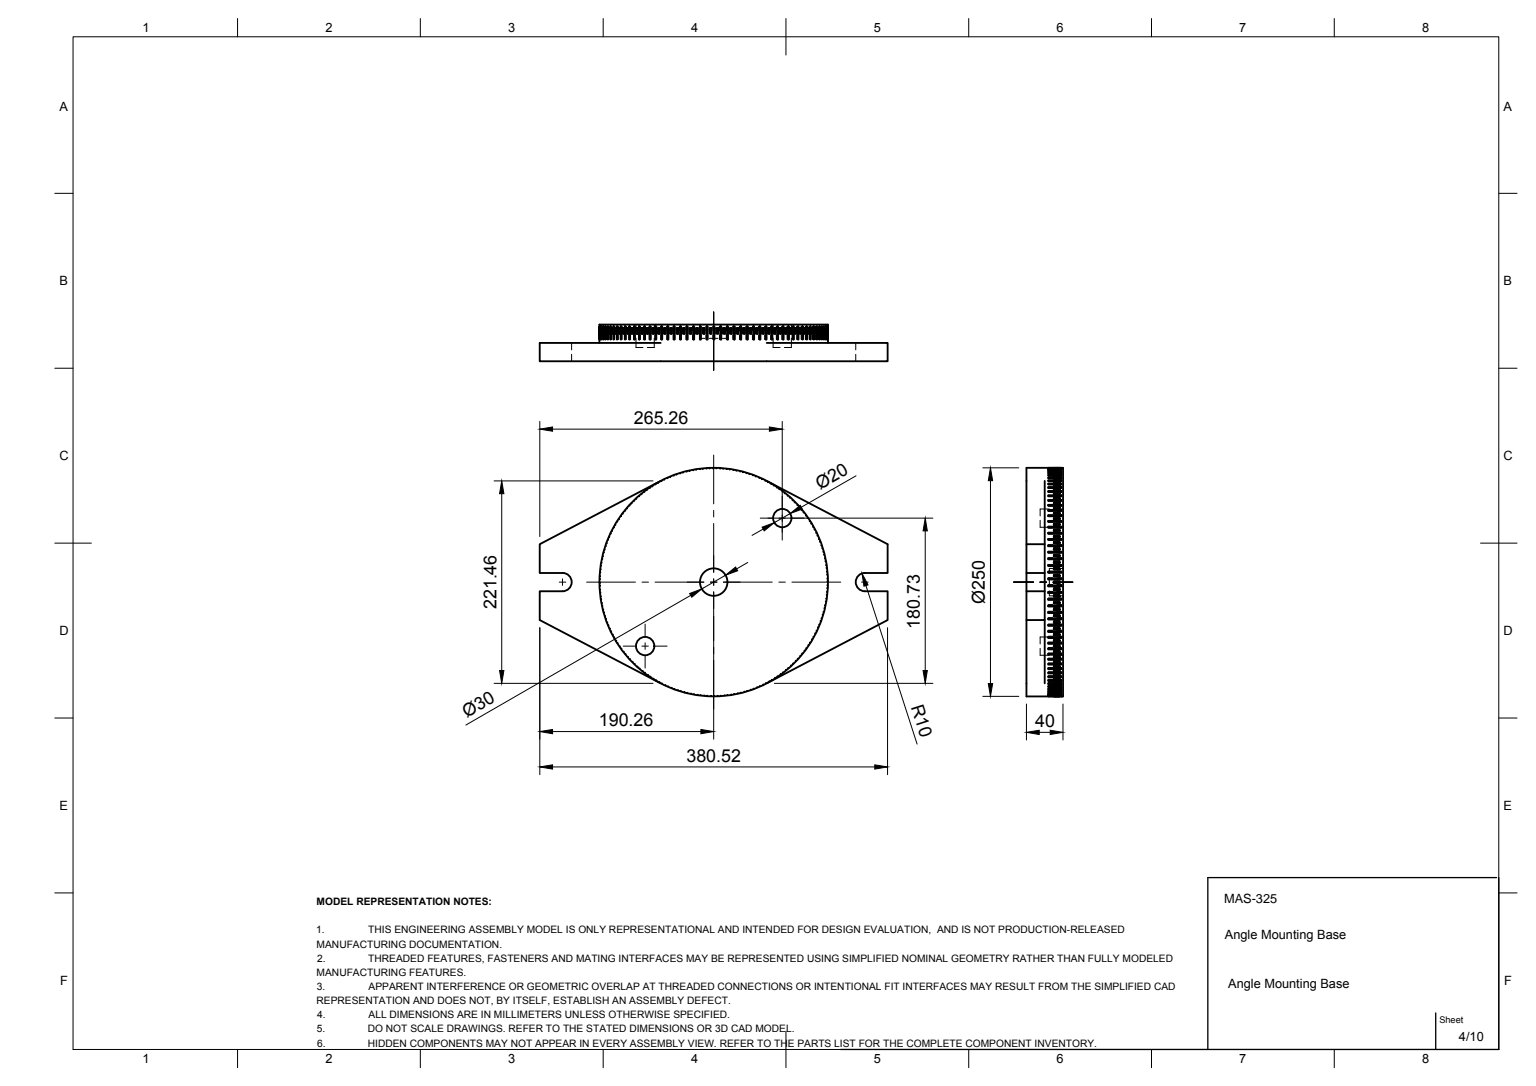
ISO-10303-21;
HEADER;
FILE_DESCRIPTION (('STEP AP214'),
    '1' );
FILE_NAME ('Angle Mounting Base.step',
    '2026-10-08T01:23:29',
    ( '' ),
    ( '' ),
    'SwSTEP 2.0',
    'SolidWorks 2025',
    '' );
FILE_SCHEMA (( 'AUTOMOTIVE_DESIGN' ));
ENDSEC;

DATA;
#2=FACE_OUTER_BOUND ( 'NONE', #26944, .T. ) ;
#3=VERTEX_POINT ( 'NONE', #17850 ) ;
#4=VERTEX_POINT ( 'NONE', #2063 ) ;
#5=EDGE_LOOP ( 'NONE', ( #45365, #39449, #49591, #6514 ) ) ;
#9=FACE_OUTER_BOUND ( 'NONE', #31225, .T. ) ;
#10=ORIENTED_EDGE ( 'NONE', *, *, #44040, .F. ) ;
#12=ORIENTED_EDGE ( 'NONE', *, *, #51700, .T. ) ;
#13=ORIENTED_EDGE ( 'NONE', *, *, #43268, .F. ) ;
#16=EDGE_CURVE ( 'NONE', #34125, #29247, #18107, .T. ) ;
#17=ADVANCED_FACE ( 'NONE', ( #34134 ), #14181, .T. ) ;
#18=ORIENTED_EDGE ( 'NONE', *, *, #15943, .T. ) ;
#19=AXIS2_PLACEMENT_3D ( 'NONE', #21420, #9597, #9087 ) ;
#21=EDGE_CURVE ( 'NONE', #1891, #35017, #9977, .T. ) ;
#22=CARTESIAN_POINT ( 'NONE',  ( -159.8192355313504720, -177.1207230881787780, -56.81883646197830018 ) ) ;
#24=CARTESIAN_POINT ( 'NONE',  ( -0.3054481938615447034, -177.1207230881787780, 115.3442529744090592 ) ) ;
#26=ORIENTED_EDGE ( 'NONE', *, *, #11216, .F. ) ;
#27=DIRECTION ( 'NONE',  ( -0.000000000000000000, 1.000000000000000000, -0.000000000000000000 ) ) ;
#28=EDGE_LOOP ( 'NONE', ( #8074, #9559, #4118, #19918 ) ) ;
#30=ORIENTED_EDGE ( 'NONE', *, *, #16889, .F. ) ;
#32=LINE ( 'NONE', #15292, #22958 ) ;
#33=CARTESIAN_POINT ( 'NONE',  ( -56.05401443572774411, -175.3837268820161057, 124.7702732086912931 ) ) ;
#34=CARTESIAN_POINT ( 'NONE',  ( 15.29189835570547551, -175.3837268820161057, 106.3450133598704213 ) ) ;
#35=VERTEX_POINT ( 'NONE', #9196 ) ;
#37=FACE_OUTER_BOUND ( 'NONE', #25266, .T. ) ;
#39=AXIS2_PLACEMENT_3D ( 'NONE', #35953, #36729, #8094 ) ;
#40=ORIENTED_EDGE ( 'NONE', *, *, #10845, .T. ) ;
#41=EDGE_CURVE ( 'NONE', #38866, #36143, #5787, .T. ) ;
#42=DIRECTION ( 'NONE',  ( -0.000000000000000000, 1.000000000000000000, -0.000000000000000000 ) ) ;
#44=DIRECTION ( 'NONE',  ( -0.8455960035018311727, 0.000000000000000000, 0.5338233779647826305 ) ) ;
#46=CARTESIAN_POINT ( 'NONE',  ( 63.31225588004632243, -183.6283474603465606, 55.92572546981597981 ) ) ;
#48=EDGE_CURVE ( 'NONE', #19235, #10210, #19545, .T. ) ;
#49=ORIENTED_EDGE ( 'NONE', *, *, #34843, .T. ) ;
#50=DIRECTION ( 'NONE',  ( -0.4031234292879665171, 0.000000000000000000, -0.9151456172430210145 ) ) ;
#51=ORIENTED_EDGE ( 'NONE', *, *, #6223, .F. ) ;
#53=CARTESIAN_POINT ( 'NONE',  ( -47.55243714407702527, -193.5000000000000000, 0.3758275821142491591 ) ) ;
#56=CARTESIAN_POINT ( 'NONE',  ( 74.95461934957533856, -175.3837268820161057, -11.83705339977243121 ) ) ;
#57=PLANE ( 'NONE',  #3915 ) ;
#58=CIRCLE ( 'NONE', #10119, 125.0000000000000000 ) ;
#61=LINE ( 'NONE', #8461, #49088 ) ;
#62=CARTESIAN_POINT ( 'NONE',  ( -135.4449840867448813, -193.5000000000000000, -88.39086586114740385 ) ) ;
#67=ORIENTED_EDGE ( 'NONE', *, *, #21766, .T. ) ;
#70=ORIENTED_EDGE ( 'NONE', *, *, #36153, .T. ) ;
#71=CARTESIAN_POINT ( 'NONE',  ( 74.13662511985246795, -189.7472609257535510, 18.47640724094593523 ) ) ;
#72=DIRECTION ( 'NONE',  ( 0.000000000000000000, 0.000000000000000000, 1.000000000000000000 ) ) ;
#73=EDGE_CURVE ( 'NONE', #1427, #18230, #29600, .T. ) ;
#74=CARTESIAN_POINT ( 'NONE',  ( -52.47502265695594303, -183.6283474603465606, -124.9361149384469627 ) ) ;
#75=DIRECTION ( 'NONE',  ( 0.000000000000000000, -0.000000000000000000, 1.000000000000000000 ) ) ;
#78=ORIENTED_EDGE ( 'NONE', *, *, #31301, .F. ) ;
#79=DIRECTION ( 'NONE',  ( -0.000000000000000000, 1.000000000000000000, -0.000000000000000000 ) ) ;
#80=DIRECTION ( 'NONE',  ( 0.6749830015182038956, 0.000000000000000000, 0.7378332790417333475 ) ) ;
#82=LINE ( 'NONE', #16386, #13659 ) ;
#83=FACE_OUTER_BOUND ( 'NONE', #49301, .T. ) ;
#85=DIRECTION ( 'NONE',  ( -0.000000000000000000, 1.000000000000000000, -0.000000000000000000 ) ) ;
#86=AXIS2_PLACEMENT_3D ( 'NONE', #8984, #303, #32633 ) ;
#88=CARTESIAN_POINT ( 'NONE',  ( -29.73468717939733708, -193.5000000000000000, 123.5865930638410930 ) ) ;
#89=DIRECTION ( 'NONE',  ( -0.2059786187411094538, 0.000000000000000000, 0.9785564922995017012 ) ) ;
#91=ORIENTED_EDGE ( 'NONE', *, *, #37914, .F. ) ;
#93=CARTESIAN_POINT ( 'NONE',  ( -171.9740864388383557, -189.7472609257535510, -11.18012358327903577 ) ) ;
#94=DIRECTION ( 'NONE',  ( -0.8757349421956412971, 0.000000000000000000, 0.4827922027307366970 ) ) ;
#97=LINE ( 'NONE', #16919, #528 ) ;
#98=DIRECTION ( 'NONE',  ( -0.9982437317643214625, 0.000000000000000000, -0.05924062789371441901 ) ) ;
#99=CARTESIAN_POINT ( 'NONE',  ( 141.7825277784304205, -193.5000000000000000, -9.999999999999987566 ) ) ;
#100=ORIENTED_EDGE ( 'NONE', *, *, #32040, .F. ) ;
#101=LINE ( 'NONE', #40291, #9133 ) ;
#102=ORIENTED_EDGE ( 'NONE', *, *, #46111, .F. ) ;
#105=LINE ( 'NONE', #39778, #22073 ) ;
#106=FACE_BOUND ( 'NONE', #42826, .T. ) ;
#108=DIRECTION ( 'NONE',  ( -0.1768902751225802927, 0.000000000000000000, 0.9842305779475953864 ) ) ;
#109=ORIENTED_EDGE ( 'NONE', *, *, #36766, .T. ) ;
#111=DIRECTION ( 'NONE',  ( 0.9785564922995032555, 0.000000000000000000, 0.2059786187411021818 ) ) ;
#112=DIRECTION ( 'NONE',  ( 0.000000000000000000, -1.000000000000000000, 0.000000000000000000 ) ) ;
#113=EDGE_CURVE ( 'NONE', #39629, #40896, #21795, .T. ) ;
#115=EDGE_LOOP ( 'NONE', ( #6615, #26573, #34341, #46200 ) ) ;
#116=CARTESIAN_POINT ( 'NONE',  ( -162.3451783319732726, -183.6283474603465606, 51.57055649762781968 ) ) ;
#117=VERTEX_POINT ( 'NONE', #22299 ) ;
#118=EDGE_LOOP ( 'NONE', ( #5505, #7567, #35660, #29019 ) ) ;
#119=CARTESIAN_POINT ( 'NONE',  ( -47.97059563285962724, -189.7472609257535510, -0.8610436117673480050 ) ) ;
#120=DIRECTION ( 'NONE',  ( 0.000000000000000000, 0.000000000000000000, -1.000000000000000000 ) ) ;
#121=VERTEX_POINT ( 'NONE', #29930 ) ;
#122=VECTOR ( 'NONE', #5953, 1000.000000000000000 ) ;
#123=ORIENTED_EDGE ( 'NONE', *, *, #8914, .F. ) ;
#124=CARTESIAN_POINT ( 'NONE',  ( 76.04209377433248562, -193.5000000000000000, -10.93003379476866677 ) ) ;
#125=CIRCLE ( 'NONE', #14436, 125.0000000000000000 ) ;
#126=AXIS2_PLACEMENT_3D ( 'NONE', #20035, #19509, #35530 ) ;
#127=EDGE_CURVE ( 'NONE', #48981, #10059, #6022, .T. ) ;
#128=CARTESIAN_POINT ( 'NONE',  ( 23.33927677392131628, -183.6283474603465606, -102.3089288139528747 ) ) ;
#130=FACE_OUTER_BOUND ( 'NONE', #50584, .T. ) ;
#131=FACE_OUTER_BOUND ( 'NONE', #2320, .T. ) ;
#134=DIRECTION ( 'NONE',  ( 0.000000000000000000, 0.000000000000000000, -1.000000000000000000 ) ) ;
#138=VERTEX_POINT ( 'NONE', #51213 ) ;
#140=EDGE_CURVE ( 'NONE', #35696, #40857, #2842, .T. ) ;
#142=FACE_OUTER_BOUND ( 'NONE', #28523, .T. ) ;
#143=FACE_OUTER_BOUND ( 'NONE', #34738, .T. ) ;
#145=AXIS2_PLACEMENT_3D ( 'NONE', #44882, #32531, #8363 ) ;
#148=CARTESIAN_POINT ( 'NONE',  ( -49.42645310536303782, -193.5000000000000000, -0.3202698538628417357 ) ) ;
#150=VERTEX_POINT ( 'NONE', #38840 ) ;
#151=DIRECTION ( 'NONE',  ( 0.000000000000000000, -0.000000000000000000, 1.000000000000000000 ) ) ;
#152=ORIENTED_EDGE ( 'NONE', *, *, #45435, .F. ) ;
#157=VECTOR ( 'NONE', #9488, 1000.000000000000000 ) ;
#159=CARTESIAN_POINT ( 'NONE',  ( -84.53143451966467126, -175.3837268820161057, -118.6432945265036807 ) ) ;
#162=AXIS2_PLACEMENT_3D ( 'NONE', #7997, #20089, #36113 ) ;
#163=ORIENTED_EDGE ( 'NONE', *, *, #20136, .T. ) ;
#165=ORIENTED_EDGE ( 'NONE', *, *, #4140, .T. ) ;
#166=DIRECTION ( 'NONE',  ( 0.000000000000000000, -0.000000000000000000, 1.000000000000000000 ) ) ;
#167=CARTESIAN_POINT ( 'NONE',  ( -139.0630283577175987, -193.5000000000000000, -86.13684908212448477 ) ) ;
#168=CARTESIAN_POINT ( 'NONE',  ( -15.24927435600541692, -177.1207230881787780, 120.5021863277719234 ) ) ;
#170=CARTESIAN_POINT ( 'NONE',  ( -144.0067397530739299, -183.6283474603465606, -80.61932246194588458 ) ) ;
#171=CARTESIAN_POINT ( 'NONE',  ( -41.24387117724851493, -189.7472609257535510, 124.7904286264581231 ) ) ;
#172=VERTEX_POINT ( 'NONE', #26760 ) ;
#173=DIRECTION ( 'NONE',  ( -0.8896570909947467687, 0.000000000000000000, -0.4566292373937140270 ) ) ;
#174=CARTESIAN_POINT ( 'NONE',  ( -134.9734323446613473, -175.3837268820161057, 88.85232316304892208 ) ) ;
#175=CIRCLE ( 'NONE', #31206, 125.0000000000000000 ) ;
#176=FACE_BOUND ( 'NONE', #45465, .T. ) ;
#177=VERTEX_POINT ( 'NONE', #42529 ) ;
#180=DIRECTION ( 'NONE',  ( -0.000000000000000000, 1.000000000000000000, -0.000000000000000000 ) ) ;
#183=ORIENTED_EDGE ( 'NONE', *, *, #47786, .F. ) ;
#185=DIRECTION ( 'NONE',  ( 0.4827922027307366970, 0.000000000000000000, 0.8757349421956412971 ) ) ;
#187=CARTESIAN_POINT ( 'NONE',  ( -148.0127667507368585, -183.6283474603465606, -75.61781872352626976 ) ) ;
#188=CARTESIAN_POINT ( 'NONE',  ( -48.47912675150885065, -193.5000000000000000, 6.938893903907228378E-15 ) ) ;
#189=DIRECTION ( 'NONE',  ( 0.000000000000000000, 0.000000000000000000, 1.000000000000000000 ) ) ;
#192=ADVANCED_FACE ( 'NONE', ( #46484 ), #50954, .F. ) ;
#193=FACE_OUTER_BOUND ( 'NONE', #27346, .T. ) ;
#194=VERTEX_POINT ( 'NONE', #14955 ) ;
#195=EDGE_CURVE ( 'NONE', #34486, #40282, #15361, .T. ) ;
#202=EDGE_CURVE ( 'NONE', #8838, #28521, #30963, .T. ) ;
#203=AXIS2_PLACEMENT_3D ( 'NONE', #1568, #37299, #37818 ) ;
#204=AXIS2_PLACEMENT_3D ( 'NONE', #4568, #29258, #44511 ) ;
#205=CARTESIAN_POINT ( 'NONE',  ( -157.8637630444124795, -175.3837268820161057, -60.49794494914009135 ) ) ;
#207=ORIENTED_EDGE ( 'NONE', *, *, #866, .T. ) ;
#209=DIRECTION ( 'NONE',  ( 0.000000000000000000, 0.000000000000000000, 1.000000000000000000 ) ) ;
#210=VERTEX_POINT ( 'NONE', #34890 ) ;
#211=AXIS2_PLACEMENT_3D ( 'NONE', #44344, #36428, #28543 ) ;
#212=AXIS2_PLACEMENT_3D ( 'NONE', #15523, #6858, #2909 ) ;
#213=EDGE_LOOP ( 'NONE', ( #16091, #33158, #8108, #2239 ) ) ;
#215=ORIENTED_EDGE ( 'NONE', *, *, #9578, .T. ) ;
#219=DIRECTION ( 'NONE',  ( 0.000000000000000000, 1.000000000000000000, 0.000000000000000000 ) ) ;
#220=ORIENTED_EDGE ( 'NONE', *, *, #16410, .F. ) ;
#223=ORIENTED_EDGE ( 'NONE', *, *, #649, .T. ) ;
#224=ORIENTED_EDGE ( 'NONE', *, *, #48940, .F. ) ;
#225=FACE_OUTER_BOUND ( 'NONE', #49522, .T. ) ;
#226=DIRECTION ( 'NONE',  ( -0.9890401873221633666, 0.000000000000000000, -0.1476465640024850756 ) ) ;
#227=FACE_OUTER_BOUND ( 'NONE', #2223, .T. ) ;
#229=FACE_OUTER_BOUND ( 'NONE', #4833, .T. ) ;
#230=CIRCLE ( 'NONE', #6149, 125.0000000000000000 ) ;
#234=CARTESIAN_POINT ( 'NONE',  ( -47.82630463331833681, -177.1207230881787780, 0.7575112421616305713 ) ) ;
#236=ADVANCED_FACE ( 'NONE', ( #38589 ), #47005, .T. ) ;
#238=ORIENTED_EDGE ( 'NONE', *, *, #26470, .F. ) ;
#239=CARTESIAN_POINT ( 'NONE',  ( 74.49773146996551532, -183.6283474603465606, -22.39848972532281834 ) ) ;
#241=FACE_OUTER_BOUND ( 'NONE', #10500, .T. ) ;
#243=EDGE_CURVE ( 'NONE', #48355, #27011, #50682, .T. ) ;
#244=ORIENTED_EDGE ( 'NONE', *, *, #45271, .T. ) ;
#245=EDGE_CURVE ( 'NONE', #35901, #35187, #7056, .T. ) ;
#246=VERTEX_POINT ( 'NONE', #50438 ) ;
#247=CIRCLE ( 'NONE', #6976, 125.0000000000000000 ) ;
#248=EDGE_LOOP ( 'NONE', ( #15059, #26707, #42311, #35212 ) ) ;
#249=CIRCLE ( 'NONE', #45592, 125.0000000000000000 ) ;
#251=LINE ( 'NONE', #40705, #46952 ) ;
#252=AXIS2_PLACEMENT_3D ( 'NONE', #33154, #25277, #24755 ) ;
#253=ADVANCED_FACE ( 'NONE', ( #3105 ), #7314, .F. ) ;
#255=CARTESIAN_POINT ( 'NONE',  ( -157.8637630444124795, -175.3837268820161057, -60.49794494914009846 ) ) ;
#257=EDGE_LOOP ( 'NONE', ( #21171, #20586, #46600, #11240 ) ) ;
#258=AXIS2_PLACEMENT_3D ( 'NONE', #32515, #48563, #24621 ) ;
#263=ORIENTED_EDGE ( 'NONE', *, *, #26885, .T. ) ;
#265=VERTEX_POINT ( 'NONE', #44078 ) ;
#266=CARTESIAN_POINT ( 'NONE',  ( -111.6834028793037987, -175.3837268820161057, 106.6827995071088253 ) ) ;
#267=VECTOR ( 'NONE', #9756, 1000.000000000000000 ) ;
#268=EDGE_CURVE ( 'NONE', #19322, #4539, #40375, .T. ) ;
#270=ADVANCED_FACE ( 'NONE', ( #39602 ), #440, .T. ) ;
#271=AXIS2_PLACEMENT_3D ( 'NONE', #37551, #38049, #18093 ) ;
#272=CARTESIAN_POINT ( 'NONE',  ( -102.9981419485577732, -193.5000000000000000, -111.3726929437936377 ) ) ;
#273=LINE ( 'NONE', #29176, #44951 ) ;
#274=DIRECTION ( 'NONE',  ( -0.6300878435817094392, 0.000000000000000000, -0.7765238627180437447 ) ) ;
#275=DIRECTION ( 'NONE',  ( 0.000000000000000000, 0.000000000000000000, -1.000000000000000000 ) ) ;
#278=ORIENTED_EDGE ( 'NONE', *, *, #14380, .F. ) ;
#280=ORIENTED_EDGE ( 'NONE', *, *, #40635, .T. ) ;
#281=DIRECTION ( 'NONE',  ( 0.000000000000000000, 0.000000000000000000, 1.000000000000000000 ) ) ;
#282=CARTESIAN_POINT ( 'NONE',  ( -117.6201219941651601, -193.5000000000000000, 104.1370384486469902 ) ) ;
#283=DIRECTION ( 'NONE',  ( 0.9785564922995060311, 0.000000000000000000, -0.2059786187410889424 ) ) ;
#285=VECTOR ( 'NONE', #4558, 999.9999999999998863 ) ;
#287=EDGE_LOOP ( 'NONE', ( #13570, #29381, #45686, #19106 ) ) ;
#291=( NAMED_UNIT ( * ) SI_UNIT ( $, .STERADIAN. ) SOLID_ANGLE_UNIT ( ) );
#292=ORIENTED_EDGE ( 'NONE', *, *, #4293, .T. ) ;
#293=DIRECTION ( 'NONE',  ( -0.7378332790417285736, 0.000000000000000000, 0.6749830015182091136 ) ) ;
#294=DIRECTION ( 'NONE',  ( 0.000000000000000000, 1.000000000000000000, 0.000000000000000000 ) ) ;
#297=PLANE ( 'NONE',  #12496 ) ;
#299=ORIENTED_EDGE ( 'NONE', *, *, #48513, .F. ) ;
#300=DIRECTION ( 'NONE',  ( -0.000000000000000000, 1.000000000000000000, -0.000000000000000000 ) ) ;
#302=LINE ( 'NONE', #51846, #44972 ) ;
#303=DIRECTION ( 'NONE',  ( 0.000000000000000000, -1.000000000000000000, -0.000000000000000000 ) ) ;
#307=DIRECTION ( 'NONE',  ( 0.000000000000000000, 1.000000000000000000, 0.000000000000000000 ) ) ;
#309=ADVANCED_FACE ( 'NONE', ( #15976 ), #8082, .T. ) ;
#310=AXIS2_PLACEMENT_3D ( 'NONE', #50252, #42607, #38132 ) ;
#311=EDGE_CURVE ( 'NONE', #37290, #775, #44603, .T. ) ;
#312=DIRECTION ( 'NONE',  ( -0.000000000000000000, 1.000000000000000000, -0.000000000000000000 ) ) ;
#313=EDGE_CURVE ( 'NONE', #8692, #47336, #37219, .T. ) ;
#317=EDGE_LOOP ( 'NONE', ( #32171, #36986, #20388, #10523 ) ) ;
#318=EDGE_LOOP ( 'NONE', ( #38235, #13867, #475, #2486 ) ) ;
#319=CARTESIAN_POINT ( 'NONE',  ( 52.36832552120769435, -189.7472609257535510, -72.15117186584490128 ) ) ;
#320=CARTESIAN_POINT ( 'NONE',  ( -41.24387117724851493, -189.7472609257535510, 124.7904286264581231 ) ) ;
#321=EDGE_LOOP ( 'NONE', ( #34166, #26853, #15993, #21976 ) ) ;
#322=EDGE_LOOP ( 'NONE', ( #10542, #48454, #37812, #15490 ) ) ;
#323=EDGE_CURVE ( 'NONE', #36975, #28008, #47779, .T. ) ;
#324=ORIENTED_EDGE ( 'NONE', *, *, #11588, .T. ) ;
#326=DIRECTION ( 'NONE',  ( 0.000000000000000000, 0.000000000000000000, 1.000000000000000000 ) ) ;
#327=CARTESIAN_POINT ( 'NONE',  ( -66.64622755927948106, -193.5000000000000000, 123.6727797384707515 ) ) ;
#328=ORIENTED_EDGE ( 'NONE', *, *, #49475, .F. ) ;
#330=EDGE_CURVE ( 'NONE', #27930, #47785, #15401, .T. ) ;
#331=ORIENTED_EDGE ( 'NONE', *, *, #18307, .T. ) ;
#332=DIRECTION ( 'NONE',  ( 0.000000000000000000, 0.000000000000000000, -1.000000000000000000 ) ) ;
#334=DIRECTION ( 'NONE',  ( 0.000000000000000000, -1.000000000000000000, 0.000000000000000000 ) ) ;
#335=EDGE_LOOP ( 'NONE', ( #354, #13466, #39178, #31091 ) ) ;
#337=CARTESIAN_POINT ( 'NONE',  ( -84.19171550243321178, -175.3837268820161057, 119.7898618611247485 ) ) ;
#341=VECTOR ( 'NONE', #5496, 1000.000000000000000 ) ;
#342=DIRECTION ( 'NONE',  ( 0.000000000000000000, 0.000000000000000000, -1.000000000000000000 ) ) ;
#345=VECTOR ( 'NONE', #6207, 1000.000000000000000 ) ;
#346=VERTEX_POINT ( 'NONE', #3887 ) ;
#347=ORIENTED_EDGE ( 'NONE', *, *, #7630, .T. ) ;
#348=EDGE_LOOP ( 'NONE', ( #40499, #34840, #43093, #48028 ) ) ;
#351=ORIENTED_EDGE ( 'NONE', *, *, #10876, .T. ) ;
#352=DIRECTION ( 'NONE',  ( 0.000000000000000000, 0.000000000000000000, 1.000000000000000000 ) ) ;
#354=ORIENTED_EDGE ( 'NONE', *, *, #40714, .F. ) ;
#355=CARTESIAN_POINT ( 'NONE',  ( -59.28786813212836648, -183.6283474603465606, 124.5318076226587465 ) ) ;
#357=CARTESIAN_POINT ( 'NONE',  ( 27.50603775690333563, -175.3837268820161057, -99.25348746834811209 ) ) ;
#360=ORIENTED_EDGE ( 'NONE', *, *, #30567, .T. ) ;
#361=FACE_BOUND ( 'NONE', #24793, .T. ) ;
#362=DIRECTION ( 'NONE',  ( 0.000000000000000000, -1.000000000000000000, 0.000000000000000000 ) ) ;
#363=ORIENTED_EDGE ( 'NONE', *, *, #47489, .F. ) ;
#370=ORIENTED_EDGE ( 'NONE', *, *, #34030, .F. ) ;
#375=DIRECTION ( 'NONE',  ( -0.000000000000000000, 1.000000000000000000, -0.000000000000000000 ) ) ;
#377=CIRCLE ( 'NONE', #16331, 125.0000000000000000 ) ;
#380=CARTESIAN_POINT ( 'NONE',  ( 67.66641500972446011, -193.5000000000000000, 46.20836643931067300 ) ) ;
#381=AXIS2_PLACEMENT_3D ( 'NONE', #38755, #31139, #39013 ) ;
#382=CARTESIAN_POINT ( 'NONE',  ( 67.29303306501927295, -175.3837268820161057, 47.13604789772129777 ) ) ;
#384=LINE ( 'NONE', #24315, #19709 ) ;
#385=EDGE_CURVE ( 'NONE', #3976, #38174, #2777, .T. ) ;
#388=PLANE ( 'NONE',  #37573 ) ;
#389=DIRECTION ( 'NONE',  ( -0.4566292373937018145, 0.000000000000000000, -0.8896570909947529859 ) ) ;
#390=AXIS2_PLACEMENT_3D ( 'NONE', #5869, #10563, #18713 ) ;
#391=LINE ( 'NONE', #24573, #45885 ) ;
#393=ORIENTED_EDGE ( 'NONE', *, *, #9573, .T. ) ;
#394=EDGE_CURVE ( 'NONE', #38668, #51204, #28813, .T. ) ;
#396=DIRECTION ( 'NONE',  ( -0.000000000000000000, 1.000000000000000000, -0.000000000000000000 ) ) ;
#397=CARTESIAN_POINT ( 'NONE',  ( -105.4063847101408840, -189.7472609257535510, -111.2847127925096657 ) ) ;
#404=DIRECTION ( 'NONE',  ( 0.000000000000000000, -0.000000000000000000, -1.000000000000000000 ) ) ;
#405=ORIENTED_EDGE ( 'NONE', *, *, #47135, .T. ) ;
#406=ORIENTED_EDGE ( 'NONE', *, *, #20390, .F. ) ;
#408=DIRECTION ( 'NONE',  ( 0.000000000000000000, 0.000000000000000000, -1.000000000000000000 ) ) ;
#409=DIRECTION ( 'NONE',  ( -0.000000000000000000, 1.000000000000000000, -0.000000000000000000 ) ) ;
#410=VECTOR ( 'NONE', #3277, 1000.000000000000000 ) ;
#411=VECTOR ( 'NONE', #28290, 1000.000000000000114 ) ;
#413=CARTESIAN_POINT ( 'NONE',  ( 61.38599058177058510, -189.7472609257535510, 59.62093586438192716 ) ) ;
#414=ORIENTED_EDGE ( 'NONE', *, *, #28899, .F. ) ;
#415=CARTESIAN_POINT ( 'NONE',  ( -161.6832731452239500, -175.3837268820161057, -53.00774697410101055 ) ) ;
#416=ORIENTED_EDGE ( 'NONE', *, *, #12405, .T. ) ;
#417=AXIS2_PLACEMENT_3D ( 'NONE', #40245, #307, #23211 ) ;
#418=ADVANCED_FACE ( 'NONE', ( #4154 ), #32244, .T. ) ;
#419=ORIENTED_EDGE ( 'NONE', *, *, #11216, .T. ) ;
#420=CARTESIAN_POINT ( 'NONE',  ( -58.17235712592530916, -183.6283474603465606, 123.6213615703899649 ) ) ;
#421=AXIS2_PLACEMENT_3D ( 'NONE', #37260, #26195, #17811 ) ;
#423=PLANE ( 'NONE',  #17324 ) ;
#424=VECTOR ( 'NONE', #5391, 999.9999999999998863 ) ;
#425=DIRECTION ( 'NONE',  ( 0.000000000000000000, -1.000000000000000000, 0.000000000000000000 ) ) ;
#426=DIRECTION ( 'NONE',  ( 0.000000000000000000, -1.000000000000000000, 0.000000000000000000 ) ) ;
#427=CARTESIAN_POINT ( 'NONE',  ( -172.9089226952081617, -175.3837268820161057, 11.92584929509620117 ) ) ;
#429=ORIENTED_EDGE ( 'NONE', *, *, #25783, .T. ) ;
#430=VECTOR ( 'NONE', #3916, 1000.000000000000227 ) ;
#432=DIRECTION ( 'NONE',  ( -0.6528221181905227155, 0.000000000000000000, 0.7575112421616191360 ) ) ;
#433=AXIS2_PLACEMENT_3D ( 'NONE', #44101, #16519, #40659 ) ;
#434=FACE_BOUND ( 'NONE', #5358, .T. ) ;
#435=ORIENTED_EDGE ( 'NONE', *, *, #51093, .T. ) ;
#436=EDGE_CURVE ( 'NONE', #23558, #41176, #21468, .T. ) ;
#437=DIRECTION ( 'NONE',  ( -0.000000000000000000, 1.000000000000000000, -0.000000000000000000 ) ) ;
#439=EDGE_LOOP ( 'NONE', ( #48444, #5234, #33273, #2136 ) ) ;
#440=PLANE ( 'NONE',  #29634 ) ;
#441=ORIENTED_EDGE ( 'NONE', *, *, #34593, .F. ) ;
#442=LINE ( 'NONE', #40137, #35182 ) ;
#444=FACE_BOUND ( 'NONE', #2815, .T. ) ;
#447=EDGE_CURVE ( 'NONE', #41848, #50197, #50115, .T. ) ;
#450=DIRECTION ( 'NONE',  ( -0.000000000000000000, 1.000000000000000000, -0.000000000000000000 ) ) ;
#451=ORIENTED_EDGE ( 'NONE', *, *, #12405, .F. ) ;
#452=ORIENTED_EDGE ( 'NONE', *, *, #45255, .T. ) ;
#454=ORIENTED_EDGE ( 'NONE', *, *, #27223, .T. ) ;
#455=CIRCLE ( 'NONE', #14742, 125.0000000000000000 ) ;
#457=VECTOR ( 'NONE', #6292, 1000.000000000000000 ) ;
#459=LINE ( 'NONE', #16516, #47341 ) ;
#460=CIRCLE ( 'NONE', #37427, 125.0000000000000000 ) ;
#461=VECTOR ( 'NONE', #50848, 1000.000000000000000 ) ;
#462=DIRECTION ( 'NONE',  ( -0.000000000000000000, 1.000000000000000000, -0.000000000000000000 ) ) ;
#463=ORIENTED_EDGE ( 'NONE', *, *, #19689, .T. ) ;
#464=LINE ( 'NONE', #17047, #51738 ) ;
#465=DIRECTION ( 'NONE',  ( -0.000000000000000000, 1.000000000000000000, -0.000000000000000000 ) ) ;
#466=ORIENTED_EDGE ( 'NONE', *, *, #5475, .F. ) ;
#467=VERTEX_POINT ( 'NONE', #40910 ) ;
#468=DIRECTION ( 'NONE',  ( 0.000000000000000000, 0.000000000000000000, 1.000000000000000000 ) ) ;
#470=LINE ( 'NONE', #12822, #33168 ) ;
#471=VERTEX_POINT ( 'NONE', #25411 ) ;
#472=EDGE_CURVE ( 'NONE', #25437, #18236, #29078, .T. ) ;
#474=DIRECTION ( 'NONE',  ( 0.000000000000000000, 1.000000000000000000, 0.000000000000000000 ) ) ;
#475=ORIENTED_EDGE ( 'NONE', *, *, #47971, .T. ) ;
#476=CARTESIAN_POINT ( 'NONE',  ( -111.3904503173946523, -193.5000000000000000, -106.8558168688113312 ) ) ;
#477=CARTESIAN_POINT ( 'NONE',  ( -171.2727421180348415, -193.5000000000000000, 23.38221600314377113 ) ) ;
#478=ORIENTED_EDGE ( 'NONE', *, *, #41754, .F. ) ;
#480=DIRECTION ( 'NONE',  ( -0.9982437317643222396, 0.000000000000000000, 0.05924062789370006937 ) ) ;
#481=PLANE ( 'NONE',  #41527 ) ;
#482=DIRECTION ( 'NONE',  ( 0.000000000000000000, 0.000000000000000000, 1.000000000000000000 ) ) ;
#484=DIRECTION ( 'NONE',  ( -0.000000000000000000, 1.000000000000000000, 0.000000000000000000 ) ) ;
#485=AXIS2_PLACEMENT_3D ( 'NONE', #11794, #47566, #31787 ) ;
#486=PLANE ( 'NONE',  #22221 ) ;
#487=VECTOR ( 'NONE', #43426, 1000.000000000000000 ) ;
#489=DIRECTION ( 'NONE',  ( 0.000000000000000000, 0.000000000000000000, -1.000000000000000000 ) ) ;
#490=EDGE_CURVE ( 'NONE', #1315, #121, #1960, .T. ) ;
#492=LINE ( 'NONE', #31262, #6402 ) ;
#493=EDGE_CURVE ( 'NONE', #46777, #16167, #41946, .T. ) ;
#494=DIRECTION ( 'NONE',  ( 0.7378332790417285736, 0.000000000000000000, -0.6749830015182091136 ) ) ;
#496=EDGE_LOOP ( 'NONE', ( #18205, #42343, #51625, #42919 ) ) ;
#498=DIRECTION ( 'NONE',  ( 0.7175072570443249420, 0.000000000000000000, 0.6965510290630033685 ) ) ;
#501=CARTESIAN_POINT ( 'NONE',  ( -47.51449116960048968, -175.3837268820161057, 0.2635871660690785045 ) ) ;
#502=CARTESIAN_POINT ( 'NONE',  ( 3.652658254809377336, -183.6283474603465606, -112.5098962032389522 ) ) ;
#503=VERTEX_POINT ( 'NONE', #45393 ) ;
#507=AXIS2_PLACEMENT_3D ( 'NONE', #38992, #47165, #35568 ) ;
#508=LINE ( 'NONE', #40199, #762 ) ;
#512=VERTEX_POINT ( 'NONE', #41693 ) ;
#514=DIRECTION ( 'NONE',  ( -0.000000000000000000, 1.000000000000000000, -0.000000000000000000 ) ) ;
#515=EDGE_LOOP ( 'NONE', ( #35303, #20587, #15349, #40172 ) ) ;
#516=DIRECTION ( 'NONE',  ( -0.000000000000000000, 1.000000000000000000, -0.000000000000000000 ) ) ;
#517=ORIENTED_EDGE ( 'NONE', *, *, #50630, .F. ) ;
#518=AXIS2_PLACEMENT_3D ( 'NONE', #30428, #18860, #10727 ) ;
#520=EDGE_LOOP ( 'NONE', ( #44694, #25345, #12703, #2844 ) ) ;
#523=CARTESIAN_POINT ( 'NONE',  ( -48.65601702663143868, -175.3837268820161057, 0.9842305779476024918 ) ) ;
#524=DIRECTION ( 'NONE',  ( 0.000000000000000000, 1.000000000000000000, 0.000000000000000000 ) ) ;
#525=DIRECTION ( 'NONE',  ( 0.9564009842765244240, 0.000000000000000000, -0.2920567706369695538 ) ) ;
#528=VECTOR ( 'NONE', #5098, 1000.000000000000000 ) ;
#530=VECTOR ( 'NONE', #17595, 1000.000000000000114 ) ;
#532=VECTOR ( 'NONE', #16412, 1000.000000000000000 ) ;
#533=ORIENTED_EDGE ( 'NONE', *, *, #2819, .F. ) ;
#535=CARTESIAN_POINT ( 'NONE',  ( -48.47912675150885065, -177.1207230881787780, 6.938893903907228378E-15 ) ) ;
#537=EDGE_CURVE ( 'NONE', #48832, #33712, #33804, .T. ) ;
#540=CYLINDRICAL_SURFACE ( 'NONE', #26625, 125.0000000000000000 ) ;
#541=CIRCLE ( 'NONE', #34986, 125.0000000000000000 ) ;
#542=PLANE ( 'NONE',  #18314 ) ;
#543=PLANE ( 'NONE',  #42489 ) ;
#545=ORIENTED_EDGE ( 'NONE', *, *, #18432, .T. ) ;
#546=ADVANCED_FACE ( 'NONE', ( #5447 ), #41169, .F. ) ;
#547=AXIS2_PLACEMENT_3D ( 'NONE', #8240, #28457, #27946 ) ;
#550=DIRECTION ( 'NONE',  ( -0.000000000000000000, -1.000000000000000000, 0.000000000000000000 ) ) ;
#551=ORIENTED_EDGE ( 'NONE', *, *, #41443, .F. ) ;
#553=CARTESIAN_POINT ( 'NONE',  ( -47.82630463331833681, -175.3837268820161057, 0.7575112421616305713 ) ) ;
#554=CARTESIAN_POINT ( 'NONE',  ( -59.86929868745811945, -183.6283474603465606, -124.4799742258549458 ) ) ;
#555=EDGE_CURVE ( 'NONE', #9556, #9203, #5961, .T. ) ;
#556=DIRECTION ( 'NONE',  ( 0.8455960035018234011, 0.000000000000000000, 0.5338233779647948429 ) ) ;
#558=CARTESIAN_POINT ( 'NONE',  ( -165.2002711502080672, -177.1207230881787780, 44.73448837594998651 ) ) ;
#560=DIRECTION ( 'NONE',  ( 0.000000000000000000, -1.000000000000000000, 0.000000000000000000 ) ) ;
#561=ADVANCED_FACE ( 'NONE', ( #17273 ), #45651, .T. ) ;
#562=ADVANCED_FACE ( 'NONE', ( #30126 ), #20957, .T. ) ;
#563=VERTEX_POINT ( 'NONE', #10148 ) ;
#564=DIRECTION ( 'NONE',  ( 0.000000000000000000, 0.000000000000000000, -1.000000000000000000 ) ) ;
#565=ORIENTED_EDGE ( 'NONE', *, *, #9989, .F. ) ;
#568=EDGE_CURVE ( 'NONE', #13340, #30763, #46948, .T. ) ;
#570=DIRECTION ( 'NONE',  ( -0.000000000000000000, 1.000000000000000000, -0.000000000000000000 ) ) ;
#571=AXIS2_PLACEMENT_3D ( 'NONE', #47908, #11884, #19515 ) ;
#572=EDGE_CURVE ( 'NONE', #18675, #17957, #26165, .T. ) ;
#573=DIRECTION ( 'NONE',  ( 0.4566292373937077542, 0.000000000000000000, 0.8896570909947499883 ) ) ;
#574=LINE ( 'NONE', #20541, #13865 ) ;
#576=DIRECTION ( 'NONE',  ( 0.000000000000000000, 0.000000000000000000, -1.000000000000000000 ) ) ;
#577=VECTOR ( 'NONE', #4041, 1000.000000000000000 ) ;
#581=ORIENTED_EDGE ( 'NONE', *, *, #32751, .F. ) ;
#583=AXIS2_PLACEMENT_3D ( 'NONE', #26617, #42121, #49770 ) ;
#585=CARTESIAN_POINT ( 'NONE',  ( -116.2964108826154330, -193.5000000000000000, -105.0038855142073260 ) ) ;
#586=AXIS2_PLACEMENT_3D ( 'NONE', #20301, #16649, #32387 ) ;
#588=AXIS2_PLACEMENT_3D ( 'NONE', #26268, #42293, #6829 ) ;
#589=LINE ( 'NONE', #24496, #50635 ) ;
#591=ORIENTED_EDGE ( 'NONE', *, *, #49335, .F. ) ;
#592=EDGE_LOOP ( 'NONE', ( #44540, #11697, #28068, #50995 ) ) ;
#593=DIRECTION ( 'NONE',  ( 0.9473263538541899509, 0.000000000000000000, 0.3202698538628415692 ) ) ;
#594=CARTESIAN_POINT ( 'NONE',  ( 76.28370911321322012, -177.1207230881787780, -7.696413904697510411 ) ) ;
#596=ORIENTED_EDGE ( 'NONE', *, *, #42681, .F. ) ;
#597=ADVANCED_FACE ( 'NONE', ( #6737 ), #50883, .T. ) ;
#598=DIRECTION ( 'NONE',  ( -0.000000000000000000, 1.000000000000000000, -0.000000000000000000 ) ) ;
#599=DIRECTION ( 'NONE',  ( -0.000000000000000000, 1.000000000000000000, -0.000000000000000000 ) ) ;
#600=VECTOR ( 'NONE', #9609, 1000.000000000000000 ) ;
#601=FACE_OUTER_BOUND ( 'NONE', #39994, .T. ) ;
#602=VERTEX_POINT ( 'NONE', #27200 ) ;
#603=CIRCLE ( 'NONE', #46761, 125.0000000000000000 ) ;
#604=DIRECTION ( 'NONE',  ( -0.9960498426152158968, 0.000000000000000000, -0.08879589532294571153 ) ) ;
#605=CARTESIAN_POINT ( 'NONE',  ( 67.29303306501925874, -175.3837268820161057, 47.13604789772129777 ) ) ;
#606=ORIENTED_EDGE ( 'NONE', *, *, #1748, .F. ) ;
#608=VECTOR ( 'NONE', #44679, 1000.000000000000114 ) ;
#609=EDGE_LOOP ( 'NONE', ( #43892, #41673, #35161, #47597 ) ) ;
#611=ADVANCED_FACE ( 'NONE', ( #22233 ), #22758, .F. ) ;
#613=ADVANCED_FACE ( 'NONE', ( #30368 ), #18310, .T. ) ;
#614=CARTESIAN_POINT ( 'NONE',  ( -102.0975050429523776, -183.6283474603465606, -111.8087531435654682 ) ) ;
#615=LINE ( 'NONE', #29498, #4504 ) ;
#616=DIRECTION ( 'NONE',  ( -0.7948544414133523750, 0.000000000000000000, -0.6068001458185945385 ) ) ;
#621=CARTESIAN_POINT ( 'NONE',  ( -47.55243714407701816, -189.7472609257535510, -0.3758275821142288420 ) ) ;
#622=DIRECTION ( 'NONE',  ( 0.000000000000000000, 0.000000000000000000, -1.000000000000000000 ) ) ;
#624=ORIENTED_EDGE ( 'NONE', *, *, #8566, .T. ) ;
#627=DIRECTION ( 'NONE',  ( 0.000000000000000000, -1.000000000000000000, -0.000000000000000000 ) ) ;
#628=AXIS2_PLACEMENT_3D ( 'NONE', #14923, #21763, #1775 ) ;
#633=EDGE_CURVE ( 'NONE', #35850, #14215, #51404, .T. ) ;
#635=EDGE_CURVE ( 'NONE', #30065, #6051, #38528, .T. ) ;
#637=ORIENTED_EDGE ( 'NONE', *, *, #43796, .F. ) ;
#638=CARTESIAN_POINT ( 'NONE',  ( -23.01747912075234836, -193.5000000000000000, -122.3793467049370634 ) ) ;
#641=EDGE_CURVE ( 'NONE', #20455, #18266, #17916, .T. ) ;
#642=FACE_OUTER_BOUND ( 'NONE', #50489, .T. ) ;
#644=EDGE_CURVE ( 'NONE', #25704, #37475, #2776, .T. ) ;
#645=DIRECTION ( 'NONE',  ( -0.8757349421956412971, 0.000000000000000000, 0.4827922027307366970 ) ) ;
#646=DIRECTION ( 'NONE',  ( 1.000000000000000000, -0.000000000000000000, 6.978251959525016136E-17 ) ) ;
#649=EDGE_CURVE ( 'NONE', #21906, #4350, #15399, .T. ) ;
#650=VERTEX_POINT ( 'NONE', #26700 ) ;
#651=CARTESIAN_POINT ( 'NONE',  ( -81.70897914701308196, -183.6283474603465606, -120.5021863277716534 ) ) ;
#652=ORIENTED_EDGE ( 'NONE', *, *, #33377, .T. ) ;
#653=VERTEX_POINT ( 'NONE', #42734 ) ;
#654=CIRCLE ( 'NONE', #29192, 125.0000000000000000 ) ;
#655=VECTOR ( 'NONE', #37602, 1000.000000000000114 ) ;
#656=CARTESIAN_POINT ( 'NONE',  ( -92.43312097795266880, -175.3837268820161057, -115.9484881370935483 ) ) ;
#657=DIRECTION ( 'NONE',  ( 0.000000000000000000, -1.000000000000000000, 0.000000000000000000 ) ) ;
#659=ORIENTED_EDGE ( 'NONE', *, *, #1459, .T. ) ;
#661=EDGE_CURVE ( 'NONE', #39966, #40406, #17095, .T. ) ;
#664=VERTEX_POINT ( 'NONE', #28494 ) ;
#665=CARTESIAN_POINT ( 'NONE',  ( 9.518239912201957864, -213.5000000000000000, 110.7307791902283043 ) ) ;
#666=ORIENTED_EDGE ( 'NONE', *, *, #48169, .F. ) ;
#668=CARTESIAN_POINT ( 'NONE',  ( -48.71401279728984690, -175.3837268820161057, 0.9720229140804159673 ) ) ;
#669=CARTESIAN_POINT ( 'NONE',  ( -9.671950287350391307, -177.1207230881787780, -118.8234112238815641 ) ) ;
#671=ORIENTED_EDGE ( 'NONE', *, *, #14170, .F. ) ;
#672=VERTEX_POINT ( 'NONE', #23531 ) ;
#675=CARTESIAN_POINT ( 'NONE',  ( 70.68712318874649725, -193.5000000000000000, -37.74128873232327663 ) ) ;
#676=CARTESIAN_POINT ( 'NONE',  ( -59.28786813212837359, -177.1207230881787780, 124.5318076226587323 ) ) ;
#677=DIRECTION ( 'NONE',  ( 0.000000000000000000, 0.000000000000000000, -1.000000000000000000 ) ) ;
#679=DIRECTION ( 'NONE',  ( 0.000000000000000000, -0.000000000000000000, -1.000000000000000000 ) ) ;
#682=ADVANCED_FACE ( 'NONE', ( #43509 ), #31674, .F. ) ;
#684=CARTESIAN_POINT ( 'NONE',  ( 2.266533711611407043, -189.7472609257535510, 113.1409892739925453 ) ) ;
#685=ORIENTED_EDGE ( 'NONE', *, *, #39363, .T. ) ;
#686=PLANE ( 'NONE',  #7824 ) ;
#688=ORIENTED_EDGE ( 'NONE', *, *, #14374, .T. ) ;
#691=CIRCLE ( 'NONE', #15817, 125.0000000000000000 ) ;
#694=CARTESIAN_POINT ( 'NONE',  ( -162.3451783319732442, -193.5000000000000000, 51.57055649762783389 ) ) ;
#697=FACE_OUTER_BOUND ( 'NONE', #41985, .T. ) ;
#698=ORIENTED_EDGE ( 'NONE', *, *, #20067, .T. ) ;
#702=ADVANCED_FACE ( 'NONE', ( #27983 ), #12209, .T. ) ;
#703=CARTESIAN_POINT ( 'NONE',  ( 75.02564229359539638, -175.3837268820161057, -19.27620354518634826 ) ) ;
#705=LINE ( 'NONE', #17971, #36499 ) ;
#707=FACE_OUTER_BOUND ( 'NONE', #11234, .T. ) ;
#708=DIRECTION ( 'NONE',  ( 0.6965510290629982615, 0.000000000000000000, -0.7175072570443298270 ) ) ;
#709=ORIENTED_EDGE ( 'NONE', *, *, #13446, .T. ) ;
#710=LINE ( 'NONE', #28803, #21329 ) ;
#712=ADVANCED_FACE ( 'NONE', ( #16169 ), #36129, .F. ) ;
#713=VECTOR ( 'NONE', #18142, 1000.000000000000000 ) ;
#714=LINE ( 'NONE', #49585, #32837 ) ;
#715=FACE_BOUND ( 'NONE', #39731, .T. ) ;
#716=VERTEX_POINT ( 'NONE', #8281 ) ;
#717=FACE_OUTER_BOUND ( 'NONE', #32723, .T. ) ;
#718=ORIENTED_EDGE ( 'NONE', *, *, #2218, .F. ) ;
#723=CARTESIAN_POINT ( 'NONE',  ( -106.2948367055610106, -189.7472609257535510, -110.8257356506552185 ) ) ;
#726=FACE_BOUND ( 'NONE', #3636, .T. ) ;
#728=VERTEX_POINT ( 'NONE', #39544 ) ;
#729=VECTOR ( 'NONE', #13592, 1000.000000000000114 ) ;
#731=EDGE_LOOP ( 'NONE', ( #11953, #13338, #18048, #14655 ) ) ;
#732=ORIENTED_EDGE ( 'NONE', *, *, #40407, .F. ) ;
#733=CARTESIAN_POINT ( 'NONE',  ( -49.45768324380835423, -183.6283474603465606, 0.2059786187410958813 ) ) ;
#735=CARTESIAN_POINT ( 'NONE',  ( -127.4665351220365892, -177.1207230881787780, -96.88131563365291754 ) ) ;
#736=ORIENTED_EDGE ( 'NONE', *, *, #2249, .F. ) ;
#741=VECTOR ( 'NONE', #42768, 1000.000000000000000 ) ;
#742=DIRECTION ( 'NONE',  ( 0.000000000000000000, -1.000000000000000000, 0.000000000000000000 ) ) ;
#743=LINE ( 'NONE', #44889, #7201 ) ;
#744=ORIENTED_EDGE ( 'NONE', *, *, #18260, .T. ) ;
#747=EDGE_LOOP ( 'NONE', ( #32037, #24725, #215, #545 ) ) ;
#749=PLANE ( 'NONE',  #44990 ) ;
#751=DIRECTION ( 'NONE',  ( -0.000000000000000000, -1.000000000000000000, 0.000000000000000000 ) ) ;
#752=ORIENTED_EDGE ( 'NONE', *, *, #16107, .F. ) ;
#754=LINE ( 'NONE', #16800, #2405 ) ;
#757=DIRECTION ( 'NONE',  ( -0.000000000000000000, 1.000000000000000000, -0.000000000000000000 ) ) ;
#758=ORIENTED_EDGE ( 'NONE', *, *, #47440, .F. ) ;
#760=CARTESIAN_POINT ( 'NONE',  ( -37.78865854180985195, -183.6283474603465606, -123.5388265266451242 ) ) ;
#762=VECTOR ( 'NONE', #33094, 1000.000000000000000 ) ;
#763=ADVANCED_FACE ( 'NONE', ( #11698 ), #48503, .F. ) ;
#765=CARTESIAN_POINT ( 'NONE',  ( 22.03849146056077757, -175.3837268820161057, 103.2098131075567267 ) ) ;
#767=AXIS2_PLACEMENT_3D ( 'NONE', #28514, #22135, #9088 ) ;
#768=CARTESIAN_POINT ( 'NONE',  ( -160.4991136281923332, -193.5000000000000000, 53.17445600718630061 ) ) ;
#770=CARTESIAN_POINT ( 'NONE',  ( -48.47912675150885065, -189.7472609257535510, 6.938893903907228378E-15 ) ) ;
#773=DIRECTION ( 'NONE',  ( 0.000000000000000000, -1.000000000000000000, 0.000000000000000000 ) ) ;
#774=EDGE_LOOP ( 'NONE', ( #44968, #19861, #24735, #2334 ) ) ;
#775=VERTEX_POINT ( 'NONE', #27723 ) ;
#776=DIRECTION ( 'NONE',  ( 0.000000000000000000, -0.000000000000000000, -1.000000000000000000 ) ) ;
#777=DIRECTION ( 'NONE',  ( 0.000000000000000000, 0.000000000000000000, -1.000000000000000000 ) ) ;
#779=VERTEX_POINT ( 'NONE', #32188 ) ;
#780=ORIENTED_EDGE ( 'NONE', *, *, #5158, .F. ) ;
#781=ORIENTED_EDGE ( 'NONE', *, *, #37550, .T. ) ;
#782=VECTOR ( 'NONE', #29574, 1000.000000000000000 ) ;
#783=DIRECTION ( 'NONE',  ( 0.000000000000000000, 0.000000000000000000, -1.000000000000000000 ) ) ;
#784=DIRECTION ( 'NONE',  ( 0.9720229140804089729, 0.000000000000000000, 0.2348860457809911206 ) ) ;
#787=VERTEX_POINT ( 'NONE', #11430 ) ;
#790=CARTESIAN_POINT ( 'NONE',  ( 23.33927677392130917, -183.6283474603465606, -102.3089288139528747 ) ) ;
#791=ORIENTED_EDGE ( 'NONE', *, *, #493, .T. ) ;
#792=CARTESIAN_POINT ( 'NONE',  ( -164.3791542526839180, -175.3837268820161057, 46.82076062204521349 ) ) ;
#794=VERTEX_POINT ( 'NONE', #32452 ) ;
#797=DIRECTION ( 'NONE',  ( -0.7765238627180393038, 0.000000000000000000, -0.6300878435817147682 ) ) ;
#799=EDGE_CURVE ( 'NONE', #11174, #43506, #40316, .T. ) ;
#800=EDGE_CURVE ( 'NONE', #35554, #10123, #31928, .T. ) ;
#801=LINE ( 'NONE', #5808, #45204 ) ;
#806=ORIENTED_EDGE ( 'NONE', *, *, #37358, .F. ) ;
#807=EDGE_CURVE ( 'NONE', #6494, #17445, #2198, .T. ) ;
#808=DIRECTION ( 'NONE',  ( -0.9027978299657416494, 0.000000000000000000, -0.4300652022765245608 ) ) ;
#810=LINE ( 'NONE', #33403, #44881 ) ;
#811=CARTESIAN_POINT ( 'NONE',  ( -124.9871112439422092, -175.3837268820161057, -98.85104101073275729 ) ) ;
#813=CARTESIAN_POINT ( 'NONE',  ( -140.5285791076019279, -189.7472609257535510, -83.08371579725672973 ) ) ;
#817=VECTOR ( 'NONE', #4352, 999.9999999999998863 ) ;
#823=DIRECTION ( 'NONE',  ( 0.05924062789371441901, 0.000000000000000000, -0.9982437317643214625 ) ) ;
#829=ORIENTED_EDGE ( 'NONE', *, *, #34198, .F. ) ;
#832=CARTESIAN_POINT ( 'NONE',  ( -171.7300019102062549, -193.5000000000000000, -20.83798868929510562 ) ) ;
#833=DIRECTION ( 'NONE',  ( 0.1768902751225666370, 0.000000000000000000, 0.9842305779475979399 ) ) ;
#834=DIRECTION ( 'NONE',  ( 0.000000000000000000, 0.000000000000000000, 1.000000000000000000 ) ) ;
#836=CARTESIAN_POINT ( 'NONE',  ( 63.10841233855954613, -193.5000000000000000, -54.07611884703302962 ) ) ;
#838=DIRECTION ( 'NONE',  ( -0.000000000000000000, 1.000000000000000000, -0.000000000000000000 ) ) ;
#839=DIRECTION ( 'NONE',  ( 0.000000000000000000, 1.000000000000000000, -0.000000000000000000 ) ) ;
#840=VERTEX_POINT ( 'NONE', #40068 ) ;
#842=EDGE_CURVE ( 'NONE', #32383, #1430, #31407, .T. ) ;
#845=CIRCLE ( 'NONE', #30231, 124.9999999999999858 ) ;
#846=AXIS2_PLACEMENT_3D ( 'NONE', #1945, #25341, #16944 ) ;
#849=ORIENTED_EDGE ( 'NONE', *, *, #7386, .T. ) ;
#850=ORIENTED_EDGE ( 'NONE', *, *, #23322, .T. ) ;
#851=DIRECTION ( 'NONE',  ( 0.000000000000000000, -1.000000000000000000, 0.000000000000000000 ) ) ;
#853=LINE ( 'NONE', #25048, #29478 ) ;
#854=CARTESIAN_POINT ( 'NONE',  ( -47.47956591500005885, -193.5000000000000000, -0.02963332782254939762 ) ) ;
#856=ORIENTED_EDGE ( 'NONE', *, *, #47489, .T. ) ;
#858=CARTESIAN_POINT ( 'NONE',  ( -5.113431607746556473, -193.5000000000000000, 117.2365833888819537 ) ) ;
#859=FACE_OUTER_BOUND ( 'NONE', #28097, .T. ) ;
#860=ORIENTED_EDGE ( 'NONE', *, *, #5508, .F. ) ;
#861=EDGE_CURVE ( 'NONE', #38326, #8427, #29287, .T. ) ;
#864=ORIENTED_EDGE ( 'NONE', *, *, #28901, .F. ) ;
#866=EDGE_CURVE ( 'NONE', #47840, #37031, #15636, .T. ) ;
#867=EDGE_LOOP ( 'NONE', ( #46785, #23788, #50525, #40212 ) ) ;
#869=LINE ( 'NONE', #16911, #34690 ) ;
#870=CARTESIAN_POINT ( 'NONE',  ( -153.7332855749581881, -193.5000000000000000, 67.42819922234390617 ) ) ;
#871=ORIENTED_EDGE ( 'NONE', *, *, #43423, .T. ) ;
#874=DIRECTION ( 'NONE',  ( -0.5586467658036415873, 0.000000000000000000, -0.8294056854502090959 ) ) ;
#875=VERTEX_POINT ( 'NONE', #37695 ) ;
#876=CARTESIAN_POINT ( 'NONE',  ( -37.08895481556041318, -183.6283474603465606, 124.4799742258550452 ) ) ;
#877=CARTESIAN_POINT ( 'NONE',  ( 75.43907105790114542, -193.5000000000000000, -4.503971736580765217 ) ) ;
#882=VECTOR ( 'NONE', #10796, 1000.000000000000000 ) ;
#883=ORIENTED_EDGE ( 'NONE', *, *, #5967, .F. ) ;
#885=VERTEX_POINT ( 'NONE', #20900 ) ;
#886=FACE_BOUND ( 'NONE', #8884, .T. ) ;
#887=PLANE ( 'NONE',  #37947 ) ;
#890=DIRECTION ( 'NONE',  ( 0.000000000000000000, 0.000000000000000000, -1.000000000000000000 ) ) ;
#894=CARTESIAN_POINT ( 'NONE',  ( 39.18328161278952138, -189.7472609257535510, 89.10837311819237527 ) ) ;
#895=VERTEX_POINT ( 'NONE', #24825 ) ;
#896=EDGE_CURVE ( 'NONE', #15597, #13271, #36917, .T. ) ;
#897=ORIENTED_EDGE ( 'NONE', *, *, #18009, .T. ) ;
#904=EDGE_CURVE ( 'NONE', #21757, #43156, #32958, .T. ) ;
#906=EDGE_CURVE ( 'NONE', #39920, #28294, #29044, .T. ) ;
#909=ORIENTED_EDGE ( 'NONE', *, *, #36556, .F. ) ;
#910=CARTESIAN_POINT ( 'NONE',  ( -48.47912675150885065, -177.1207230881787780, 6.938893903907228378E-15 ) ) ;
#911=EDGE_CURVE ( 'NONE', #19332, #33563, #21674, .T. ) ;
#912=ORIENTED_EDGE ( 'NONE', *, *, #15930, .T. ) ;
#913=DIRECTION ( 'NONE',  ( 0.8610436117673514467, 0.000000000000000000, 0.5085311186492273983 ) ) ;
#914=DIRECTION ( 'NONE',  ( 0.000000000000000000, 0.000000000000000000, -1.000000000000000000 ) ) ;
#923=EDGE_LOOP ( 'NONE', ( #21309, #38408, #51549, #25066 ) ) ;
#925=PLANE ( 'NONE',  #21797 ) ;
#926=EDGE_CURVE ( 'NONE', #40282, #34006, #49542, .T. ) ;
#929=DIRECTION ( 'NONE',  ( 0.2348860457809775482, 0.000000000000000000, 0.9720229140804121926 ) ) ;
#932=ADVANCED_FACE ( 'NONE', ( #28749 ), #41114, .T. ) ;
#933=EDGE_CURVE ( 'NONE', #20143, #3616, #35758, .T. ) ;
#934=ORIENTED_EDGE ( 'NONE', *, *, #18476, .T. ) ;
#935=DIRECTION ( 'NONE',  ( 0.000000000000000000, 0.000000000000000000, 1.000000000000000000 ) ) ;
#936=ORIENTED_EDGE ( 'NONE', *, *, #35799, .T. ) ;
#937=ORIENTED_EDGE ( 'NONE', *, *, #49984, .T. ) ;
#938=AXIS2_PLACEMENT_3D ( 'NONE', #18449, #43124, #7129 ) ;
#939=PLANE ( 'NONE',  #35045 ) ;
#940=PLANE ( 'NONE',  #18272 ) ;
#943=ORIENTED_EDGE ( 'NONE', *, *, #8920, .F. ) ;
#944=DIRECTION ( 'NONE',  ( 0.000000000000000000, -1.000000000000000000, 0.000000000000000000 ) ) ;
#946=EDGE_CURVE ( 'NONE', #41454, #49394, #18152, .T. ) ;
#947=ORIENTED_EDGE ( 'NONE', *, *, #41395, .F. ) ;
#948=CARTESIAN_POINT ( 'NONE',  ( -1.771278280434274155, -177.1207230881787780, -115.9455772817710084 ) ) ;
#949=DIRECTION ( 'NONE',  ( 0.000000000000000000, 0.000000000000000000, 1.000000000000000000 ) ) ;
#950=VECTOR ( 'NONE', #32180, 1000.000000000000000 ) ;
#951=DIRECTION ( 'NONE',  ( -0.8610436117673548884, 0.000000000000000000, -0.5085311186492216251 ) ) ;
#952=DIRECTION ( 'NONE',  ( -0.000000000000000000, 1.000000000000000000, -0.000000000000000000 ) ) ;
#953=DIRECTION ( 'NONE',  ( 0.000000000000000000, -0.000000000000000000, 1.000000000000000000 ) ) ;
#954=EDGE_LOOP ( 'NONE', ( #27376, #42178, #35892, #9109 ) ) ;
#955=FACE_OUTER_BOUND ( 'NONE', #46614, .T. ) ;
#958=DIRECTION ( 'NONE',  ( -0.000000000000000000, 1.000000000000000000, 0.000000000000000000 ) ) ;
#959=FACE_BOUND ( 'NONE', #7939, .T. ) ;
#961=CARTESIAN_POINT ( 'NONE',  ( 20.10322172534453244, -175.3837268820161057, -103.3076327631962954 ) ) ;
#962=EDGE_LOOP ( 'NONE', ( #46378, #36787, #38995, #31564 ) ) ;
#963=CARTESIAN_POINT ( 'NONE',  ( -48.47912675150885065, -177.1207230881787780, 6.938893903907228378E-15 ) ) ;
#964=EDGE_CURVE ( 'NONE', #13900, #12470, #48136, .T. ) ;
#967=CARTESIAN_POINT ( 'NONE',  ( 36.84288420123323249, -193.5000000000000000, 91.35181687837503262 ) ) ;
#968=ORIENTED_EDGE ( 'NONE', *, *, #13302, .F. ) ;
#970=EDGE_CURVE ( 'NONE', #42763, #14296, #20524, .T. ) ;
#971=EDGE_CURVE ( 'NONE', #12481, #41605, #26539, .T. ) ;
#973=AXIS2_PLACEMENT_3D ( 'NONE', #43646, #11589, #36993 ) ;
#974=CARTESIAN_POINT ( 'NONE',  ( -106.4764934152196645, -193.5000000000000000, -110.7307791902283043 ) ) ;
#975=VERTEX_POINT ( 'NONE', #15835 ) ;
#976=LINE ( 'NONE', #17029, #29407 ) ;
#979=ORIENTED_EDGE ( 'NONE', *, *, #41691, .T. ) ;
#980=DIRECTION ( 'NONE',  ( -0.000000000000000000, -1.000000000000000000, 0.000000000000000000 ) ) ;
#983=ORIENTED_EDGE ( 'NONE', *, *, #25650, .T. ) ;
#985=CARTESIAN_POINT ( 'NONE',  ( -49.47517659412406488, -175.3837268820161057, -0.08879589532293878651 ) ) ;
#986=CYLINDRICAL_SURFACE ( 'NONE', #16278, 125.0000000000000000 ) ;
#987=VECTOR ( 'NONE', #1151, 1000.000000000000000 ) ;
#989=EDGE_CURVE ( 'NONE', #1891, #26506, #4719, .T. ) ;
#990=VECTOR ( 'NONE', #16883, 1000.000000000000000 ) ;
#991=CARTESIAN_POINT ( 'NONE',  ( -48.24424070572786860, -193.5000000000000000, -0.9720229140804037549 ) ) ;
#992=CARTESIAN_POINT ( 'NONE',  ( -70.24606818074174441, -175.3837268820161057, -122.0745693923548885 ) ) ;
#993=VERTEX_POINT ( 'NONE', #554 ) ;
#994=CARTESIAN_POINT ( 'NONE',  ( -46.06708674231131084, -177.1207230881787780, -124.9767260852756863 ) ) ;
#996=ORIENTED_EDGE ( 'NONE', *, *, #9660, .T. ) ;
#997=EDGE_LOOP ( 'NONE', ( #1624, #5799, #27642, #44383 ) ) ;
#998=CARTESIAN_POINT ( 'NONE',  ( -48.47912675150885065, -175.3837268820161057, 6.938893903907228378E-15 ) ) ;
#999=EDGE_LOOP ( 'NONE', ( #14345, #29915, #10914, #12170 ) ) ;
#1002=CARTESIAN_POINT ( 'NONE',  ( -72.96029774493611342, -193.5000000000000000, 122.5792489240759409 ) ) ;
#1004=ORIENTED_EDGE ( 'NONE', *, *, #33599, .F. ) ;
#1005=CARTESIAN_POINT ( 'NONE',  ( -172.7479958471413966, -177.1207230881787780, -13.49993235881363418 ) ) ;
#1006=ORIENTED_EDGE ( 'NONE', *, *, #3159, .T. ) ;
#1007=AXIS2_PLACEMENT_3D ( 'NONE', #42136, #33499, #37944 ) ;
#1011=CARTESIAN_POINT ( 'NONE',  ( -1.578537454945990293, -183.6283474603465606, 114.7887733785766926 ) ) ;
#1012=AXIS2_PLACEMENT_3D ( 'NONE', #3323, #35369, #51682 ) ;
#1013=LINE ( 'NONE', #49120, #20489 ) ;
#1014=CARTESIAN_POINT ( 'NONE',  ( -154.2693405752510500, -189.7472609257535510, 66.58401203837827609 ) ) ;
#1015=ORIENTED_EDGE ( 'NONE', *, *, #49773, .T. ) ;
#1017=DIRECTION ( 'NONE',  ( 0.000000000000000000, 0.000000000000000000, -1.000000000000000000 ) ) ;
#1018=CARTESIAN_POINT ( 'NONE',  ( 21.49274850782854074, -193.5000000000000000, -103.5805805771126700 ) ) ;
#1019=DIRECTION ( 'NONE',  ( 0.000000000000000000, -1.000000000000000000, 0.000000000000000000 ) ) ;
#1020=DIRECTION ( 'NONE',  ( 0.000000000000000000, 0.000000000000000000, 1.000000000000000000 ) ) ;
#1024=DIRECTION ( 'NONE',  ( 0.000000000000000000, -1.000000000000000000, 0.000000000000000000 ) ) ;
#1028=ORIENTED_EDGE ( 'NONE', *, *, #30753, .T. ) ;
#1029=ORIENTED_EDGE ( 'NONE', *, *, #9171, .T. ) ;
#1031=PLANE ( 'NONE',  #16725 ) ;
#1032=LINE ( 'NONE', #44675, #32050 ) ;
#1034=DIRECTION ( 'NONE',  ( -0.000000000000000000, 1.000000000000000000, 0.000000000000000000 ) ) ;
#1035=VERTEX_POINT ( 'NONE', #35777 ) ;
#1038=VECTOR ( 'NONE', #4734, 1000.000000000000227 ) ;
#1040=AXIS2_PLACEMENT_3D ( 'NONE', #5163, #8318, #16466 ) ;
#1041=DIRECTION ( 'NONE',  ( 0.000000000000000000, 0.000000000000000000, 1.000000000000000000 ) ) ;
#1042=ORIENTED_EDGE ( 'NONE', *, *, #34030, .T. ) ;
#1044=DIRECTION ( 'NONE',  ( -0.9960498426152177842, 0.000000000000000000, 0.08879589532292482545 ) ) ;
#1045=VECTOR ( 'NONE', #12771, 1000.000000000000227 ) ;
#1047=ORIENTED_EDGE ( 'NONE', *, *, #10383, .F. ) ;
#1048=EDGE_CURVE ( 'NONE', #47759, #11883, #36044, .T. ) ;
#1052=CARTESIAN_POINT ( 'NONE',  ( 60.90550954139437323, -175.3837268820161057, 60.49794494914087295 ) ) ;
#1057=CARTESIAN_POINT ( 'NONE',  ( -155.9608607592037401, -183.6283474603465606, 63.81752780153057358 ) ) ;
#1059=DIRECTION ( 'NONE',  ( -0.000000000000000000, 1.000000000000000000, 0.000000000000000000 ) ) ;
#1060=ORIENTED_EDGE ( 'NONE', *, *, #36657, .T. ) ;
#1062=DIRECTION ( 'NONE',  ( 0.000000000000000000, -1.000000000000000000, 0.000000000000000000 ) ) ;
#1063=DIRECTION ( 'NONE',  ( 0.000000000000000000, 0.000000000000000000, 1.000000000000000000 ) ) ;
#1065=EDGE_LOOP ( 'NONE', ( #26857, #9484, #32742, #48666 ) ) ;
#1067=CARTESIAN_POINT ( 'NONE',  ( -168.9345475356665247, -193.5000000000000000, 29.43839964798726427 ) ) ;
#1069=DIRECTION ( 'NONE',  ( -0.000000000000000000, -1.000000000000000000, 0.000000000000000000 ) ) ;
#1070=ADVANCED_FACE ( 'NONE', ( #24224 ), #43672, .T. ) ;
#1072=LINE ( 'NONE', #4247, #48477 ) ;
#1074=CARTESIAN_POINT ( 'NONE',  ( -171.2399149993172500, -189.7472609257535510, -17.48697739784461547 ) ) ;
#1077=VECTOR ( 'NONE', #10028, 1000.000000000000114 ) ;
#1078=LINE ( 'NONE', #17655, #267 ) ;
#1082=FACE_OUTER_BOUND ( 'NONE', #774, .T. ) ;
#1083=EDGE_LOOP ( 'NONE', ( #33373, #19923, #40663, #49967 ) ) ;
#1084=AXIS2_PLACEMENT_3D ( 'NONE', #4869, #16702, #32704 ) ;
#1086=DIRECTION ( 'NONE',  ( -0.000000000000000000, 1.000000000000000000, -0.000000000000000000 ) ) ;
#1087=CARTESIAN_POINT ( 'NONE',  ( -172.6359455740846442, -177.1207230881787780, -14.49428645563791562 ) ) ;
#1088=CARTESIAN_POINT ( 'NONE',  ( -47.64924157374594671, -193.5000000000000000, 124.9972451320097377 ) ) ;
#1092=DIRECTION ( 'NONE',  ( -0.9929810960135169173, 0.000000000000000000, -0.1182731709213660498 ) ) ;
#1093=CARTESIAN_POINT ( 'NONE',  ( 36.10886851198522152, -177.1207230881787780, 92.03190238880812046 ) ) ;
#1095=VERTEX_POINT ( 'NONE', #48668 ) ;
#1098=DIRECTION ( 'NONE',  ( -0.1476465640024779702, 0.000000000000000000, -0.9890401873221644768 ) ) ;
#1099=CIRCLE ( 'NONE', #43897, 125.0000000000000000 ) ;
#1101=DIRECTION ( 'NONE',  ( 0.000000000000000000, -1.000000000000000000, 0.000000000000000000 ) ) ;
#1104=EDGE_LOOP ( 'NONE', ( #39856, #48441, #16840, #32095 ) ) ;
#1106=PLANE ( 'NONE',  #22538 ) ;
#1108=CARTESIAN_POINT ( 'NONE',  ( -48.47912675150885065, -183.6283474603465606, 1.000000000000006883 ) ) ;
#1109=ORIENTED_EDGE ( 'NONE', *, *, #6562, .F. ) ;
#1111=DIRECTION ( 'NONE',  ( -0.000000000000000000, 1.000000000000000000, 0.000000000000000000 ) ) ;
#1112=ORIENTED_EDGE ( 'NONE', *, *, #36486, .T. ) ;
#1115=EDGE_LOOP ( 'NONE', ( #13335, #18984, #15871, #12888 ) ) ;
#1116=DIRECTION ( 'NONE',  ( -0.000000000000000000, 1.000000000000000000, 0.000000000000000000 ) ) ;
#1117=ORIENTED_EDGE ( 'NONE', *, *, #17462, .T. ) ;
#1118=AXIS2_PLACEMENT_3D ( 'NONE', #44291, #51657, #20104 ) ;
#1119=DIRECTION ( 'NONE',  ( -0.5338233779647887367, 0.000000000000000000, -0.8455960035018273979 ) ) ;
#1121=DIRECTION ( 'NONE',  ( 0.6068001458185890984, 0.000000000000000000, 0.7948544414133565938 ) ) ;
#1122=EDGE_LOOP ( 'NONE', ( #3944, #25050, #48076, #48134 ) ) ;
#1123=ORIENTED_EDGE ( 'NONE', *, *, #4358, .F. ) ;
#1124=DIRECTION ( 'NONE',  ( -0.2920567706369628924, 0.000000000000000000, -0.9564009842765264224 ) ) ;
#1125=LINE ( 'NONE', #21898, #22530 ) ;
#1127=DIRECTION ( 'NONE',  ( 0.000000000000000000, 1.000000000000000000, 0.000000000000000000 ) ) ;
#1129=DIRECTION ( 'NONE',  ( 0.000000000000000000, 0.000000000000000000, 1.000000000000000000 ) ) ;
#1130=EDGE_CURVE ( 'NONE', #12681, #24651, #10601, .T. ) ;
#1131=ADVANCED_FACE ( 'NONE', ( #17398 ), #13432, .T. ) ;
#1132=ORIENTED_EDGE ( 'NONE', *, *, #23366, .T. ) ;
#1135=AXIS2_PLACEMENT_3D ( 'NONE', #38655, #26314, #14244 ) ;
#1136=ORIENTED_EDGE ( 'NONE', *, *, #6330, .F. ) ;
#1137=PLANE ( 'NONE',  #20696 ) ;
#1138=ORIENTED_EDGE ( 'NONE', *, *, #36258, .F. ) ;
#1139=CARTESIAN_POINT ( 'NONE',  ( -84.82349129030166068, -193.5000000000000000, -119.5996955107802222 ) ) ;
#1142=ORIENTED_EDGE ( 'NONE', *, *, #1857, .F. ) ;
#1144=DIRECTION ( 'NONE',  ( 0.000000000000000000, 0.000000000000000000, -1.000000000000000000 ) ) ;
#1146=ADVANCED_FACE ( 'NONE', ( #41812 ), #1852, .T. ) ;
#1147=AXIS2_PLACEMENT_3D ( 'NONE', #10818, #4415, #40654 ) ;
#1150=ORIENTED_EDGE ( 'NONE', *, *, #42462, .T. ) ;
#1151=DIRECTION ( 'NONE',  ( 0.4031234292879730674, 0.000000000000000000, -0.9151456172430181280 ) ) ;
#1156=DIRECTION ( 'NONE',  ( -0.000000000000000000, 1.000000000000000000, -0.000000000000000000 ) ) ;
#1159=VERTEX_POINT ( 'NONE', #10021 ) ;
#1160=DIRECTION ( 'NONE',  ( 0.000000000000000000, 0.000000000000000000, -1.000000000000000000 ) ) ;
#1162=LINE ( 'NONE', #12987, #20148 ) ;
#1164=DIRECTION ( 'NONE',  ( 0.000000000000000000, 0.000000000000000000, -1.000000000000000000 ) ) ;
#1166=CARTESIAN_POINT ( 'NONE',  ( -48.98765787015808115, -175.3837268820161057, 0.8610436117673582190 ) ) ;
#1169=CIRCLE ( 'NONE', #45683, 125.0000000000000000 ) ;
#1171=DIRECTION ( 'NONE',  ( 0.000000000000000000, -1.000000000000000000, 0.000000000000000000 ) ) ;
#1174=CIRCLE ( 'NONE', #7886, 125.0000000000000000 ) ;
#1175=ORIENTED_EDGE ( 'NONE', *, *, #16877, .T. ) ;
#1176=CARTESIAN_POINT ( 'NONE',  ( -15.81236726369127155, -183.6283474603465606, -120.6560517527615559 ) ) ;
#1177=DIRECTION ( 'NONE',  ( -0.8124868780056863082, 0.000000000000000000, 0.5829794791144649047 ) ) ;
#1178=CARTESIAN_POINT ( 'NONE',  ( -151.9915035862630646, -183.6283474603465606, 70.07273251429430161 ) ) ;
#1179=DIRECTION ( 'NONE',  ( 0.000000000000000000, 1.000000000000000000, 0.000000000000000000 ) ) ;
#1180=ORIENTED_EDGE ( 'NONE', *, *, #48158, .T. ) ;
#1181=AXIS2_PLACEMENT_3D ( 'NONE', #46702, #38019, #2299 ) ;
#1182=ORIENTED_EDGE ( 'NONE', *, *, #51706, .F. ) ;
#1186=CARTESIAN_POINT ( 'NONE',  ( 28.02885774092381865, -193.5000000000000000, 98.85104101073331151 ) ) ;
#1187=LINE ( 'NONE', #5418, #4841 ) ;
#1189=CARTESIAN_POINT ( 'NONE',  ( 18.00181100848372751, -183.6283474603465606, -105.8550183720733742 ) ) ;
#1190=EDGE_CURVE ( 'NONE', #42645, #40857, #17379, .T. ) ;
#1191=EDGE_CURVE ( 'NONE', #36985, #10779, #37494, .T. ) ;
#1192=DIRECTION ( 'NONE',  ( 0.7378332790417285736, 0.000000000000000000, -0.6749830015182091136 ) ) ;
#1194=DIRECTION ( 'NONE',  ( -0.000000000000000000, 1.000000000000000000, -0.000000000000000000 ) ) ;
#1195=EDGE_LOOP ( 'NONE', ( #16137, #29792, #13880, #18999 ) ) ;
#1196=ADVANCED_FACE ( 'NONE', ( #1614 ), #13179, .T. ) ;
#1198=PLANE ( 'NONE',  #3612 ) ;
#1200=FACE_OUTER_BOUND ( 'NONE', #51358, .T. ) ;
#1212=ADVANCED_FACE ( 'NONE', ( #27051 ), #30739, .T. ) ;
#1213=DIRECTION ( 'NONE',  ( -0.000000000000000000, 1.000000000000000000, -0.000000000000000000 ) ) ;
#1214=DIRECTION ( 'NONE',  ( 0.000000000000000000, 0.000000000000000000, 1.000000000000000000 ) ) ;
#1215=ORIENTED_EDGE ( 'NONE', *, *, #12852, .F. ) ;
#1216=EDGE_CURVE ( 'NONE', #37425, #42355, #6840, .T. ) ;
#1217=CARTESIAN_POINT ( 'NONE',  ( -106.2948367055610106, -193.5000000000000000, -110.8257356506552185 ) ) ;
#1218=ORIENTED_EDGE ( 'NONE', *, *, #43325, .F. ) ;
#1219=DIRECTION ( 'NONE',  ( 0.8610436117673585521, 0.000000000000000000, -0.5085311186492154079 ) ) ;
#1220=ADVANCED_FACE ( 'NONE', ( #2388 ), #51001, .T. ) ;
#1221=ORIENTED_EDGE ( 'NONE', *, *, #11832, .F. ) ;
#1223=VECTOR ( 'NONE', #24581, 1000.000000000000000 ) ;
#1225=DIRECTION ( 'NONE',  ( 0.000000000000000000, -0.000000000000000000, -1.000000000000000000 ) ) ;
#1228=VERTEX_POINT ( 'NONE', #26542 ) ;
#1230=EDGE_CURVE ( 'NONE', #41535, #24657, #42580, .T. ) ;
#1232=ORIENTED_EDGE ( 'NONE', *, *, #19726, .F. ) ;
#1233=ORIENTED_EDGE ( 'NONE', *, *, #37875, .T. ) ;
#1234=CARTESIAN_POINT ( 'NONE',  ( -88.78924379339714790, -193.5000000000000000, -118.3219948448692520 ) ) ;
#1236=VECTOR ( 'NONE', #14406, 1000.000000000000227 ) ;
#1239=PLANE ( 'NONE',  #145 ) ;
#1240=DIRECTION ( 'NONE',  ( 0.9785564922995060311, 0.000000000000000000, -0.2059786187410889424 ) ) ;
#1243=VECTOR ( 'NONE', #46234, 1000.000000000000000 ) ;
#1244=DIRECTION ( 'NONE',  ( 0.000000000000000000, 0.000000000000000000, 1.000000000000000000 ) ) ;
#1245=EDGE_CURVE ( 'NONE', #23736, #38723, #34435, .T. ) ;
#1246=CARTESIAN_POINT ( 'NONE',  ( 5.542374969221969039, -193.5000000000000000, 112.7238987608088365 ) ) ;
#1247=EDGE_LOOP ( 'NONE', ( #17224, #10364, #28770, #36287 ) ) ;
#1248=DIRECTION ( 'NONE',  ( 0.000000000000000000, -0.000000000000000000, 1.000000000000000000 ) ) ;
#1250=ORIENTED_EDGE ( 'NONE', *, *, #49274, .T. ) ;
#1254=CARTESIAN_POINT ( 'NONE',  ( 141.7825277784304205, -213.5000000000000000, 41.45482488023466772 ) ) ;
#1255=VECTOR ( 'NONE', #11183, 1000.000000000000000 ) ;
#1258=DIRECTION ( 'NONE',  ( 0.9785564922995032555, 0.000000000000000000, 0.2059786187411021818 ) ) ;
#1260=ADVANCED_FACE ( 'NONE', ( #11024 ), #43360, .T. ) ;
#1262=ORIENTED_EDGE ( 'NONE', *, *, #23043, .T. ) ;
#1263=DIRECTION ( 'NONE',  ( 0.000000000000000000, -1.000000000000000000, 0.000000000000000000 ) ) ;
#1264=AXIS2_PLACEMENT_3D ( 'NONE', #4825, #20847, #25057 ) ;
#1265=ORIENTED_EDGE ( 'NONE', *, *, #8650, .T. ) ;
#1267=CIRCLE ( 'NONE', #16395, 125.0000000000000000 ) ;
#1268=ORIENTED_EDGE ( 'NONE', *, *, #14115, .F. ) ;
#1269=LINE ( 'NONE', #1786, #32901 ) ;
#1272=CARTESIAN_POINT ( 'NONE',  ( -152.0588566364588132, -193.5000000000000000, -68.17212999877146729 ) ) ;
#1273=ORIENTED_EDGE ( 'NONE', *, *, #35449, .T. ) ;
#1277=CARTESIAN_POINT ( 'NONE',  ( -49.21696003055058810, -177.1207230881787780, 0.6749830015182108900 ) ) ;
#1280=CARTESIAN_POINT ( 'NONE',  ( -78.00521078983982193, -189.7472609257535510, 121.4627941443857111 ) ) ;
#1281=ORIENTED_EDGE ( 'NONE', *, *, #36487, .T. ) ;
#1282=AXIS2_PLACEMENT_3D ( 'NONE', #5837, #40755, #21323 ) ;
#1284=CIRCLE ( 'NONE', #23934, 125.0000000000000000 ) ;
#1286=CYLINDRICAL_SURFACE ( 'NONE', #37013, 125.0000000000000000 ) ;
#1287=ADVANCED_FACE ( 'NONE', ( #10509 ), #34685, .T. ) ;
#1288=DIRECTION ( 'NONE',  ( -0.000000000000000000, 1.000000000000000000, -0.000000000000000000 ) ) ;
#1290=DIRECTION ( 'NONE',  ( 0.9027978299657416494, 0.000000000000000000, 0.4300652022765245608 ) ) ;
#1291=EDGE_LOOP ( 'NONE', ( #28690, #31738, #8081, #30017 ) ) ;
#1292=AXIS2_PLACEMENT_3D ( 'NONE', #20681, #31736, #20159 ) ;
#1294=LINE ( 'NONE', #1811, #23423 ) ;
#1295=CARTESIAN_POINT ( 'NONE',  ( 41.41233698655025108, -183.6283474603465606, 86.85922373029362120 ) ) ;
#1296=VECTOR ( 'NONE', #32739, 1000.000000000000000 ) ;
#1298=DIRECTION ( 'NONE',  ( -0.000000000000000000, 1.000000000000000000, -0.000000000000000000 ) ) ;
#1300=ORIENTED_EDGE ( 'NONE', *, *, #51415, .F. ) ;
#1301=DIRECTION ( 'NONE',  ( 0.000000000000000000, 0.000000000000000000, 1.000000000000000000 ) ) ;
#1302=AXIS2_PLACEMENT_3D ( 'NONE', #21570, #13935, #41795 ) ;
#1303=CARTESIAN_POINT ( 'NONE',  ( -41.90263914168910730, -175.3837268820161057, -124.8268793598473536 ) ) ;
#1304=ORIENTED_EDGE ( 'NONE', *, *, #40768, .T. ) ;
#1305=DIRECTION ( 'NONE',  ( 0.000000000000000000, -1.000000000000000000, 0.000000000000000000 ) ) ;
#1306=ADVANCED_FACE ( 'NONE', ( #6325 ), #51257, .T. ) ;
#1307=VERTEX_POINT ( 'NONE', #39395 ) ;
#1309=DIRECTION ( 'NONE',  ( 0.000000000000000000, 0.000000000000000000, 1.000000000000000000 ) ) ;
#1311=DIRECTION ( 'NONE',  ( 0.000000000000000000, 0.000000000000000000, -1.000000000000000000 ) ) ;
#1315=VERTEX_POINT ( 'NONE', #31256 ) ;
#1317=CARTESIAN_POINT ( 'NONE',  ( -169.3144491972411458, -193.5000000000000000, -27.83926365844662243 ) ) ;
#1319=AXIS2_PLACEMENT_3D ( 'NONE', #32034, #7374, #44132 ) ;
#1320=CYLINDRICAL_SURFACE ( 'NONE', #34823, 125.0000000000000000 ) ;
#1321=AXIS2_PLACEMENT_3D ( 'NONE', #40544, #44773, #48975 ) ;
#1324=VERTEX_POINT ( 'NONE', #3403 ) ;
#1326=EDGE_CURVE ( 'NONE', #33159, #27840, #47310, .T. ) ;
#1328=CARTESIAN_POINT ( 'NONE',  ( -27.18512803868276251, -175.3837268820161057, -123.1729094355498404 ) ) ;
#1329=CARTESIAN_POINT ( 'NONE',  ( -49.03777351731249468, -183.6283474603465606, -0.8294056854502022125 ) ) ;
#1330=CYLINDRICAL_SURFACE ( 'NONE', #2156, 125.0000000000000000 ) ;
#1331=VERTEX_POINT ( 'NONE', #12050 ) ;
#1333=CARTESIAN_POINT ( 'NONE',  ( -28.74596282265200387, -183.6283474603465606, 123.4325817657431230 ) ) ;
#1336=ORIENTED_EDGE ( 'NONE', *, *, #2039, .T. ) ;
#1337=CIRCLE ( 'NONE', #12241, 125.0000000000000000 ) ;
#1339=CARTESIAN_POINT ( 'NONE',  ( -48.59739992243022755, -193.5000000000000000, 0.9929810960135230236 ) ) ;
#1340=FACE_OUTER_BOUND ( 'NONE', #45350, .T. ) ;
#1341=VECTOR ( 'NONE', #36641, 1000.000000000000114 ) ;
#1343=ORIENTED_EDGE ( 'NONE', *, *, #38802, .T. ) ;
#1347=VECTOR ( 'NONE', #15644, 1000.000000000000000 ) ;
#1350=LINE ( 'NONE', #33919, #27318 ) ;
#1352=EDGE_CURVE ( 'NONE', #50157, #51897, #16548, .T. ) ;
#1355=EDGE_CURVE ( 'NONE', #17812, #19399, #35716, .T. ) ;
#1356=DIRECTION ( 'NONE',  ( -0.000000000000000000, 1.000000000000000000, -0.000000000000000000 ) ) ;
#1357=CIRCLE ( 'NONE', #6443, 124.9999999999999858 ) ;
#1358=AXIS2_PLACEMENT_3D ( 'NONE', #26818, #2910, #38904 ) ;
#1362=ORIENTED_EDGE ( 'NONE', *, *, #1875, .F. ) ;
#1363=AXIS2_PLACEMENT_3D ( 'NONE', #49455, #13429, #21315 ) ;
#1364=AXIS2_PLACEMENT_3D ( 'NONE', #15252, #31267, #31014 ) ;
#1365=EDGE_LOOP ( 'NONE', ( #28857, #5254, #34237, #45166 ) ) ;
#1368=LINE ( 'NONE', #17925, #36265 ) ;
#1369=ORIENTED_EDGE ( 'NONE', *, *, #13916, .T. ) ;
#1370=AXIS2_PLACEMENT_3D ( 'NONE', #25566, #10325, #29765 ) ;
#1371=ORIENTED_EDGE ( 'NONE', *, *, #44149, .F. ) ;
#1374=CARTESIAN_POINT ( 'NONE',  ( -55.99477380783410041, -189.7472609257535510, 123.7720294769269742 ) ) ;
#1375=AXIS2_PLACEMENT_3D ( 'NONE', #1800, #6273, #26223 ) ;
#1377=DIRECTION ( 'NONE',  ( 0.000000000000000000, 1.000000000000000000, -0.000000000000000000 ) ) ;
#1378=AXIS2_PLACEMENT_3D ( 'NONE', #23024, #34580, #2290 ) ;
#1379=DIRECTION ( 'NONE',  ( -0.9842305779475967187, 0.000000000000000000, -0.1768902751225733538 ) ) ;
#1380=EDGE_LOOP ( 'NONE', ( #18598, #51441, #27941, #10825 ) ) ;
#1381=EDGE_CURVE ( 'NONE', #30637, #50432, #14027, .T. ) ;
#1382=CIRCLE ( 'NONE', #547, 125.0000000000000000 ) ;
#1385=ORIENTED_EDGE ( 'NONE', *, *, #18610, .T. ) ;
#1386=DIRECTION ( 'NONE',  ( 0.000000000000000000, -0.000000000000000000, -1.000000000000000000 ) ) ;
#1387=ORIENTED_EDGE ( 'NONE', *, *, #32294, .F. ) ;
#1388=CARTESIAN_POINT ( 'NONE',  ( -165.5546359831674295, -183.6283474603465606, 43.79868877201490562 ) ) ;
#1389=ORIENTED_EDGE ( 'NONE', *, *, #5272, .T. ) ;
#1390=ADVANCED_FACE ( 'NONE', ( #229 ), #43860, .T. ) ;
#1391=FACE_OUTER_BOUND ( 'NONE', #37604, .T. ) ;
#1392=CARTESIAN_POINT ( 'NONE',  ( 9.518239912201957864, -193.5000000000000000, 110.7307791902283043 ) ) ;
#1393=DIRECTION ( 'NONE',  ( -0.000000000000000000, 1.000000000000000000, -0.000000000000000000 ) ) ;
#1397=ORIENTED_EDGE ( 'NONE', *, *, #43576, .F. ) ;
#1398=CARTESIAN_POINT ( 'NONE',  ( 14.43219681437621205, -175.3837268820161057, 106.8558168688117860 ) ) ;
#1400=CARTESIAN_POINT ( 'NONE',  ( -48.47912675150885065, -175.3837268820161057, 6.938893903907228378E-15 ) ) ;
#1402=DIRECTION ( 'NONE',  ( -0.4566292373937018145, 0.000000000000000000, -0.8896570909947529859 ) ) ;
#1403=AXIS2_PLACEMENT_3D ( 'NONE', #46707, #26453, #42759 ) ;
#1404=VERTEX_POINT ( 'NONE', #4447 ) ;
#1407=VERTEX_POINT ( 'NONE', #31513 ) ;
#1409=EDGE_LOOP ( 'NONE', ( #45324, #25123, #5443, #33590 ) ) ;
#1410=VECTOR ( 'NONE', #21939, 1000.000000000000000 ) ;
#1411=FACE_OUTER_BOUND ( 'NONE', #11537, .T. ) ;
#1413=DIRECTION ( 'NONE',  ( -0.000000000000000000, 1.000000000000000000, -0.000000000000000000 ) ) ;
#1415=ORIENTED_EDGE ( 'NONE', *, *, #21138, .T. ) ;
#1416=VECTOR ( 'NONE', #47097, 1000.000000000000114 ) ;
#1417=CIRCLE ( 'NONE', #25764, 124.9999999999999858 ) ;
#1418=CARTESIAN_POINT ( 'NONE',  ( -166.6265240196292439, -193.5000000000000000, 40.81902153125349741 ) ) ;
#1419=CARTESIAN_POINT ( 'NONE',  ( 43.86477233319989466, -189.7472609257535510, -84.24728067915975771 ) ) ;
#1420=CARTESIAN_POINT ( 'NONE',  ( 72.12732647922463514, -193.5000000000000000, 28.81338593824055394 ) ) ;
#1421=AXIS2_PLACEMENT_3D ( 'NONE', #13531, #9336, #48766 ) ;
#1422=CARTESIAN_POINT ( 'NONE',  ( -171.9838957966129556, -189.7472609257535510, 19.27620354518722579 ) ) ;
#1423=ORIENTED_EDGE ( 'NONE', *, *, #37765, .F. ) ;
#1424=PLANE ( 'NONE',  #45461 ) ;
#1425=CIRCLE ( 'NONE', #36683, 124.9999999999999858 ) ;
#1426=EDGE_LOOP ( 'NONE', ( #34689, #15461, #25125, #12672 ) ) ;
#1427=VERTEX_POINT ( 'NONE', #27581 ) ;
#1428=DIRECTION ( 'NONE',  ( 0.000000000000000000, -0.000000000000000000, -1.000000000000000000 ) ) ;
#1430=VERTEX_POINT ( 'NONE', #8129 ) ;
#1431=ORIENTED_EDGE ( 'NONE', *, *, #38871, .T. ) ;
#1432=CARTESIAN_POINT ( 'NONE',  ( -48.47912675150885065, -188.5000000000000284, 15.00000000000000711 ) ) ;
#1433=LINE ( 'NONE', #13523, #32982 ) ;
#1434=AXIS2_PLACEMENT_3D ( 'NONE', #10702, #26728, #42764 ) ;
#1435=AXIS2_PLACEMENT_3D ( 'NONE', #12915, #12651, #28675 ) ;
#1437=DIRECTION ( 'NONE',  ( 0.9995608365087940150, 0.000000000000000000, 0.02963332782257007206 ) ) ;
#1438=ORIENTED_EDGE ( 'NONE', *, *, #13221, .T. ) ;
#1441=VECTOR ( 'NONE', #40097, 1000.000000000000000 ) ;
#1442=ADVANCED_FACE ( 'NONE', ( #43610 ), #32285, .T. ) ;
#1443=CARTESIAN_POINT ( 'NONE',  ( -49.29161362951453640, -177.1207230881787780, 0.5829794791144718991 ) ) ;
#1446=VERTEX_POINT ( 'NONE', #39904 ) ;
#1448=EDGE_CURVE ( 'NONE', #4651, #32642, #39181, .T. ) ;
#1452=VECTOR ( 'NONE', #32909, 1000.000000000000000 ) ;
#1454=CARTESIAN_POINT ( 'NONE',  ( 71.97629403264900816, -193.5000000000000000, -29.43839964798648268 ) ) ;
#1455=CARTESIAN_POINT ( 'NONE',  ( -22.62315034598912433, -183.6283474603465606, 121.2748789083720879 ) ) ;
#1456=ORIENTED_EDGE ( 'NONE', *, *, #49931, .F. ) ;
#1458=VECTOR ( 'NONE', #12419, 1000.000000000000000 ) ;
#1459=EDGE_CURVE ( 'NONE', #26931, #31330, #7607, .T. ) ;
#1460=EDGE_CURVE ( 'NONE', #6422, #44107, #5635, .T. ) ;
#1461=CIRCLE ( 'NONE', #44264, 125.0000000000000000 ) ;
#1464=ORIENTED_EDGE ( 'NONE', *, *, #42679, .F. ) ;
#1465=FACE_OUTER_BOUND ( 'NONE', #49649, .T. ) ;
#1466=VERTEX_POINT ( 'NONE', #15782 ) ;
#1469=DIRECTION ( 'NONE',  ( -0.000000000000000000, 1.000000000000000000, -0.000000000000000000 ) ) ;
#1472=VERTEX_POINT ( 'NONE', #28350 ) ;
#1473=CARTESIAN_POINT ( 'NONE',  ( 66.36634345758741915, -189.7472609257535510, 46.76022031560703596 ) ) ;
#1474=EDGE_LOOP ( 'NONE', ( #39536, #6604, #3195, #26345 ) ) ;
#1476=CYLINDRICAL_SURFACE ( 'NONE', #46396, 125.0000000000000000 ) ;
#1478=AXIS2_PLACEMENT_3D ( 'NONE', #9676, #2040, #17822 ) ;
#1480=ORIENTED_EDGE ( 'NONE', *, *, #21090, .F. ) ;
#1482=CARTESIAN_POINT ( 'NONE',  ( -121.1142239062970418, -193.5000000000000000, 101.7307360698549132 ) ) ;
#1484=DIRECTION ( 'NONE',  ( 0.000000000000000000, -0.000000000000000000, -1.000000000000000000 ) ) ;
#1485=LINE ( 'NONE', #44852, #45041 ) ;
#1486=CARTESIAN_POINT ( 'NONE',  ( -80.17897391495031911, -183.6283474603465606, 120.9136869416132498 ) ) ;
#1488=ORIENTED_EDGE ( 'NONE', *, *, #1518, .F. ) ;
#1490=CARTESIAN_POINT ( 'NONE',  ( -49.35486169370448550, -193.5000000000000000, -0.4827922027307481878 ) ) ;
#1491=ORIENTED_EDGE ( 'NONE', *, *, #11344, .F. ) ;
#1492=VERTEX_POINT ( 'NONE', #35991 ) ;
#1493=CARTESIAN_POINT ( 'NONE',  ( 57.12946453413545100, -193.5000000000000000, 66.87170886602000053 ) ) ;
#1496=FACE_OUTER_BOUND ( 'NONE', #51419, .T. ) ;
#1497=LINE ( 'NONE', #49596, #21745 ) ;
#1499=ORIENTED_EDGE ( 'NONE', *, *, #25402, .F. ) ;
#1500=EDGE_CURVE ( 'NONE', #31475, #26646, #15679, .T. ) ;
#1501=ADVANCED_FACE ( 'NONE', ( #31792 ), #47827, .F. ) ;
#1502=FACE_OUTER_BOUND ( 'NONE', #47137, .T. ) ;
#1503=VERTEX_POINT ( 'NONE', #31885 ) ;
#1504=ORIENTED_EDGE ( 'NONE', *, *, #23750, .F. ) ;
#1509=VECTOR ( 'NONE', #49312, 1000.000000000000000 ) ;
#1511=DIRECTION ( 'NONE',  ( -0.1768902751225592818, 0.000000000000000000, -0.9842305779475992722 ) ) ;
#1512=ADVANCED_FACE ( 'NONE', ( #47158 ), #35308, .T. ) ;
#1513=CARTESIAN_POINT ( 'NONE',  ( -46.12632737020501850, -177.1207230881787780, -123.9784823535113532 ) ) ;
#1517=EDGE_CURVE ( 'NONE', #37290, #42583, #47923, .T. ) ;
#1518=EDGE_CURVE ( 'NONE', #16167, #12446, #40015, .T. ) ;
#1523=ORIENTED_EDGE ( 'NONE', *, *, #45643, .F. ) ;
#1524=CIRCLE ( 'NONE', #51063, 125.0000000000000000 ) ;
#1526=ADVANCED_FACE ( 'NONE', ( #35827 ), #23242, .T. ) ;
#1529=DIRECTION ( 'NONE',  ( 0.000000000000000000, 0.000000000000000000, 1.000000000000000000 ) ) ;
#1530=ORIENTED_EDGE ( 'NONE', *, *, #4318, .T. ) ;
#1536=EDGE_LOOP ( 'NONE', ( #49246, #12763, #14368, #6720 ) ) ;
#1537=AXIS2_PLACEMENT_3D ( 'NONE', #40671, #219, #8630 ) ;
#1539=DIRECTION ( 'NONE',  ( -0.000000000000000000, 1.000000000000000000, 0.000000000000000000 ) ) ;
#1540=CARTESIAN_POINT ( 'NONE',  ( -31.47951320919342777, -177.1207230881787780, -122.8300162461135301 ) ) ;
#1543=ORIENTED_EDGE ( 'NONE', *, *, #21168, .F. ) ;
#1545=CARTESIAN_POINT ( 'NONE',  ( 76.09804998693969935, -189.7472609257535510, 10.27263529369908035 ) ) ;
#1547=CARTESIAN_POINT ( 'NONE',  ( -87.28630321566652128, -183.6283474603465606, 118.8234112238818483 ) ) ;
#1548=EDGE_LOOP ( 'NONE', ( #37061, #47666, #15788, #32243 ) ) ;
#1550=DIRECTION ( 'NONE',  ( 0.000000000000000000, 0.000000000000000000, 1.000000000000000000 ) ) ;
#1551=CARTESIAN_POINT ( 'NONE',  ( -157.5429198988176438, -175.3837268820161057, 61.07445476073480961 ) ) ;
#1554=EDGE_LOOP ( 'NONE', ( #48728, #48848, #29321, #42812 ) ) ;
#1555=AXIS2_PLACEMENT_3D ( 'NONE', #46658, #7224, #10650 ) ;
#1556=CIRCLE ( 'NONE', #18330, 125.0000000000000000 ) ;
#1557=VECTOR ( 'NONE', #5013, 1000.000000000000114 ) ;
#1558=FACE_OUTER_BOUND ( 'NONE', #34449, .T. ) ;
#1559=PLANE ( 'NONE',  #7687 ) ;
#1561=CARTESIAN_POINT ( 'NONE',  ( -48.47912675150885065, -177.1207230881787780, 6.938893903907228378E-15 ) ) ;
#1565=LINE ( 'NONE', #33617, #30129 ) ;
#1566=CARTESIAN_POINT ( 'NONE',  ( -19.28375372365792728, -189.7472609257535510, 121.5427093402341114 ) ) ;
#1567=DIRECTION ( 'NONE',  ( 0.000000000000000000, 0.000000000000000000, -1.000000000000000000 ) ) ;
#1568=CARTESIAN_POINT ( 'NONE',  ( -49.29161362951453640, -183.6283474603465606, 0.5829794791144718991 ) ) ;
#1569=EDGE_CURVE ( 'NONE', #44024, #49925, #28264, .T. ) ;
#1570=ADVANCED_FACE ( 'NONE', ( #27421 ), #7471, .F. ) ;
#1572=DIRECTION ( 'NONE',  ( 0.000000000000000000, 0.000000000000000000, -1.000000000000000000 ) ) ;
#1575=VERTEX_POINT ( 'NONE', #15106 ) ;
#1577=VECTOR ( 'NONE', #46399, 1000.000000000000114 ) ;
#1579=EDGE_LOOP ( 'NONE', ( #13682, #26359, #41007, #16265 ) ) ;
#1581=ORIENTED_EDGE ( 'NONE', *, *, #49509, .T. ) ;
#1583=FACE_OUTER_BOUND ( 'NONE', #3576, .T. ) ;
#1585=EDGE_CURVE ( 'NONE', #49925, #31203, #27158, .T. ) ;
#1587=DIRECTION ( 'NONE',  ( 0.000000000000000000, 0.000000000000000000, -1.000000000000000000 ) ) ;
#1589=ORIENTED_EDGE ( 'NONE', *, *, #20475, .T. ) ;
#1592=ORIENTED_EDGE ( 'NONE', *, *, #16049, .F. ) ;
#1594=EDGE_CURVE ( 'NONE', #38089, #37325, #46907, .T. ) ;
#1596=CARTESIAN_POINT ( 'NONE',  ( -32.87124591993210743, -193.5000000000000000, 124.0217483183788119 ) ) ;
#1599=VECTOR ( 'NONE', #1511, 1000.000000000000000 ) ;
#1600=ORIENTED_EDGE ( 'NONE', *, *, #14060, .T. ) ;
#1601=EDGE_CURVE ( 'NONE', #45652, #30169, #23292, .T. ) ;
#1602=CARTESIAN_POINT ( 'NONE',  ( 18.00181100848376303, -193.5000000000000000, -105.8550183720733742 ) ) ;
#1603=CARTESIAN_POINT ( 'NONE',  ( 55.91309001144630031, -183.6283474603465606, 68.75510947788670535 ) ) ;
#1605=VERTEX_POINT ( 'NONE', #9276 ) ;
#1608=AXIS2_PLACEMENT_3D ( 'NONE', #17791, #50624, #41950 ) ;
#1609=LINE ( 'NONE', #49691, #13125 ) ;
#1610=FACE_BOUND ( 'NONE', #35499, .T. ) ;
#1611=CARTESIAN_POINT ( 'NONE',  ( -159.8192355313504720, -177.1207230881787780, -56.81883646197830018 ) ) ;
#1613=CARTESIAN_POINT ( 'NONE',  ( -47.87232660569026166, -177.1207230881787780, 0.7948544414133635883 ) ) ;
#1614=FACE_OUTER_BOUND ( 'NONE', #12502, .T. ) ;
#1615=CARTESIAN_POINT ( 'NONE',  ( 38.71172987070728055, -175.3837268820161057, -89.56983042009262874 ) ) ;
#1616=CARTESIAN_POINT ( 'NONE',  ( 51.65665342072240662, -177.1207230881787780, 74.81861753132422166 ) ) ;
#1617=ORIENTED_EDGE ( 'NONE', *, *, #41907, .F. ) ;
#1618=CARTESIAN_POINT ( 'NONE',  ( -164.3791542526839180, -175.3837268820161057, 46.82076062204521349 ) ) ;
#1619=EDGE_CURVE ( 'NONE', #33402, #4, #12936, .T. ) ;
#1621=VECTOR ( 'NONE', #1192, 1000.000000000000000 ) ;
#1622=EDGE_CURVE ( 'NONE', #34403, #5990, #24777, .T. ) ;
#1624=ORIENTED_EDGE ( 'NONE', *, *, #28231, .F. ) ;
#1626=DIRECTION ( 'NONE',  ( 0.000000000000000000, 0.000000000000000000, 1.000000000000000000 ) ) ;
#1627=LINE ( 'NONE', #17664, #43724 ) ;
#1631=DIRECTION ( 'NONE',  ( 0.000000000000000000, 1.000000000000000000, 0.000000000000000000 ) ) ;
#1632=CARTESIAN_POINT ( 'NONE',  ( 54.54686566053560881, -177.1207230881787780, 69.00559874123592863 ) ) ;
#1638=ADVANCED_FACE ( 'NONE', ( #16383 ), #40795, .T. ) ;
#1639=PLANE ( 'NONE',  #41690 ) ;
#1640=ADVANCED_FACE ( 'NONE', ( #601 ), #44756, .F. ) ;
#1641=EDGE_CURVE ( 'NONE', #36857, #41966, #48448, .T. ) ;
#1643=DIRECTION ( 'NONE',  ( 0.000000000000000000, 0.000000000000000000, -1.000000000000000000 ) ) ;
#1644=ORIENTED_EDGE ( 'NONE', *, *, #44601, .F. ) ;
#1645=ORIENTED_EDGE ( 'NONE', *, *, #27554, .T. ) ;
#1647=CARTESIAN_POINT ( 'NONE',  ( 69.66827051661184100, -189.7472609257535510, -40.81902153125260213 ) ) ;
#1648=LINE ( 'NONE', #41309, #30310 ) ;
#1649=DIRECTION ( 'NONE',  ( 0.05924062789371441901, 0.000000000000000000, -0.9982437317643214625 ) ) ;
#1650=ORIENTED_EDGE ( 'NONE', *, *, #18108, .F. ) ;
#1651=AXIS2_PLACEMENT_3D ( 'NONE', #15372, #42953, #19316 ) ;
#1652=CARTESIAN_POINT ( 'NONE',  ( -58.29063029684667896, -183.6283474603465606, 124.6143426664034735 ) ) ;
#1654=ORIENTED_EDGE ( 'NONE', *, *, #39305, .F. ) ;
#1655=ADVANCED_FACE ( 'NONE', ( #16656 ), #8739, .F. ) ;
#1656=CARTESIAN_POINT ( 'NONE',  ( -48.47912675150885065, -183.6283474603465606, 6.938893903907228378E-15 ) ) ;
#1657=ORIENTED_EDGE ( 'NONE', *, *, #8173, .F. ) ;
#1658=CARTESIAN_POINT ( 'NONE',  ( -143.3583119192899744, -193.5000000000000000, -81.38144888055202841 ) ) ;
#1659=ORIENTED_EDGE ( 'NONE', *, *, #47832, .T. ) ;
#1660=DIRECTION ( 'NONE',  ( 0.000000000000000000, 0.000000000000000000, 1.000000000000000000 ) ) ;
#1661=LINE ( 'NONE', #1392, #15608 ) ;
#1664=ORIENTED_EDGE ( 'NONE', *, *, #10936, .T. ) ;
#1665=ORIENTED_EDGE ( 'NONE', *, *, #5139, .F. ) ;
#1666=CARTESIAN_POINT ( 'NONE',  ( -129.3001299485802633, -175.3837268820161057, -94.04236105995796891 ) ) ;
#1668=VECTOR ( 'NONE', #24624, 1000.000000000000000 ) ;
#1669=EDGE_LOOP ( 'NONE', ( #25620, #39974, #32774, #39054 ) ) ;
#1670=DIRECTION ( 'NONE',  ( -0.000000000000000000, -1.000000000000000000, 0.000000000000000000 ) ) ;
#1671=VERTEX_POINT ( 'NONE', #36084 ) ;
#1672=DIRECTION ( 'NONE',  ( -0.2920567706369764371, 0.000000000000000000, 0.9564009842765223146 ) ) ;
#1673=DIRECTION ( 'NONE',  ( 0.000000000000000000, 1.000000000000000000, 0.000000000000000000 ) ) ;
#1677=DIRECTION ( 'NONE',  ( -0.000000000000000000, 1.000000000000000000, -0.000000000000000000 ) ) ;
#1678=FACE_OUTER_BOUND ( 'NONE', #16337, .T. ) ;
#1680=ORIENTED_EDGE ( 'NONE', *, *, #6740, .T. ) ;
#1681=FACE_OUTER_BOUND ( 'NONE', #23617, .T. ) ;
#1682=DIRECTION ( 'NONE',  ( -0.000000000000000000, 1.000000000000000000, -0.000000000000000000 ) ) ;
#1683=PLANE ( 'NONE',  #41686 ) ;
#1684=CARTESIAN_POINT ( 'NONE',  ( -146.0653709326077490, -175.3837268820161057, -78.11481899503411341 ) ) ;
#1685=CIRCLE ( 'NONE', #22652, 125.0000000000000000 ) ;
#1688=DIRECTION ( 'NONE',  ( 0.000000000000000000, 1.000000000000000000, 0.000000000000000000 ) ) ;
#1691=DIRECTION ( 'NONE',  ( 0.000000000000000000, 0.000000000000000000, 1.000000000000000000 ) ) ;
#1692=ORIENTED_EDGE ( 'NONE', *, *, #36282, .T. ) ;
#1693=ORIENTED_EDGE ( 'NONE', *, *, #22106, .T. ) ;
#1694=DIRECTION ( 'NONE',  ( -0.000000000000000000, 1.000000000000000000, -0.000000000000000000 ) ) ;
#1697=ORIENTED_EDGE ( 'NONE', *, *, #26896, .T. ) ;
#1698=AXIS2_PLACEMENT_3D ( 'NONE', #42605, #6618, #30510 ) ;
#1700=ORIENTED_EDGE ( 'NONE', *, *, #15194, .T. ) ;
#1702=CARTESIAN_POINT ( 'NONE',  ( 64.01121016852529522, -189.7472609257535510, -54.50618404930953176 ) ) ;
#1703=PLANE ( 'NONE',  #31958 ) ;
#1705=ORIENTED_EDGE ( 'NONE', *, *, #22438, .T. ) ;
#1710=CARTESIAN_POINT ( 'NONE',  ( -171.5592422664403216, -193.5000000000000000, -21.82395850507255730 ) ) ;
#1711=CARTESIAN_POINT ( 'NONE',  ( 20.10322172534453244, -193.5000000000000000, -103.3076327631963096 ) ) ;
#1712=VERTEX_POINT ( 'NONE', #32663 ) ;
#1713=UNCERTAINTY_MEASURE_WITH_UNIT (LENGTH_MEASURE( 1.000000000000000082E-05 ), #20522, 'distance_accuracy_value', 'NONE');
#1715=VECTOR ( 'NONE', #14032, 1000.000000000000000 ) ;
#1716=ORIENTED_EDGE ( 'NONE', *, *, #3686, .F. ) ;
#1720=DIRECTION ( 'NONE',  ( -0.000000000000000000, 1.000000000000000000, -0.000000000000000000 ) ) ;
#1721=ADVANCED_FACE ( 'NONE', ( #20845 ), #48960, .T. ) ;
#1723=CARTESIAN_POINT ( 'NONE',  ( -77.77032474405883988, -189.7472609257535510, 120.4907712303052989 ) ) ;
#1724=CARTESIAN_POINT ( 'NONE',  ( -160.3527926973206661, -189.7472609257535510, -53.48161459190847467 ) ) ;
#1725=ORIENTED_EDGE ( 'NONE', *, *, #20475, .F. ) ;
#1726=CARTESIAN_POINT ( 'NONE',  ( -48.47912675150885065, -213.5000000000000000, 125.0000000000000568 ) ) ;
#1727=ADVANCED_FACE ( 'NONE', ( #859 ), #9020, .T. ) ;
#1728=ORIENTED_EDGE ( 'NONE', *, *, #38691, .F. ) ;
#1729=ORIENTED_EDGE ( 'NONE', *, *, #7976, .F. ) ;
#1730=CARTESIAN_POINT ( 'NONE',  ( 33.75048693540708911, -189.7472609257535510, 94.14505102712816154 ) ) ;
#1731=AXIS2_PLACEMENT_3D ( 'NONE', #9393, #41436, #5458 ) ;
#1732=EDGE_CURVE ( 'NONE', #23376, #3470, #13196, .T. ) ;
#1733=PLANE ( 'NONE',  #18597 ) ;
#1734=ORIENTED_EDGE ( 'NONE', *, *, #16599, .F. ) ;
#1735=CARTESIAN_POINT ( 'NONE',  ( -87.28630321566652128, -177.1207230881787780, 118.8234112238818483 ) ) ;
#1736=PLANE ( 'NONE',  #41465 ) ;
#1738=LINE ( 'NONE', #45901, #51749 ) ;
#1739=EDGE_CURVE ( 'NONE', #787, #51398, #33176, .T. ) ;
#1740=CARTESIAN_POINT ( 'NONE',  ( -160.3527926973206945, -193.5000000000000000, -53.48161459190837519 ) ) ;
#1742=ORIENTED_EDGE ( 'NONE', *, *, #10900, .F. ) ;
#1743=DIRECTION ( 'NONE',  ( 0.000000000000000000, -0.000000000000000000, -1.000000000000000000 ) ) ;
#1745=VECTOR ( 'NONE', #50030, 1000.000000000000000 ) ;
#1747=CARTESIAN_POINT ( 'NONE',  ( -168.4003408533108086, -183.6283474603465606, -35.26900067126609173 ) ) ;
#1748=EDGE_CURVE ( 'NONE', #24620, #11600, #35022, .T. ) ;
#1749=ORIENTED_EDGE ( 'NONE', *, *, #19202, .F. ) ;
#1751=AXIS2_PLACEMENT_3D ( 'NONE', #32827, #1024, #48879 ) ;
#1753=ADVANCED_FACE ( 'NONE', ( #14258 ), #37651, .T. ) ;
#1754=DIRECTION ( 'NONE',  ( -0.000000000000000000, 1.000000000000000000, -0.000000000000000000 ) ) ;
#1755=CARTESIAN_POINT ( 'NONE',  ( -48.47912675150885065, -175.3837268820161057, 6.938893903907228378E-15 ) ) ;
#1757=CARTESIAN_POINT ( 'NONE',  ( 76.51419089073348800, -183.6283474603465606, -1.292495564988658030 ) ) ;
#1758=VERTEX_POINT ( 'NONE', #22138 ) ;
#1761=PLANE ( 'NONE',  #9145 ) ;
#1762=LINE ( 'NONE', #12804, #36908 ) ;
#1763=CIRCLE ( 'NONE', #43702, 125.0000000000000000 ) ;
#1764=ADVANCED_FACE ( 'NONE', ( #25550 ), #13731, .F. ) ;
#1771=PLANE ( 'NONE',  #17215 ) ;
#1772=VERTEX_POINT ( 'NONE', #33947 ) ;
#1773=VERTEX_POINT ( 'NONE', #2430 ) ;
#1774=VERTEX_POINT ( 'NONE', #18201 ) ;
#1775=DIRECTION ( 'NONE',  ( 0.000000000000000000, 0.000000000000000000, 1.000000000000000000 ) ) ;
#1777=CIRCLE ( 'NONE', #28590, 125.0000000000000000 ) ;
#1778=EDGE_LOOP ( 'NONE', ( #14927, #1845, #30448, #207 ) ) ;
#1780=CARTESIAN_POINT ( 'NONE',  ( -137.9639882952644712, -183.6283474603465606, 87.27805883780237650 ) ) ;
#1781=VERTEX_POINT ( 'NONE', #5604 ) ;
#1782=CARTESIAN_POINT ( 'NONE',  ( -166.1003692892502102, -183.6283474603465606, -42.31126686685032467 ) ) ;
#1783=ORIENTED_EDGE ( 'NONE', *, *, #1517, .F. ) ;
#1785=ORIENTED_EDGE ( 'NONE', *, *, #48329, .T. ) ;
#1786=CARTESIAN_POINT ( 'NONE',  ( 141.7825277784304205, -193.5000000000000000, 41.45482488023466772 ) ) ;
#1787=DIRECTION ( 'NONE',  ( -0.000000000000000000, 1.000000000000000000, -0.000000000000000000 ) ) ;
#1790=ORIENTED_EDGE ( 'NONE', *, *, #41593, .T. ) ;
#1792=DIRECTION ( 'NONE',  ( -0.000000000000000000, 1.000000000000000000, -0.000000000000000000 ) ) ;
#1793=ADVANCED_FACE ( 'NONE', ( #42622 ), #49500, .T. ) ;
#1794=EDGE_CURVE ( 'NONE', #46340, #41311, #39223, .T. ) ;
#1795=PLANE ( 'NONE',  #271 ) ;
#1797=ORIENTED_EDGE ( 'NONE', *, *, #14382, .F. ) ;
#1798=CARTESIAN_POINT ( 'NONE',  ( -172.4465090799742484, -175.3837268820161057, -2.844930291600662908 ) ) ;
#1799=FACE_OUTER_BOUND ( 'NONE', #32616, .T. ) ;
#1800=CARTESIAN_POINT ( 'NONE',  ( -49.08592689732745384, -175.3837268820161057, 0.7948544414133550395 ) ) ;
#1803=DIRECTION ( 'NONE',  ( 0.000000000000000000, 1.000000000000000000, 0.000000000000000000 ) ) ;
#1804=DIRECTION ( 'NONE',  ( -0.000000000000000000, -1.000000000000000000, 0.000000000000000000 ) ) ;
#1805=CARTESIAN_POINT ( 'NONE',  ( -48.47912675150885065, -183.6283474603465606, 6.938893903907228378E-15 ) ) ;
#1806=VERTEX_POINT ( 'NONE', #34472 ) ;
#1808=ADVANCED_FACE ( 'NONE', ( #17692 ), #10307, .T. ) ;
#1811=CARTESIAN_POINT ( 'NONE',  ( 11.61413489515543418, -193.5000000000000000, -109.6074810615842381 ) ) ;
#1814=FACE_OUTER_BOUND ( 'NONE', #30369, .T. ) ;
#1818=CIRCLE ( 'NONE', #21103, 125.0000000000000000 ) ;
#1820=ORIENTED_EDGE ( 'NONE', *, *, #1619, .F. ) ;
#1821=AXIS2_PLACEMENT_3D ( 'NONE', #19278, #7447, #47383 ) ;
#1822=FACE_OUTER_BOUND ( 'NONE', #37747, .T. ) ;
#1823=ORIENTED_EDGE ( 'NONE', *, *, #22345, .F. ) ;
#1824=EDGE_CURVE ( 'NONE', #48760, #20039, #27474, .T. ) ;
#1825=CARTESIAN_POINT ( 'NONE',  ( -169.6719064342497916, -177.1207230881787780, 30.61552143554989414 ) ) ;
#1826=ORIENTED_EDGE ( 'NONE', *, *, #21827, .F. ) ;
#1827=DIRECTION ( 'NONE',  ( 0.000000000000000000, -1.000000000000000000, 0.000000000000000000 ) ) ;
#1828=VERTEX_POINT ( 'NONE', #49740 ) ;
#1829=VECTOR ( 'NONE', #24491, 1000.000000000000000 ) ;
#1830=FACE_OUTER_BOUND ( 'NONE', #26391, .T. ) ;
#1831=DIRECTION ( 'NONE',  ( -0.05924062789372142729, 0.000000000000000000, 0.9982437317643209074 ) ) ;
#1832=EDGE_LOOP ( 'NONE', ( #9607, #5027, #18686, #29002 ) ) ;
#1833=CARTESIAN_POINT ( 'NONE',  ( 62.13187335169531877, -183.6283474603465606, -58.22548115875871844 ) ) ;
#1838=ORIENTED_EDGE ( 'NONE', *, *, #18840, .T. ) ;
#1840=ORIENTED_EDGE ( 'NONE', *, *, #43935, .F. ) ;
#1843=CARTESIAN_POINT ( 'NONE',  ( -47.87232660569026166, -193.5000000000000000, 0.7948544414133635883 ) ) ;
#1844=ORIENTED_EDGE ( 'NONE', *, *, #39099, .T. ) ;
#1845=ORIENTED_EDGE ( 'NONE', *, *, #15707, .T. ) ;
#1847=ORIENTED_EDGE ( 'NONE', *, *, #37755, .T. ) ;
#1849=CARTESIAN_POINT ( 'NONE',  ( -170.9948556092908518, -175.3837268820161057, 19.12855698118476511 ) ) ;
#1850=ORIENTED_EDGE ( 'NONE', *, *, #38795, .F. ) ;
#1852=PLANE ( 'NONE',  #43357 ) ;
#1853=CARTESIAN_POINT ( 'NONE',  ( -126.8597349762179363, -183.6283474603465606, -96.08646119223961080 ) ) ;
#1854=VECTOR ( 'NONE', #46525, 999.9999999999998863 ) ;
#1857=EDGE_CURVE ( 'NONE', #27687, #15211, #7648, .T. ) ;
#1858=ORIENTED_EDGE ( 'NONE', *, *, #14910, .T. ) ;
#1860=AXIS2_PLACEMENT_3D ( 'NONE', #20882, #362, #28732 ) ;
#1862=CARTESIAN_POINT ( 'NONE',  ( 30.05499637021958392, -177.1207230881787780, -97.24912084693205827 ) ) ;
#1863=EDGE_CURVE ( 'NONE', #34248, #50432, #27093, .T. ) ;
#1866=VERTEX_POINT ( 'NONE', #2929 ) ;
#1869=DIRECTION ( 'NONE',  ( 0.000000000000000000, 0.000000000000000000, -1.000000000000000000 ) ) ;
#1872=EDGE_CURVE ( 'NONE', #18062, #31552, #18967, .T. ) ;
#1873=VECTOR ( 'NONE', #24437, 1000.000000000000000 ) ;
#1874=AXIS2_PLACEMENT_3D ( 'NONE', #3336, #35914, #19621 ) ;
#1875=EDGE_CURVE ( 'NONE', #31640, #9002, #31299, .T. ) ;
#1876=DIRECTION ( 'NONE',  ( 0.000000000000000000, 0.000000000000000000, 1.000000000000000000 ) ) ;
#1877=AXIS2_PLACEMENT_3D ( 'NONE', #1277, #24674, #489 ) ;
#1880=LINE ( 'NONE', #2407, #26158 ) ;
#1881=DIRECTION ( 'NONE',  ( -0.9646355819083614058, 0.000000000000000000, 0.2635871660690581320 ) ) ;
#1882=CARTESIAN_POINT ( 'NONE',  ( 71.44208735029287993, -193.5000000000000000, 35.26900067126700833 ) ) ;
#1884=EDGE_CURVE ( 'NONE', #29517, #13511, #23667, .T. ) ;
#1885=ORIENTED_EDGE ( 'NONE', *, *, #18794, .F. ) ;
#1887=DIRECTION ( 'NONE',  ( 0.000000000000000000, 1.000000000000000000, 0.000000000000000000 ) ) ;
#1888=DIRECTION ( 'NONE',  ( -0.1768902751225802927, 0.000000000000000000, 0.9842305779475953864 ) ) ;
#1889=ORIENTED_EDGE ( 'NONE', *, *, #2045, .T. ) ;
#1890=EDGE_LOOP ( 'NONE', ( #11084, #37044, #22681, #14693 ) ) ;
#1891=VERTEX_POINT ( 'NONE', #22657 ) ;
#1892=DIRECTION ( 'NONE',  ( 0.000000000000000000, -0.000000000000000000, -1.000000000000000000 ) ) ;
#1893=CIRCLE ( 'NONE', #11110, 125.0000000000000000 ) ;
#1894=FACE_OUTER_BOUND ( 'NONE', #25378, .T. ) ;
#1895=LINE ( 'NONE', #6114, #25506 ) ;
#1896=ORIENTED_EDGE ( 'NONE', *, *, #8682, .T. ) ;
#1897=EDGE_CURVE ( 'NONE', #31784, #30580, #42556, .T. ) ;
#1898=VECTOR ( 'NONE', #49414, 1000.000000000000000 ) ;
#1899=CARTESIAN_POINT ( 'NONE',  ( -166.9790462269952229, -183.6283474603465606, 36.52255268223130713 ) ) ;
#1901=ORIENTED_EDGE ( 'NONE', *, *, #33781, .F. ) ;
#1902=CARTESIAN_POINT ( 'NONE',  ( 43.57032560458359427, -175.3837268820161057, 83.08371579725745448 ) ) ;
#1903=ORIENTED_EDGE ( 'NONE', *, *, #6379, .T. ) ;
#1906=DIRECTION ( 'NONE',  ( 0.000000000000000000, -1.000000000000000000, 0.000000000000000000 ) ) ;
#1907=LINE ( 'NONE', #30284, #42263 ) ;
#1909=VECTOR ( 'NONE', #42535, 1000.000000000000000 ) ;
#1910=VECTOR ( 'NONE', #46145, 1000.000000000000000 ) ;
#1911=EDGE_LOOP ( 'NONE', ( #49021, #35930, #48876, #34096 ) ) ;
#1914=VERTEX_POINT ( 'NONE', #11065 ) ;
#1915=AXIS2_PLACEMENT_3D ( 'NONE', #1931, #29773, #33730 ) ;
#1917=CARTESIAN_POINT ( 'NONE',  ( 53.18081239921338721, -175.3837268820161057, -72.73415134495935774 ) ) ;
#1918=VERTEX_POINT ( 'NONE', #34725 ) ;
#1919=LINE ( 'NONE', #30290, #29956 ) ;
#1922=ORIENTED_EDGE ( 'NONE', *, *, #5475, .T. ) ;
#1924=VECTOR ( 'NONE', #39357, 1000.000000000000000 ) ;
#1926=EDGE_CURVE ( 'NONE', #44533, #27697, #19905, .T. ) ;
#1931=CARTESIAN_POINT ( 'NONE',  ( 19.33815737959698566, -193.5000000000000000, 105.0038855142078233 ) ) ;
#1932=CYLINDRICAL_SURFACE ( 'NONE', #30648, 124.9999999999999858 ) ;
#1933=DIRECTION ( 'NONE',  ( 0.000000000000000000, 1.000000000000000000, -0.000000000000000000 ) ) ;
#1934=VERTEX_POINT ( 'NONE', #43654 ) ;
#1935=AXIS2_PLACEMENT_3D ( 'NONE', #1986, #6721, #18026 ) ;
#1938=DIRECTION ( 'NONE',  ( -0.000000000000000000, 1.000000000000000000, -0.000000000000000000 ) ) ;
#1941=ORIENTED_EDGE ( 'NONE', *, *, #32061, .F. ) ;
#1942=LINE ( 'NONE', #42660, #19538 ) ;
#1943=EDGE_LOOP ( 'NONE', ( #11528, #24173, #21189, #38544 ) ) ;
#1944=ADVANCED_FACE ( 'NONE', ( #14779 ), #51815, .T. ) ;
#1945=CARTESIAN_POINT ( 'NONE',  ( -48.47912675150885065, -183.6283474603465606, 6.938893903907228378E-15 ) ) ;
#1946=CARTESIAN_POINT ( 'NONE',  ( 1.352451982137498288, -175.3837268820161057, 113.5465278748097120 ) ) ;
#1949=ORIENTED_EDGE ( 'NONE', *, *, #19178, .F. ) ;
#1952=ADVANCED_FACE ( 'NONE', ( #20507 ), #12362, .F. ) ;
#1955=ORIENTED_EDGE ( 'NONE', *, *, #25292, .T. ) ;
#1957=ORIENTED_EDGE ( 'NONE', *, *, #24495, .F. ) ;
#1958=CARTESIAN_POINT ( 'NONE',  ( 141.7825277784304205, -213.5000000000000000, -41.45482488023466061 ) ) ;
#1960=CIRCLE ( 'NONE', #9507, 125.0000000000000000 ) ;
#1963=ORIENTED_EDGE ( 'NONE', *, *, #18900, .T. ) ;
#1964=ORIENTED_EDGE ( 'NONE', *, *, #34614, .F. ) ;
#1966=CARTESIAN_POINT ( 'NONE',  ( 67.04262753014327814, -193.5000000000000000, -47.74645837849745078 ) ) ;
#1967=LINE ( 'NONE', #41909, #51215 ) ;
#1969=DIRECTION ( 'NONE',  ( 0.000000000000000000, 0.000000000000000000, -1.000000000000000000 ) ) ;
#1971=EDGE_LOOP ( 'NONE', ( #5226, #20764, #28467, #41892 ) ) ;
#1972=VECTOR ( 'NONE', #21782, 999.9999999999998863 ) ;
#1975=ORIENTED_EDGE ( 'NONE', *, *, #11541, .T. ) ;
#1978=CARTESIAN_POINT ( 'NONE',  ( 70.20858612167234014, -193.5000000000000000, 35.90758392117750475 ) ) ;
#1982=ORIENTED_EDGE ( 'NONE', *, *, #45039, .F. ) ;
#1984=ORIENTED_EDGE ( 'NONE', *, *, #32401, .F. ) ;
#1985=EDGE_LOOP ( 'NONE', ( #5666, #21081, #8976, #23007 ) ) ;
#1986=CARTESIAN_POINT ( 'NONE',  ( -48.47912675150885065, -177.1207230881787780, 6.938893903907228378E-15 ) ) ;
#1988=CARTESIAN_POINT ( 'NONE',  ( -37.67038537088846084, -193.5000000000000000, -124.5318076226586470 ) ) ;
#1989=ORIENTED_EDGE ( 'NONE', *, *, #51641, .F. ) ;
#1990=PLANE ( 'NONE',  #15601 ) ;
#1991=LINE ( 'NONE', #24874, #37273 ) ;
#1992=CARTESIAN_POINT ( 'NONE',  ( -77.03256798524175508, -193.5000000000000000, 121.6951149130964893 ) ) ;
#1994=FACE_OUTER_BOUND ( 'NONE', #3922, .T. ) ;
#1995=ORIENTED_EDGE ( 'NONE', *, *, #26288, .T. ) ;
#1997=DIRECTION ( 'NONE',  ( -0.000000000000000000, 1.000000000000000000, -0.000000000000000000 ) ) ;
#1998=EDGE_LOOP ( 'NONE', ( #183, #26411, #20566, #24622, #17383, #13588, #43539, #23784, #24926, #42730, #22517, #11040, #16486, #25501, #28493, #28545 ) ) ;
#2001=DIRECTION ( 'NONE',  ( 0.3482016354344059095, 0.000000000000000000, -0.9374196611341183427 ) ) ;
#2003=VECTOR ( 'NONE', #50671, 1000.000000000000000 ) ;
#2006=DIRECTION ( 'NONE',  ( -0.9027978299657387629, 0.000000000000000000, -0.4300652022765304450 ) ) ;
#2012=VECTOR ( 'NONE', #17562, 1000.000000000000114 ) ;
#2014=ORIENTED_EDGE ( 'NONE', *, *, #47509, .F. ) ;
#2015=ORIENTED_EDGE ( 'NONE', *, *, #42050, .T. ) ;
#2016=ORIENTED_EDGE ( 'NONE', *, *, #51904, .F. ) ;
#2017=DIRECTION ( 'NONE',  ( -0.000000000000000000, 1.000000000000000000, 0.000000000000000000 ) ) ;
#2018=DIRECTION ( 'NONE',  ( -0.9995608365087946812, 0.000000000000000000, 0.02963332782254913048 ) ) ;
#2019=PLANE ( 'NONE',  #17588 ) ;
#2020=CARTESIAN_POINT ( 'NONE',  ( -120.5074237604784315, -177.1207230881787780, 100.9358816284415781 ) ) ;
#2024=CARTESIAN_POINT ( 'NONE',  ( -141.2664123866436512, -189.7472609257535510, -83.75869879877495805 ) ) ;
#2025=ORIENTED_EDGE ( 'NONE', *, *, #35634, .T. ) ;
#2026=CARTESIAN_POINT ( 'NONE',  ( -48.47912675150885065, -189.7472609257535510, 6.938893903907228378E-15 ) ) ;
#2028=ORIENTED_EDGE ( 'NONE', *, *, #12541, .F. ) ;
#2030=EDGE_LOOP ( 'NONE', ( #1657, #44514, #47588, #33493 ) ) ;
#2031=DIRECTION ( 'NONE',  ( -0.000000000000000000, 1.000000000000000000, -0.000000000000000000 ) ) ;
#2032=VECTOR ( 'NONE', #85, 1000.000000000000000 ) ;
#2035=FACE_OUTER_BOUND ( 'NONE', #23237, .T. ) ;
#2036=EDGE_CURVE ( 'NONE', #28777, #33835, #10716, .T. ) ;
#2037=DIRECTION ( 'NONE',  ( -0.4031234292879792847, 0.000000000000000000, 0.9151456172430153524 ) ) ;
#2038=ORIENTED_EDGE ( 'NONE', *, *, #26229, .T. ) ;
#2039=EDGE_CURVE ( 'NONE', #24589, #21989, #4230, .T. ) ;
#2040=DIRECTION ( 'NONE',  ( 0.000000000000000000, -1.000000000000000000, 0.000000000000000000 ) ) ;
#2041=ORIENTED_EDGE ( 'NONE', *, *, #7479, .F. ) ;
#2042=CIRCLE ( 'NONE', #39797, 125.0000000000000000 ) ;
#2043=ORIENTED_EDGE ( 'NONE', *, *, #3488, .T. ) ;
#2044=CARTESIAN_POINT ( 'NONE',  ( -88.23625491228469286, -177.1207230881787780, 118.5089480183148254 ) ) ;
#2045=EDGE_CURVE ( 'NONE', #33001, #21060, #49330, .T. ) ;
#2046=DIRECTION ( 'NONE',  ( -0.000000000000000000, 1.000000000000000000, -0.000000000000000000 ) ) ;
#2049=DIRECTION ( 'NONE',  ( 0.000000000000000000, -1.000000000000000000, 0.000000000000000000 ) ) ;
#2051=CARTESIAN_POINT ( 'NONE',  ( -111.3295483157475445, -175.3837268820161057, 108.0501018472332504 ) ) ;
#2053=ORIENTED_EDGE ( 'NONE', *, *, #17300, .F. ) ;
#2054=AXIS2_PLACEMENT_3D ( 'NONE', #46645, #14851, #6948 ) ;
#2055=DIRECTION ( 'NONE',  ( 0.000000000000000000, -0.000000000000000000, -1.000000000000000000 ) ) ;
#2058=ORIENTED_EDGE ( 'NONE', *, *, #5070, .T. ) ;
#2061=DIRECTION ( 'NONE',  ( 0.000000000000000000, 0.000000000000000000, -1.000000000000000000 ) ) ;
#2062=EDGE_LOOP ( 'NONE', ( #4658, #12449, #38211, #24993 ) ) ;
#2063=CARTESIAN_POINT ( 'NONE',  ( -163.3245969606054473, -175.3837268820161057, -46.76022031560624015 ) ) ;
#2065=DIRECTION ( 'NONE',  ( 0.000000000000000000, 0.000000000000000000, 1.000000000000000000 ) ) ;
#2066=CARTESIAN_POINT ( 'NONE',  ( 70.98542830588607444, -177.1207230881787780, -36.78613984829961936 ) ) ;
#2067=DIRECTION ( 'NONE',  ( 0.000000000000000000, 1.000000000000000000, 0.000000000000000000 ) ) ;
#2068=CIRCLE ( 'NONE', #22220, 125.0000000000000000 ) ;
#2069=AXIS2_PLACEMENT_3D ( 'NONE', #33598, #33076, #49122 ) ;
#2070=CARTESIAN_POINT ( 'NONE',  ( -135.4449840867448813, -175.3837268820161057, -88.39086586114741806 ) ) ;
#2071=DIRECTION ( 'NONE',  ( 0.000000000000000000, 0.000000000000000000, 1.000000000000000000 ) ) ;
#2072=ORIENTED_EDGE ( 'NONE', *, *, #42858, .T. ) ;
#2073=AXIS2_PLACEMENT_3D ( 'NONE', #8206, #4261, #7684 ) ;
#2076=DIRECTION ( 'NONE',  ( -0.000000000000000000, 1.000000000000000000, -0.000000000000000000 ) ) ;
#2077=VERTEX_POINT ( 'NONE', #36808 ) ;
#2079=DIRECTION ( 'NONE',  ( 0.9929810960135178055, 0.000000000000000000, -0.1182731709213592358 ) ) ;
#2080=EDGE_CURVE ( 'NONE', #11778, #9277, #42598, .T. ) ;
#2081=CIRCLE ( 'NONE', #7973, 125.0000000000000000 ) ;
#2082=PLANE ( 'NONE',  #36811 ) ;
#2084=DIRECTION ( 'NONE',  ( 0.000000000000000000, 0.000000000000000000, -1.000000000000000000 ) ) ;
#2085=VERTEX_POINT ( 'NONE', #4491 ) ;
#2086=LINE ( 'NONE', #14200, #33435 ) ;
#2087=DIRECTION ( 'NONE',  ( 0.000000000000000000, 0.000000000000000000, -1.000000000000000000 ) ) ;
#2089=DIRECTION ( 'NONE',  ( 0.1182731709213523247, 0.000000000000000000, 0.9929810960135185827 ) ) ;
#2090=ORIENTED_EDGE ( 'NONE', *, *, #48491, .F. ) ;
#2091=DIRECTION ( 'NONE',  ( 0.000000000000000000, 0.000000000000000000, -1.000000000000000000 ) ) ;
#2094=CARTESIAN_POINT ( 'NONE',  ( 43.18784210722336780, -193.5000000000000000, -84.98333260264752198 ) ) ;
#2097=ORIENTED_EDGE ( 'NONE', *, *, #23885, .F. ) ;
#2099=EDGE_CURVE ( 'NONE', #40342, #34406, #37057, .T. ) ;
#2100=DIRECTION ( 'NONE',  ( 0.000000000000000000, 0.000000000000000000, -1.000000000000000000 ) ) ;
#2102=CARTESIAN_POINT ( 'NONE',  ( -45.12595152424214717, -177.1207230881787780, -123.9551692589637355 ) ) ;
#2103=EDGE_CURVE ( 'NONE', #5601, #15102, #31679, .T. ) ;
#2105=DIRECTION ( 'NONE',  ( -0.1768902751225802927, 0.000000000000000000, 0.9842305779475953864 ) ) ;
#2106=ORIENTED_EDGE ( 'NONE', *, *, #22584, .F. ) ;
#2107=CARTESIAN_POINT ( 'NONE',  ( 76.43863189440992301, -193.5000000000000000, -4.533605064403313456 ) ) ;
#2108=DIRECTION ( 'NONE',  ( 0.000000000000000000, 0.000000000000000000, 1.000000000000000000 ) ) ;
#2109=DIRECTION ( 'NONE',  ( 0.000000000000000000, -1.000000000000000000, -0.000000000000000000 ) ) ;
#2110=CARTESIAN_POINT ( 'NONE',  ( -162.7543581613524282, -177.1207230881787780, 50.65739320402010293 ) ) ;
#2112=LINE ( 'NONE', #34687, #2235 ) ;
#2114=ORIENTED_EDGE ( 'NONE', *, *, #17253, .F. ) ;
#2116=CARTESIAN_POINT ( 'NONE',  ( 71.44208735029287993, -193.5000000000000000, 35.26900067126700833 ) ) ;
#2117=VECTOR ( 'NONE', #32241, 1000.000000000000000 ) ;
#2118=DIRECTION ( 'NONE',  ( 0.000000000000000000, -0.000000000000000000, -1.000000000000000000 ) ) ;
#2122=AXIS2_PLACEMENT_3D ( 'NONE', #25183, #5984, #17568 ) ;
#2124=CARTESIAN_POINT ( 'NONE',  ( -76.79768193946081567, -189.7472609257535510, 120.7230919990160629 ) ) ;
#2125=DIRECTION ( 'NONE',  ( -0.8455960035018272869, 0.000000000000000000, 0.5338233779647886257 ) ) ;
#2126=CIRCLE ( 'NONE', #11346, 124.9999999999999858 ) ;
#2128=CIRCLE ( 'NONE', #24792, 125.0000000000000000 ) ;
#2129=CARTESIAN_POINT ( 'NONE',  ( -129.4514457347087273, -189.7472609257535510, 95.22858582633115532 ) ) ;
#2130=DIRECTION ( 'NONE',  ( 0.000000000000000000, -0.000000000000000000, 1.000000000000000000 ) ) ;
#2132=EDGE_LOOP ( 'NONE', ( #33701, #19771, #39541, #1015 ) ) ;
#2134=CARTESIAN_POINT ( 'NONE',  ( -48.47912675150885065, -177.1207230881787780, 6.938893903907228378E-15 ) ) ;
#2135=LINE ( 'NONE', #5331, #21984 ) ;
#2136=ORIENTED_EDGE ( 'NONE', *, *, #14737, .T. ) ;
#2137=EDGE_LOOP ( 'NONE', ( #2561, #78, #22612, #13279 ) ) ;
#2138=AXIS2_PLACEMENT_3D ( 'NONE', #39710, #3723, #28411 ) ;
#2139=ORIENTED_EDGE ( 'NONE', *, *, #42202, .F. ) ;
#2140=LINE ( 'NONE', #26062, #48572 ) ;
#2141=AXIS2_PLACEMENT_3D ( 'NONE', #4836, #36098, #32677 ) ;
#2142=VECTOR ( 'NONE', #41033, 1000.000000000000000 ) ;
#2144=ADVANCED_FACE ( 'NONE', ( #13154 ), #49936, .T. ) ;
#2146=DIRECTION ( 'NONE',  ( 0.000000000000000000, 0.000000000000000000, -1.000000000000000000 ) ) ;
#2147=CARTESIAN_POINT ( 'NONE',  ( -47.50057025920934706, -193.5000000000000000, 0.2059786187411091207 ) ) ;
#2148=ORIENTED_EDGE ( 'NONE', *, *, #17541, .T. ) ;
#2149=EDGE_CURVE ( 'NONE', #35111, #467, #45480, .T. ) ;
#2151=CARTESIAN_POINT ( 'NONE',  ( -18.54723674587610560, -175.3837268820161057, 120.3332351033025702 ) ) ;
#2152=DIRECTION ( 'NONE',  ( -0.000000000000000000, 1.000000000000000000, -0.000000000000000000 ) ) ;
#2153=DIRECTION ( 'NONE',  ( 0.000000000000000000, 0.000000000000000000, 1.000000000000000000 ) ) ;
#2156=AXIS2_PLACEMENT_3D ( 'NONE', #1843, #26531, #17388 ) ;
#2158=CIRCLE ( 'NONE', #26462, 125.0000000000000000 ) ;
#2166=DIRECTION ( 'NONE',  ( 0.000000000000000000, 0.000000000000000000, 1.000000000000000000 ) ) ;
#2169=AXIS2_PLACEMENT_3D ( 'NONE', #27163, #26913, #21756 ) ;
#2172=DIRECTION ( 'NONE',  ( 0.000000000000000000, -1.000000000000000000, 0.000000000000000000 ) ) ;
#2173=EDGE_CURVE ( 'NONE', #23894, #7466, #29954, .T. ) ;
#2174=LINE ( 'NONE', #6137, #44325 ) ;
#2175=VERTEX_POINT ( 'NONE', #14201 ) ;
#2176=LINE ( 'NONE', #34241, #43353 ) ;
#2177=ADVANCED_FACE ( 'NONE', ( #25759 ), #22068, .T. ) ;
#2178=ORIENTED_EDGE ( 'NONE', *, *, #4779, .F. ) ;
#2181=ORIENTED_EDGE ( 'NONE', *, *, #15241, .F. ) ;
#2182=DIRECTION ( 'NONE',  ( 0.000000000000000000, 1.000000000000000000, 0.000000000000000000 ) ) ;
#2183=ORIENTED_EDGE ( 'NONE', *, *, #5257, .T. ) ;
#2184=CIRCLE ( 'NONE', #42431, 125.0000000000000000 ) ;
#2186=DIRECTION ( 'NONE',  ( 0.05924062789372142729, 0.000000000000000000, -0.9982437317643209074 ) ) ;
#2189=AXIS2_PLACEMENT_3D ( 'NONE', #51766, #24168, #16022 ) ;
#2190=AXIS2_PLACEMENT_3D ( 'NONE', #2950, #14798, #2446 ) ;
#2193=DIRECTION ( 'NONE',  ( -0.000000000000000000, 1.000000000000000000, -0.000000000000000000 ) ) ;
#2194=ADVANCED_FACE ( 'NONE', ( #17875 ), #34415, .F. ) ;
#2195=EDGE_LOOP ( 'NONE', ( #8009, #47301, #15968, #2015 ) ) ;
#2197=ORIENTED_EDGE ( 'NONE', *, *, #48323, .T. ) ;
#2198=CIRCLE ( 'NONE', #4753, 125.0000000000000000 ) ;
#2204=CIRCLE ( 'NONE', #11538, 125.0000000000000000 ) ;
#2205=ORIENTED_EDGE ( 'NONE', *, *, #34534, .F. ) ;
#2206=DIRECTION ( 'NONE',  ( -0.9646355819083556327, 0.000000000000000000, -0.2635871660690782825 ) ) ;
#2207=AXIS2_PLACEMENT_3D ( 'NONE', #30730, #26794, #13685 ) ;
#2208=VECTOR ( 'NONE', #14856, 1000.000000000000000 ) ;
#2209=EDGE_CURVE ( 'NONE', #47040, #41966, #11300, .T. ) ;
#2213=ORIENTED_EDGE ( 'NONE', *, *, #24726, .T. ) ;
#2215=CARTESIAN_POINT ( 'NONE',  ( 72.89680503569744019, -189.7472609257535510, -25.37485791684303393 ) ) ;
#2217=EDGE_CURVE ( 'NONE', #46918, #35839, #50792, .T. ) ;
#2218=EDGE_CURVE ( 'NONE', #10123, #9353, #50208, .T. ) ;
#2219=EDGE_CURVE ( 'NONE', #24784, #51869, #10240, .T. ) ;
#2220=DIRECTION ( 'NONE',  ( 0.000000000000000000, 1.000000000000000000, -0.000000000000000000 ) ) ;
#2222=VERTEX_POINT ( 'NONE', #6304 ) ;
#2223=EDGE_LOOP ( 'NONE', ( #35752, #2510, #22672, #6847 ) ) ;
#2224=EDGE_CURVE ( 'NONE', #47240, #1828, #23907, .T. ) ;
#2227=LINE ( 'NONE', #14318, #31906 ) ;
#2230=EDGE_CURVE ( 'NONE', #41581, #27267, #31452, .T. ) ;
#2234=ORIENTED_EDGE ( 'NONE', *, *, #2553, .T. ) ;
#2235=VECTOR ( 'NONE', #22867, 999.9999999999998863 ) ;
#2236=EDGE_CURVE ( 'NONE', #20990, #18846, #14455, .T. ) ;
#2237=PLANE ( 'NONE',  #6429 ) ;
#2239=ORIENTED_EDGE ( 'NONE', *, *, #33660, .T. ) ;
#2242=AXIS2_PLACEMENT_3D ( 'NONE', #9038, #24282, #12444 ) ;
#2243=EDGE_CURVE ( 'NONE', #38668, #12031, #16385, .T. ) ;
#2244=DIRECTION ( 'NONE',  ( -0.05924062789372142729, 0.000000000000000000, 0.9982437317643209074 ) ) ;
#2246=DIRECTION ( 'NONE',  ( 0.000000000000000000, 1.000000000000000000, -0.000000000000000000 ) ) ;
#2247=AXIS2_PLACEMENT_3D ( 'NONE', #18861, #2837, #43043 ) ;
#2248=CIRCLE ( 'NONE', #8958, 125.0000000000000000 ) ;
#2249=EDGE_CURVE ( 'NONE', #15667, #19112, #3129, .T. ) ;
#2251=DIRECTION ( 'NONE',  ( 0.000000000000000000, 0.000000000000000000, 1.000000000000000000 ) ) ;
#2253=CARTESIAN_POINT ( 'NONE',  ( -163.4524646452521210, -189.7472609257535510, 46.44493303993096589 ) ) ;
#2254=AXIS2_PLACEMENT_3D ( 'NONE', #31687, #44306, #15153 ) ;
#2256=ADVANCED_FACE ( 'NONE', ( #39376 ), #26517, .T. ) ;
#2257=AXIS2_PLACEMENT_3D ( 'NONE', #20316, #616, #24522 ) ;
#2258=ORIENTED_EDGE ( 'NONE', *, *, #635, .T. ) ;
#2259=CARTESIAN_POINT ( 'NONE',  ( -48.71401279728984690, -193.5000000000000000, 0.9720229140804159673 ) ) ;
#2261=ORIENTED_EDGE ( 'NONE', *, *, #14771, .F. ) ;
#2262=CARTESIAN_POINT ( 'NONE',  ( 11.61413489515541997, -183.6283474603465606, -109.6074810615842381 ) ) ;
#2263=CARTESIAN_POINT ( 'NONE',  ( -47.63353074800702558, -193.5000000000000000, -0.5338233779647817423 ) ) ;
#2264=PLANE ( 'NONE',  #5271 ) ;
#2266=EDGE_CURVE ( 'NONE', #39640, #346, #7965, .T. ) ;
#2267=CARTESIAN_POINT ( 'NONE',  ( 38.01517884164422867, -189.7472609257535510, -88.85232316304832523 ) ) ;
#2268=ORIENTED_EDGE ( 'NONE', *, *, #32272, .F. ) ;
#2269=AXIS2_PLACEMENT_3D ( 'NONE', #44005, #40052, #10918 ) ;
#2272=ORIENTED_EDGE ( 'NONE', *, *, #7273, .F. ) ;
#2274=VERTEX_POINT ( 'NONE', #19166 ) ;
#2276=ORIENTED_EDGE ( 'NONE', *, *, #44355, .T. ) ;
#2277=CYLINDRICAL_SURFACE ( 'NONE', #18436, 125.0000000000000000 ) ;
#2279=FACE_OUTER_BOUND ( 'NONE', #45736, .T. ) ;
#2280=VECTOR ( 'NONE', #39192, 1000.000000000000227 ) ;
#2281=LINE ( 'NONE', #22767, #40526 ) ;
#2282=VERTEX_POINT ( 'NONE', #51234 ) ;
#2284=AXIS2_PLACEMENT_3D ( 'NONE', #9800, #38156, #25827 ) ;
#2285=CIRCLE ( 'NONE', #30784, 125.0000000000000000 ) ;
#2287=EDGE_CURVE ( 'NONE', #31475, #39687, #7343, .T. ) ;
#2288=AXIS2_PLACEMENT_3D ( 'NONE', #31879, #16117, #32132 ) ;
#2290=DIRECTION ( 'NONE',  ( 0.000000000000000000, 0.000000000000000000, 1.000000000000000000 ) ) ;
#2292=EDGE_LOOP ( 'NONE', ( #29245, #12023, #38810, #31381 ) ) ;
#2293=ORIENTED_EDGE ( 'NONE', *, *, #29216, .T. ) ;
#2295=DIRECTION ( 'NONE',  ( 0.000000000000000000, 1.000000000000000000, -0.000000000000000000 ) ) ;
#2296=DIRECTION ( 'NONE',  ( 0.000000000000000000, 0.000000000000000000, 1.000000000000000000 ) ) ;
#2298=LINE ( 'NONE', #18060, #28679 ) ;
#2299=DIRECTION ( 'NONE',  ( 0.000000000000000000, -0.000000000000000000, -1.000000000000000000 ) ) ;
#2303=CARTESIAN_POINT ( 'NONE',  ( -213.8817838414232426, -213.5000000000000000, 2.819679052520814125E-14 ) ) ;
#2306=ORIENTED_EDGE ( 'NONE', *, *, #30099, .F. ) ;
#2307=VECTOR ( 'NONE', #39160, 1000.000000000000000 ) ;
#2309=EDGE_CURVE ( 'NONE', #3221, #17784, #23371, .T. ) ;
#2310=VERTEX_POINT ( 'NONE', #38610 ) ;
#2311=PLANE ( 'NONE',  #21612 ) ;
#2312=VERTEX_POINT ( 'NONE', #11002 ) ;
#2314=FACE_OUTER_BOUND ( 'NONE', #26511, .T. ) ;
#2316=VERTEX_POINT ( 'NONE', #31235 ) ;
#2317=DIRECTION ( 'NONE',  ( -0.9473263538541899509, 0.000000000000000000, -0.3202698538628415692 ) ) ;
#2318=EDGE_LOOP ( 'NONE', ( #43891, #46362, #7589, #50847 ) ) ;
#2319=EDGE_CURVE ( 'NONE', #23283, #13008, #37350, .T. ) ;
#2320=EDGE_LOOP ( 'NONE', ( #363, #35446, #1659, #50731 ) ) ;
#2321=CARTESIAN_POINT ( 'NONE',  ( -159.0901268547125653, -177.1207230881787780, 58.22548115875957109 ) ) ;
#2322=VECTOR ( 'NONE', #598, 1000.000000000000000 ) ;
#2323=LINE ( 'NONE', #26474, #22249 ) ;
#2324=VECTOR ( 'NONE', #28642, 1000.000000000000000 ) ;
#2325=CARTESIAN_POINT ( 'NONE',  ( -55.05561436132770581, -193.5000000000000000, 124.8268793598474105 ) ) ;
#2327=EDGE_LOOP ( 'NONE', ( #48897, #47615, #28463, #49873 ) ) ;
#2328=VECTOR ( 'NONE', #22791, 1000.000000000000227 ) ;
#2334=ORIENTED_EDGE ( 'NONE', *, *, #40185, .T. ) ;
#2336=DIRECTION ( 'NONE',  ( -0.9027978299657446470, 0.000000000000000000, 0.4300652022765183435 ) ) ;
#2337=CIRCLE ( 'NONE', #31691, 125.0000000000000000 ) ;
#2338=CARTESIAN_POINT ( 'NONE',  ( -48.47912675150885065, -183.6283474603465606, 6.938893903907228378E-15 ) ) ;
#2340=DIRECTION ( 'NONE',  ( 0.000000000000000000, 0.000000000000000000, 1.000000000000000000 ) ) ;
#2341=CARTESIAN_POINT ( 'NONE',  ( -49.08592689732743963, -193.5000000000000000, -0.7948544414133539293 ) ) ;
#2342=VERTEX_POINT ( 'NONE', #11259 ) ;
#2343=DIRECTION ( 'NONE',  ( -0.000000000000000000, 1.000000000000000000, -0.000000000000000000 ) ) ;
#2344=VERTEX_POINT ( 'NONE', #27292 ) ;
#2345=VECTOR ( 'NONE', #42432, 1000.000000000000000 ) ;
#2348=DIRECTION ( 'NONE',  ( -0.9374196611341254481, 0.000000000000000000, 0.3482016354343867026 ) ) ;
#2350=AXIS2_PLACEMENT_3D ( 'NONE', #11123, #46898, #50569 ) ;
#2356=ORIENTED_EDGE ( 'NONE', *, *, #41519, .F. ) ;
#2358=VECTOR ( 'NONE', #40582, 1000.000000000000000 ) ;
#2359=ORIENTED_EDGE ( 'NONE', *, *, #51003, .T. ) ;
#2360=CARTESIAN_POINT ( 'NONE',  ( -117.6201219941651601, -189.7472609257535510, 104.1370384486469902 ) ) ;
#2363=DIRECTION ( 'NONE',  ( 0.000000000000000000, 0.000000000000000000, -1.000000000000000000 ) ) ;
#2366=DIRECTION ( 'NONE',  ( 0.000000000000000000, 0.000000000000000000, 1.000000000000000000 ) ) ;
#2367=ORIENTED_EDGE ( 'NONE', *, *, #31110, .T. ) ;
#2368=EDGE_CURVE ( 'NONE', #27409, #46293, #27248, .T. ) ;
#2370=DIRECTION ( 'NONE',  ( -0.000000000000000000, 1.000000000000000000, -0.000000000000000000 ) ) ;
#2371=ORIENTED_EDGE ( 'NONE', *, *, #35913, .T. ) ;
#2372=DIRECTION ( 'NONE',  ( 0.000000000000000000, -1.000000000000000000, 0.000000000000000000 ) ) ;
#2374=LINE ( 'NONE', #50719, #16669 ) ;
#2376=CARTESIAN_POINT ( 'NONE',  ( -47.74129347246712740, -193.5000000000000000, -0.6749830015182022303 ) ) ;
#2377=EDGE_LOOP ( 'NONE', ( #25299, #3325, #5231, #11655 ) ) ;
#2378=VERTEX_POINT ( 'NONE', #24649 ) ;
#2381=ORIENTED_EDGE ( 'NONE', *, *, #926, .F. ) ;
#2383=VECTOR ( 'NONE', #39835, 1000.000000000000114 ) ;
#2384=LINE ( 'NONE', #10505, #39086 ) ;
#2385=ORIENTED_EDGE ( 'NONE', *, *, #50042, .F. ) ;
#2388=FACE_OUTER_BOUND ( 'NONE', #37197, .T. ) ;
#2389=DIRECTION ( 'NONE',  ( 0.000000000000000000, 0.000000000000000000, 1.000000000000000000 ) ) ;
#2390=VECTOR ( 'NONE', #35749, 1000.000000000000114 ) ;
#2391=DIRECTION ( 'NONE',  ( 0.05924062789370006937, 0.000000000000000000, 0.9982437317643222396 ) ) ;
#2392=ORIENTED_EDGE ( 'NONE', *, *, #3355, .T. ) ;
#2393=CARTESIAN_POINT ( 'NONE',  ( -47.97059563285962724, -193.5000000000000000, -0.8610436117673480050 ) ) ;
#2394=FACE_OUTER_BOUND ( 'NONE', #9117, .T. ) ;
#2395=FACE_OUTER_BOUND ( 'NONE', #31810, .T. ) ;
#2396=ORIENTED_EDGE ( 'NONE', *, *, #26685, .F. ) ;
#2398=DIRECTION ( 'NONE',  ( 0.000000000000000000, -0.000000000000000000, -1.000000000000000000 ) ) ;
#2402=CARTESIAN_POINT ( 'NONE',  ( -48.07600332222087758, -193.5000000000000000, -0.9151456172430111335 ) ) ;
#2403=ORIENTED_EDGE ( 'NONE', *, *, #46389, .F. ) ;
#2404=DIRECTION ( 'NONE',  ( 0.000000000000000000, -1.000000000000000000, 0.000000000000000000 ) ) ;
#2405=VECTOR ( 'NONE', #32806, 1000.000000000000000 ) ;
#2407=CARTESIAN_POINT ( 'NONE',  ( 75.27070168362158142, -189.7472609257535510, 17.63462396184792524 ) ) ;
#2409=CARTESIAN_POINT ( 'NONE',  ( -164.0008810331606526, -175.3837268820161057, 47.74645837849825369 ) ) ;
#2410=EDGE_LOOP ( 'NONE', ( #3687, #37134, #46087, #48529 ) ) ;
#2414=DIRECTION ( 'NONE',  ( -0.000000000000000000, 1.000000000000000000, -0.000000000000000000 ) ) ;
#2418=EDGE_CURVE ( 'NONE', #24544, #32491, #3911, .T. ) ;
#2420=VERTEX_POINT ( 'NONE', #36213 ) ;
#2421=CARTESIAN_POINT ( 'NONE',  ( -158.0280232639029236, -193.5000000000000000, 60.19999396110247147 ) ) ;
#2422=VECTOR ( 'NONE', #45411, 1000.000000000000000 ) ;
#2424=PLANE ( 'NONE',  #5374 ) ;
#2428=VECTOR ( 'NONE', #37249, 1000.000000000000114 ) ;
#2429=CARTESIAN_POINT ( 'NONE',  ( -48.47912675150885065, -189.7472609257535510, 6.938893903907228378E-15 ) ) ;
#2430=CARTESIAN_POINT ( 'NONE',  ( -150.5215542367829755, -189.7472609257535510, -72.19655804061973470 ) ) ;
#2431=VERTEX_POINT ( 'NONE', #52017 ) ;
#2432=EDGE_CURVE ( 'NONE', #13215, #8540, #31769, .T. ) ;
#2433=DIRECTION ( 'NONE',  ( 0.9960498426152165630, 0.000000000000000000, 0.08879589532293852283 ) ) ;
#2436=ORIENTED_EDGE ( 'NONE', *, *, #40280, .T. ) ;
#2437=DIRECTION ( 'NONE',  ( 0.000000000000000000, -1.000000000000000000, -0.000000000000000000 ) ) ;
#2439=DIRECTION ( 'NONE',  ( 0.000000000000000000, -1.000000000000000000, -0.000000000000000000 ) ) ;
#2441=ORIENTED_EDGE ( 'NONE', *, *, #7273, .T. ) ;
#2442=CARTESIAN_POINT ( 'NONE',  ( -162.7543581613524282, -193.5000000000000000, 50.65739320402010293 ) ) ;
#2443=LINE ( 'NONE', #10574, #12410 ) ;
#2445=CARTESIAN_POINT ( 'NONE',  ( -112.1919339979530150, -189.7472609257535510, 107.5438431188761825 ) ) ;
#2446=DIRECTION ( 'NONE',  ( 0.3482016354344059095, 0.000000000000000000, -0.9374196611341183427 ) ) ;
#2449=CARTESIAN_POINT ( 'NONE',  ( 32.59960422616970988, -193.5000000000000000, -93.82025162277999186 ) ) ;
#2450=ORIENTED_EDGE ( 'NONE', *, *, #21802, .T. ) ;
#2451=DIRECTION ( 'NONE',  ( -0.000000000000000000, -1.000000000000000000, 0.000000000000000000 ) ) ;
#2454=CARTESIAN_POINT ( 'NONE',  ( -168.1141659785444915, -183.6283474603465606, -36.22785377503947046 ) ) ;
#2456=ORIENTED_EDGE ( 'NONE', *, *, #39642, .F. ) ;
#2459=ADVANCED_FACE ( 'NONE', ( #32011 ), #39883, .T. ) ;
#2460=CARTESIAN_POINT ( 'NONE',  ( -66.64622755927952369, -183.6283474603465606, 123.6727797384707372 ) ) ;
#2462=EDGE_CURVE ( 'NONE', #3624, #9307, #32539, .T. ) ;
#2463=ORIENTED_EDGE ( 'NONE', *, *, #47204, .F. ) ;
#2464=CARTESIAN_POINT ( 'NONE',  ( -124.9871112439422092, -189.7472609257535510, -98.85104101073275729 ) ) ;
#2465=ORIENTED_EDGE ( 'NONE', *, *, #39109, .F. ) ;
#2466=DIRECTION ( 'NONE',  ( 0.3482016354343995812, 0.000000000000000000, -0.9374196611341205632 ) ) ;
#2467=DIRECTION ( 'NONE',  ( -0.000000000000000000, 1.000000000000000000, -0.000000000000000000 ) ) ;
#2471=DIRECTION ( 'NONE',  ( -0.8757349421956310831, 0.000000000000000000, -0.4827922027307550712 ) ) ;
#2472=ADVANCED_FACE ( 'NONE', ( #44104 ), #40404, .T. ) ;
#2474=CIRCLE ( 'NONE', #15910, 125.0000000000000000 ) ;
#2476=ORIENTED_EDGE ( 'NONE', *, *, #18009, .F. ) ;
#2478=LINE ( 'NONE', #3492, #22267 ) ;
#2479=ORIENTED_EDGE ( 'NONE', *, *, #18877, .F. ) ;
#2480=CARTESIAN_POINT ( 'NONE',  ( -105.4063847101409692, -193.5000000000000000, -111.2847127925096231 ) ) ;
#2481=LINE ( 'NONE', #51111, #38427 ) ;
#2482=ADVANCED_FACE ( 'NONE', ( #12815 ), #27803, .T. ) ;
#2483=CARTESIAN_POINT ( 'NONE',  ( -48.47912675150885065, -175.3837268820161057, 6.938893903907228378E-15 ) ) ;
#2485=VERTEX_POINT ( 'NONE', #24920 ) ;
#2486=ORIENTED_EDGE ( 'NONE', *, *, #26176, .T. ) ;
#2487=ORIENTED_EDGE ( 'NONE', *, *, #30184, .F. ) ;
#2488=FACE_OUTER_BOUND ( 'NONE', #4253, .T. ) ;
#2489=CARTESIAN_POINT ( 'NONE',  ( -140.8230258362169707, -193.5000000000000000, 84.24728067916045404 ) ) ;
#2490=AXIS2_PLACEMENT_3D ( 'NONE', #7512, #26951, #23532 ) ;
#2492=CARTESIAN_POINT ( 'NONE',  ( -48.47912675150885065, -183.6283474603465606, 6.938893903907228378E-15 ) ) ;
#2493=ORIENTED_EDGE ( 'NONE', *, *, #18568, .T. ) ;
#2499=DIRECTION ( 'NONE',  ( 0.000000000000000000, 0.000000000000000000, 1.000000000000000000 ) ) ;
#2501=PLANE ( 'NONE',  #37696 ) ;
#2502=EDGE_LOOP ( 'NONE', ( #48239, #12553, #26115, #45439 ) ) ;
#2505=EDGE_CURVE ( 'NONE', #14785, #35111, #40937, .T. ) ;
#2506=APPLICATION_CONTEXT ( 'automotive_design' ) ;
#2508=LINE ( 'NONE', #42958, #48072 ) ;
#2509=CARTESIAN_POINT ( 'NONE',  ( 41.41233698655026529, -177.1207230881787780, 86.85922373029363541 ) ) ;
#2510=ORIENTED_EDGE ( 'NONE', *, *, #44355, .F. ) ;
#2511=EDGE_CURVE ( 'NONE', #29270, #18052, #20980, .T. ) ;
#2512=DIRECTION ( 'NONE',  ( -0.000000000000000000, 1.000000000000000000, -0.000000000000000000 ) ) ;
#2513=ADVANCED_FACE ( 'NONE', ( #22007 ), #1771, .T. ) ;
#2515=DIRECTION ( 'NONE',  ( 0.000000000000000000, -0.000000000000000000, -1.000000000000000000 ) ) ;
#2516=EDGE_CURVE ( 'NONE', #23682, #37758, #30616, .T. ) ;
#2520=EDGE_LOOP ( 'NONE', ( #49314, #26680, #12572, #49787 ) ) ;
#2521=AXIS2_PLACEMENT_3D ( 'NONE', #48638, #40455, #32587 ) ;
#2522=EDGE_CURVE ( 'NONE', #28521, #34600, #21239, .T. ) ;
#2523=CARTESIAN_POINT ( 'NONE',  ( 76.47090317495664635, -175.3837268820161057, -3.534122433557446374 ) ) ;
#2524=ORIENTED_EDGE ( 'NONE', *, *, #17558, .T. ) ;
#2526=DIRECTION ( 'NONE',  ( 0.000000000000000000, 1.000000000000000000, -0.000000000000000000 ) ) ;
#2528=ORIENTED_EDGE ( 'NONE', *, *, #33555, .F. ) ;
#2529=ADVANCED_FACE ( 'NONE', ( #45172 ), #5742, .F. ) ;
#2532=EDGE_CURVE ( 'NONE', #25859, #10098, #455, .T. ) ;
#2533=CARTESIAN_POINT ( 'NONE',  ( -49.38192458147459263, -193.5000000000000000, -0.4300652022765235616 ) ) ;
#2535=ORIENTED_EDGE ( 'NONE', *, *, #8208, .F. ) ;
#2536=DIRECTION ( 'NONE',  ( 0.000000000000000000, -1.000000000000000000, 0.000000000000000000 ) ) ;
#2538=LINE ( 'NONE', #43246, #5122 ) ;
#2540=ORIENTED_EDGE ( 'NONE', *, *, #21536, .F. ) ;
#2541=EDGE_LOOP ( 'NONE', ( #42345, #44908, #36123, #29624 ) ) ;
#2542=EDGE_CURVE ( 'NONE', #39427, #44067, #45945, .T. ) ;
#2544=AXIS2_PLACEMENT_3D ( 'NONE', #5844, #10530, #13704 ) ;
#2545=VERTEX_POINT ( 'NONE', #29107 ) ;
#2546=EDGE_CURVE ( 'NONE', #46197, #47219, #50829, .T. ) ;
#2547=DIRECTION ( 'NONE',  ( -0.000000000000000000, 1.000000000000000000, -0.000000000000000000 ) ) ;
#2548=DIRECTION ( 'NONE',  ( 0.8124868780056825335, 0.000000000000000000, -0.5829794791144703447 ) ) ;
#2550=DIRECTION ( 'NONE',  ( 0.000000000000000000, 0.000000000000000000, 1.000000000000000000 ) ) ;
#2551=CARTESIAN_POINT ( 'NONE',  ( -173.0003472773501301, -193.5000000000000000, 10.93003379476953363 ) ) ;
#2552=VERTEX_POINT ( 'NONE', #37773 ) ;
#2553=EDGE_CURVE ( 'NONE', #37393, #9572, #24779, .T. ) ;
#2554=DIRECTION ( 'NONE',  ( 0.000000000000000000, 0.000000000000000000, 1.000000000000000000 ) ) ;
#2555=ORIENTED_EDGE ( 'NONE', *, *, #23636, .T. ) ;
#2557=ORIENTED_EDGE ( 'NONE', *, *, #32057, .F. ) ;
#2558=ORIENTED_EDGE ( 'NONE', *, *, #42644, .F. ) ;
#2559=AXIS2_PLACEMENT_3D ( 'NONE', #25166, #40920, #28315 ) ;
#2560=DIRECTION ( 'NONE',  ( -0.000000000000000000, 1.000000000000000000, -0.000000000000000000 ) ) ;
#2561=ORIENTED_EDGE ( 'NONE', *, *, #40726, .F. ) ;
#2564=FACE_OUTER_BOUND ( 'NONE', #15807, .T. ) ;
#2565=ORIENTED_EDGE ( 'NONE', *, *, #37242, .T. ) ;
#2566=DIRECTION ( 'NONE',  ( 0.000000000000000000, -1.000000000000000000, -0.000000000000000000 ) ) ;
#2567=ORIENTED_EDGE ( 'NONE', *, *, #23366, .F. ) ;
#2568=ORIENTED_EDGE ( 'NONE', *, *, #36896, .T. ) ;
#2569=CARTESIAN_POINT ( 'NONE',  ( 45.24245851652180761, -177.1207230881787780, -81.19354792697733103 ) ) ;
#2570=CARTESIAN_POINT ( 'NONE',  ( -173.3968853974275817, -189.7472609257535510, 4.533605064404172325 ) ) ;
#2571=FACE_OUTER_BOUND ( 'NONE', #38785, .T. ) ;
#2572=ORIENTED_EDGE ( 'NONE', *, *, #5502, .T. ) ;
#2575=EDGE_CURVE ( 'NONE', #11294, #18907, #49367, .T. ) ;
#2580=LINE ( 'NONE', #26748, #34707 ) ;
#2581=FACE_OUTER_BOUND ( 'NONE', #41266, .T. ) ;
#2583=EDGE_CURVE ( 'NONE', #35261, #563, #6240, .T. ) ;
#2584=AXIS2_PLACEMENT_3D ( 'NONE', #9700, #14426, #14179 ) ;
#2587=ORIENTED_EDGE ( 'NONE', *, *, #23706, .F. ) ;
#2590=ORIENTED_EDGE ( 'NONE', *, *, #36258, .T. ) ;
#2591=DIRECTION ( 'NONE',  ( 0.7378332790417189146, 0.000000000000000000, 0.6749830015182196608 ) ) ;
#2592=VERTEX_POINT ( 'NONE', #46198 ) ;
#2593=DIRECTION ( 'NONE',  ( -0.000000000000000000, 1.000000000000000000, -0.000000000000000000 ) ) ;
#2595=EDGE_CURVE ( 'NONE', #32858, #10769, #10175, .T. ) ;
#2596=CARTESIAN_POINT ( 'NONE',  ( -48.98765787015808115, -177.1207230881787780, 0.8610436117673582190 ) ) ;
#2598=CARTESIAN_POINT ( 'NONE',  ( 76.52053249983504202, -177.1207230881787780, -0.2918682030015415929 ) ) ;
#2600=EDGE_LOOP ( 'NONE', ( #29938, #35646, #9190, #20573 ) ) ;
#2605=ORIENTED_EDGE ( 'NONE', *, *, #15077, .T. ) ;
#2606=LINE ( 'NONE', #2360, #6627 ) ;
#2607=CIRCLE ( 'NONE', #31972, 125.0000000000000000 ) ;
#2608=VECTOR ( 'NONE', #8345, 1000.000000000000000 ) ;
#2609=LINE ( 'NONE', #18393, #50257 ) ;
#2610=LINE ( 'NONE', #46507, #25614 ) ;
#2611=ORIENTED_EDGE ( 'NONE', *, *, #31301, .T. ) ;
#2612=CARTESIAN_POINT ( 'NONE',  ( -1.230335819511603423, -177.1207230881787780, 115.7261930397108216 ) ) ;
#2613=DIRECTION ( 'NONE',  ( 0.000000000000000000, -1.000000000000000000, 0.000000000000000000 ) ) ;
#2616=ORIENTED_EDGE ( 'NONE', *, *, #33444, .F. ) ;
#2617=DIRECTION ( 'NONE',  ( 0.000000000000000000, 0.000000000000000000, 1.000000000000000000 ) ) ;
#2618=ORIENTED_EDGE ( 'NONE', *, *, #38250, .F. ) ;
#2619=CYLINDRICAL_SURFACE ( 'NONE', #46048, 125.0000000000000000 ) ;
#2620=DIRECTION ( 'NONE',  ( 0.000000000000000000, 1.000000000000000000, 0.000000000000000000 ) ) ;
#2621=DIRECTION ( 'NONE',  ( -0.000000000000000000, 1.000000000000000000, -0.000000000000000000 ) ) ;
#2623=ORIENTED_EDGE ( 'NONE', *, *, #43907, .T. ) ;
#2624=CARTESIAN_POINT ( 'NONE',  ( -165.7578939544008847, -177.1207230881787780, -43.25148278810627289 ) ) ;
#2625=ORIENTED_EDGE ( 'NONE', *, *, #34946, .T. ) ;
#2626=CYLINDRICAL_SURFACE ( 'NONE', #30391, 125.0000000000000000 ) ;
#2627=CARTESIAN_POINT ( 'NONE',  ( -48.47912675150885065, -183.6283474603465606, 6.938893903907228378E-15 ) ) ;
#2628=CIRCLE ( 'NONE', #24452, 125.0000000000000000 ) ;
#2630=CARTESIAN_POINT ( 'NONE',  ( -48.82732838694323618, -193.5000000000000000, -0.9374196611341184537 ) ) ;
#2631=CARTESIAN_POINT ( 'NONE',  ( -48.47912675150885065, -175.3837268820161057, 6.938893903907228378E-15 ) ) ;
#2632=CARTESIAN_POINT ( 'NONE',  ( -173.2765435274470178, -177.1207230881787780, -7.113702696401505321 ) ) ;
#2634=DIRECTION ( 'NONE',  ( 0.9995608365087940150, 0.000000000000000000, 0.02963332782257007206 ) ) ;
#2636=ADVANCED_FACE ( 'NONE', ( #42492 ), #26724, .T. ) ;
#2637=FACE_OUTER_BOUND ( 'NONE', #47312, .T. ) ;
#2638=DIRECTION ( 'NONE',  ( 0.000000000000000000, 1.000000000000000000, -0.000000000000000000 ) ) ;
#2640=EDGE_LOOP ( 'NONE', ( #1975, #28396, #14696, #2611 ) ) ;
#2641=FACE_OUTER_BOUND ( 'NONE', #17449, .T. ) ;
#2642=CARTESIAN_POINT ( 'NONE',  ( -142.6204786402482512, -193.5000000000000000, -80.70646587903381430 ) ) ;
#2643=AXIS2_PLACEMENT_3D ( 'NONE', #9378, #17008, #13042 ) ;
#2644=FACE_OUTER_BOUND ( 'NONE', #5378, .T. ) ;
#2645=DIRECTION ( 'NONE',  ( -0.000000000000000000, 1.000000000000000000, -0.000000000000000000 ) ) ;
#2646=VERTEX_POINT ( 'NONE', #50648 ) ;
#2647=AXIS2_PLACEMENT_3D ( 'NONE', #50867, #22499, #38513 ) ;
#2649=DIRECTION ( 'NONE',  ( 0.000000000000000000, 0.000000000000000000, 1.000000000000000000 ) ) ;
#2650=EDGE_CURVE ( 'NONE', #23558, #3648, #13912, .T. ) ;
#2651=DIRECTION ( 'NONE',  ( 0.000000000000000000, -0.000000000000000000, -1.000000000000000000 ) ) ;
#2652=PLANE ( 'NONE',  #17006 ) ;
#2653=VERTEX_POINT ( 'NONE', #50394 ) ;
#2654=DIRECTION ( 'NONE',  ( -0.9473263538541946138, 0.000000000000000000, 0.3202698538628279690 ) ) ;
#2655=VECTOR ( 'NONE', #16564, 1000.000000000000000 ) ;
#2656=EDGE_CURVE ( 'NONE', #14204, #8140, #22541, .T. ) ;
#2658=ORIENTED_EDGE ( 'NONE', *, *, #8920, .T. ) ;
#2659=VERTEX_POINT ( 'NONE', #47233 ) ;
#2660=AXIS2_PLACEMENT_3D ( 'NONE', #15162, #50910, #22781 ) ;
#2661=EDGE_LOOP ( 'NONE', ( #31636, #28193, #50067, #25252 ) ) ;
#2663=EDGE_CURVE ( 'NONE', #45569, #15488, #18072, .T. ) ;
#2664=PLANE ( 'NONE',  #31209 ) ;
#2665=DIRECTION ( 'NONE',  ( -0.7948544414133523750, 0.000000000000000000, -0.6068001458185945385 ) ) ;
#2666=ORIENTED_EDGE ( 'NONE', *, *, #21957, .F. ) ;
#2667=CARTESIAN_POINT ( 'NONE',  ( -48.47912675150885065, -177.1207230881787780, 6.938893903907228378E-15 ) ) ;
#2668=DIRECTION ( 'NONE',  ( 0.000000000000000000, 0.000000000000000000, 1.000000000000000000 ) ) ;
#2669=CARTESIAN_POINT ( 'NONE',  ( -109.9568094315246327, -193.5000000000000000, -108.8370090194290611 ) ) ;
#2671=ORIENTED_EDGE ( 'NONE', *, *, #13934, .T. ) ;
#2673=ORIENTED_EDGE ( 'NONE', *, *, #29493, .F. ) ;
#2674=DIRECTION ( 'NONE',  ( 0.9995608365087944591, 0.000000000000000000, -0.02963332782255633305 ) ) ;
#2677=CARTESIAN_POINT ( 'NONE',  ( -48.47912675150885065, -177.1207230881787780, 6.938893903907228378E-15 ) ) ;
#2679=CIRCLE ( 'NONE', #162, 125.0000000000000000 ) ;
#2680=FACE_OUTER_BOUND ( 'NONE', #16960, .T. ) ;
#2681=ORIENTED_EDGE ( 'NONE', *, *, #31985, .T. ) ;
#2683=EDGE_CURVE ( 'NONE', #25185, #3968, #40708, .T. ) ;
#2684=ORIENTED_EDGE ( 'NONE', *, *, #21170, .F. ) ;
#2686=DIRECTION ( 'NONE',  ( 0.1768902751225733261, 0.000000000000000000, -0.9842305779475966077 ) ) ;
#2687=ORIENTED_EDGE ( 'NONE', *, *, #25384, .F. ) ;
#2691=ADVANCED_FACE ( 'NONE', ( #46448 ), #14644, .F. ) ;
#2694=CARTESIAN_POINT ( 'NONE',  ( 56.46549106873199975, -193.5000000000000000, -66.05018866041275771 ) ) ;
#2695=ORIENTED_EDGE ( 'NONE', *, *, #19894, .T. ) ;
#2696=DIRECTION ( 'NONE',  ( -0.7765238627180482966, 0.000000000000000000, 0.6300878435817038881 ) ) ;
#2697=ORIENTED_EDGE ( 'NONE', *, *, #48030, .T. ) ;
#2698=VECTOR ( 'NONE', #20468, 1000.000000000000227 ) ;
#2700=VECTOR ( 'NONE', #15612, 999.9999999999998863 ) ;
#2701=FACE_OUTER_BOUND ( 'NONE', #12692, .T. ) ;
#2704=CARTESIAN_POINT ( 'NONE',  ( 72.31641062551800303, -175.3837268820161057, 32.14713283941990341 ) ) ;
#2705=EDGE_CURVE ( 'NONE', #38799, #6533, #30656, .T. ) ;
#2707=FACE_OUTER_BOUND ( 'NONE', #37893, .T. ) ;
#2708=VERTEX_POINT ( 'NONE', #11205 ) ;
#2709=DIRECTION ( 'NONE',  ( 0.000000000000000000, 0.000000000000000000, 1.000000000000000000 ) ) ;
#2710=DIRECTION ( 'NONE',  ( -0.000000000000000000, 1.000000000000000000, -0.000000000000000000 ) ) ;
#2711=ADVANCED_FACE ( 'NONE', ( #6766 ), #50917, .F. ) ;
#2712=DIRECTION ( 'NONE',  ( -0.000000000000000000, -1.000000000000000000, 0.000000000000000000 ) ) ;
#2713=CARTESIAN_POINT ( 'NONE',  ( -47.51449116960048968, -175.3837268820161057, -0.2635871660690578544 ) ) ;
#2716=ORIENTED_EDGE ( 'NONE', *, *, #33376, .T. ) ;
#2718=VECTOR ( 'NONE', #45275, 1000.000000000000114 ) ;
#2720=ORIENTED_EDGE ( 'NONE', *, *, #17747, .T. ) ;
#2721=DIRECTION ( 'NONE',  ( -0.000000000000000000, 1.000000000000000000, -0.000000000000000000 ) ) ;
#2723=DIRECTION ( 'NONE',  ( 0.000000000000000000, 0.000000000000000000, -1.000000000000000000 ) ) ;
#2724=DIRECTION ( 'NONE',  ( -0.000000000000000000, 1.000000000000000000, -0.000000000000000000 ) ) ;
#2725=CARTESIAN_POINT ( 'NONE',  ( -12.42681898335384894, -175.3837268820161057, 118.6432945265039365 ) ) ;
#2729=ORIENTED_EDGE ( 'NONE', *, *, #49819, .F. ) ;
#2731=EDGE_LOOP ( 'NONE', ( #36758, #38492, #14858, #19836 ) ) ;
#2732=PLANE ( 'NONE',  #45962 ) ;
#2733=DIRECTION ( 'NONE',  ( 0.5586467658036476935, 0.000000000000000000, 0.8294056854502049880 ) ) ;
#2734=VECTOR ( 'NONE', #46732, 999.9999999999998863 ) ;
#2736=LINE ( 'NONE', #3508, #15313 ) ;
#2738=ORIENTED_EDGE ( 'NONE', *, *, #39768, .T. ) ;
#2739=EDGE_CURVE ( 'NONE', #38573, #25631, #20615, .T. ) ;
#2741=EDGE_CURVE ( 'NONE', #44939, #32649, #46975, .T. ) ;
#2742=DIRECTION ( 'NONE',  ( -0.000000000000000000, 1.000000000000000000, -0.000000000000000000 ) ) ;
#2744=ORIENTED_EDGE ( 'NONE', *, *, #51706, .T. ) ;
#2745=ORIENTED_EDGE ( 'NONE', *, *, #39538, .T. ) ;
#2748=PLANE ( 'NONE',  #38418 ) ;
#2750=AXIS2_PLACEMENT_3D ( 'NONE', #2259, #50351, #46404 ) ;
#2751=CARTESIAN_POINT ( 'NONE',  ( -149.9407190013152160, -175.3837268820161057, -73.01058346660458653 ) ) ;
#2752=CARTESIAN_POINT ( 'NONE',  ( -72.96029774493612763, -183.6283474603465606, 122.5792489240759551 ) ) ;
#2753=ORIENTED_EDGE ( 'NONE', *, *, #51082, .T. ) ;
#2754=EDGE_CURVE ( 'NONE', #11828, #31627, #7016, .T. ) ;
#2755=DIRECTION ( 'NONE',  ( 0.1476465640024851034, 0.000000000000000000, -0.9890401873221634776 ) ) ;
#2756=EDGE_CURVE ( 'NONE', #23765, #23329, #39055, .T. ) ;
#2758=VERTEX_POINT ( 'NONE', #39328 ) ;
#2759=DIRECTION ( 'NONE',  ( -0.000000000000000000, 1.000000000000000000, -0.000000000000000000 ) ) ;
#2762=EDGE_LOOP ( 'NONE', ( #32489, #11370, #14078, #37120 ) ) ;
#2763=FACE_OUTER_BOUND ( 'NONE', #10866, .T. ) ;
#2764=FACE_OUTER_BOUND ( 'NONE', #6925, .T. ) ;
#2765=DIRECTION ( 'NONE',  ( 0.000000000000000000, 0.000000000000000000, 1.000000000000000000 ) ) ;
#2766=VECTOR ( 'NONE', #31801, 1000.000000000000000 ) ;
#2768=AXIS2_PLACEMENT_3D ( 'NONE', #11508, #44083, #43820 ) ;
#2769=DIRECTION ( 'NONE',  ( 0.000000000000000000, 0.000000000000000000, 1.000000000000000000 ) ) ;
#2772=CARTESIAN_POINT ( 'NONE',  ( -48.30223647638628393, -177.1207230881787780, 0.9842305779476049343 ) ) ;
#2773=LINE ( 'NONE', #19839, #47981 ) ;
#2775=ORIENTED_EDGE ( 'NONE', *, *, #16233, .F. ) ;
#2776=LINE ( 'NONE', #39301, #47285 ) ;
#2777=CIRCLE ( 'NONE', #49803, 125.0000000000000000 ) ;
#2778=ORIENTED_EDGE ( 'NONE', *, *, #22631, .F. ) ;
#2780=EDGE_LOOP ( 'NONE', ( #20754, #6754, #3639, #10849 ) ) ;
#2783=ORIENTED_EDGE ( 'NONE', *, *, #39292, .F. ) ;
#2789=ORIENTED_EDGE ( 'NONE', *, *, #28552, .T. ) ;
#2790=CIRCLE ( 'NONE', #9518, 125.0000000000000000 ) ;
#2794=CARTESIAN_POINT ( 'NONE',  ( -30.31202594373736403, -183.6283474603465606, -123.6727797384705951 ) ) ;
#2795=DIRECTION ( 'NONE',  ( 0.000000000000000000, -0.000000000000000000, 1.000000000000000000 ) ) ;
#2796=CARTESIAN_POINT ( 'NONE',  ( -53.47502265695599277, -183.6283474603465606, -123.9001241957025883 ) ) ;
#2797=ORIENTED_EDGE ( 'NONE', *, *, #15728, .F. ) ;
#2798=EDGE_CURVE ( 'NONE', #22576, #12684, #35686, .T. ) ;
#2800=EDGE_CURVE ( 'NONE', #875, #23517, #12747, .T. ) ;
#2802=EDGE_CURVE ( 'NONE', #50437, #895, #27749, .T. ) ;
#2803=CARTESIAN_POINT ( 'NONE',  ( 36.19006208304271155, -183.6283474603465606, 90.59430563621340582 ) ) ;
#2804=VERTEX_POINT ( 'NONE', #31955 ) ;
#2805=DIRECTION ( 'NONE',  ( 0.9564009842765244240, 0.000000000000000000, -0.2920567706369695538 ) ) ;
#2808=ORIENTED_EDGE ( 'NONE', *, *, #15183, .F. ) ;
#2809=ADVANCED_FACE ( 'NONE', ( #23556 ), #12237, .T. ) ;
#2810=CARTESIAN_POINT ( 'NONE',  ( -48.82732838694325750, -175.3837268820161057, 0.9374196611341252261 ) ) ;
#2812=DIRECTION ( 'NONE',  ( -0.000000000000000000, 1.000000000000000000, 0.000000000000000000 ) ) ;
#2814=DIRECTION ( 'NONE',  ( 0.000000000000000000, -0.000000000000000000, 1.000000000000000000 ) ) ;
#2815=EDGE_LOOP ( 'NONE', ( #38971, #23611, #27214, #47047 ) ) ;
#2816=EDGE_CURVE ( 'NONE', #20677, #44868, #51959, .T. ) ;
#2818=ORIENTED_EDGE ( 'NONE', *, *, #42612, .T. ) ;
#2819=EDGE_CURVE ( 'NONE', #31354, #6533, #39569, .T. ) ;
#2821=CARTESIAN_POINT ( 'NONE',  ( 69.66827051661184100, -189.7472609257535510, -40.81902153125259503 ) ) ;
#2822=CARTESIAN_POINT ( 'NONE',  ( -118.4510020108455137, -193.5000000000000000, 103.5805805771131674 ) ) ;
#2824=CARTESIAN_POINT ( 'NONE',  ( -49.47868758801764955, -183.6283474603465606, -0.02963332782256313663 ) ) ;
#2825=DIRECTION ( 'NONE',  ( 0.000000000000000000, 1.000000000000000000, 0.000000000000000000 ) ) ;
#2826=ORIENTED_EDGE ( 'NONE', *, *, #19915, .F. ) ;
#2827=DIRECTION ( 'NONE',  ( -0.05924062789370006937, 0.000000000000000000, -0.9982437317643222396 ) ) ;
#2828=VECTOR ( 'NONE', #40963, 1000.000000000000114 ) ;
#2829=DIRECTION ( 'NONE',  ( -0.000000000000000000, 1.000000000000000000, 0.000000000000000000 ) ) ;
#2830=ADVANCED_FACE ( 'NONE', ( #19614 ), #28007, .F. ) ;
#2833=VERTEX_POINT ( 'NONE', #8047 ) ;
#2834=DIRECTION ( 'NONE',  ( -0.000000000000000000, 1.000000000000000000, -0.000000000000000000 ) ) ;
#2835=DIRECTION ( 'NONE',  ( 0.000000000000000000, 0.000000000000000000, 1.000000000000000000 ) ) ;
#2837=DIRECTION ( 'NONE',  ( -0.9564009842765264224, 0.000000000000000000, 0.2920567706369628924 ) ) ;
#2838=EDGE_LOOP ( 'NONE', ( #36866, #51259, #46977, #20278 ) ) ;
#2839=DIRECTION ( 'NONE',  ( 0.000000000000000000, 0.000000000000000000, 1.000000000000000000 ) ) ;
#2840=LINE ( 'NONE', #50952, #5182 ) ;
#2842=LINE ( 'NONE', #43569, #1924 ) ;
#2843=VECTOR ( 'NONE', #42616, 1000.000000000000000 ) ;
#2844=ORIENTED_EDGE ( 'NONE', *, *, #27890, .T. ) ;
#2845=ADVANCED_FACE ( 'NONE', ( #24588 ), #51689, .T. ) ;
#2846=DIRECTION ( 'NONE',  ( 0.9374196611341183427, 0.000000000000000000, 0.3482016354344059095 ) ) ;
#2847=FACE_BOUND ( 'NONE', #3385, .T. ) ;
#2850=VERTEX_POINT ( 'NONE', #35905 ) ;
#2851=ORIENTED_EDGE ( 'NONE', *, *, #33148, .F. ) ;
#2852=ADVANCED_FACE ( 'NONE', ( #15948 ), #36157, .T. ) ;
#2854=ORIENTED_EDGE ( 'NONE', *, *, #33907, .F. ) ;
#2855=CARTESIAN_POINT ( 'NONE',  ( -47.53180039765465636, -193.5000000000000000, -0.3202698538628280800 ) ) ;
#2857=CIRCLE ( 'NONE', #35600, 125.0000000000000000 ) ;
#2861=AXIS2_PLACEMENT_3D ( 'NONE', #30360, #6475, #34315 ) ;
#2862=ADVANCED_FACE ( 'NONE', ( #48779 ), #8312, .T. ) ;
#2864=CARTESIAN_POINT ( 'NONE',  ( 62.59443091842027940, -183.6283474603465606, -57.33816169485142211 ) ) ;
#2865=ORIENTED_EDGE ( 'NONE', *, *, #40463, .T. ) ;
#2866=CARTESIAN_POINT ( 'NONE',  ( -47.97059563285963435, -183.6283474603465606, 0.8610436117673654355 ) ) ;
#2868=VERTEX_POINT ( 'NONE', #684 ) ;
#2869=CARTESIAN_POINT ( 'NONE',  ( 9.518239912201957864, -213.5000000000000000, -110.7307791902283043 ) ) ;
#2870=VERTEX_POINT ( 'NONE', #12507 ) ;
#2871=DIRECTION ( 'NONE',  ( -0.4566292373937018145, 0.000000000000000000, -0.8896570909947529859 ) ) ;
#2872=ORIENTED_EDGE ( 'NONE', *, *, #6919, .F. ) ;
#2873=DIRECTION ( 'NONE',  ( 0.000000000000000000, 0.000000000000000000, 1.000000000000000000 ) ) ;
#2874=ORIENTED_EDGE ( 'NONE', *, *, #6026, .T. ) ;
#2875=EDGE_CURVE ( 'NONE', #25045, #32314, #22264, .T. ) ;
#2878=ORIENTED_EDGE ( 'NONE', *, *, #23932, .T. ) ;
#2882=EDGE_LOOP ( 'NONE', ( #45557, #45621, #1268, #44318 ) ) ;
#2883=CARTESIAN_POINT ( 'NONE',  ( -47.78257572244585560, -193.5000000000000000, -0.7175072570443230546 ) ) ;
#2886=EDGE_LOOP ( 'NONE', ( #13, #47836, #40281, #29504 ) ) ;
#2887=CYLINDRICAL_SURFACE ( 'NONE', #23860, 125.0000000000000000 ) ;
#2889=CARTESIAN_POINT ( 'NONE',  ( -165.6791976657750354, -193.5000000000000000, 40.49875167739066484 ) ) ;
#2890=SHAPE_REPRESENTATION ( 'Angle Mounting Base', ( #31742 ), #46023 ) ;
#2892=EDGE_CURVE ( 'NONE', #30709, #13937, #25888, .T. ) ;
#2893=EDGE_LOOP ( 'NONE', ( #13406, #34994, #35244, #25037 ) ) ;
#2894=LINE ( 'NONE', #10269, #38868 ) ;
#2895=DIRECTION ( 'NONE',  ( -0.000000000000000000, 1.000000000000000000, -0.000000000000000000 ) ) ;
#2896=EDGE_CURVE ( 'NONE', #39380, #11174, #39873, .T. ) ;
#2897=CARTESIAN_POINT ( 'NONE',  ( 71.44208735029287993, -183.6283474603465606, 35.26900067126700833 ) ) ;
#2898=VERTEX_POINT ( 'NONE', #21425 ) ;
#2901=AXIS2_PLACEMENT_3D ( 'NONE', #3705, #31833, #19474 ) ;
#2903=AXIS2_PLACEMENT_3D ( 'NONE', #29131, #37549, #37280 ) ;
#2904=PLANE ( 'NONE',  #6793 ) ;
#2905=FACE_OUTER_BOUND ( 'NONE', #6954, .T. ) ;
#2908=ADVANCED_FACE ( 'NONE', ( #9350 ), #25376, .T. ) ;
#2909=DIRECTION ( 'NONE',  ( 0.1182731709213523247, 0.000000000000000000, 0.9929810960135185827 ) ) ;
#2910=DIRECTION ( 'NONE',  ( -0.000000000000000000, -1.000000000000000000, 0.000000000000000000 ) ) ;
#2912=CARTESIAN_POINT ( 'NONE',  ( -164.2512865680372727, -193.5000000000000000, -47.13604789772046644 ) ) ;
#2913=CARTESIAN_POINT ( 'NONE',  ( -170.9669310976187830, -193.5000000000000000, -24.93467037017130394 ) ) ;
#2914=ORIENTED_EDGE ( 'NONE', *, *, #26626, .F. ) ;
#2915=AXIS2_PLACEMENT_3D ( 'NONE', #4289, #20311, #40535 ) ;
#2917=CYLINDRICAL_SURFACE ( 'NONE', #1135, 125.0000000000000000 ) ;
#2919=ORIENTED_EDGE ( 'NONE', *, *, #23417, .F. ) ;
#2923=EDGE_CURVE ( 'NONE', #25127, #43983, #33772, .T. ) ;
#2924=DIRECTION ( 'NONE',  ( 0.05924062789370748011, 0.000000000000000000, 0.9982437317643217956 ) ) ;
#2926=DIRECTION ( 'NONE',  ( -0.000000000000000000, 1.000000000000000000, -0.000000000000000000 ) ) ;
#2928=LINE ( 'NONE', #18966, #28309 ) ;
#2929=CARTESIAN_POINT ( 'NONE',  ( -164.6073096293132494, -177.1207230881787780, 43.47841891815208726 ) ) ;
#2931=LINE ( 'NONE', #23933, #8839 ) ;
#2934=LINE ( 'NONE', #6376, #35599 ) ;
#2935=VERTEX_POINT ( 'NONE', #50080 ) ;
#2936=VECTOR ( 'NONE', #7553, 1000.000000000000000 ) ;
#2937=CARTESIAN_POINT ( 'NONE',  ( -37.67038537088847505, -183.6283474603465606, -124.5318076226586470 ) ) ;
#2938=FACE_OUTER_BOUND ( 'NONE', #31043, .T. ) ;
#2939=DIRECTION ( 'NONE',  ( 0.000000000000000000, -1.000000000000000000, -0.000000000000000000 ) ) ;
#2940=VECTOR ( 'NONE', #26490, 999.9999999999998863 ) ;
#2941=EDGE_LOOP ( 'NONE', ( #10313, #30842, #37717, #37536 ) ) ;
#2943=DIRECTION ( 'NONE',  ( -0.000000000000000000, 1.000000000000000000, -0.000000000000000000 ) ) ;
#2944=DIRECTION ( 'NONE',  ( 0.000000000000000000, 0.000000000000000000, 1.000000000000000000 ) ) ;
#2947=EDGE_CURVE ( 'NONE', #48835, #49515, #19779, .T. ) ;
#2948=CARTESIAN_POINT ( 'NONE',  ( -29.85296035031868911, -177.1207230881787780, 122.5936119678275844 ) ) ;
#2950=CARTESIAN_POINT ( 'NONE',  ( -4.794493649713349015, -193.5000000000000000, -117.1181148702518726 ) ) ;
#2954=LINE ( 'NONE', #18734, #18101 ) ;
#2955=EDGE_CURVE ( 'NONE', #44801, #16051, #10562, .T. ) ;
#2956=VECTOR ( 'NONE', #9154, 1000.000000000000000 ) ;
#2957=ORIENTED_EDGE ( 'NONE', *, *, #8334, .F. ) ;
#2961=CARTESIAN_POINT ( 'NONE',  ( -170.6250538923603131, -189.7472609257535510, 26.55884942729649723 ) ) ;
#2963=CARTESIAN_POINT ( 'NONE',  ( -49.47868758801764955, -177.1207230881787780, -0.02963332782256313663 ) ) ;
#2965=CARTESIAN_POINT ( 'NONE',  ( -103.4012653778457462, -183.6283474603465606, -112.2878385610366649 ) ) ;
#2966=ORIENTED_EDGE ( 'NONE', *, *, #30159, .T. ) ;
#2967=CARTESIAN_POINT ( 'NONE',  ( -109.5001801941309196, -183.6283474603465606, -107.9473519284343297 ) ) ;
#2969=DIRECTION ( 'NONE',  ( 0.000000000000000000, -1.000000000000000000, 0.000000000000000000 ) ) ;
#2970=CARTESIAN_POINT ( 'NONE',  ( 43.57032560458359427, -193.5000000000000000, 83.08371579725746869 ) ) ;
#2973=VECTOR ( 'NONE', #14794, 1000.000000000000000 ) ;
#2974=AXIS2_PLACEMENT_3D ( 'NONE', #47893, #24748, #16346 ) ;
#2975=ORIENTED_EDGE ( 'NONE', *, *, #31753, .F. ) ;
#2976=DIRECTION ( 'NONE',  ( 0.000000000000000000, 0.000000000000000000, 1.000000000000000000 ) ) ;
#2977=PLANE ( 'NONE',  #48113 ) ;
#2979=ORIENTED_EDGE ( 'NONE', *, *, #51076, .F. ) ;
#2980=DIRECTION ( 'NONE',  ( -0.9374196611341206742, 0.000000000000000000, -0.3482016354343996367 ) ) ;
#2984=DIRECTION ( 'NONE',  ( 0.000000000000000000, 0.000000000000000000, -1.000000000000000000 ) ) ;
#2985=VECTOR ( 'NONE', #49150, 1000.000000000000000 ) ;
#2986=EDGE_CURVE ( 'NONE', #10698, #24816, #16980, .T. ) ;
#2987=DIRECTION ( 'NONE',  ( -0.4566292373937200777, 0.000000000000000000, 0.8896570909947436601 ) ) ;
#2991=ORIENTED_EDGE ( 'NONE', *, *, #23932, .F. ) ;
#2993=CIRCLE ( 'NONE', #32357, 125.0000000000000000 ) ;
#2994=CARTESIAN_POINT ( 'NONE',  ( 15.23368049493604381, -175.3837268820161057, -107.5438431188757420 ) ) ;
#2996=DIRECTION ( 'NONE',  ( -0.9151456172430181280, 0.000000000000000000, -0.4031234292879730674 ) ) ;
#2998=CARTESIAN_POINT ( 'NONE',  ( -96.65280530915691770, -177.1207230881787780, -115.3442529744087324 ) ) ;
#2999=ORIENTED_EDGE ( 'NONE', *, *, #10007, .F. ) ;
#3002=ORIENTED_EDGE ( 'NONE', *, *, #25192, .T. ) ;
#3003=ORIENTED_EDGE ( 'NONE', *, *, #37644, .F. ) ;
#3005=CARTESIAN_POINT ( 'NONE',  ( 66.42899531795131907, -177.1207230881787780, 49.20491319441622124 ) ) ;
#3006=DIRECTION ( 'NONE',  ( -0.1182731709213523247, 0.000000000000000000, -0.9929810960135185827 ) ) ;
#3009=VECTOR ( 'NONE', #26277, 1000.000000000000114 ) ;
#3012=CARTESIAN_POINT ( 'NONE',  ( -70.75782287548091176, -193.5000000000000000, 122.9986166548864901 ) ) ;
#3013=CARTESIAN_POINT ( 'NONE',  ( -139.4082623311987277, -175.3837268820161057, 84.30834960113001841 ) ) ;
#3014=ORIENTED_EDGE ( 'NONE', *, *, #49400, .T. ) ;
#3016=VERTEX_POINT ( 'NONE', #5934 ) ;
#3017=FACE_OUTER_BOUND ( 'NONE', #25613, .T. ) ;
#3018=VECTOR ( 'NONE', #35769, 1000.000000000000000 ) ;
#3019=PLANE ( 'NONE',  #44621 ) ;
#3021=AXIS2_PLACEMENT_3D ( 'NONE', #42183, #18796, #50100 ) ;
#3022=CYLINDRICAL_SURFACE ( 'NONE', #14781, 125.0000000000000000 ) ;
#3023=DIRECTION ( 'NONE',  ( 0.6965510290629882695, 0.000000000000000000, 0.7175072570443395970 ) ) ;
#3024=DIRECTION ( 'NONE',  ( -0.5829794791144820021, 0.000000000000000000, 0.8124868780056742068 ) ) ;
#3025=AXIS2_PLACEMENT_3D ( 'NONE', #14367, #25930, #18321 ) ;
#3026=CARTESIAN_POINT ( 'NONE',  ( -118.1688136093591908, -193.5000000000000000, -103.7706487676296661 ) ) ;
#3028=VECTOR ( 'NONE', #25182, 1000.000000000000227 ) ;
#3029=VERTEX_POINT ( 'NONE', #34032 ) ;
#3030=DIRECTION ( 'NONE',  ( 0.000000000000000000, 1.000000000000000000, 0.000000000000000000 ) ) ;
#3031=CARTESIAN_POINT ( 'NONE',  ( -48.07600332222088468, -183.6283474603465606, 0.9151456172430280089 ) ) ;
#3032=EDGE_LOOP ( 'NONE', ( #2625, #17208, #41097, #37453 ) ) ;
#3034=VERTEX_POINT ( 'NONE', #8812 ) ;
#3035=DIRECTION ( 'NONE',  ( 0.000000000000000000, 0.000000000000000000, 1.000000000000000000 ) ) ;
#3036=EDGE_LOOP ( 'NONE', ( #29313, #32102, #4306, #26916 ) ) ;
#3038=PLANE ( 'NONE',  #41079 ) ;
#3039=AXIS2_PLACEMENT_3D ( 'NONE', #40366, #33015, #32504 ) ;
#3044=VERTEX_POINT ( 'NONE', #3983 ) ;
#3050=ORIENTED_EDGE ( 'NONE', *, *, #20215, .F. ) ;
#3051=ORIENTED_EDGE ( 'NONE', *, *, #800, .T. ) ;
#3052=EDGE_CURVE ( 'NONE', #24818, #177, #30697, .T. ) ;
#3053=ORIENTED_EDGE ( 'NONE', *, *, #4211, .F. ) ;
#3054=PLANE ( 'NONE',  #30107 ) ;
#3055=CARTESIAN_POINT ( 'NONE',  ( -23.01747912075234836, -177.1207230881787780, -122.3793467049370776 ) ) ;
#3057=EDGE_CURVE ( 'NONE', #5120, #41700, #23681, .T. ) ;
#3058=CARTESIAN_POINT ( 'NONE',  ( -156.7610986364826999, -183.6283474603465606, -62.45009659481509345 ) ) ;
#3060=DIRECTION ( 'NONE',  ( 0.000000000000000000, -1.000000000000000000, 0.000000000000000000 ) ) ;
#3061=AXIS2_PLACEMENT_3D ( 'NONE', #18088, #17832, #5240 ) ;
#3062=CYLINDRICAL_SURFACE ( 'NONE', #20469, 125.0000000000000000 ) ;
#3063=ORIENTED_EDGE ( 'NONE', *, *, #46846, .F. ) ;
#3064=CIRCLE ( 'NONE', #49224, 125.0000000000000000 ) ;
#3065=PLANE ( 'NONE',  #19855 ) ;
#3067=DIRECTION ( 'NONE',  ( 0.000000000000000000, 0.000000000000000000, 1.000000000000000000 ) ) ;
#3068=VERTEX_POINT ( 'NONE', #7423 ) ;
#3069=VERTEX_POINT ( 'NONE', #47100 ) ;
#3070=DIRECTION ( 'NONE',  ( 0.000000000000000000, -1.000000000000000000, 0.000000000000000000 ) ) ;
#3072=ADVANCED_FACE ( 'NONE', ( #23444 ), #18980, .T. ) ;
#3073=DIRECTION ( 'NONE',  ( 0.000000000000000000, -0.000000000000000000, -1.000000000000000000 ) ) ;
#3074=DIRECTION ( 'NONE',  ( -0.1768902751225666370, 0.000000000000000000, -0.9842305779475979399 ) ) ;
#3075=DIRECTION ( 'NONE',  ( 0.6300878435817148793, 0.000000000000000000, -0.7765238627180394149 ) ) ;
#3076=ORIENTED_EDGE ( 'NONE', *, *, #47711, .T. ) ;
#3077=FACE_OUTER_BOUND ( 'NONE', #12073, .T. ) ;
#3078=VERTEX_POINT ( 'NONE', #34 ) ;
#3079=ORIENTED_EDGE ( 'NONE', *, *, #4152, .T. ) ;
#3080=CARTESIAN_POINT ( 'NONE',  ( 11.10560377650620012, -177.1207230881787780, -108.7464374498168951 ) ) ;
#3081=AXIS2_PLACEMENT_3D ( 'NONE', #13770, #38898, #15013 ) ;
#3082=CARTESIAN_POINT ( 'NONE',  ( 46.01898237923986557, -193.5000000000000000, -81.82363577055902226 ) ) ;
#3083=VECTOR ( 'NONE', #40563, 1000.000000000000000 ) ;
#3087=CARTESIAN_POINT ( 'NONE',  ( -129.9529520667707914, -175.3837268820161057, -94.79987230211959570 ) ) ;
#3088=VECTOR ( 'NONE', #45524, 1000.000000000000000 ) ;
#3090=CARTESIAN_POINT ( 'NONE',  ( -49.47517659412406488, -177.1207230881787780, -0.08879589532293878651 ) ) ;
#3092=CARTESIAN_POINT ( 'NONE',  ( -99.22478721462988460, -193.5000000000000000, -113.1409892739921901 ) ) ;
#3093=PLANE ( 'NONE',  #8942 ) ;
#3097=AXIS2_PLACEMENT_3D ( 'NONE', #45252, #17896, #49183 ) ;
#3098=PLANE ( 'NONE',  #40657 ) ;
#3100=VECTOR ( 'NONE', #26864, 1000.000000000000000 ) ;
#3101=CARTESIAN_POINT ( 'NONE',  ( 31.28129687248616619, -183.6283474603465606, 96.24590808611479531 ) ) ;
#3103=ORIENTED_EDGE ( 'NONE', *, *, #44152, .F. ) ;
#3104=EDGE_CURVE ( 'NONE', #47705, #1934, #47877, .T. ) ;
#3105=FACE_OUTER_BOUND ( 'NONE', #21896, .T. ) ;
#3109=FACE_BOUND ( 'NONE', #5872, .T. ) ;
#3110=DIRECTION ( 'NONE',  ( 0.000000000000000000, 1.000000000000000000, 0.000000000000000000 ) ) ;
#3111=ADVANCED_FACE ( 'NONE', ( #35001 ), #35505, .T. ) ;
#3112=EDGE_CURVE ( 'NONE', #41165, #35901, #7227, .T. ) ;
#3113=PLANE ( 'NONE',  #19333 ) ;
#3114=ORIENTED_EDGE ( 'NONE', *, *, #18878, .F. ) ;
#3116=ORIENTED_EDGE ( 'NONE', *, *, #22392, .F. ) ;
#3117=DIRECTION ( 'NONE',  ( 0.000000000000000000, 1.000000000000000000, 0.000000000000000000 ) ) ;
#3119=VECTOR ( 'NONE', #28363, 1000.000000000000000 ) ;
#3121=EDGE_LOOP ( 'NONE', ( #15323, #40152, #28164, #32190 ) ) ;
#3122=DIRECTION ( 'NONE',  ( -0.000000000000000000, -1.000000000000000000, 0.000000000000000000 ) ) ;
#3123=AXIS2_PLACEMENT_3D ( 'NONE', #668, #4342, #27991 ) ;
#3124=ADVANCED_FACE ( 'NONE', ( #11077 ), #43139, .T. ) ;
#3129=LINE ( 'NONE', #30715, #7153 ) ;
#3130=ORIENTED_EDGE ( 'NONE', *, *, #18472, .F. ) ;
#3132=AXIS2_PLACEMENT_3D ( 'NONE', #26330, #21355, #13998 ) ;
#3134=CARTESIAN_POINT ( 'NONE',  ( -167.9436818089035626, -183.6283474603465606, 36.78613984830037253 ) ) ;
#3135=ORIENTED_EDGE ( 'NONE', *, *, #15115, .F. ) ;
#3136=CARTESIAN_POINT ( 'NONE',  ( 72.14504940832446778, -175.3837268820161057, -32.78426643622660208 ) ) ;
#3137=ORIENTED_EDGE ( 'NONE', *, *, #21168, .T. ) ;
#3138=AXIS2_PLACEMENT_3D ( 'NONE', #20212, #28603, #28349 ) ;
#3139=LINE ( 'NONE', #11784, #27555 ) ;
#3142=DIRECTION ( 'NONE',  ( 0.000000000000000000, 0.000000000000000000, 1.000000000000000000 ) ) ;
#3144=CIRCLE ( 'NONE', #32518, 125.0000000000000000 ) ;
#3145=LINE ( 'NONE', #43604, #15646 ) ;
#3146=EDGE_CURVE ( 'NONE', #16791, #46777, #7146, .T. ) ;
#3147=VERTEX_POINT ( 'NONE', #23186 ) ;
#3151=DIRECTION ( 'NONE',  ( -0.9842305779475992722, 0.000000000000000000, 0.1768902751225592818 ) ) ;
#3152=CARTESIAN_POINT ( 'NONE',  ( 17.15229921100054611, -193.5000000000000000, -106.3838142112212921 ) ) ;
#3157=CARTESIAN_POINT ( 'NONE',  ( 72.89680503569744019, -175.3837268820161057, -25.37485791684304104 ) ) ;
#3158=DIRECTION ( 'NONE',  ( 0.000000000000000000, -0.000000000000000000, -1.000000000000000000 ) ) ;
#3159=EDGE_CURVE ( 'NONE', #47840, #4101, #20007, .T. ) ;
#3160=DIRECTION ( 'NONE',  ( 0.000000000000000000, 0.000000000000000000, -1.000000000000000000 ) ) ;
#3162=CIRCLE ( 'NONE', #36734, 125.0000000000000000 ) ;
#3163=VECTOR ( 'NONE', #33338, 1000.000000000000114 ) ;
#3164=CARTESIAN_POINT ( 'NONE',  ( -157.5429198988176438, -175.3837268820161057, 61.07445476073478829 ) ) ;
#3166=DIRECTION ( 'NONE',  ( 0.7765238627180393038, 0.000000000000000000, 0.6300878435817147682 ) ) ;
#3167=CIRCLE ( 'NONE', #16614, 125.0000000000000000 ) ;
#3168=ADVANCED_FACE ( 'NONE', ( #51824 ), #15827, .F. ) ;
#3169=CARTESIAN_POINT ( 'NONE',  ( -9.070200226166578616, -183.6283474603465606, -117.5715283571803980 ) ) ;
#3170=EDGE_CURVE ( 'NONE', #41712, #41605, #3212, .T. ) ;
#3172=EDGE_LOOP ( 'NONE', ( #6180, #10770, #244, #46153 ) ) ;
#3174=EDGE_CURVE ( 'NONE', #172, #14931, #16075, .T. ) ;
#3178=EDGE_CURVE ( 'NONE', #45491, #50412, #37419, .T. ) ;
#3179=PLANE ( 'NONE',  #51395 ) ;
#3187=AXIS2_PLACEMENT_3D ( 'NONE', #17874, #21564, #37593 ) ;
#3188=EDGE_LOOP ( 'NONE', ( #1250, #23013, #46451, #42945 ) ) ;
#3191=ORIENTED_EDGE ( 'NONE', *, *, #24243, .F. ) ;
#3193=ADVANCED_FACE ( 'NONE', ( #4503 ), #28915, .T. ) ;
#3194=CARTESIAN_POINT ( 'NONE',  ( -71.22983192549011733, -193.5000000000000000, -121.8950816227732759 ) ) ;
#3195=ORIENTED_EDGE ( 'NONE', *, *, #34838, .T. ) ;
#3196=EDGE_CURVE ( 'NONE', #2898, #19322, #17290, .T. ) ;
#3202=VERTEX_POINT ( 'NONE', #44706 ) ;
#3203=VECTOR ( 'NONE', #38566, 1000.000000000000000 ) ;
#3204=DIRECTION ( 'NONE',  ( -0.000000000000000000, 1.000000000000000000, -0.000000000000000000 ) ) ;
#3205=ORIENTED_EDGE ( 'NONE', *, *, #15658, .F. ) ;
#3206=DIRECTION ( 'NONE',  ( -0.000000000000000000, 1.000000000000000000, -0.000000000000000000 ) ) ;
#3208=EDGE_LOOP ( 'NONE', ( #33028, #12217, #24797, #7841 ) ) ;
#3210=LINE ( 'NONE', #36284, #21274 ) ;
#3212=LINE ( 'NONE', #43913, #15596 ) ;
#3213=EDGE_CURVE ( 'NONE', #15652, #2485, #44976, .T. ) ;
#3214=ORIENTED_EDGE ( 'NONE', *, *, #14447, .F. ) ;
#3215=ADVANCED_FACE ( 'NONE', ( #16322 ), #44183, .T. ) ;
#3216=CIRCLE ( 'NONE', #39296, 10.00000000000000000 ) ;
#3217=DIRECTION ( 'NONE',  ( -0.8896570909947530970, 0.000000000000000000, 0.4566292373937018700 ) ) ;
#3218=EDGE_LOOP ( 'NONE', ( #25213, #23302, #5416, #36452 ) ) ;
#3220=FACE_OUTER_BOUND ( 'NONE', #22079, .T. ) ;
#3221=VERTEX_POINT ( 'NONE', #37067 ) ;
#3222=CARTESIAN_POINT ( 'NONE',  ( -44.48323084606168720, -183.6283474603465606, 124.9361149384469769 ) ) ;
#3223=CARTESIAN_POINT ( 'NONE',  ( -160.0666658415768211, -189.7472609257535510, 54.07611884703388228 ) ) ;
#3224=ORIENTED_EDGE ( 'NONE', *, *, #49030, .F. ) ;
#3227=VECTOR ( 'NONE', #30725, 1000.000000000000114 ) ;
#3228=VERTEX_POINT ( 'NONE', #40481 ) ;
#3229=DIRECTION ( 'NONE',  ( -0.9995608365087946812, 0.000000000000000000, 0.02963332782254913048 ) ) ;
#3230=VERTEX_POINT ( 'NONE', #5292 ) ;
#3231=CARTESIAN_POINT ( 'NONE',  ( -32.87124591993210743, -189.7472609257535510, 124.0217483183788119 ) ) ;
#3233=ORIENTED_EDGE ( 'NONE', *, *, #42858, .F. ) ;
#3234=EDGE_CURVE ( 'NONE', #31475, #44335, #32337, .T. ) ;
#3235=DIRECTION ( 'NONE',  ( 0.000000000000000000, -1.000000000000000000, 0.000000000000000000 ) ) ;
#3236=FACE_OUTER_BOUND ( 'NONE', #16434, .T. ) ;
#3237=LINE ( 'NONE', #11103, #27422 ) ;
#3238=ADVANCED_FACE ( 'NONE', ( #21308 ), #28653, .T. ) ;
#3239=EDGE_CURVE ( 'NONE', #42978, #2870, #16859, .T. ) ;
#3240=DIRECTION ( 'NONE',  ( 0.000000000000000000, -1.000000000000000000, 0.000000000000000000 ) ) ;
#3241=EDGE_CURVE ( 'NONE', #33090, #39789, #12099, .T. ) ;
#3243=CIRCLE ( 'NONE', #27576, 125.0000000000000000 ) ;
#3244=CIRCLE ( 'NONE', #11634, 125.0000000000000000 ) ;
#3245=FACE_OUTER_BOUND ( 'NONE', #3352, .T. ) ;
#3246=LINE ( 'NONE', #2970, #39435 ) ;
#3247=DIRECTION ( 'NONE',  ( 0.000000000000000000, 0.000000000000000000, -1.000000000000000000 ) ) ;
#3248=EDGE_LOOP ( 'NONE', ( #17782, #36932, #27312, #37146 ) ) ;
#3250=ORIENTED_EDGE ( 'NONE', *, *, #19208, .F. ) ;
#3251=FACE_OUTER_BOUND ( 'NONE', #51139, .T. ) ;
#3253=ORIENTED_EDGE ( 'NONE', *, *, #9309, .F. ) ;
#3255=EDGE_LOOP ( 'NONE', ( #32611, #29820, #3806, #22783 ) ) ;
#3256=LINE ( 'NONE', #31353, #44938 ) ;
#3258=CARTESIAN_POINT ( 'NONE',  ( -47.48307690889363641, -193.5000000000000000, 0.08879589532294547560 ) ) ;
#3259=DIRECTION ( 'NONE',  ( 0.000000000000000000, -1.000000000000000000, -0.000000000000000000 ) ) ;
#3261=FACE_OUTER_BOUND ( 'NONE', #23587, .T. ) ;
#3262=ORIENTED_EDGE ( 'NONE', *, *, #33020, .T. ) ;
#3263=ORIENTED_EDGE ( 'NONE', *, *, #21170, .T. ) ;
#3269=DIRECTION ( 'NONE',  ( -0.000000000000000000, 1.000000000000000000, 0.000000000000000000 ) ) ;
#3271=PLANE ( 'NONE',  #34788 ) ;
#3272=ORIENTED_EDGE ( 'NONE', *, *, #34338, .F. ) ;
#3273=DIRECTION ( 'NONE',  ( 0.000000000000000000, -1.000000000000000000, -0.000000000000000000 ) ) ;
#3274=LINE ( 'NONE', #50849, #15651 ) ;
#3277=DIRECTION ( 'NONE',  ( -0.9785564922995060311, 0.000000000000000000, 0.2059786187410889424 ) ) ;
#3278=DIRECTION ( 'NONE',  ( -0.5586467658036535777, 0.000000000000000000, 0.8294056854502011022 ) ) ;
#3280=ORIENTED_EDGE ( 'NONE', *, *, #2319, .T. ) ;
#3281=DIRECTION ( 'NONE',  ( 0.000000000000000000, 0.000000000000000000, -1.000000000000000000 ) ) ;
#3282=VECTOR ( 'NONE', #26512, 1000.000000000000227 ) ;
#3287=ORIENTED_EDGE ( 'NONE', *, *, #19178, .T. ) ;
#3290=DIRECTION ( 'NONE',  ( -0.000000000000000000, 1.000000000000000000, 0.000000000000000000 ) ) ;
#3295=EDGE_CURVE ( 'NONE', #39399, #14153, #9229, .T. ) ;
#3296=LINE ( 'NONE', #4077, #47590 ) ;
#3297=AXIS2_PLACEMENT_3D ( 'NONE', #30598, #51624, #11677 ) ;
#3298=LINE ( 'NONE', #24302, #51346 ) ;
#3300=VERTEX_POINT ( 'NONE', #46271 ) ;
#3301=CARTESIAN_POINT ( 'NONE',  ( -126.3604277550460750, -193.5000000000000000, 96.49160960477099991 ) ) ;
#3305=DIRECTION ( 'NONE',  ( 0.6528221181905227155, 0.000000000000000000, -0.7575112421616191360 ) ) ;
#3309=CARTESIAN_POINT ( 'NONE',  ( -63.96873441216510514, -193.5000000000000000, -123.0287672223651612 ) ) ;
#3312=ORIENTED_EDGE ( 'NONE', *, *, #3999, .F. ) ;
#3313=DIRECTION ( 'NONE',  ( -0.000000000000000000, 1.000000000000000000, -0.000000000000000000 ) ) ;
#3314=AXIS2_PLACEMENT_3D ( 'NONE', #24386, #13346, #48581 ) ;
#3317=ORIENTED_EDGE ( 'NONE', *, *, #1641, .F. ) ;
#3318=VERTEX_POINT ( 'NONE', #30475 ) ;
#3321=DIRECTION ( 'NONE',  ( 0.000000000000000000, -1.000000000000000000, 0.000000000000000000 ) ) ;
#3322=DIRECTION ( 'NONE',  ( 0.000000000000000000, -0.000000000000000000, 1.000000000000000000 ) ) ;
#3323=CARTESIAN_POINT ( 'NONE',  ( -154.0877180371535928, -193.5000000000000000, -66.87170886601927577 ) ) ;
#3325=ORIENTED_EDGE ( 'NONE', *, *, #32706, .F. ) ;
#3326=EDGE_CURVE ( 'NONE', #33929, #15769, #22077, .T. ) ;
#3327=VECTOR ( 'NONE', #33820, 1000.000000000000000 ) ;
#3329=ORIENTED_EDGE ( 'NONE', *, *, #5103, .T. ) ;
#3331=EDGE_LOOP ( 'NONE', ( #41235, #21299, #11048, #39196 ) ) ;
#3332=ORIENTED_EDGE ( 'NONE', *, *, #37399, .F. ) ;
#3333=ADVANCED_FACE ( 'NONE', ( #10252 ), #1330, .T. ) ;
#3334=CARTESIAN_POINT ( 'NONE',  ( -48.30901192927175458, -189.7472609257535510, -123.9998842437354227 ) ) ;
#3335=DIRECTION ( 'NONE',  ( -0.8124868780056863082, 0.000000000000000000, 0.5829794791144649047 ) ) ;
#3336=CARTESIAN_POINT ( 'NONE',  ( 74.60098876342242136, -177.1207230881787780, 21.82395850507348811 ) ) ;
#3337=CARTESIAN_POINT ( 'NONE',  ( -118.4510020108455137, -175.3837268820161057, 103.5805805771131674 ) ) ;
#3338=EDGE_LOOP ( 'NONE', ( #51, #12060, #16979, #19414 ) ) ;
#3339=DIRECTION ( 'NONE',  ( -0.1768902751225802927, 0.000000000000000000, 0.9842305779475953864 ) ) ;
#3340=ORIENTED_EDGE ( 'NONE', *, *, #50117, .F. ) ;
#3342=VERTEX_POINT ( 'NONE', #33408 ) ;
#3343=CARTESIAN_POINT ( 'NONE',  ( -48.47912675150885065, -183.6283474603465606, 6.938893903907228378E-15 ) ) ;
#3344=CARTESIAN_POINT ( 'NONE',  ( 8.750818922897904528, -175.3837268820161057, -111.1293539894138434 ) ) ;
#3346=DIRECTION ( 'NONE',  ( 0.7175072570443348230, 0.000000000000000000, -0.6965510290629933765 ) ) ;
#3347=LINE ( 'NONE', #15447, #49201 ) ;
#3348=PLANE ( 'NONE',  #34808 ) ;
#3349=LINE ( 'NONE', #22285, #2003 ) ;
#3351=ADVANCED_FACE ( 'NONE', ( #6583 ), #14210, .T. ) ;
#3352=EDGE_LOOP ( 'NONE', ( #51491, #5309, #27605, #29110 ) ) ;
#3353=DIRECTION ( 'NONE',  ( 0.000000000000000000, 0.000000000000000000, 1.000000000000000000 ) ) ;
#3354=DIRECTION ( 'NONE',  ( 0.8455960035018234011, 0.000000000000000000, 0.5338233779647948429 ) ) ;
#3355=EDGE_CURVE ( 'NONE', #43312, #40054, #1337, .T. ) ;
#3356=FACE_OUTER_BOUND ( 'NONE', #1998, .T. ) ;
#3358=ADVANCED_FACE ( 'NONE', ( #21580 ), #9740, .F. ) ;
#3359=CARTESIAN_POINT ( 'NONE',  ( -146.2338470511239166, -193.5000000000000000, 76.29032973288703090 ) ) ;
#3360=CYLINDRICAL_SURFACE ( 'NONE', #33676, 125.0000000000000000 ) ;
#3361=ORIENTED_EDGE ( 'NONE', *, *, #2511, .F. ) ;
#3363=VERTEX_POINT ( 'NONE', #46518 ) ;
#3364=AXIS2_PLACEMENT_3D ( 'NONE', #22470, #50329, #22198 ) ;
#3365=AXIS2_PLACEMENT_3D ( 'NONE', #10603, #26108, #30063 ) ;
#3367=FACE_BOUND ( 'NONE', #35965, .T. ) ;
#3368=CARTESIAN_POINT ( 'NONE',  ( -48.47912675150885065, -189.7472609257535510, -0.9999999999999931166 ) ) ;
#3369=EDGE_CURVE ( 'NONE', #38792, #48181, #51830, .T. ) ;
#3370=CARTESIAN_POINT ( 'NONE',  ( -40.24578378811990831, -189.7472609257535510, 124.7285535218268251 ) ) ;
#3372=VERTEX_POINT ( 'NONE', #13680 ) ;
#3374=AXIS2_PLACEMENT_3D ( 'NONE', #51221, #7823, #27544 ) ;
#3376=DIRECTION ( 'NONE',  ( -0.000000000000000000, 1.000000000000000000, -0.000000000000000000 ) ) ;
#3377=EDGE_CURVE ( 'NONE', #48181, #6100, #25504, .T. ) ;
#3378=DIRECTION ( 'NONE',  ( -0.7378332790417333475, 0.000000000000000000, 0.6749830015182038956 ) ) ;
#3382=DIRECTION ( 'NONE',  ( 0.000000000000000000, 0.000000000000000000, -1.000000000000000000 ) ) ;
#3384=LINE ( 'NONE', #7842, #26468 ) ;
#3385=EDGE_LOOP ( 'NONE', ( #29736, #48906, #996, #36839 ) ) ;
#3386=CARTESIAN_POINT ( 'NONE',  ( 28.02885774092381865, -193.5000000000000000, 98.85104101073331151 ) ) ;
#3389=ADVANCED_FACE ( 'NONE', ( #50470 ), #5822, .T. ) ;
#3391=ORIENTED_EDGE ( 'NONE', *, *, #16645, .T. ) ;
#3392=DIRECTION ( 'NONE',  ( 0.000000000000000000, 0.000000000000000000, 1.000000000000000000 ) ) ;
#3394=ORIENTED_EDGE ( 'NONE', *, *, #20125, .F. ) ;
#3398=ORIENTED_EDGE ( 'NONE', *, *, #3355, .F. ) ;
#3400=DIRECTION ( 'NONE',  ( 0.000000000000000000, -0.000000000000000000, -1.000000000000000000 ) ) ;
#3402=DIRECTION ( 'NONE',  ( 0.1768902751225802927, 0.000000000000000000, -0.9842305779475953864 ) ) ;
#3403=CARTESIAN_POINT ( 'NONE',  ( -155.9608607592036833, -177.1207230881787780, 63.81752780153064464 ) ) ;
#3405=ORIENTED_EDGE ( 'NONE', *, *, #13325, .F. ) ;
#3407=LINE ( 'NONE', #6844, #23762 ) ;
#3410=PLANE ( 'NONE',  #39661 ) ;
#3412=ADVANCED_FACE ( 'NONE', ( #38365 ), #42294, .T. ) ;
#3413=AXIS2_PLACEMENT_3D ( 'NONE', #41633, #49804, #37435 ) ;
#3414=CARTESIAN_POINT ( 'NONE',  ( -33.86391487983341619, -193.5000000000000000, 124.1426420773540542 ) ) ;
#3415=DIRECTION ( 'NONE',  ( 0.000000000000000000, 1.000000000000000000, 0.000000000000000000 ) ) ;
#3417=CARTESIAN_POINT ( 'NONE',  ( 75.17589904515341459, -189.7472609257535510, -18.28755301364250840 ) ) ;
#3418=FACE_OUTER_BOUND ( 'NONE', #12100, .T. ) ;
#3419=VERTEX_POINT ( 'NONE', #50721 ) ;
#3420=ORIENTED_EDGE ( 'NONE', *, *, #51153, .F. ) ;
#3424=CARTESIAN_POINT ( 'NONE',  ( 75.48400724637754422, -177.1207230881787780, -16.06677968424457248 ) ) ;
#3425=LINE ( 'NONE', #10802, #22018 ) ;
#3429=AXIS2_PLACEMENT_3D ( 'NONE', #42594, #6608, #22630 ) ;
#3430=ORIENTED_EDGE ( 'NONE', *, *, #28488, .F. ) ;
#3432=VERTEX_POINT ( 'NONE', #35443 ) ;
#3433=CARTESIAN_POINT ( 'NONE',  ( -238.7407812814481076, -213.5000000000000000, 41.45482488023466772 ) ) ;
#3434=CARTESIAN_POINT ( 'NONE',  ( -137.9639882952644143, -177.1207230881787780, 87.27805883780240492 ) ) ;
#3435=VERTEX_POINT ( 'NONE', #22856 ) ;
#3438=DIRECTION ( 'NONE',  ( -0.7765238627180437447, 0.000000000000000000, 0.6300878435817094392 ) ) ;
#3440=ORIENTED_EDGE ( 'NONE', *, *, #33669, .F. ) ;
#3441=EDGE_CURVE ( 'NONE', #6834, #16650, #6830, .T. ) ;
#3442=DIRECTION ( 'NONE',  ( 0.000000000000000000, 0.000000000000000000, 1.000000000000000000 ) ) ;
#3443=ORIENTED_EDGE ( 'NONE', *, *, #29152, .T. ) ;
#3444=FACE_OUTER_BOUND ( 'NONE', #21415, .T. ) ;
#3445=EDGE_LOOP ( 'NONE', ( #14608, #14809, #20458, #12759 ) ) ;
#3446=EDGE_CURVE ( 'NONE', #47743, #3034, #15233, .T. ) ;
#3448=EDGE_CURVE ( 'NONE', #716, #19679, #26645, .T. ) ;
#3449=PLANE ( 'NONE',  #28266 ) ;
#3450=CARTESIAN_POINT ( 'NONE',  ( -48.13092511607445090, -189.7472609257535510, -0.9374196611341135688 ) ) ;
#3453=ORIENTED_EDGE ( 'NONE', *, *, #34271, .F. ) ;
#3454=ADVANCED_FACE ( 'NONE', ( #11013 ), #42821, .T. ) ;
#3455=DIRECTION ( 'NONE',  ( -0.000000000000000000, -1.000000000000000000, 0.000000000000000000 ) ) ;
#3456=CARTESIAN_POINT ( 'NONE',  ( 5.139251539934009294, -193.5000000000000000, 111.8087531435658093 ) ) ;
#3457=SHAPE_REPRESENTATION_RELATIONSHIP ( 'NONE' , 'NONE' ,  #2890, #36813 ) ;
#3458=ORIENTED_EDGE ( 'NONE', *, *, #48473, .F. ) ;
#3460=LINE ( 'NONE', #15560, #14024 ) ;
#3462=LINE ( 'NONE', #18471, #31550 ) ;
#3466=CARTESIAN_POINT ( 'NONE',  ( 70.19984492582109681, -189.7472609257535510, 39.24667733211968823 ) ) ;
#3467=EDGE_CURVE ( 'NONE', #50634, #25658, #43347, .T. ) ;
#3469=DIRECTION ( 'NONE',  ( 0.000000000000000000, 0.000000000000000000, 1.000000000000000000 ) ) ;
#3470=VERTEX_POINT ( 'NONE', #51495 ) ;
#3471=EDGE_CURVE ( 'NONE', #194, #34268, #35193, .T. ) ;
#3473=FACE_OUTER_BOUND ( 'NONE', #49138, .T. ) ;
#3475=DIRECTION ( 'NONE',  ( 0.000000000000000000, 1.000000000000000000, -0.000000000000000000 ) ) ;
#3476=CARTESIAN_POINT ( 'NONE',  ( 57.66105628977221897, -189.7472609257535510, 66.02470404298190942 ) ) ;
#3478=AXIS2_PLACEMENT_3D ( 'NONE', #45075, #48227, #120 ) ;
#3482=CARTESIAN_POINT ( 'NONE',  ( 74.77174840718836890, -177.1207230881787780, 20.83798868929603643 ) ) ;
#3484=CARTESIAN_POINT ( 'NONE',  ( -131.8938452225253855, -193.5000000000000000, 93.09664195018558530 ) ) ;
#3485=ORIENTED_EDGE ( 'NONE', *, *, #45972, .F. ) ;
#3486=ORIENTED_EDGE ( 'NONE', *, *, #22210, .T. ) ;
#3488=EDGE_CURVE ( 'NONE', #16247, #46453, #38618, .T. ) ;
#3492=CARTESIAN_POINT ( 'NONE',  ( -10.02015192278479816, -193.5000000000000000, -117.8859915627474351 ) ) ;
#3493=ORIENTED_EDGE ( 'NONE', *, *, #21501, .F. ) ;
#3495=DIRECTION ( 'NONE',  ( 0.000000000000000000, 0.000000000000000000, -1.000000000000000000 ) ) ;
#3497=CARTESIAN_POINT ( 'NONE',  ( -96.65280530915693191, -183.6283474603465606, -115.3442529744087466 ) ) ;
#3498=CARTESIAN_POINT ( 'NONE',  ( -5.732832253866456007, -193.5000000000000000, -117.4638425504666657 ) ) ;
#3499=CIRCLE ( 'NONE', #26911, 125.0000000000000000 ) ;
#3501=ORIENTED_EDGE ( 'NONE', *, *, #7872, .F. ) ;
#3503=ORIENTED_EDGE ( 'NONE', *, *, #40056, .F. ) ;
#3505=CARTESIAN_POINT ( 'NONE',  ( -167.1668396246903114, -183.6283474603465606, -35.90758392117663078 ) ) ;
#3506=CARTESIAN_POINT ( 'NONE',  ( 72.95485052494851175, -177.1207230881787780, -29.64437826672757481 ) ) ;
#3507=DIRECTION ( 'NONE',  ( 1.000000000000000000, 0.000000000000000000, -6.978251959525016136E-17 ) ) ;
#3508=CARTESIAN_POINT ( 'NONE',  ( 62.86098202833237281, -177.1207230881787780, 56.81883646197908178 ) ) ;
#3509=DIRECTION ( 'NONE',  ( 0.8858462335218260097, 0.000000000000000000, 0.4639789333096864810 ) ) ;
#3510=ORIENTED_EDGE ( 'NONE', *, *, #20220, .T. ) ;
#3511=PLANE ( 'NONE',  #37265 ) ;
#3512=EDGE_CURVE ( 'NONE', #32383, #25127, #28319, .T. ) ;
#3514=EDGE_CURVE ( 'NONE', #27512, #39811, #15771, .T. ) ;
#3515=DIRECTION ( 'NONE',  ( 0.9646355819083594074, 0.000000000000000000, -0.2635871660690647933 ) ) ;
#3517=AXIS2_PLACEMENT_3D ( 'NONE', #39236, #31600, #7449 ) ;
#3518=EDGE_CURVE ( 'NONE', #32642, #26711, #11787, .T. ) ;
#3519=ORIENTED_EDGE ( 'NONE', *, *, #6256, .T. ) ;
#3520=ORIENTED_EDGE ( 'NONE', *, *, #42548, .T. ) ;
#3521=CIRCLE ( 'NONE', #24526, 125.0000000000000000 ) ;
#3522=EDGE_LOOP ( 'NONE', ( #20710, #17163, #20618, #27399 ) ) ;
#3523=CIRCLE ( 'NONE', #29518, 124.9999999999999858 ) ;
#3525=CARTESIAN_POINT ( 'NONE',  ( 51.65665342072240662, -193.5000000000000000, 74.81861753132422166 ) ) ;
#3528=CARTESIAN_POINT ( 'NONE',  ( 16.59365244519689497, -177.1207230881787780, -105.5544085257710805 ) ) ;
#3535=CARTESIAN_POINT ( 'NONE',  ( -140.5933766095837427, -193.5000000000000000, -84.49831343337065448 ) ) ;
#3536=VERTEX_POINT ( 'NONE', #40674 ) ;
#3537=AXIS2_PLACEMENT_3D ( 'NONE', #27575, #39391, #28346 ) ;
#3542=CARTESIAN_POINT ( 'NONE',  ( -59.86929868745821182, -177.1207230881787780, -124.4799742258549600 ) ) ;
#3543=EDGE_CURVE ( 'NONE', #2646, #9485, #17440, .T. ) ;
#3544=AXIS2_PLACEMENT_3D ( 'NONE', #17089, #5521, #33095 ) ;
#3546=ORIENTED_EDGE ( 'NONE', *, *, #5199, .T. ) ;
#3549=LINE ( 'NONE', #8013, #32962 ) ;
#3555=DIRECTION ( 'NONE',  ( -0.000000000000000000, 1.000000000000000000, -0.000000000000000000 ) ) ;
#3556=VECTOR ( 'NONE', #19381, 1000.000000000000000 ) ;
#3557=AXIS2_PLACEMENT_3D ( 'NONE', #42425, #30334, #46386 ) ;
#3560=CARTESIAN_POINT ( 'NONE',  ( -166.6265240196292439, -189.7472609257535510, 40.81902153125349031 ) ) ;
#3561=ORIENTED_EDGE ( 'NONE', *, *, #20174, .T. ) ;
#3564=PLANE ( 'NONE',  #16864 ) ;
#3565=DIRECTION ( 'NONE',  ( 0.000000000000000000, 0.000000000000000000, 1.000000000000000000 ) ) ;
#3569=LINE ( 'NONE', #31946, #6456 ) ;
#3570=DIRECTION ( 'NONE',  ( -0.000000000000000000, 1.000000000000000000, -0.000000000000000000 ) ) ;
#3571=DIRECTION ( 'NONE',  ( -0.9960498426152177842, 0.000000000000000000, 0.08879589532292482545 ) ) ;
#3573=FACE_OUTER_BOUND ( 'NONE', #49897, .T. ) ;
#3574=FACE_OUTER_BOUND ( 'NONE', #7080, .T. ) ;
#3576=EDGE_LOOP ( 'NONE', ( #33450, #11548, #45678, #21384 ) ) ;
#3577=EDGE_CURVE ( 'NONE', #21083, #43984, #39245, .T. ) ;
#3579=AXIS2_PLACEMENT_3D ( 'NONE', #33927, #46051, #2651 ) ;
#3580=DIRECTION ( 'NONE',  ( 0.000000000000000000, 1.000000000000000000, 0.000000000000000000 ) ) ;
#3583=EDGE_LOOP ( 'NONE', ( #15764, #3824, #5741, #16773 ) ) ;
#3584=VERTEX_POINT ( 'NONE', #8634 ) ;
#3585=CARTESIAN_POINT ( 'NONE',  ( 60.02977459919873837, -189.7472609257535510, 60.01515274641012354 ) ) ;
#3587=DIRECTION ( 'NONE',  ( -0.000000000000000000, -1.000000000000000000, 0.000000000000000000 ) ) ;
#3588=CARTESIAN_POINT ( 'NONE',  ( -81.14588623932559130, -193.5000000000000000, 120.6560517527618117 ) ) ;
#3589=VERTEX_POINT ( 'NONE', #36476 ) ;
#3590=PLANE ( 'NONE',  #36779 ) ;
#3591=EDGE_LOOP ( 'NONE', ( #33582, #4812, #21268, #17034 ) ) ;
#3592=AXIS2_PLACEMENT_3D ( 'NONE', #10470, #34643, #23354 ) ;
#3593=ORIENTED_EDGE ( 'NONE', *, *, #34601, .F. ) ;
#3594=CARTESIAN_POINT ( 'NONE',  ( -140.5285791076019279, -193.5000000000000000, -83.08371579725672973 ) ) ;
#3595=VECTOR ( 'NONE', #37562, 1000.000000000000114 ) ;
#3597=AXIS2_PLACEMENT_3D ( 'NONE', #2464, #26367, #6670 ) ;
#3598=EDGE_CURVE ( 'NONE', #20728, #14521, #45183, .T. ) ;
#3599=LINE ( 'NONE', #35393, #38722 ) ;
#3600=DIRECTION ( 'NONE',  ( -0.000000000000000000, -1.000000000000000000, 0.000000000000000000 ) ) ;
#3601=CARTESIAN_POINT ( 'NONE',  ( -62.43888699632653783, -189.7472609257535510, 124.2180546213279371 ) ) ;
#3602=DIRECTION ( 'NONE',  ( 0.000000000000000000, 1.000000000000000000, 0.000000000000000000 ) ) ;
#3604=AXIS2_PLACEMENT_3D ( 'NONE', #8347, #20686, #44356 ) ;
#3609=DIRECTION ( 'NONE',  ( 0.000000000000000000, 0.000000000000000000, -1.000000000000000000 ) ) ;
#3610=ORIENTED_EDGE ( 'NONE', *, *, #799, .T. ) ;
#3611=CARTESIAN_POINT ( 'NONE',  ( -47.60339180931321579, -175.3837268820161057, -0.4827922027307358088 ) ) ;
#3612=AXIS2_PLACEMENT_3D ( 'NONE', #17524, #28534, #24602 ) ;
#3615=DIRECTION ( 'NONE',  ( -0.5085311186492216251, 0.000000000000000000, 0.8610436117673548884 ) ) ;
#3616=VERTEX_POINT ( 'NONE', #20202 ) ;
#3617=VECTOR ( 'NONE', #19775, 1000.000000000000000 ) ;
#3618=DIRECTION ( 'NONE',  ( -0.8896570909947530970, 0.000000000000000000, 0.4566292373937018700 ) ) ;
#3619=FACE_BOUND ( 'NONE', #26900, .T. ) ;
#3621=EDGE_LOOP ( 'NONE', ( #35276, #11424, #48111, #42430 ) ) ;
#3622=LINE ( 'NONE', #39366, #20176 ) ;
#3623=CIRCLE ( 'NONE', #45591, 125.0000000000000000 ) ;
#3624=VERTEX_POINT ( 'NONE', #1005 ) ;
#3625=EDGE_CURVE ( 'NONE', #20913, #8106, #40417, .T. ) ;
#3627=DIRECTION ( 'NONE',  ( -0.000000000000000000, 1.000000000000000000, -0.000000000000000000 ) ) ;
#3631=DIRECTION ( 'NONE',  ( 0.000000000000000000, 0.000000000000000000, -1.000000000000000000 ) ) ;
#3632=EDGE_CURVE ( 'NONE', #21416, #51078, #4440, .T. ) ;
#3635=CARTESIAN_POINT ( 'NONE',  ( 64.46023522152407281, -177.1207230881787780, -51.19472891551279758 ) ) ;
#3636=EDGE_LOOP ( 'NONE', ( #41958, #31796, #11032, #22327 ) ) ;
#3639=ORIENTED_EDGE ( 'NONE', *, *, #16504, .T. ) ;
#3642=DIRECTION ( 'NONE',  ( -0.000000000000000000, 1.000000000000000000, -0.000000000000000000 ) ) ;
#3643=ORIENTED_EDGE ( 'NONE', *, *, #33662, .T. ) ;
#3644=DIRECTION ( 'NONE',  ( -0.000000000000000000, 1.000000000000000000, -0.000000000000000000 ) ) ;
#3645=CIRCLE ( 'NONE', #41390, 125.0000000000000000 ) ;
#3647=CARTESIAN_POINT ( 'NONE',  ( -48.47912675150885065, -189.7472609257535510, 6.938893903907228378E-15 ) ) ;
#3648=VERTEX_POINT ( 'NONE', #12577 ) ;
#3651=EDGE_LOOP ( 'NONE', ( #3780, #414, #50924, #21620 ) ) ;
#3652=AXIS2_PLACEMENT_3D ( 'NONE', #13894, #21001, #1017 ) ;
#3654=ORIENTED_EDGE ( 'NONE', *, *, #25015, .T. ) ;
#3656=DIRECTION ( 'NONE',  ( 0.000000000000000000, 0.000000000000000000, 1.000000000000000000 ) ) ;
#3658=LINE ( 'NONE', #52037, #37267 ) ;
#3659=PLANE ( 'NONE',  #19945 ) ;
#3660=DIRECTION ( 'NONE',  ( -0.000000000000000000, 1.000000000000000000, -0.000000000000000000 ) ) ;
#3661=FACE_OUTER_BOUND ( 'NONE', #318, .T. ) ;
#3663=ORIENTED_EDGE ( 'NONE', *, *, #17023, .F. ) ;
#3666=LINE ( 'NONE', #19963, #26308 ) ;
#3667=CARTESIAN_POINT ( 'NONE',  ( -48.47912675150885065, -189.7472609257535510, 6.938893903907228378E-15 ) ) ;
#3668=CARTESIAN_POINT ( 'NONE',  ( 62.86098202833237281, -193.5000000000000000, 56.81883646197908178 ) ) ;
#3671=DIRECTION ( 'NONE',  ( 0.000000000000000000, -1.000000000000000000, 0.000000000000000000 ) ) ;
#3674=ORIENTED_EDGE ( 'NONE', *, *, #11614, .T. ) ;
#3675=ORIENTED_EDGE ( 'NONE', *, *, #4659, .F. ) ;
#3678=DIRECTION ( 'NONE',  ( 0.000000000000000000, 1.000000000000000000, -0.000000000000000000 ) ) ;
#3681=ORIENTED_EDGE ( 'NONE', *, *, #33800, .F. ) ;
#3682=VECTOR ( 'NONE', #30122, 1000.000000000000000 ) ;
#3685=AXIS2_PLACEMENT_3D ( 'NONE', #39846, #426, #43801 ) ;
#3686=EDGE_CURVE ( 'NONE', #1781, #2708, #38422, .T. ) ;
#3687=ORIENTED_EDGE ( 'NONE', *, *, #7290, .F. ) ;
#3688=VERTEX_POINT ( 'NONE', #16803 ) ;
#3689=VERTEX_POINT ( 'NONE', #32809 ) ;
#3690=LINE ( 'NONE', #19718, #7417 ) ;
#3691=ADVANCED_FACE ( 'NONE', ( #13097 ), #33066, .T. ) ;
#3692=VECTOR ( 'NONE', #36741, 999.9999999999998863 ) ;
#3694=EDGE_CURVE ( 'NONE', #44232, #19435, #24140, .T. ) ;
#3695=EDGE_CURVE ( 'NONE', #34352, #1095, #14921, .T. ) ;
#3696=DIRECTION ( 'NONE',  ( 0.000000000000000000, 0.000000000000000000, 1.000000000000000000 ) ) ;
#3697=DIRECTION ( 'NONE',  ( 0.000000000000000000, 0.000000000000000000, -1.000000000000000000 ) ) ;
#3698=FACE_OUTER_BOUND ( 'NONE', #20305, .T. ) ;
#3700=ORIENTED_EDGE ( 'NONE', *, *, #38529, .T. ) ;
#3701=ADVANCED_FACE ( 'NONE', ( #29637 ), #6253, .T. ) ;
#3704=VERTEX_POINT ( 'NONE', #33845 ) ;
#3705=CARTESIAN_POINT ( 'NONE',  ( -48.98765787015808115, -193.5000000000000000, 0.8610436117673582190 ) ) ;
#3706=VERTEX_POINT ( 'NONE', #38038 ) ;
#3708=DIRECTION ( 'NONE',  ( 0.5338233779647826305, 0.000000000000000000, 0.8455960035018311727 ) ) ;
#3710=DIRECTION ( 'NONE',  ( 0.000000000000000000, 0.000000000000000000, 1.000000000000000000 ) ) ;
#3713=CARTESIAN_POINT ( 'NONE',  ( -12.13476221271688615, -175.3837268820161057, 119.5996955107804638 ) ) ;
#3714=CARTESIAN_POINT ( 'NONE',  ( 0.000000000000000000, 0.000000000000000000, 0.000000000000000000 ) ) ;
#3715=ORIENTED_EDGE ( 'NONE', *, *, #33903, .F. ) ;
#3719=CARTESIAN_POINT ( 'NONE',  ( -41.90263914168912152, -189.7472609257535510, -124.8268793598473536 ) ) ;
#3721=ORIENTED_EDGE ( 'NONE', *, *, #970, .T. ) ;
#3722=LINE ( 'NONE', #47634, #21732 ) ;
#3723=DIRECTION ( 'NONE',  ( -0.08879589532293158394, 0.000000000000000000, -0.9960498426152172291 ) ) ;
#3724=AXIS2_PLACEMENT_3D ( 'NONE', #33735, #41100, #24813 ) ;
#3725=ORIENTED_EDGE ( 'NONE', *, *, #47380, .F. ) ;
#3726=PLANE ( 'NONE',  #21571 ) ;
#3730=DIRECTION ( 'NONE',  ( 0.000000000000000000, -0.000000000000000000, -1.000000000000000000 ) ) ;
#3731=DIRECTION ( 'NONE',  ( -0.000000000000000000, 1.000000000000000000, -0.000000000000000000 ) ) ;
#3732=CARTESIAN_POINT ( 'NONE',  ( -168.8371699641976420, -193.5000000000000000, 33.74820638215509661 ) ) ;
#3733=CIRCLE ( 'NONE', #51577, 125.0000000000000000 ) ;
#3734=DIRECTION ( 'NONE',  ( 0.000000000000000000, 1.000000000000000000, 0.000000000000000000 ) ) ;
#3736=CARTESIAN_POINT ( 'NONE',  ( -128.7986236165182561, -189.7472609257535510, 94.47107458416955694 ) ) ;
#3737=DIRECTION ( 'NONE',  ( 0.000000000000000000, -1.000000000000000000, 0.000000000000000000 ) ) ;
#3742=EDGE_CURVE ( 'NONE', #45844, #6703, #45430, .T. ) ;
#3749=ORIENTED_EDGE ( 'NONE', *, *, #43872, .T. ) ;
#3751=PLANE ( 'NONE',  #37614 ) ;
#3752=ADVANCED_FACE ( 'NONE', ( #13364 ), #21251, .T. ) ;
#3753=VECTOR ( 'NONE', #41517, 999.9999999999998863 ) ;
#3754=AXIS2_PLACEMENT_3D ( 'NONE', #27662, #51580, #11636 ) ;
#3755=ADVANCED_FACE ( 'NONE', ( #38297 ), #41984, .T. ) ;
#3756=LINE ( 'NONE', #19785, #16895 ) ;
#3758=ORIENTED_EDGE ( 'NONE', *, *, #11765, .T. ) ;
#3759=VERTEX_POINT ( 'NONE', #45958 ) ;
#3760=CIRCLE ( 'NONE', #417, 125.0000000000000000 ) ;
#3761=ADVANCED_FACE ( 'NONE', ( #37535 ), #5490, .F. ) ;
#3762=ORIENTED_EDGE ( 'NONE', *, *, #47933, .F. ) ;
#3767=AXIS2_PLACEMENT_3D ( 'NONE', #11777, #44892, #8883 ) ;
#3768=CARTESIAN_POINT ( 'NONE',  ( -80.85382946868867293, -183.6283474603465606, 119.6996507684852702 ) ) ;
#3769=CIRCLE ( 'NONE', #24782, 125.0000000000000000 ) ;
#3770=DIRECTION ( 'NONE',  ( -0.000000000000000000, 0.000000000000000000, 1.000000000000000000 ) ) ;
#3771=ORIENTED_EDGE ( 'NONE', *, *, #29189, .F. ) ;
#3772=FACE_OUTER_BOUND ( 'NONE', #41187, .T. ) ;
#3775=AXIS2_PLACEMENT_3D ( 'NONE', #37382, #48963, #33462 ) ;
#3779=EDGE_LOOP ( 'NONE', ( #28599, #10335, #2234, #9123 ) ) ;
#3780=ORIENTED_EDGE ( 'NONE', *, *, #51858, .F. ) ;
#3781=DIRECTION ( 'NONE',  ( 0.000000000000000000, 0.000000000000000000, -1.000000000000000000 ) ) ;
#3783=ORIENTED_EDGE ( 'NONE', *, *, #24230, .F. ) ;
#3789=ADVANCED_FACE ( 'NONE', ( #9945 ), #14152, .T. ) ;
#3791=CARTESIAN_POINT ( 'NONE',  ( 41.00573479224733120, -193.5000000000000000, -87.27805883780175122 ) ) ;
#3792=LINE ( 'NONE', #27450, #43895 ) ;
#3793=FACE_BOUND ( 'NONE', #51894, .T. ) ;
#3796=EDGE_LOOP ( 'NONE', ( #30914, #37786, #31611, #20331 ) ) ;
#3797=VECTOR ( 'NONE', #47550, 1000.000000000000000 ) ;
#3798=AXIS2_PLACEMENT_3D ( 'NONE', #34752, #15073, #47642 ) ;
#3799=CARTESIAN_POINT ( 'NONE',  ( -104.9497554727471851, -189.7472609257535510, -110.3950557015149059 ) ) ;
#3800=DIRECTION ( 'NONE',  ( 0.000000000000000000, 1.000000000000000000, 0.000000000000000000 ) ) ;
#3801=CARTESIAN_POINT ( 'NONE',  ( -48.47912675150885065, -188.5000000000000284, 6.938893903907228378E-15 ) ) ;
#3803=CIRCLE ( 'NONE', #1292, 125.0000000000000000 ) ;
#3805=DIRECTION ( 'NONE',  ( 0.9785564922995046988, 0.000000000000000000, -0.2059786187410953262 ) ) ;
#3806=ORIENTED_EDGE ( 'NONE', *, *, #6979, .T. ) ;
#3807=EDGE_CURVE ( 'NONE', #40896, #36109, #23352, .T. ) ;
#3808=EDGE_LOOP ( 'NONE', ( #16865, #1142, #41787, #25674 ) ) ;
#3809=AXIS2_PLACEMENT_3D ( 'NONE', #15432, #47479, #11463 ) ;
#3810=LINE ( 'NONE', #31669, #46183 ) ;
#3811=LINE ( 'NONE', #11172, #19423 ) ;
#3815=EDGE_CURVE ( 'NONE', #30848, #16149, #10739, .T. ) ;
#3817=EDGE_CURVE ( 'NONE', #38590, #27501, #47241, .T. ) ;
#3819=ADVANCED_FACE ( 'NONE', ( #3077 ), #11214, .T. ) ;
#3820=VECTOR ( 'NONE', #31240, 1000.000000000000000 ) ;
#3822=VECTOR ( 'NONE', #15616, 1000.000000000000000 ) ;
#3823=CARTESIAN_POINT ( 'NONE',  ( 56.77503207194100554, -189.7472609257535510, -67.42819922234311036 ) ) ;
#3824=ORIENTED_EDGE ( 'NONE', *, *, #29102, .T. ) ;
#3825=CARTESIAN_POINT ( 'NONE',  ( -34.51936650669028239, -193.5000000000000000, -124.2180546213278092 ) ) ;
#3829=DIRECTION ( 'NONE',  ( 0.000000000000000000, 1.000000000000000000, 0.000000000000000000 ) ) ;
#3830=DIRECTION ( 'NONE',  ( -0.8896570909947467687, 0.000000000000000000, -0.4566292373937140270 ) ) ;
#3831=EDGE_CURVE ( 'NONE', #30477, #33788, #6524, .T. ) ;
#3833=CYLINDRICAL_SURFACE ( 'NONE', #50092, 125.0000000000000000 ) ;
#3835=EDGE_LOOP ( 'NONE', ( #49525, #43121, #26532, #32502 ) ) ;
#3836=EDGE_CURVE ( 'NONE', #40857, #26725, #46717, .T. ) ;
#3837=VERTEX_POINT ( 'NONE', #19120 ) ;
#3838=DIRECTION ( 'NONE',  ( 0.000000000000000000, 1.000000000000000000, 0.000000000000000000 ) ) ;
#3840=AXIS2_PLACEMENT_3D ( 'NONE', #16280, #31799, #36491 ) ;
#3841=ADVANCED_FACE ( 'NONE', ( #6775 ), #3590, .T. ) ;
#3842=CARTESIAN_POINT ( 'NONE',  ( 75.95066919219054569, -175.3837268820161057, -11.92584929509534852 ) ) ;
#3845=DIRECTION ( 'NONE',  ( 0.000000000000000000, 1.000000000000000000, 0.000000000000000000 ) ) ;
#3846=ORIENTED_EDGE ( 'NONE', *, *, #19059, .T. ) ;
#3848=EDGE_CURVE ( 'NONE', #794, #14931, #34610, .T. ) ;
#3849=EDGE_CURVE ( 'NONE', #49882, #20620, #50223, .T. ) ;
#3851=ORIENTED_EDGE ( 'NONE', *, *, #8610, .F. ) ;
#3852=CARTESIAN_POINT ( 'NONE',  ( -152.3176060415594861, -193.5000000000000000, -69.58857822034967455 ) ) ;
#3853=ORIENTED_EDGE ( 'NONE', *, *, #33442, .T. ) ;
#3854=VERTEX_POINT ( 'NONE', #46983 ) ;
#3856=AXIS2_PLACEMENT_3D ( 'NONE', #21699, #49302, #935 ) ;
#3858=AXIS2_PLACEMENT_3D ( 'NONE', #27969, #15906, #43496 ) ;
#3859=DIRECTION ( 'NONE',  ( 0.000000000000000000, 0.000000000000000000, 1.000000000000000000 ) ) ;
#3860=CARTESIAN_POINT ( 'NONE',  ( -108.5723883981724640, -183.6283474603465606, 109.6074810615846076 ) ) ;
#3863=VECTOR ( 'NONE', #4430, 1000.000000000000000 ) ;
#3864=ORIENTED_EDGE ( 'NONE', *, *, #31105, .F. ) ;
#3866=AXIS2_PLACEMENT_3D ( 'NONE', #18798, #28583, #26398 ) ;
#3867=ORIENTED_EDGE ( 'NONE', *, *, #25349, .T. ) ;
#3868=LINE ( 'NONE', #31968, #7780 ) ;
#3869=LINE ( 'NONE', #36422, #39936 ) ;
#3870=CARTESIAN_POINT ( 'NONE',  ( -92.78132261338707565, -189.7472609257535510, -116.8859077982276773 ) ) ;
#3871=CARTESIAN_POINT ( 'NONE',  ( 74.03660210627325000, -175.3837268820161057, -19.12855698118388048 ) ) ;
#3872=CARTESIAN_POINT ( 'NONE',  ( 70.91428087927182844, -175.3837268820161057, -33.48461921608517855 ) ) ;
#3873=ORIENTED_EDGE ( 'NONE', *, *, #38240, .T. ) ;
#3876=FACE_BOUND ( 'NONE', #49373, .T. ) ;
#3878=CIRCLE ( 'NONE', #18212, 125.0000000000000000 ) ;
#3881=AXIS2_PLACEMENT_3D ( 'NONE', #35987, #23884, #31252 ) ;
#3886=ADVANCED_FACE ( 'NONE', ( #15441 ), #31445, .T. ) ;
#3887=CARTESIAN_POINT ( 'NONE',  ( -136.1415351158078408, -189.7472609257535510, -89.10837311819175000 ) ) ;
#3888=VERTEX_POINT ( 'NONE', #46460 ) ;
#3890=FACE_BOUND ( 'NONE', #1247, .T. ) ;
#3892=DIRECTION ( 'NONE',  ( 0.000000000000000000, -0.000000000000000000, 1.000000000000000000 ) ) ;
#3893=EDGE_LOOP ( 'NONE', ( #21888, #46622, #33513, #1785 ) ) ;
#3896=AXIS2_PLACEMENT_3D ( 'NONE', #6064, #22081, #46022 ) ;
#3898=ORIENTED_EDGE ( 'NONE', *, *, #36868, .T. ) ;
#3900=CIRCLE ( 'NONE', #17352, 125.0000000000000000 ) ;
#3901=DIRECTION ( 'NONE',  ( -0.000000000000000000, 1.000000000000000000, -0.000000000000000000 ) ) ;
#3905=DIRECTION ( 'NONE',  ( -0.9842305779475967187, 0.000000000000000000, -0.1768902751225733538 ) ) ;
#3906=EDGE_CURVE ( 'NONE', #9933, #12964, #35083, .T. ) ;
#3908=DIRECTION ( 'NONE',  ( 0.9890401873221623674, 0.000000000000000000, 0.1476465640024917925 ) ) ;
#3909=ORIENTED_EDGE ( 'NONE', *, *, #33659, .T. ) ;
#3910=LINE ( 'NONE', #35966, #19985 ) ;
#3911=LINE ( 'NONE', #8370, #28936 ) ;
#3914=EDGE_LOOP ( 'NONE', ( #31853, #31954, #5133, #18373 ) ) ;
#3915=AXIS2_PLACEMENT_3D ( 'NONE', #3732, #45000, #16098 ) ;
#3916=DIRECTION ( 'NONE',  ( 0.9960498426152171181, 0.000000000000000000, -0.08879589532293157006 ) ) ;
#3920=CIRCLE ( 'NONE', #1403, 125.0000000000000000 ) ;
#3921=DIRECTION ( 'NONE',  ( 0.000000000000000000, -1.000000000000000000, 0.000000000000000000 ) ) ;
#3922=EDGE_LOOP ( 'NONE', ( #22340, #34109, #41447, #45541 ) ) ;
#3926=ORIENTED_EDGE ( 'NONE', *, *, #2947, .F. ) ;
#3928=VECTOR ( 'NONE', #36672, 1000.000000000000000 ) ;
#3930=AXIS2_PLACEMENT_3D ( 'NONE', #20465, #23629, #12584 ) ;
#3931=CARTESIAN_POINT ( 'NONE',  ( 48.06131630543706734, -189.7472609257535510, -79.40367028273054473 ) ) ;
#3934=VECTOR ( 'NONE', #20581, 1000.000000000000000 ) ;
#3935=VECTOR ( 'NONE', #12702, 1000.000000000000114 ) ;
#3937=VERTEX_POINT ( 'NONE', #31965 ) ;
#3940=CARTESIAN_POINT ( 'NONE',  ( 75.17589904515342880, -193.5000000000000000, -18.28755301364250130 ) ) ;
#3943=DIRECTION ( 'NONE',  ( 0.000000000000000000, 0.000000000000000000, -1.000000000000000000 ) ) ;
#3944=ORIENTED_EDGE ( 'NONE', *, *, #46560, .F. ) ;
#3945=PLANE ( 'NONE',  #30724 ) ;
#3946=CARTESIAN_POINT ( 'NONE',  ( -117.8923552450418697, -193.5000000000000000, 102.7511748916629699 ) ) ;
#3948=ORIENTED_EDGE ( 'NONE', *, *, #47365, .T. ) ;
#3950=ORIENTED_EDGE ( 'NONE', *, *, #13011, .T. ) ;
#3953=CARTESIAN_POINT ( 'NONE',  ( 14.37129481273059106, -193.5000000000000000, -108.0501018472328241 ) ) ;
#3956=DIRECTION ( 'NONE',  ( 0.000000000000000000, -0.000000000000000000, -1.000000000000000000 ) ) ;
#3957=AXIS2_PLACEMENT_3D ( 'NONE', #27496, #39326, #47231 ) ;
#3961=ORIENTED_EDGE ( 'NONE', *, *, #21032, .F. ) ;
#3963=ORIENTED_EDGE ( 'NONE', *, *, #44529, .F. ) ;
#3965=DIRECTION ( 'NONE',  ( -0.000000000000000000, 1.000000000000000000, -0.000000000000000000 ) ) ;
#3966=VECTOR ( 'NONE', #42362, 1000.000000000000227 ) ;
#3968=VERTEX_POINT ( 'NONE', #48543 ) ;
#3970=FACE_OUTER_BOUND ( 'NONE', #28921, .T. ) ;
#3971=CARTESIAN_POINT ( 'NONE',  ( -47.49008656418669005, -193.5000000000000000, -0.1476465640024710591 ) ) ;
#3972=CARTESIAN_POINT ( 'NONE',  ( 61.38599058177057799, -193.5000000000000000, 59.62093586438192006 ) ) ;
#3975=DIRECTION ( 'NONE',  ( -0.000000000000000000, 1.000000000000000000, -0.000000000000000000 ) ) ;
#3976=VERTEX_POINT ( 'NONE', #36167 ) ;
#3977=CARTESIAN_POINT ( 'NONE',  ( -15.81236726369125023, -177.1207230881787780, -120.6560517527615417 ) ) ;
#3978=ORIENTED_EDGE ( 'NONE', *, *, #20019, .T. ) ;
#3980=EDGE_CURVE ( 'NONE', #26956, #24349, #40970, .T. ) ;
#3983=CARTESIAN_POINT ( 'NONE',  ( 72.82672500347334221, -189.7472609257535510, 25.70779184431859221 ) ) ;
#3984=ORIENTED_EDGE ( 'NONE', *, *, #46384, .F. ) ;
#3988=AXIS2_PLACEMENT_3D ( 'NONE', #46783, #19421, #3142 ) ;
#3989=CARTESIAN_POINT ( 'NONE',  ( -48.47912675150885065, -177.1207230881787780, 6.938893903907228378E-15 ) ) ;
#3990=EDGE_LOOP ( 'NONE', ( #1850, #328, #47951, #29352 ) ) ;
#3991=LINE ( 'NONE', #8190, #4806 ) ;
#3992=DIRECTION ( 'NONE',  ( 0.000000000000000000, 1.000000000000000000, -0.000000000000000000 ) ) ;
#3994=DIRECTION ( 'NONE',  ( 0.000000000000000000, -0.000000000000000000, 1.000000000000000000 ) ) ;
#3995=EDGE_CURVE ( 'NONE', #3221, #47296, #9097, .T. ) ;
#3996=VERTEX_POINT ( 'NONE', #48788 ) ;
#3997=DIRECTION ( 'NONE',  ( 0.000000000000000000, 1.000000000000000000, -0.000000000000000000 ) ) ;
#3999=EDGE_CURVE ( 'NONE', #2485, #25619, #44327, .T. ) ;
#4000=ORIENTED_EDGE ( 'NONE', *, *, #8294, .T. ) ;
#4006=CARTESIAN_POINT ( 'NONE',  ( 7.991501969728815880, -189.7472609257535510, 110.3950557015152611 ) ) ;
#4008=DIRECTION ( 'NONE',  ( 0.000000000000000000, 0.000000000000000000, -1.000000000000000000 ) ) ;
#4011=EDGE_CURVE ( 'NONE', #19237, #2758, #11984, .T. ) ;
#4012=AXIS2_PLACEMENT_3D ( 'NONE', #15781, #27822, #32560 ) ;
#4014=DIRECTION ( 'NONE',  ( 0.000000000000000000, 0.000000000000000000, -1.000000000000000000 ) ) ;
#4016=EDGE_CURVE ( 'NONE', #41557, #3584, #8058, .T. ) ;
#4017=CYLINDRICAL_SURFACE ( 'NONE', #126, 125.0000000000000000 ) ;
#4018=CARTESIAN_POINT ( 'NONE',  ( -124.1938582159088327, -193.5000000000000000, -99.45993886622791536 ) ) ;
#4020=EDGE_LOOP ( 'NONE', ( #24596, #9949, #28125, #19542 ) ) ;
#4021=ORIENTED_EDGE ( 'NONE', *, *, #2650, .F. ) ;
#4022=CARTESIAN_POINT ( 'NONE',  ( -49.42645310536304493, -177.1207230881787780, 0.3202698538628349079 ) ) ;
#4023=DIRECTION ( 'NONE',  ( -0.000000000000000000, 1.000000000000000000, -0.000000000000000000 ) ) ;
#4025=VECTOR ( 'NONE', #38998, 1000.000000000000227 ) ;
#4026=VECTOR ( 'NONE', #33269, 1000.000000000000000 ) ;
#4030=DIRECTION ( 'NONE',  ( 0.000000000000000000, -1.000000000000000000, 0.000000000000000000 ) ) ;
#4031=LINE ( 'NONE', #23985, #10742 ) ;
#4032=AXIS2_PLACEMENT_3D ( 'NONE', #15098, #35052, #26894 ) ;
#4033=FACE_OUTER_BOUND ( 'NONE', #29892, .T. ) ;
#4035=EDGE_LOOP ( 'NONE', ( #36750, #17969, #34335, #27032 ) ) ;
#4037=ORIENTED_EDGE ( 'NONE', *, *, #40112, .F. ) ;
#4039=DIRECTION ( 'NONE',  ( -0.08879589532294572540, 0.000000000000000000, 0.9960498426152160079 ) ) ;
#4041=DIRECTION ( 'NONE',  ( 0.000000000000000000, 0.000000000000000000, 1.000000000000000000 ) ) ;
#4045=DIRECTION ( 'NONE',  ( -0.5586467658036535777, 0.000000000000000000, 0.8294056854502011022 ) ) ;
#4048=LINE ( 'NONE', #35835, #19019 ) ;
#4050=ORIENTED_EDGE ( 'NONE', *, *, #33519, .F. ) ;
#4051=VERTEX_POINT ( 'NONE', #44838 ) ;
#4052=ORIENTED_EDGE ( 'NONE', *, *, #3467, .T. ) ;
#4054=LINE ( 'NONE', #23505, #4865 ) ;
#4055=VERTEX_POINT ( 'NONE', #32222 ) ;
#4059=EDGE_CURVE ( 'NONE', #39414, #30881, #24346, .T. ) ;
#4060=FACE_OUTER_BOUND ( 'NONE', #45746, .T. ) ;
#4061=EDGE_LOOP ( 'NONE', ( #35971, #44863, #7815, #34052 ) ) ;
#4062=DIRECTION ( 'NONE',  ( -0.000000000000000000, -1.000000000000000000, 0.000000000000000000 ) ) ;
#4063=ORIENTED_EDGE ( 'NONE', *, *, #51076, .T. ) ;
#4065=ORIENTED_EDGE ( 'NONE', *, *, #30121, .T. ) ;
#4066=DIRECTION ( 'NONE',  ( -0.000000000000000000, 1.000000000000000000, -0.000000000000000000 ) ) ;
#4067=FACE_BOUND ( 'NONE', #49442, .T. ) ;
#4068=VECTOR ( 'NONE', #47425, 1000.000000000000000 ) ;
#4069=AXIS2_PLACEMENT_3D ( 'NONE', #17936, #13996, #48249 ) ;
#4070=DIRECTION ( 'NONE',  ( -0.6528221181905174975, 0.000000000000000000, -0.7575112421616236880 ) ) ;
#4071=ORIENTED_EDGE ( 'NONE', *, *, #40206, .F. ) ;
#4074=DIRECTION ( 'NONE',  ( 0.000000000000000000, 1.000000000000000000, 0.000000000000000000 ) ) ;
#4075=CARTESIAN_POINT ( 'NONE',  ( 46.31065297101394407, -183.6283474603465606, 79.94433946042836681 ) ) ;
#4076=EDGE_CURVE ( 'NONE', #503, #28684, #12760, .T. ) ;
#4077=CARTESIAN_POINT ( 'NONE',  ( -158.6498865914718124, -193.5000000000000000, 56.90809649257574421 ) ) ;
#4082=VERTEX_POINT ( 'NONE', #415 ) ;
#4083=VECTOR ( 'NONE', #35684, 1000.000000000000000 ) ;
#4084=ADVANCED_FACE ( 'NONE', ( #697 ), #40882, .T. ) ;
#4086=LINE ( 'NONE', #40573, #5192 ) ;
#4087=ORIENTED_EDGE ( 'NONE', *, *, #5082, .F. ) ;
#4088=ADVANCED_FACE ( 'NONE', ( #32997 ), #37466, .T. ) ;
#4089=VERTEX_POINT ( 'NONE', #1473 ) ;
#4090=DIRECTION ( 'NONE',  ( 0.000000000000000000, 0.000000000000000000, -1.000000000000000000 ) ) ;
#4091=CIRCLE ( 'NONE', #1537, 125.0000000000000000 ) ;
#4095=CARTESIAN_POINT ( 'NONE',  ( 52.98246549829695340, -175.3837268820161057, 73.01058346660533971 ) ) ;
#4096=ORIENTED_EDGE ( 'NONE', *, *, #2705, .T. ) ;
#4097=DIRECTION ( 'NONE',  ( -0.000000000000000000, 1.000000000000000000, -0.000000000000000000 ) ) ;
#4098=CARTESIAN_POINT ( 'NONE',  ( 25.43954814678888710, -193.5000000000000000, 100.8019320314832754 ) ) ;
#4101=VERTEX_POINT ( 'NONE', #29576 ) ;
#4102=EDGE_LOOP ( 'NONE', ( #26664, #13919, #30502, #51583 ) ) ;
#4103=VERTEX_POINT ( 'NONE', #9106 ) ;
#4104=DIRECTION ( 'NONE',  ( 0.000000000000000000, -0.000000000000000000, -1.000000000000000000 ) ) ;
#4106=DIRECTION ( 'NONE',  ( 0.7175072570443348230, 0.000000000000000000, -0.6965510290629933765 ) ) ;
#4107=VECTOR ( 'NONE', #16339, 1000.000000000000000 ) ;
#4109=DIRECTION ( 'NONE',  ( -0.000000000000000000, 1.000000000000000000, -0.000000000000000000 ) ) ;
#4112=ORIENTED_EDGE ( 'NONE', *, *, #31050, .T. ) ;
#4113=CIRCLE ( 'NONE', #39325, 125.0000000000000000 ) ;
#4114=CARTESIAN_POINT ( 'NONE',  ( -48.47912675150885065, -189.7472609257535510, 6.938893903907228378E-15 ) ) ;
#4116=VERTEX_POINT ( 'NONE', #13027 ) ;
#4118=ORIENTED_EDGE ( 'NONE', *, *, #6032, .F. ) ;
#4120=ORIENTED_EDGE ( 'NONE', *, *, #16380, .T. ) ;
#4121=DIRECTION ( 'NONE',  ( 0.8757349421956412971, 0.000000000000000000, -0.4827922027307366970 ) ) ;
#4122=PLANE ( 'NONE',  #9860 ) ;
#4123=EDGE_CURVE ( 'NONE', #46209, #20432, #41149, .T. ) ;
#4125=EDGE_CURVE ( 'NONE', #25351, #1446, #51867, .T. ) ;
#4127=CARTESIAN_POINT ( 'NONE',  ( -48.47912675150885065, -189.7472609257535510, 6.938893903907228378E-15 ) ) ;
#4128=EDGE_LOOP ( 'NONE', ( #13411, #34901, #51105, #15440 ) ) ;
#4130=VERTEX_POINT ( 'NONE', #1726 ) ;
#4131=EDGE_CURVE ( 'NONE', #40700, #7086, #13554, .T. ) ;
#4134=CARTESIAN_POINT ( 'NONE',  ( -168.8371699641976420, -189.7472609257535510, 33.74820638215509661 ) ) ;
#4135=EDGE_CURVE ( 'NONE', #9572, #12713, #45116, .T. ) ;
#4137=CARTESIAN_POINT ( 'NONE',  ( -164.3791542526839180, -175.3837268820161057, 46.82076062204521349 ) ) ;
#4138=CARTESIAN_POINT ( 'NONE',  ( 53.56330073376472001, -175.3837268820161057, 72.19655804062048787 ) ) ;
#4139=DIRECTION ( 'NONE',  ( -0.000000000000000000, 1.000000000000000000, -0.000000000000000000 ) ) ;
#4140=EDGE_CURVE ( 'NONE', #44024, #33166, #5422, .T. ) ;
#4144=EDGE_CURVE ( 'NONE', #47580, #36397, #25388, .T. ) ;
#4145=FACE_BOUND ( 'NONE', #15335, .T. ) ;
#4149=LINE ( 'NONE', #16226, #2117 ) ;
#4152=EDGE_CURVE ( 'NONE', #35261, #2420, #17522, .T. ) ;
#4153=VERTEX_POINT ( 'NONE', #33783 ) ;
#4154=FACE_OUTER_BOUND ( 'NONE', #11429, .T. ) ;
#4155=VERTEX_POINT ( 'NONE', #29835 ) ;
#4156=EDGE_CURVE ( 'NONE', #20290, #11975, #8220, .T. ) ;
#4157=PLANE ( 'NONE',  #7515 ) ;
#4158=FACE_BOUND ( 'NONE', #36801, .T. ) ;
#4160=ORIENTED_EDGE ( 'NONE', *, *, #25675, .F. ) ;
#4162=EDGE_CURVE ( 'NONE', #35348, #16442, #29266, .T. ) ;
#4164=AXIS2_PLACEMENT_3D ( 'NONE', #28924, #33420, #27957 ) ;
#4165=ORIENTED_EDGE ( 'NONE', *, *, #25943, .T. ) ;
#4166=CARTESIAN_POINT ( 'NONE',  ( -121.5885020763900997, -177.1207230881787780, -101.3904297239420913 ) ) ;
#4171=CARTESIAN_POINT ( 'NONE',  ( 64.72501964220592185, -189.7472609257535510, 53.00774697410174952 ) ) ;
#4172=EDGE_LOOP ( 'NONE', ( #8707, #13728, #4050, #28756 ) ) ;
#4174=VERTEX_POINT ( 'NONE', #42174 ) ;
#4176=VECTOR ( 'NONE', #28040, 1000.000000000000114 ) ;
#4177=FACE_OUTER_BOUND ( 'NONE', #20003, .T. ) ;
#4178=ORIENTED_EDGE ( 'NONE', *, *, #8611, .F. ) ;
#4179=DIRECTION ( 'NONE',  ( 0.000000000000000000, -1.000000000000000000, -0.000000000000000000 ) ) ;
#4180=VERTEX_POINT ( 'NONE', #37979 ) ;
#4182=EDGE_CURVE ( 'NONE', #7899, #43082, #30102, .T. ) ;
#4183=CARTESIAN_POINT ( 'NONE',  ( 56.77503207194101265, -193.5000000000000000, -67.42819922234311036 ) ) ;
#4184=ORIENTED_EDGE ( 'NONE', *, *, #7927, .T. ) ;
#4185=DIRECTION ( 'NONE',  ( 0.000000000000000000, 0.000000000000000000, -1.000000000000000000 ) ) ;
#4187=ADVANCED_FACE ( 'NONE', ( #10131 ), #26146, .F. ) ;
#4189=ORIENTED_EDGE ( 'NONE', *, *, #3471, .T. ) ;
#4190=FACE_OUTER_BOUND ( 'NONE', #38485, .T. ) ;
#4191=DIRECTION ( 'NONE',  ( -0.000000000000000000, 1.000000000000000000, -0.000000000000000000 ) ) ;
#4196=ORIENTED_EDGE ( 'NONE', *, *, #1190, .T. ) ;
#4200=CIRCLE ( 'NONE', #24331, 125.0000000000000000 ) ;
#4201=AXIS2_PLACEMENT_3D ( 'NONE', #9570, #24820, #33994 ) ;
#4202=CARTESIAN_POINT ( 'NONE',  ( 55.35935253854128746, -177.1207230881787780, 69.58857822035042773 ) ) ;
#4203=VERTEX_POINT ( 'NONE', #2253 ) ;
#4204=FACE_OUTER_BOUND ( 'NONE', #35289, .T. ) ;
#4206=DIRECTION ( 'NONE',  ( -0.5085311186492094127, 0.000000000000000000, -0.8610436117673619938 ) ) ;
#4207=LINE ( 'NONE', #32300, #3119 ) ;
#4209=VERTEX_POINT ( 'NONE', #18790 ) ;
#4210=ORIENTED_EDGE ( 'NONE', *, *, #18447, .T. ) ;
#4211=EDGE_CURVE ( 'NONE', #17485, #20084, #3243, .T. ) ;
#4214=CARTESIAN_POINT ( 'NONE',  ( -45.06671089634842531, -183.6283474603465606, -124.9534129907280686 ) ) ;
#4215=DIRECTION ( 'NONE',  ( -0.000000000000000000, 1.000000000000000000, -0.000000000000000000 ) ) ;
#4217=ORIENTED_EDGE ( 'NONE', *, *, #38282, .T. ) ;
#4218=CARTESIAN_POINT ( 'NONE',  ( 43.18784210722336780, -189.7472609257535510, -84.98333260264752198 ) ) ;
#4219=VERTEX_POINT ( 'NONE', #14870 ) ;
#4220=ORIENTED_EDGE ( 'NONE', *, *, #48097, .F. ) ;
#4222=PLANE ( 'NONE',  #8261 ) ;
#4223=ADVANCED_FACE ( 'NONE', ( #30882 ), #6466, .T. ) ;
#4225=VECTOR ( 'NONE', #49225, 1000.000000000000114 ) ;
#4226=CIRCLE ( 'NONE', #19352, 125.0000000000000000 ) ;
#4229=CARTESIAN_POINT ( 'NONE',  ( 68.59638248015004081, -183.6283474603465606, -43.79868877201407429 ) ) ;
#4230=LINE ( 'NONE', #44437, #26660 ) ;
#4231=ORIENTED_EDGE ( 'NONE', *, *, #42962, .F. ) ;
#4232=DIRECTION ( 'NONE',  ( -0.1768902751225592818, 0.000000000000000000, -0.9842305779475992722 ) ) ;
#4233=VERTEX_POINT ( 'NONE', #34548 ) ;
#4234=DIRECTION ( 'NONE',  ( 0.5586467658036535777, 0.000000000000000000, -0.8294056854502011022 ) ) ;
#4235=ORIENTED_EDGE ( 'NONE', *, *, #15568, .T. ) ;
#4238=ADVANCED_FACE ( 'NONE', ( #23265 ), #50600, .T. ) ;
#4239=CARTESIAN_POINT ( 'NONE',  ( 22.03849146056077757, -175.3837268820161057, 103.2098131075567409 ) ) ;
#4241=DIRECTION ( 'NONE',  ( 0.000000000000000000, 0.000000000000000000, 1.000000000000000000 ) ) ;
#4243=CARTESIAN_POINT ( 'NONE',  ( -170.2790847791494855, -177.1207230881787780, -28.10285082451570915 ) ) ;
#4246=VERTEX_POINT ( 'NONE', #10907 ) ;
#4247=CARTESIAN_POINT ( 'NONE',  ( -160.2705093830644216, -183.6283474603465606, -55.92572546981520532 ) ) ;
#4249=CARTESIAN_POINT ( 'NONE',  ( 60.19403481868999961, -189.7472609257535510, -59.71720175837096178 ) ) ;
#4250=ORIENTED_EDGE ( 'NONE', *, *, #5910, .T. ) ;
#4251=DIRECTION ( 'NONE',  ( -0.000000000000000000, 0.000000000000000000, 1.000000000000000000 ) ) ;
#4253=EDGE_LOOP ( 'NONE', ( #2783, #29583, #4518, #10762 ) ) ;
#4254=LINE ( 'NONE', #24477, #11163 ) ;
#4256=DIRECTION ( 'NONE',  ( -0.000000000000000000, 1.000000000000000000, -0.000000000000000000 ) ) ;
#4257=CYLINDRICAL_SURFACE ( 'NONE', #15215, 124.9999999999999858 ) ;
#4258=EDGE_CURVE ( 'NONE', #993, #30377, #22493, .T. ) ;
#4259=AXIS2_PLACEMENT_3D ( 'NONE', #33486, #1933, #41604 ) ;
#4260=CARTESIAN_POINT ( 'NONE',  ( -169.0136227435421006, -189.7472609257535510, -33.11246405730813080 ) ) ;
#4261=DIRECTION ( 'NONE',  ( -0.000000000000000000, 1.000000000000000000, -0.000000000000000000 ) ) ;
#4264=CIRCLE ( 'NONE', #16881, 125.0000000000000000 ) ;
#4265=CARTESIAN_POINT ( 'NONE',  ( -49.44376233341720450, -183.6283474603465606, -0.2635871660690713436 ) ) ;
#4266=LINE ( 'NONE', #51579, #29502 ) ;
#4268=DIRECTION ( 'NONE',  ( 0.000000000000000000, -0.000000000000000000, -1.000000000000000000 ) ) ;
#4270=DIRECTION ( 'NONE',  ( 0.000000000000000000, 1.000000000000000000, 0.000000000000000000 ) ) ;
#4271=EDGE_CURVE ( 'NONE', #1934, #26319, #31786, .T. ) ;
#4272=CARTESIAN_POINT ( 'NONE',  ( -157.1522883217072604, -193.5000000000000000, 59.71720175837172206 ) ) ;
#4274=ORIENTED_EDGE ( 'NONE', *, *, #29167, .T. ) ;
#4275=VECTOR ( 'NONE', #14574, 1000.000000000000000 ) ;
#4276=EDGE_LOOP ( 'NONE', ( #30527, #32688, #9706, #20593 ) ) ;
#4277=DIRECTION ( 'NONE',  ( -0.7378332790417239107, 0.000000000000000000, -0.6749830015182142207 ) ) ;
#4279=CARTESIAN_POINT ( 'NONE',  ( -121.0298553105864556, -193.5000000000000000, -100.5610240384918939 ) ) ;
#4280=ORIENTED_EDGE ( 'NONE', *, *, #32049, .F. ) ;
#4282=ORIENTED_EDGE ( 'NONE', *, *, #3518, .F. ) ;
#4283=EDGE_CURVE ( 'NONE', #49807, #47473, #42662, .T. ) ;
#4284=CARTESIAN_POINT ( 'NONE',  ( -40.96347969518279086, -189.7472609257535510, -123.7720294769269174 ) ) ;
#4285=DIRECTION ( 'NONE',  ( 0.000000000000000000, -0.000000000000000000, -1.000000000000000000 ) ) ;
#4288=DIRECTION ( 'NONE',  ( -0.05924062789370748011, 0.000000000000000000, -0.9982437317643217956 ) ) ;
#4289=CARTESIAN_POINT ( 'NONE',  ( -48.47912675150885065, -175.3837268820161057, 6.938893903907228378E-15 ) ) ;
#4290=ORIENTED_EDGE ( 'NONE', *, *, #38831, .T. ) ;
#4291=CARTESIAN_POINT ( 'NONE',  ( 67.66641500972446011, -189.7472609257535510, 46.20836643931067300 ) ) ;
#4292=AXIS2_PLACEMENT_3D ( 'NONE', #5312, #21599, #1626 ) ;
#4293=EDGE_CURVE ( 'NONE', #16129, #47736, #15852, .T. ) ;
#4294=DIRECTION ( 'NONE',  ( -0.000000000000000000, 1.000000000000000000, -0.000000000000000000 ) ) ;
#4296=DIRECTION ( 'NONE',  ( 0.000000000000000000, 0.000000000000000000, -1.000000000000000000 ) ) ;
#4297=LINE ( 'NONE', #16133, #40837 ) ;
#4298=AXIS2_PLACEMENT_3D ( 'NONE', #43565, #51211, #27263 ) ;
#4299=ORIENTED_EDGE ( 'NONE', *, *, #11765, .F. ) ;
#4301=ADVANCED_FACE ( 'NONE', ( #39279 ), #39003, .F. ) ;
#4302=VERTEX_POINT ( 'NONE', #30351 ) ;
#4304=CARTESIAN_POINT ( 'NONE',  ( -49.46816693883101124, -177.1207230881787780, -0.1476465640024848536 ) ) ;
#4306=ORIENTED_EDGE ( 'NONE', *, *, #48812, .F. ) ;
#4307=FACE_OUTER_BOUND ( 'NONE', #5428, .T. ) ;
#4308=DIRECTION ( 'NONE',  ( 0.000000000000000000, 1.000000000000000000, 0.000000000000000000 ) ) ;
#4309=ORIENTED_EDGE ( 'NONE', *, *, #11179, .T. ) ;
#4310=CARTESIAN_POINT ( 'NONE',  ( -135.6699833737243353, -193.5000000000000000, 89.56983042009326823 ) ) ;
#4311=ORIENTED_EDGE ( 'NONE', *, *, #15775, .T. ) ;
#4312=LINE ( 'NONE', #29263, #26578 ) ;
#4313=VERTEX_POINT ( 'NONE', #51383 ) ;
#4314=CARTESIAN_POINT ( 'NONE',  ( -33.52607327456453845, -175.3837268820161057, -124.1024020384603261 ) ) ;
#4315=FACE_BOUND ( 'NONE', #34583, .T. ) ;
#4316=VECTOR ( 'NONE', #40787, 1000.000000000000114 ) ;
#4317=CARTESIAN_POINT ( 'NONE',  ( -238.7407812814481076, -193.5000000000000000, -41.45482488023466061 ) ) ;
#4318=EDGE_CURVE ( 'NONE', #44107, #25533, #15374, .T. ) ;
#4322=DIRECTION ( 'NONE',  ( 0.000000000000000000, 0.000000000000000000, 1.000000000000000000 ) ) ;
#4323=CARTESIAN_POINT ( 'NONE',  ( -48.47912675150885065, -175.3837268820161057, 6.938893903907228378E-15 ) ) ;
#4324=VERTEX_POINT ( 'NONE', #27446 ) ;
#4325=DIRECTION ( 'NONE',  ( -0.1182731709213730997, 0.000000000000000000, 0.9929810960135161402 ) ) ;
#4326=EDGE_LOOP ( 'NONE', ( #15229, #15017, #23343, #38726 ) ) ;
#4327=ORIENTED_EDGE ( 'NONE', *, *, #7454, .F. ) ;
#4330=ORIENTED_EDGE ( 'NONE', *, *, #22980, .T. ) ;
#4332=EDGE_LOOP ( 'NONE', ( #33824, #856, #51355, #20098 ) ) ;
#4333=CARTESIAN_POINT ( 'NONE',  ( -95.18697522258266019, -193.5000000000000000, 115.9455772817713353 ) ) ;
#4334=VECTOR ( 'NONE', #36421, 1000.000000000000114 ) ;
#4335=AXIS2_PLACEMENT_3D ( 'NONE', #28942, #8996, #25032 ) ;
#4337=VERTEX_POINT ( 'NONE', #7492 ) ;
#4342=DIRECTION ( 'NONE',  ( 0.000000000000000000, -1.000000000000000000, -0.000000000000000000 ) ) ;
#4343=EDGE_CURVE ( 'NONE', #23051, #42721, #23511, .T. ) ;
#4346=CARTESIAN_POINT ( 'NONE',  ( -22.44626007086657182, -193.5000000000000000, 122.2591094863196730 ) ) ;
#4348=CIRCLE ( 'NONE', #33722, 125.0000000000000000 ) ;
#4350=VERTEX_POINT ( 'NONE', #28725 ) ;
#4351=LINE ( 'NONE', #47737, #18226 ) ;
#4352=DIRECTION ( 'NONE',  ( -0.8124868780056742068, 0.000000000000000000, -0.5829794791144820021 ) ) ;
#4356=DIRECTION ( 'NONE',  ( -0.000000000000000000, 1.000000000000000000, -0.000000000000000000 ) ) ;
#4357=ORIENTED_EDGE ( 'NONE', *, *, #26907, .T. ) ;
#4358=EDGE_CURVE ( 'NONE', #15950, #4441, #47698, .T. ) ;
#4359=EDGE_CURVE ( 'NONE', #46675, #35017, #19181, .T. ) ;
#4360=VERTEX_POINT ( 'NONE', #44780 ) ;
#4361=CARTESIAN_POINT ( 'NONE',  ( 61.38599058177057799, -189.7472609257535510, 59.62093586438192006 ) ) ;
#4363=ORIENTED_EDGE ( 'NONE', *, *, #23692, .T. ) ;
#4364=EDGE_CURVE ( 'NONE', #28891, #6751, #28388, .T. ) ;
#4365=PLANE ( 'NONE',  #34189 ) ;
#4367=AXIS2_PLACEMENT_3D ( 'NONE', #35197, #34430, #11018 ) ;
#4374=AXIS2_PLACEMENT_3D ( 'NONE', #5002, #41231, #12340 ) ;
#4375=ORIENTED_EDGE ( 'NONE', *, *, #28128, .T. ) ;
#4376=CARTESIAN_POINT ( 'NONE',  ( -62.32061382540517513, -193.5000000000000000, 123.2250735253144285 ) ) ;
#4378=DIRECTION ( 'NONE',  ( 0.000000000000000000, -1.000000000000000000, -0.000000000000000000 ) ) ;
#4380=DIRECTION ( 'NONE',  ( -0.000000000000000000, 1.000000000000000000, -0.000000000000000000 ) ) ;
#4383=CARTESIAN_POINT ( 'NONE',  ( -83.89965873179625078, -175.3837268820161057, 118.8334608768482354 ) ) ;
#4384=LINE ( 'NONE', #41161, #21512 ) ;
#4388=FACE_BOUND ( 'NONE', #15368, .T. ) ;
#4391=VECTOR ( 'NONE', #43968, 1000.000000000000000 ) ;
#4395=CARTESIAN_POINT ( 'NONE',  ( -150.1390659022305840, -175.3837268820161057, 72.73415134496005408 ) ) ;
#4396=VERTEX_POINT ( 'NONE', #355 ) ;
#4398=FACE_BOUND ( 'NONE', #31223, .T. ) ;
#4399=PLANE ( 'NONE',  #39663 ) ;
#4400=ORIENTED_EDGE ( 'NONE', *, *, #49706, .T. ) ;
#4406=ORIENTED_EDGE ( 'NONE', *, *, #43041, .T. ) ;
#4410=CARTESIAN_POINT ( 'NONE',  ( -126.8597349762179931, -177.1207230881787780, -96.08646119223956816 ) ) ;
#4411=ORIENTED_EDGE ( 'NONE', *, *, #1619, .T. ) ;
#4412=EDGE_CURVE ( 'NONE', #15918, #28294, #35851, .T. ) ;
#4413=DIRECTION ( 'NONE',  ( -0.000000000000000000, 1.000000000000000000, -0.000000000000000000 ) ) ;
#4415=DIRECTION ( 'NONE',  ( 0.000000000000000000, -1.000000000000000000, 0.000000000000000000 ) ) ;
#4417=VECTOR ( 'NONE', #13847, 1000.000000000000000 ) ;
#4421=EDGE_CURVE ( 'NONE', #26319, #38573, #101, .T. ) ;
#4425=ORIENTED_EDGE ( 'NONE', *, *, #50692, .T. ) ;
#4426=VECTOR ( 'NONE', #13631, 1000.000000000000227 ) ;
#4427=VECTOR ( 'NONE', #10079, 1000.000000000000000 ) ;
#4430=DIRECTION ( 'NONE',  ( -0.000000000000000000, 1.000000000000000000, -0.000000000000000000 ) ) ;
#4432=CARTESIAN_POINT ( 'NONE',  ( 74.49773146996551532, -177.1207230881787780, -22.39848972532283256 ) ) ;
#4434=ADVANCED_FACE ( 'NONE', ( #36106 ), #16148, .F. ) ;
#4437=DIRECTION ( 'NONE',  ( -0.000000000000000000, 1.000000000000000000, -0.000000000000000000 ) ) ;
#4438=VERTEX_POINT ( 'NONE', #24537 ) ;
#4440=LINE ( 'NONE', #20457, #25005 ) ;
#4441=VERTEX_POINT ( 'NONE', #5626 ) ;
#4442=ORIENTED_EDGE ( 'NONE', *, *, #20036, .F. ) ;
#4444=CARTESIAN_POINT ( 'NONE',  ( -49.17567778057185990, -189.7472609257535510, 0.7175072570443320474 ) ) ;
#4445=DIRECTION ( 'NONE',  ( 0.000000000000000000, 0.000000000000000000, 1.000000000000000000 ) ) ;
#4447=CARTESIAN_POINT ( 'NONE',  ( -153.7332855749581881, -189.7472609257535510, 67.42819922234392038 ) ) ;
#4448=AXIS2_PLACEMENT_3D ( 'NONE', #41669, #2759, #13822 ) ;
#4451=LINE ( 'NONE', #11623, #39596 ) ;
#4453=EDGE_CURVE ( 'NONE', #30289, #36857, #49765, .T. ) ;
#4455=AXIS2_PLACEMENT_3D ( 'NONE', #23479, #35292, #34515 ) ;
#4458=PLANE ( 'NONE',  #25670 ) ;
#4459=CARTESIAN_POINT ( 'NONE',  ( -48.47912675150885065, -177.1207230881787780, 6.938893903907228378E-15 ) ) ;
#4460=CARTESIAN_POINT ( 'NONE',  ( -49.40581635894069024, -193.5000000000000000, 0.3758275821142362250 ) ) ;
#4461=ORIENTED_EDGE ( 'NONE', *, *, #32429, .T. ) ;
#4462=ORIENTED_EDGE ( 'NONE', *, *, #40585, .F. ) ;
#4463=AXIS2_PLACEMENT_3D ( 'NONE', #8652, #40436, #4989 ) ;
#4466=ADVANCED_FACE ( 'NONE', ( #40816 ), #37400, .T. ) ;
#4467=CARTESIAN_POINT ( 'NONE',  ( -14.28570516517293676, -193.5000000000000000, 120.2323164553486663 ) ) ;
#4469=CARTESIAN_POINT ( 'NONE',  ( -134.9506378406916554, -189.7472609257535510, 90.26448786734091811 ) ) ;
#4470=DIRECTION ( 'NONE',  ( 0.8455960035018272869, 0.000000000000000000, -0.5338233779647886257 ) ) ;
#4471=FACE_OUTER_BOUND ( 'NONE', #42996, .T. ) ;
#4473=EDGE_CURVE ( 'NONE', #14259, #19641, #9042, .T. ) ;
#4474=EDGE_CURVE ( 'NONE', #26506, #46675, #25841, .T. ) ;
#4478=CARTESIAN_POINT ( 'NONE',  ( 68.79964045138288498, -183.6283474603465606, 43.25148278810711844 ) ) ;
#4479=ADVANCED_FACE ( 'NONE', ( #5885 ), #4846, .F. ) ;
#4480=DIRECTION ( 'NONE',  ( -0.4566292373937018145, 0.000000000000000000, -0.8896570909947529859 ) ) ;
#4481=ORIENTED_EDGE ( 'NONE', *, *, #2986, .F. ) ;
#4484=CYLINDRICAL_SURFACE ( 'NONE', #20837, 124.9999999999999858 ) ;
#4485=VECTOR ( 'NONE', #13696, 1000.000000000000000 ) ;
#4487=CIRCLE ( 'NONE', #3652, 125.0000000000000000 ) ;
#4489=CARTESIAN_POINT ( 'NONE',  ( -47.74129347246713451, -189.7472609257535510, 0.6749830015182212151 ) ) ;
#4490=FACE_OUTER_BOUND ( 'NONE', #25109, .T. ) ;
#4491=CARTESIAN_POINT ( 'NONE',  ( -102.5006284722404502, -177.1207230881787780, -112.7238987608084386 ) ) ;
#4492=EDGE_LOOP ( 'NONE', ( #22196, #39135, #9926, #37270 ) ) ;
#4493=EDGE_CURVE ( 'NONE', #18044, #33603, #41596, .T. ) ;
#4494=CARTESIAN_POINT ( 'NONE',  ( 74.00867759460086859, -175.3837268820161057, 24.93467037017222410 ) ) ;
#4497=CARTESIAN_POINT ( 'NONE',  ( 49.88781503343062695, -193.5000000000000000, -75.49882471933871386 ) ) ;
#4500=FACE_OUTER_BOUND ( 'NONE', #42787, .T. ) ;
#4501=FACE_OUTER_BOUND ( 'NONE', #20780, .T. ) ;
#4502=DIRECTION ( 'NONE',  ( -0.3482016354343866471, 0.000000000000000000, -0.9374196611341253371 ) ) ;
#4503=FACE_OUTER_BOUND ( 'NONE', #39069, .T. ) ;
#4504=VECTOR ( 'NONE', #9541, 1000.000000000000000 ) ;
#4507=CARTESIAN_POINT ( 'NONE',  ( -8.721998590732194856, -177.1207230881787780, -118.5089480183145270 ) ) ;
#4508=AXIS2_PLACEMENT_3D ( 'NONE', #50657, #14651, #34861 ) ;
#4509=CARTESIAN_POINT ( 'NONE',  ( 45.36094686508022988, -183.6283474603465606, -82.57748230379237953 ) ) ;
#4511=EDGE_LOOP ( 'NONE', ( #44369, #16068, #13485, #31467 ) ) ;
#4512=DIRECTION ( 'NONE',  ( 0.000000000000000000, -0.000000000000000000, 1.000000000000000000 ) ) ;
#4513=CARTESIAN_POINT ( 'NONE',  ( 59.80284513346456521, -183.6283474603465606, 62.45009659481583952 ) ) ;
#4515=LINE ( 'NONE', #558, #44397 ) ;
#4516=CARTESIAN_POINT ( 'NONE',  ( -47.74129347246712740, -175.3837268820161057, -0.6749830015182022303 ) ) ;
#4517=ADVANCED_FACE ( 'NONE', ( #33721 ), #13756, .T. ) ;
#4518=ORIENTED_EDGE ( 'NONE', *, *, #28497, .T. ) ;
#4519=CARTESIAN_POINT ( 'NONE',  ( -168.6933499419502880, -183.6283474603465606, 30.40954281680879845 ) ) ;
#4520=ORIENTED_EDGE ( 'NONE', *, *, #26121, .T. ) ;
#4522=CARTESIAN_POINT ( 'NONE',  ( 67.66641500972444589, -175.3837268820161057, 46.20836643931066590 ) ) ;
#4524=DIRECTION ( 'NONE',  ( 0.000000000000000000, -0.000000000000000000, 1.000000000000000000 ) ) ;
#4525=DIRECTION ( 'NONE',  ( -0.000000000000000000, 1.000000000000000000, -0.000000000000000000 ) ) ;
#4527=AXIS2_PLACEMENT_3D ( 'NONE', #31728, #48012, #32231 ) ;
#4532=ORIENTED_EDGE ( 'NONE', *, *, #7051, .T. ) ;
#4534=EDGE_CURVE ( 'NONE', #45319, #37719, #41870, .T. ) ;
#4536=DIRECTION ( 'NONE',  ( 0.000000000000000000, -1.000000000000000000, -0.000000000000000000 ) ) ;
#4537=DIRECTION ( 'NONE',  ( 0.000000000000000000, 0.000000000000000000, 1.000000000000000000 ) ) ;
#4538=ORIENTED_EDGE ( 'NONE', *, *, #15846, .F. ) ;
#4539=VERTEX_POINT ( 'NONE', #10074 ) ;
#4540=ORIENTED_EDGE ( 'NONE', *, *, #27541, .F. ) ;
#4541=CARTESIAN_POINT ( 'NONE',  ( 70.49476099643867144, -177.1207230881787780, 34.94873081740416865 ) ) ;
#4542=PLANE ( 'NONE',  #35367 ) ;
#4544=ORIENTED_EDGE ( 'NONE', *, *, #47788, .T. ) ;
#4546=DIRECTION ( 'NONE',  ( 0.6965510290629982615, 0.000000000000000000, -0.7175072570443298270 ) ) ;
#4549=ORIENTED_EDGE ( 'NONE', *, *, #4125, .F. ) ;
#4550=EDGE_CURVE ( 'NONE', #51567, #49394, #18474, .T. ) ;
#4551=DIRECTION ( 'NONE',  ( 0.9890401873221644768, 0.000000000000000000, -0.1476465640024779702 ) ) ;
#4552=CARTESIAN_POINT ( 'NONE',  ( -95.18697522258271704, -183.6283474603465606, 115.9455772817713211 ) ) ;
#4553=AXIS2_PLACEMENT_3D ( 'NONE', #4827, #25304, #37906 ) ;
#4554=ORIENTED_EDGE ( 'NONE', *, *, #36426, .F. ) ;
#4555=DIRECTION ( 'NONE',  ( -0.6528221181905280446, 0.000000000000000000, 0.7575112421616145841 ) ) ;
#4556=AXIS2_PLACEMENT_3D ( 'NONE', #49890, #38819, #46725 ) ;
#4557=CARTESIAN_POINT ( 'NONE',  ( -173.1763543514842070, -183.6283474603465606, 8.694908215728892387 ) ) ;
#4558=DIRECTION ( 'NONE',  ( 0.9027978299657446470, 0.000000000000000000, -0.4300652022765183435 ) ) ;
#4561=EDGE_CURVE ( 'NONE', #9866, #10499, #44362, .T. ) ;
#4562=VERTEX_POINT ( 'NONE', #51074 ) ;
#4563=ORIENTED_EDGE ( 'NONE', *, *, #33251, .T. ) ;
#4564=DIRECTION ( 'NONE',  ( 0.000000000000000000, -1.000000000000000000, 0.000000000000000000 ) ) ;
#4567=DIRECTION ( 'NONE',  ( 0.000000000000000000, 0.000000000000000000, -1.000000000000000000 ) ) ;
#4568=CARTESIAN_POINT ( 'NONE',  ( 2.066935079424583765, -175.3837268820161057, -114.3245189510257802 ) ) ;
#4569=ORIENTED_EDGE ( 'NONE', *, *, #31332, .F. ) ;
#4571=VECTOR ( 'NONE', #929, 1000.000000000000114 ) ;
#4575=ORIENTED_EDGE ( 'NONE', *, *, #1732, .F. ) ;
#4576=CARTESIAN_POINT ( 'NONE',  ( -172.4422607493951318, -193.5000000000000000, 16.06677968424543579 ) ) ;
#4577=EDGE_LOOP ( 'NONE', ( #13481, #12977, #4037, #45093 ) ) ;
#4579=CYLINDRICAL_SURFACE ( 'NONE', #29880, 125.0000000000000000 ) ;
#4580=DIRECTION ( 'NONE',  ( -0.9027978299657416494, 0.000000000000000000, -0.4300652022765245608 ) ) ;
#4581=LINE ( 'NONE', #24548, #3083 ) ;
#4583=ORIENTED_EDGE ( 'NONE', *, *, #2249, .T. ) ;
#4584=DIRECTION ( 'NONE',  ( -0.000000000000000000, -1.000000000000000000, 0.000000000000000000 ) ) ;
#4585=ORIENTED_EDGE ( 'NONE', *, *, #5919, .T. ) ;
#4586=ORIENTED_EDGE ( 'NONE', *, *, #26085, .F. ) ;
#4587=CARTESIAN_POINT ( 'NONE',  ( -56.05401443572781517, -189.7472609257535510, 124.7702732086913073 ) ) ;
#4590=CIRCLE ( 'NONE', #33952, 125.0000000000000000 ) ;
#4592=ORIENTED_EDGE ( 'NONE', *, *, #10571, .T. ) ;
#4593=DIRECTION ( 'NONE',  ( -0.000000000000000000, -1.000000000000000000, 0.000000000000000000 ) ) ;
#4598=ORIENTED_EDGE ( 'NONE', *, *, #2892, .F. ) ;
#4599=DIRECTION ( 'NONE',  ( -0.8858462335218260097, 0.000000000000000000, 0.4639789333096864810 ) ) ;
#4600=VECTOR ( 'NONE', #34095, 1000.000000000000114 ) ;
#4603=CARTESIAN_POINT ( 'NONE',  ( 8.879953965148887463, -193.5000000000000000, 109.9360785596608849 ) ) ;
#4606=DIRECTION ( 'NONE',  ( 0.000000000000000000, 0.000000000000000000, -1.000000000000000000 ) ) ;
#4608=ORIENTED_EDGE ( 'NONE', *, *, #18532, .F. ) ;
#4609=ORIENTED_EDGE ( 'NONE', *, *, #926, .T. ) ;
#4611=CARTESIAN_POINT ( 'NONE',  ( -164.0008810331606810, -175.3837268820161057, 47.74645837849822527 ) ) ;
#4612=EDGE_CURVE ( 'NONE', #1159, #16305, #30546, .T. ) ;
#4615=CARTESIAN_POINT ( 'NONE',  ( -44.48323084606168720, -177.1207230881787780, 124.9361149384469769 ) ) ;
#4616=EDGE_LOOP ( 'NONE', ( #6012, #2106, #35546, #45814 ) ) ;
#4617=EDGE_LOOP ( 'NONE', ( #13248, #5203, #688, #36367 ) ) ;
#4620=FACE_OUTER_BOUND ( 'NONE', #7190, .T. ) ;
#4621=ORIENTED_EDGE ( 'NONE', *, *, #23988, .T. ) ;
#4622=AXIS2_PLACEMENT_3D ( 'NONE', #51448, #24802, #28469 ) ;
#4625=AXIS2_PLACEMENT_3D ( 'NONE', #12304, #39889, #27808 ) ;
#4626=AXIS2_PLACEMENT_3D ( 'NONE', #22164, #46350, #2186 ) ;
#4628=DIRECTION ( 'NONE',  ( -0.000000000000000000, 1.000000000000000000, -0.000000000000000000 ) ) ;
#4629=ORIENTED_EDGE ( 'NONE', *, *, #30401, .T. ) ;
#4630=CARTESIAN_POINT ( 'NONE',  ( 59.00260725618640123, -193.5000000000000000, -63.81752780152988436 ) ) ;
#4631=VERTEX_POINT ( 'NONE', #15064 ) ;
#4635=VECTOR ( 'NONE', #23816, 1000.000000000000000 ) ;
#4637=CARTESIAN_POINT ( 'NONE',  ( 66.03142248012325410, -193.5000000000000000, 50.12318939044039467 ) ) ;
#4640=EDGE_CURVE ( 'NONE', #2552, #31987, #31067, .T. ) ;
#4641=CARTESIAN_POINT ( 'NONE',  ( -123.6678354051270361, -189.7472609257535510, 99.85818990449065780 ) ) ;
#4647=ADVANCED_FACE ( 'NONE', ( #10847 ), #51563, .T. ) ;
#4648=LINE ( 'NONE', #32764, #33705 ) ;
#4650=FACE_BOUND ( 'NONE', #14053, .T. ) ;
#4651=VERTEX_POINT ( 'NONE', #32352 ) ;
#4652=DIRECTION ( 'NONE',  ( 0.1182731709213592358, 0.000000000000000000, 0.9929810960135178055 ) ) ;
#4653=ORIENTED_EDGE ( 'NONE', *, *, #18778, .T. ) ;
#4654=CARTESIAN_POINT ( 'NONE',  ( -12.13476221271687194, -175.3837268820161057, 119.5996955107804780 ) ) ;
#4656=CARTESIAN_POINT ( 'NONE',  ( 26.52087324849106054, -173.5000000000000284, -70.00000000000002842 ) ) ;
#4658=ORIENTED_EDGE ( 'NONE', *, *, #24720, .T. ) ;
#4659=EDGE_CURVE ( 'NONE', #36146, #24293, #3722, .T. ) ;
#4660=DIRECTION ( 'NONE',  ( 0.000000000000000000, 1.000000000000000000, -0.000000000000000000 ) ) ;
#4661=ADVANCED_FACE ( 'NONE', ( #39463 ), #27647, .F. ) ;
#4664=LINE ( 'NONE', #20692, #16209 ) ;
#4667=VECTOR ( 'NONE', #41285, 1000.000000000000000 ) ;
#4668=CARTESIAN_POINT ( 'NONE',  ( 37.29583330861160562, -193.5000000000000000, -89.54698061029594669 ) ) ;
#4670=ORIENTED_EDGE ( 'NONE', *, *, #10541, .F. ) ;
#4671=LINE ( 'NONE', #20702, #43538 ) ;
#4672=DIRECTION ( 'NONE',  ( 0.6068001458185890984, 0.000000000000000000, 0.7948544414133565938 ) ) ;
#4673=ORIENTED_EDGE ( 'NONE', *, *, #48285, .T. ) ;
#4674=AXIS2_PLACEMENT_3D ( 'NONE', #28400, #49174, #8434 ) ;
#4675=ADVANCED_FACE ( 'NONE', ( #47888 ), #23954, .T. ) ;
#4676=LINE ( 'NONE', #20437, #51135 ) ;
#4677=AXIS2_PLACEMENT_3D ( 'NONE', #5702, #16753, #40892 ) ;
#4679=CARTESIAN_POINT ( 'NONE',  ( -48.47912675150885065, -177.1207230881787780, 6.938893903907228378E-15 ) ) ;
#4680=AXIS2_PLACEMENT_3D ( 'NONE', #998, #48056, #8886 ) ;
#4681=VECTOR ( 'NONE', #33708, 1000.000000000000114 ) ;
#4683=CARTESIAN_POINT ( 'NONE',  ( -67.22356632362119910, -183.6283474603465606, -123.5865930638409793 ) ) ;
#4685=DIRECTION ( 'NONE',  ( -0.6749830015182091136, 0.000000000000000000, -0.7378332790417285736 ) ) ;
#4687=ORIENTED_EDGE ( 'NONE', *, *, #30225, .T. ) ;
#4688=ORIENTED_EDGE ( 'NONE', *, *, #24709, .T. ) ;
#4690=VERTEX_POINT ( 'NONE', #7673 ) ;
#4694=CARTESIAN_POINT ( 'NONE',  ( -47.87232660569026166, -189.7472609257535510, 0.7948544414133635883 ) ) ;
#4695=VERTEX_POINT ( 'NONE', #46 ) ;
#4698=ORIENTED_EDGE ( 'NONE', *, *, #33940, .T. ) ;
#4701=AXIS2_PLACEMENT_3D ( 'NONE', #33605, #29137, #45199 ) ;
#4702=LINE ( 'NONE', #24414, #23895 ) ;
#4704=DIRECTION ( 'NONE',  ( 0.000000000000000000, -1.000000000000000000, 0.000000000000000000 ) ) ;
#4706=AXIS2_PLACEMENT_3D ( 'NONE', #39392, #48334, #3400 ) ;
#4708=VECTOR ( 'NONE', #28360, 1000.000000000000227 ) ;
#4710=EDGE_CURVE ( 'NONE', #8813, #19788, #42704, .T. ) ;
#4712=PLANE ( 'NONE',  #25368 ) ;
#4713=DIRECTION ( 'NONE',  ( 0.000000000000000000, 1.000000000000000000, -0.000000000000000000 ) ) ;
#4714=CARTESIAN_POINT ( 'NONE',  ( -60.86541030502398542, -183.6283474603465606, -124.3848060646151623 ) ) ;
#4715=FACE_OUTER_BOUND ( 'NONE', #30165, .T. ) ;
#4716=ORIENTED_EDGE ( 'NONE', *, *, #47844, .F. ) ;
#4718=DIRECTION ( 'NONE',  ( 0.000000000000000000, 0.000000000000000000, -1.000000000000000000 ) ) ;
#4719=CIRCLE ( 'NONE', #34085, 125.0000000000000000 ) ;
#4722=PLANE ( 'NONE',  #25324 ) ;
#4723=ORIENTED_EDGE ( 'NONE', *, *, #47073, .T. ) ;
#4725=EDGE_CURVE ( 'NONE', #32204, #25437, #15027, .T. ) ;
#4726=CIRCLE ( 'NONE', #46705, 125.0000000000000000 ) ;
#4727=ORIENTED_EDGE ( 'NONE', *, *, #49335, .T. ) ;
#4728=ADVANCED_FACE ( 'NONE', ( #19749 ), #297, .T. ) ;
#4731=EDGE_CURVE ( 'NONE', #3968, #48534, #35781, .T. ) ;
#4734=DIRECTION ( 'NONE',  ( 0.3482016354343995812, 0.000000000000000000, -0.9374196611341205632 ) ) ;
#4735=EDGE_CURVE ( 'NONE', #12446, #23845, #31850, .T. ) ;
#4737=CARTESIAN_POINT ( 'NONE',  ( -172.4422607493951318, -183.6283474603465606, 16.06677968424543579 ) ) ;
#4738=CARTESIAN_POINT ( 'NONE',  ( 64.29733702426837283, -193.5000000000000000, 53.91167979418564471 ) ) ;
#4741=VERTEX_POINT ( 'NONE', #27891 ) ;
#4744=ORIENTED_EDGE ( 'NONE', *, *, #24342, .T. ) ;
#4745=PLANE ( 'NONE',  #40182 ) ;
#4750=DIRECTION ( 'NONE',  ( -0.8858462335218260097, 0.000000000000000000, -0.4639789333096864810 ) ) ;
#4751=ORIENTED_EDGE ( 'NONE', *, *, #50761, .F. ) ;
#4753=AXIS2_PLACEMENT_3D ( 'NONE', #40576, #4593, #4090 ) ;
#4754=AXIS2_PLACEMENT_3D ( 'NONE', #12685, #41071, #342 ) ;
#4755=CARTESIAN_POINT ( 'NONE',  ( -115.4536696835168641, -193.5000000000000000, -105.5434062319793185 ) ) ;
#4756=VECTOR ( 'NONE', #16926, 1000.000000000000000 ) ;
#4758=DIRECTION ( 'NONE',  ( 0.000000000000000000, -1.000000000000000000, 0.000000000000000000 ) ) ;
#4761=AXIS2_PLACEMENT_3D ( 'NONE', #17497, #1171, #20632 ) ;
#4762=DIRECTION ( 'NONE',  ( 0.9785564922995032555, 0.000000000000000000, 0.2059786187411021818 ) ) ;
#4765=CIRCLE ( 'NONE', #21543, 125.0000000000000000 ) ;
#4766=EDGE_CURVE ( 'NONE', #19096, #21817, #46921, .T. ) ;
#4767=LINE ( 'NONE', #1333, #33226 ) ;
#4768=DIRECTION ( 'NONE',  ( -0.000000000000000000, 1.000000000000000000, -0.000000000000000000 ) ) ;
#4773=LINE ( 'NONE', #24471, #15670 ) ;
#4775=ADVANCED_FACE ( 'NONE', ( #32096 ), #12113, .T. ) ;
#4776=ORIENTED_EDGE ( 'NONE', *, *, #15874, .T. ) ;
#4777=EDGE_CURVE ( 'NONE', #20693, #27989, #4515, .T. ) ;
#4778=LINE ( 'NONE', #13184, #38228 ) ;
#4779=EDGE_CURVE ( 'NONE', #26640, #6875, #11345, .T. ) ;
#4780=DIRECTION ( 'NONE',  ( 0.9151456172430210145, 0.000000000000000000, -0.4031234292879665171 ) ) ;
#4781=ORIENTED_EDGE ( 'NONE', *, *, #34306, .F. ) ;
#4783=CIRCLE ( 'NONE', #8943, 125.0000000000000000 ) ;
#4786=DIRECTION ( 'NONE',  ( -0.5829794791144703447, 0.000000000000000000, -0.8124868780056825335 ) ) ;
#4788=FACE_OUTER_BOUND ( 'NONE', #5093, .T. ) ;
#4789=PLANE ( 'NONE',  #23904 ) ;
#4790=CARTESIAN_POINT ( 'NONE',  ( -36.09284319799462537, -183.6283474603465606, 124.3848060646152618 ) ) ;
#4792=ADVANCED_FACE ( 'NONE', ( #50169 ), #22561, .T. ) ;
#4794=CIRCLE ( 'NONE', #38320, 124.9999999999999858 ) ;
#4795=ADVANCED_FACE ( 'NONE', ( #34376 ), #18090, .T. ) ;
#4798=FACE_OUTER_BOUND ( 'NONE', #44198, .T. ) ;
#4799=CARTESIAN_POINT ( 'NONE',  ( 73.09196206113300320, -193.5000000000000000, 29.07697310430963356 ) ) ;
#4800=ORIENTED_EDGE ( 'NONE', *, *, #490, .F. ) ;
#4801=AXIS2_PLACEMENT_3D ( 'NONE', #41455, #40478, #32083 ) ;
#4802=AXIS2_PLACEMENT_3D ( 'NONE', #39219, #17132, #28669 ) ;
#4806=VECTOR ( 'NONE', #42, 1000.000000000000000 ) ;
#4810=ORIENTED_EDGE ( 'NONE', *, *, #45737, .T. ) ;
#4812=ORIENTED_EDGE ( 'NONE', *, *, #34491, .F. ) ;
#4813=DIRECTION ( 'NONE',  ( 0.2348860457809842095, 0.000000000000000000, -0.9720229140804107493 ) ) ;
#4814=CARTESIAN_POINT ( 'NONE',  ( -64.08700758308646073, -189.7472609257535510, -124.0217483183786982 ) ) ;
#4820=PLANE ( 'NONE',  #15978 ) ;
#4821=VECTOR ( 'NONE', #6518, 1000.000000000000000 ) ;
#4823=VERTEX_POINT ( 'NONE', #46221 ) ;
#4824=AXIS2_PLACEMENT_3D ( 'NONE', #45269, #34196, #17413 ) ;
#4825=CARTESIAN_POINT ( 'NONE',  ( -48.47912675150885065, -183.6283474603465606, 6.938893903907228378E-15 ) ) ;
#4826=ORIENTED_EDGE ( 'NONE', *, *, #50049, .T. ) ;
#4827=CARTESIAN_POINT ( 'NONE',  ( -49.29161362951452929, -189.7472609257535510, -0.5829794791144748967 ) ) ;
#4831=DIRECTION ( 'NONE',  ( -0.8858462335218260097, -0.000000000000000000, 0.4639789333096864810 ) ) ;
#4832=CARTESIAN_POINT ( 'NONE',  ( -49.40581635894068313, -193.5000000000000000, -0.3758275821142418316 ) ) ;
#4833=EDGE_LOOP ( 'NONE', ( #26547, #7152, #9128, #12730 ) ) ;
#4834=VECTOR ( 'NONE', #8231, 1000.000000000000000 ) ;
#4836=CARTESIAN_POINT ( 'NONE',  ( -48.47912675150885065, -183.6283474603465606, 6.938893903907228378E-15 ) ) ;
#4837=CARTESIAN_POINT ( 'NONE',  ( -55.71438232577009586, -175.3837268820161057, -124.7904286264580662 ) ) ;
#4838=AXIS2_PLACEMENT_3D ( 'NONE', #45796, #33459, #13475 ) ;
#4839=VERTEX_POINT ( 'NONE', #38574 ) ;
#4840=CARTESIAN_POINT ( 'NONE',  ( -2.700932609314997457, -193.5000000000000000, -116.3157639405751809 ) ) ;
#4841=VECTOR ( 'NONE', #1469, 1000.000000000000000 ) ;
#4842=LINE ( 'NONE', #24534, #43832 ) ;
#4844=EDGE_CURVE ( 'NONE', #47870, #32445, #46467, .T. ) ;
#4845=ORIENTED_EDGE ( 'NONE', *, *, #38552, .T. ) ;
#4846=PLANE ( 'NONE',  #51947 ) ;
#4849=EDGE_CURVE ( 'NONE', #36987, #11325, #45697, .T. ) ;
#4851=ADVANCED_FACE ( 'NONE', ( #42244 ), #45440, .F. ) ;
#4852=ORIENTED_EDGE ( 'NONE', *, *, #48458, .T. ) ;
#4854=VERTEX_POINT ( 'NONE', #25712 ) ;
#4857=PLANE ( 'NONE',  #23177 ) ;
#4858=CARTESIAN_POINT ( 'NONE',  ( -95.18697522258271704, -183.6283474603465606, 115.9455772817713211 ) ) ;
#4861=VERTEX_POINT ( 'NONE', #18358 ) ;
#4862=DIRECTION ( 'NONE',  ( 0.7378332790417239107, 0.000000000000000000, 0.6749830015182142207 ) ) ;
#4864=ORIENTED_EDGE ( 'NONE', *, *, #31099, .T. ) ;
#4865=VECTOR ( 'NONE', #20072, 1000.000000000000114 ) ;
#4866=VECTOR ( 'NONE', #2621, 1000.000000000000000 ) ;
#4867=EDGE_CURVE ( 'NONE', #39129, #23608, #33853, .T. ) ;
#4868=CARTESIAN_POINT ( 'NONE',  ( -238.7407812814481076, -213.5000000000000000, -41.45482488023466061 ) ) ;
#4869=CARTESIAN_POINT ( 'NONE',  ( -49.25565061422690150, -175.3837268820161057, 0.6300878435817109935 ) ) ;
#4870=EDGE_LOOP ( 'NONE', ( #49194, #278, #42297, #16027 ) ) ;
#4871=AXIS2_PLACEMENT_3D ( 'NONE', #6688, #14838, #14311 ) ;
#4872=ORIENTED_EDGE ( 'NONE', *, *, #30380, .T. ) ;
#4874=ADVANCED_FACE ( 'NONE', ( #29909 ), #9956, .F. ) ;
#4875=CARTESIAN_POINT ( 'NONE',  ( -135.6699833737243637, -189.7472609257535510, 89.56983042009322560 ) ) ;
#4877=EDGE_LOOP ( 'NONE', ( #5711, #24882, #28345, #18724 ) ) ;
#4880=DIRECTION ( 'NONE',  ( -0.6068001458185834363, 0.000000000000000000, -0.7948544414133608127 ) ) ;
#4881=DIRECTION ( 'NONE',  ( -0.9995608365087940150, 0.000000000000000000, -0.02963332782257007206 ) ) ;
#4885=ORIENTED_EDGE ( 'NONE', *, *, #26417, .T. ) ;
#4887=AXIS2_PLACEMENT_3D ( 'NONE', #49172, #36541, #24461 ) ;
#4888=DIRECTION ( 'NONE',  ( 0.000000000000000000, -0.000000000000000000, -1.000000000000000000 ) ) ;
#4889=LINE ( 'NONE', #25367, #27703 ) ;
#4890=DIRECTION ( 'NONE',  ( 0.000000000000000000, -0.000000000000000000, -1.000000000000000000 ) ) ;
#4891=CARTESIAN_POINT ( 'NONE',  ( -38.66762320617019100, -183.6283474603465606, -124.6143426664033882 ) ) ;
#4893=ORIENTED_EDGE ( 'NONE', *, *, #34825, .T. ) ;
#4894=ORIENTED_EDGE ( 'NONE', *, *, #50777, .F. ) ;
#4896=ORIENTED_EDGE ( 'NONE', *, *, #42575, .T. ) ;
#4898=ORIENTED_EDGE ( 'NONE', *, *, #19246, .T. ) ;
#4899=AXIS2_PLACEMENT_3D ( 'NONE', #44054, #48266, #20658 ) ;
#4900=DIRECTION ( 'NONE',  ( 0.000000000000000000, -1.000000000000000000, 0.000000000000000000 ) ) ;
#4901=AXIS2_PLACEMENT_3D ( 'NONE', #31826, #20248, #35491 ) ;
#4902=FACE_OUTER_BOUND ( 'NONE', #17787, .T. ) ;
#4903=VECTOR ( 'NONE', #37370, 1000.000000000000000 ) ;
#4904=DIRECTION ( 'NONE',  ( 0.000000000000000000, 0.000000000000000000, -1.000000000000000000 ) ) ;
#4905=FACE_OUTER_BOUND ( 'NONE', #322, .T. ) ;
#4906=EDGE_CURVE ( 'NONE', #32338, #38633, #38047, .T. ) ;
#4907=LINE ( 'NONE', #9104, #34320 ) ;
#4911=ORIENTED_EDGE ( 'NONE', *, *, #15194, .F. ) ;
#4912=CARTESIAN_POINT ( 'NONE',  ( 1.755575411425465360, -193.5000000000000000, 114.4616734920527392 ) ) ;
#4913=CIRCLE ( 'NONE', #34273, 124.9999999999999858 ) ;
#4915=CARTESIAN_POINT ( 'NONE',  ( -34.63763967761164508, -175.3837268820161057, -123.2250735253142864 ) ) ;
#4916=DIRECTION ( 'NONE',  ( -1.000000000000000000, -0.000000000000000000, 4.884776371667511665E-16 ) ) ;
#4917=LINE ( 'NONE', #41415, #16303 ) ;
#4918=CARTESIAN_POINT ( 'NONE',  ( 25.43954814678887644, -183.6283474603465606, 100.8019320314832754 ) ) ;
#4925=FACE_BOUND ( 'NONE', #25137, .T. ) ;
#4927=EDGE_CURVE ( 'NONE', #29810, #35254, #10720, .T. ) ;
#4928=LINE ( 'NONE', #20952, #28960 ) ;
#4930=DIRECTION ( 'NONE',  ( -0.000000000000000000, 1.000000000000000000, -0.000000000000000000 ) ) ;
#4932=DIRECTION ( 'NONE',  ( 0.9929810960135161402, 0.000000000000000000, 0.1182731709213730997 ) ) ;
#4933=ORIENTED_EDGE ( 'NONE', *, *, #7554, .F. ) ;
#4936=AXIS2_PLACEMENT_3D ( 'NONE', #22735, #14597, #30600 ) ;
#4940=ORIENTED_EDGE ( 'NONE', *, *, #48536, .T. ) ;
#4941=AXIS2_PLACEMENT_3D ( 'NONE', #49927, #22062, #22592 ) ;
#4943=CARTESIAN_POINT ( 'NONE',  ( -47.97059563285963435, -189.7472609257535510, 0.8610436117673654355 ) ) ;
#4945=EDGE_LOOP ( 'NONE', ( #14046, #15469, #22508, #16520 ) ) ;
#4949=CARTESIAN_POINT ( 'NONE',  ( -111.3295483157475729, -175.3837268820161057, 108.0501018472332362 ) ) ;
#4951=ORIENTED_EDGE ( 'NONE', *, *, #20866, .F. ) ;
#4953=CARTESIAN_POINT ( 'NONE',  ( -62.97606545226379637, -175.3837268820161057, -123.1496609813404177 ) ) ;
#4954=CARTESIAN_POINT ( 'NONE',  ( -164.3791542526839464, -189.7472609257535510, 46.82076062204520639 ) ) ;
#4955=AXIS2_PLACEMENT_3D ( 'NONE', #38295, #21768, #14396 ) ;
#4959=ORIENTED_EDGE ( 'NONE', *, *, #30356, .F. ) ;
#4960=CARTESIAN_POINT ( 'NONE',  ( -49.35486169370448550, -177.1207230881787780, -0.4827922027307481878 ) ) ;
#4963=ORIENTED_EDGE ( 'NONE', *, *, #9017, .F. ) ;
#4964=CARTESIAN_POINT ( 'NONE',  ( -99.02518858244150124, -175.3837268820161057, 114.3245189510261497 ) ) ;
#4965=ORIENTED_EDGE ( 'NONE', *, *, #23692, .F. ) ;
#4966=FACE_OUTER_BOUND ( 'NONE', #39955, .T. ) ;
#4969=EDGE_CURVE ( 'NONE', #34216, #27501, #3347, .T. ) ;
#4970=CARTESIAN_POINT ( 'NONE',  ( -48.47912675150885065, -183.6283474603465606, 6.938893903907228378E-15 ) ) ;
#4971=EDGE_LOOP ( 'NONE', ( #23890, #46570, #15532, #46947 ) ) ;
#4972=DIRECTION ( 'NONE',  ( 0.000000000000000000, 0.000000000000000000, 1.000000000000000000 ) ) ;
#4973=ORIENTED_EDGE ( 'NONE', *, *, #41733, .T. ) ;
#4974=ORIENTED_EDGE ( 'NONE', *, *, #43975, .T. ) ;
#4975=FACE_OUTER_BOUND ( 'NONE', #29299, .T. ) ;
#4976=ADVANCED_FACE ( 'NONE', ( #38822 ), #19128, .T. ) ;
#4981=ORIENTED_EDGE ( 'NONE', *, *, #51911, .T. ) ;
#4983=DIRECTION ( 'NONE',  ( 0.000000000000000000, -0.000000000000000000, -1.000000000000000000 ) ) ;
#4985=CARTESIAN_POINT ( 'NONE',  ( -48.64924157374594671, -175.3837268820161057, 124.9998842437354227 ) ) ;
#4986=LINE ( 'NONE', #49390, #2698 ) ;
#4987=LINE ( 'NONE', #17336, #2828 ) ;
#4989=DIRECTION ( 'NONE',  ( 0.000000000000000000, 0.000000000000000000, 1.000000000000000000 ) ) ;
#4991=ORIENTED_EDGE ( 'NONE', *, *, #4182, .T. ) ;
#4992=DIRECTION ( 'NONE',  ( 0.000000000000000000, 0.000000000000000000, -1.000000000000000000 ) ) ;
#4994=CARTESIAN_POINT ( 'NONE',  ( 75.21854001195777073, -177.1207230881787780, -8.665274887905439982 ) ) ;
#4995=PLANE ( 'NONE',  #14420 ) ;
#4996=AXIS2_PLACEMENT_3D ( 'NONE', #29745, #9792, #2668 ) ;
#4997=EDGE_LOOP ( 'NONE', ( #1117, #27493, #34912, #45983 ) ) ;
#4998=ORIENTED_EDGE ( 'NONE', *, *, #20880, .T. ) ;
#5001=DIRECTION ( 'NONE',  ( 0.2348860457809707758, 0.000000000000000000, 0.9720229140804138579 ) ) ;
#5002=CARTESIAN_POINT ( 'NONE',  ( -48.47912675150885065, -177.1207230881787780, 6.938893903907228378E-15 ) ) ;
#5003=FACE_OUTER_BOUND ( 'NONE', #257, .T. ) ;
#5008=CARTESIAN_POINT ( 'NONE',  ( -47.70260288879080690, -183.6283474603465606, -0.6300878435817026668 ) ) ;
#5010=DIRECTION ( 'NONE',  ( -0.000000000000000000, -1.000000000000000000, 0.000000000000000000 ) ) ;
#5011=AXIS2_PLACEMENT_3D ( 'NONE', #24563, #40578, #12727 ) ;
#5012=ORIENTED_EDGE ( 'NONE', *, *, #33400, .F. ) ;
#5013=DIRECTION ( 'NONE',  ( -0.4566292373937018145, 0.000000000000000000, -0.8896570909947529859 ) ) ;
#5014=VECTOR ( 'NONE', #10304, 1000.000000000000227 ) ;
#5015=EDGE_CURVE ( 'NONE', #38434, #8106, #15623, .T. ) ;
#5019=CARTESIAN_POINT ( 'NONE',  ( -12.13476221271688615, -175.3837268820161057, 119.5996955107804638 ) ) ;
#5021=DIRECTION ( 'NONE',  ( 0.000000000000000000, 0.000000000000000000, 1.000000000000000000 ) ) ;
#5023=DIRECTION ( 'NONE',  ( -0.9785564922995017012, 0.000000000000000000, -0.2059786187411094538 ) ) ;
#5024=ORIENTED_EDGE ( 'NONE', *, *, #40626, .F. ) ;
#5025=CARTESIAN_POINT ( 'NONE',  ( -146.0653709326077490, -189.7472609257535510, -78.11481899503411341 ) ) ;
#5026=DIRECTION ( 'NONE',  ( -0.000000000000000000, 1.000000000000000000, -0.000000000000000000 ) ) ;
#5027=ORIENTED_EDGE ( 'NONE', *, *, #17642, .F. ) ;
#5029=CARTESIAN_POINT ( 'NONE',  ( 67.66641500972444589, -189.7472609257535510, 46.20836643931066590 ) ) ;
#5030=DIRECTION ( 'NONE',  ( -0.4031234292879600778, 0.000000000000000000, -0.9151456172430237901 ) ) ;
#5031=DIRECTION ( 'NONE',  ( 0.9473263538541899509, 0.000000000000000000, 0.3202698538628415692 ) ) ;
#5037=EDGE_CURVE ( 'NONE', #51798, #2804, #27249, .T. ) ;
#5038=DIRECTION ( 'NONE',  ( 0.000000000000000000, 1.000000000000000000, -0.000000000000000000 ) ) ;
#5039=ORIENTED_EDGE ( 'NONE', *, *, #14585, .T. ) ;
#5040=CARTESIAN_POINT ( 'NONE',  ( -171.4559849729830603, -183.6283474603465606, 22.39848972532371718 ) ) ;
#5042=CARTESIAN_POINT ( 'NONE',  ( -38.66762320617019100, -177.1207230881787780, -124.6143426664033882 ) ) ;
#5043=CARTESIAN_POINT ( 'NONE',  ( -166.8403286750647680, -189.7472609257535510, -40.19484891389974734 ) ) ;
#5044=ADVANCED_FACE ( 'NONE', ( #47501 ), #7802, .F. ) ;
#5046=CARTESIAN_POINT ( 'NONE',  ( -141.5426765053792906, -183.6283474603465606, 81.94739446021134199 ) ) ;
#5047=DIRECTION ( 'NONE',  ( -0.000000000000000000, 1.000000000000000000, -0.000000000000000000 ) ) ;
#5048=ORIENTED_EDGE ( 'NONE', *, *, #36756, .F. ) ;
#5049=VECTOR ( 'NONE', #16956, 1000.000000000000000 ) ;
#5050=CARTESIAN_POINT ( 'NONE',  ( 76.04209377433249983, -189.7472609257535510, -10.93003379476865611 ) ) ;
#5052=DIRECTION ( 'NONE',  ( -0.1768902751225666370, 0.000000000000000000, -0.9842305779475979399 ) ) ;
#5053=DIRECTION ( 'NONE',  ( -0.000000000000000000, 1.000000000000000000, -0.000000000000000000 ) ) ;
#5055=CARTESIAN_POINT ( 'NONE',  ( -143.2689064740322067, -183.6283474603465606, -79.94433946042767047 ) ) ;
#5057=DIRECTION ( 'NONE',  ( -0.000000000000000000, 1.000000000000000000, -0.000000000000000000 ) ) ;
#5058=ORIENTED_EDGE ( 'NONE', *, *, #13061, .T. ) ;
#5062=VECTOR ( 'NONE', #26047, 1000.000000000000000 ) ;
#5064=ORIENTED_EDGE ( 'NONE', *, *, #34902, .F. ) ;
#5066=ORIENTED_EDGE ( 'NONE', *, *, #27417, .T. ) ;
#5067=EDGE_CURVE ( 'NONE', #21790, #47759, #31199, .T. ) ;
#5068=CARTESIAN_POINT ( 'NONE',  ( -48.47912675150885065, -177.1207230881787780, 6.938893903907228378E-15 ) ) ;
#5069=EDGE_CURVE ( 'NONE', #48404, #40700, #47252, .T. ) ;
#5070=EDGE_CURVE ( 'NONE', #25951, #26701, #11220, .T. ) ;
#5072=FACE_OUTER_BOUND ( 'NONE', #25891, .T. ) ;
#5073=CARTESIAN_POINT ( 'NONE',  ( -49.47868758801764955, -193.5000000000000000, -0.02963332782256313663 ) ) ;
#5074=ORIENTED_EDGE ( 'NONE', *, *, #34657, .F. ) ;
#5075=ORIENTED_EDGE ( 'NONE', *, *, #13394, .T. ) ;
#5078=DIRECTION ( 'NONE',  ( 0.8455960035018199594, 0.000000000000000000, 0.5338233779648003940 ) ) ;
#5079=VERTEX_POINT ( 'NONE', #44341 ) ;
#5080=CIRCLE ( 'NONE', #34444, 125.0000000000000000 ) ;
#5082=EDGE_CURVE ( 'NONE', #471, #24853, #29032, .T. ) ;
#5083=CARTESIAN_POINT ( 'NONE',  ( 76.01188277843577623, -189.7472609257535510, 11.26891947860283061 ) ) ;
#5084=VERTEX_POINT ( 'NONE', #28021 ) ;
#5087=PLANE ( 'NONE',  #38323 ) ;
#5090=CARTESIAN_POINT ( 'NONE',  ( -40.24578378811990831, -193.5000000000000000, 124.7285535218268251 ) ) ;
#5091=EDGE_CURVE ( 'NONE', #36064, #46209, #37443, .T. ) ;
#5093=EDGE_LOOP ( 'NONE', ( #12922, #7712, #8845, #13939 ) ) ;
#5094=CARTESIAN_POINT ( 'NONE',  ( 70.98542830588607444, -193.5000000000000000, -36.78613984829961936 ) ) ;
#5095=EDGE_CURVE ( 'NONE', #17485, #23694, #24870, .T. ) ;
#5096=CARTESIAN_POINT ( 'NONE',  ( -167.1668396246903114, -177.1207230881787780, -35.90758392117661657 ) ) ;
#5097=ORIENTED_EDGE ( 'NONE', *, *, #46111, .T. ) ;
#5098=DIRECTION ( 'NONE',  ( -0.000000000000000000, 1.000000000000000000, -0.000000000000000000 ) ) ;
#5099=ADVANCED_FACE ( 'NONE', ( #16751 ), #44062, .T. ) ;
#5100=CARTESIAN_POINT ( 'NONE',  ( -48.41988612361514299, -193.5000000000000000, -0.9982437317643144681 ) ) ;
#5101=VERTEX_POINT ( 'NONE', #40358 ) ;
#5103=EDGE_CURVE ( 'NONE', #38078, #5877, #10589, .T. ) ;
#5104=CARTESIAN_POINT ( 'NONE',  ( 63.82222181224018698, -175.3837268820161057, 52.57768177182521896 ) ) ;
#5105=VECTOR ( 'NONE', #33395, 1000.000000000000000 ) ;
#5106=AXIS2_PLACEMENT_3D ( 'NONE', #48415, #36310, #5052 ) ;
#5107=ORIENTED_EDGE ( 'NONE', *, *, #22979, .T. ) ;
#5108=LINE ( 'NONE', #638, #4756 ) ;
#5109=ORIENTED_EDGE ( 'NONE', *, *, #9017, .T. ) ;
#5111=LINE ( 'NONE', #13249, #29420 ) ;
#5112=VERTEX_POINT ( 'NONE', #4915 ) ;
#5113=PLANE ( 'NONE',  #22351 ) ;
#5114=CARTESIAN_POINT ( 'NONE',  ( -49.32472275501068282, -175.3837268820161057, 0.5338233779647895139 ) ) ;
#5115=CYLINDRICAL_SURFACE ( 'NONE', #12301, 125.0000000000000000 ) ;
#5116=DIRECTION ( 'NONE',  ( 0.9646355819083594074, 0.000000000000000000, -0.2635871660690647933 ) ) ;
#5117=EDGE_CURVE ( 'NONE', #12735, #1095, #3869, .T. ) ;
#5119=DIRECTION ( 'NONE',  ( -0.000000000000000000, 1.000000000000000000, -0.000000000000000000 ) ) ;
#5120=VERTEX_POINT ( 'NONE', #32756 ) ;
#5122=VECTOR ( 'NONE', #7259, 1000.000000000000000 ) ;
#5125=EDGE_LOOP ( 'NONE', ( #45449, #7926, #8710, #24424 ) ) ;
#5126=EDGE_LOOP ( 'NONE', ( #38864, #2851, #48361, #29230 ) ) ;
#5127=CARTESIAN_POINT ( 'NONE',  ( 75.47134233844786877, -193.5000000000000000, -3.504489105734896803 ) ) ;
#5128=ADVANCED_FACE ( 'NONE', ( #40616 ), #19890, .F. ) ;
#5130=CARTESIAN_POINT ( 'NONE',  ( -127.4665351220365608, -183.6283474603465606, -96.88131563365296017 ) ) ;
#5131=ORIENTED_EDGE ( 'NONE', *, *, #3446, .F. ) ;
#5132=DIRECTION ( 'NONE',  ( 0.000000000000000000, 1.000000000000000000, 0.000000000000000000 ) ) ;
#5133=ORIENTED_EDGE ( 'NONE', *, *, #47370, .T. ) ;
#5134=DIRECTION ( 'NONE',  ( -0.000000000000000000, 1.000000000000000000, -0.000000000000000000 ) ) ;
#5136=VECTOR ( 'NONE', #32364, 1000.000000000000000 ) ;
#5137=ADVANCED_FACE ( 'NONE', ( #48273 ), #423, .T. ) ;
#5138=EDGE_CURVE ( 'NONE', #4337, #30281, #32413, .T. ) ;
#5139=EDGE_CURVE ( 'NONE', #48181, #3854, #31970, .T. ) ;
#5140=DIRECTION ( 'NONE',  ( -0.000000000000000000, 1.000000000000000000, -0.000000000000000000 ) ) ;
#5143=ORIENTED_EDGE ( 'NONE', *, *, #51972, .T. ) ;
#5148=CARTESIAN_POINT ( 'NONE',  ( 76.43863189440992301, -189.7472609257535510, -4.533605064403313456 ) ) ;
#5151=PLANE ( 'NONE',  #40637 ) ;
#5152=ORIENTED_EDGE ( 'NONE', *, *, #16410, .T. ) ;
#5158=EDGE_CURVE ( 'NONE', #13423, #4690, #7250, .T. ) ;
#5159=FACE_OUTER_BOUND ( 'NONE', #50140, .T. ) ;
#5160=CARTESIAN_POINT ( 'NONE',  ( -164.8312043469690593, -193.5000000000000000, -42.87565520599202529 ) ) ;
#5161=CARTESIAN_POINT ( 'NONE',  ( -47.78257572244586271, -175.3837268820161057, 0.7175072570443418174 ) ) ;
#5162=EDGE_CURVE ( 'NONE', #13423, #2282, #11044, .T. ) ;
#5163=CARTESIAN_POINT ( 'NONE',  ( -48.47912675150885065, -177.1207230881787780, 6.938893903907228378E-15 ) ) ;
#5165=EDGE_LOOP ( 'NONE', ( #21508, #34881, #44394, #32658 ) ) ;
#5166=CARTESIAN_POINT ( 'NONE',  ( 74.77174840718836890, -193.5000000000000000, 20.83798868929603643 ) ) ;
#5168=EDGE_CURVE ( 'NONE', #15221, #12949, #31021, .T. ) ;
#5169=EDGE_LOOP ( 'NONE', ( #28365, #758, #11382, #15914 ) ) ;
#5173=ORIENTED_EDGE ( 'NONE', *, *, #14048, .T. ) ;
#5176=DIRECTION ( 'NONE',  ( -0.9374196611341254481, 0.000000000000000000, 0.3482016354343867026 ) ) ;
#5177=LINE ( 'NONE', #44849, #32921 ) ;
#5181=FACE_OUTER_BOUND ( 'NONE', #49947, .T. ) ;
#5182=VECTOR ( 'NONE', #23344, 1000.000000000000000 ) ;
#5183=CARTESIAN_POINT ( 'NONE',  ( 61.98524708613674505, -193.5000000000000000, 56.33604425924832526 ) ) ;
#5184=FACE_BOUND ( 'NONE', #9444, .T. ) ;
#5185=ORIENTED_EDGE ( 'NONE', *, *, #7290, .T. ) ;
#5186=CARTESIAN_POINT ( 'NONE',  ( 76.01188277843579044, -175.3837268820161057, 11.26891947860284482 ) ) ;
#5187=ORIENTED_EDGE ( 'NONE', *, *, #8035, .F. ) ;
#5188=CARTESIAN_POINT ( 'NONE',  ( 28.02885774092381865, -175.3837268820161057, 98.85104101073331151 ) ) ;
#5192=VECTOR ( 'NONE', #375, 1000.000000000000000 ) ;
#5193=DIRECTION ( 'NONE',  ( -0.8757349421956412971, 0.000000000000000000, 0.4827922027307366970 ) ) ;
#5196=DIRECTION ( 'NONE',  ( 0.000000000000000000, 1.000000000000000000, 0.000000000000000000 ) ) ;
#5197=ORIENTED_EDGE ( 'NONE', *, *, #34887, .T. ) ;
#5198=ADVANCED_FACE ( 'NONE', ( #47067 ), #27073, .T. ) ;
#5199=EDGE_CURVE ( 'NONE', #4116, #16039, #30718, .T. ) ;
#5201=VERTEX_POINT ( 'NONE', #15262 ) ;
#5202=VERTEX_POINT ( 'NONE', #47327 ) ;
#5203=ORIENTED_EDGE ( 'NONE', *, *, #22179, .F. ) ;
#5206=LINE ( 'NONE', #735, #33567 ) ;
#5207=EDGE_LOOP ( 'NONE', ( #18500, #49859, #9155, #27760 ) ) ;
#5208=FACE_OUTER_BOUND ( 'NONE', #6742, .T. ) ;
#5209=LINE ( 'NONE', #19465, #21120 ) ;
#5210=LINE ( 'NONE', #33574, #49032 ) ;
#5211=CIRCLE ( 'NONE', #51389, 125.0000000000000000 ) ;
#5212=ORIENTED_EDGE ( 'NONE', *, *, #7324, .F. ) ;
#5214=VECTOR ( 'NONE', #33926, 1000.000000000000114 ) ;
#5223=DIRECTION ( 'NONE',  ( 0.000000000000000000, 0.000000000000000000, -1.000000000000000000 ) ) ;
#5226=ORIENTED_EDGE ( 'NONE', *, *, #9874, .F. ) ;
#5227=DIRECTION ( 'NONE',  ( -0.000000000000000000, 1.000000000000000000, -0.000000000000000000 ) ) ;
#5228=FACE_OUTER_BOUND ( 'NONE', #31964, .T. ) ;
#5229=ORIENTED_EDGE ( 'NONE', *, *, #31741, .F. ) ;
#5231=ORIENTED_EDGE ( 'NONE', *, *, #33191, .T. ) ;
#5232=AXIS2_PLACEMENT_3D ( 'NONE', #20289, #839, #28944 ) ;
#5234=ORIENTED_EDGE ( 'NONE', *, *, #20200, .F. ) ;
#5235=DIRECTION ( 'NONE',  ( 0.000000000000000000, 0.000000000000000000, 1.000000000000000000 ) ) ;
#5236=VECTOR ( 'NONE', #17591, 1000.000000000000114 ) ;
#5237=CARTESIAN_POINT ( 'NONE',  ( -8.721998590732173540, -183.6283474603465606, -118.5089480183145128 ) ) ;
#5238=CIRCLE ( 'NONE', #36266, 125.0000000000000000 ) ;
#5239=CARTESIAN_POINT ( 'NONE',  ( 30.05499637021958392, -177.1207230881787780, -97.24912084693205827 ) ) ;
#5240=DIRECTION ( 'NONE',  ( 0.000000000000000000, 0.000000000000000000, 1.000000000000000000 ) ) ;
#5241=ORIENTED_EDGE ( 'NONE', *, *, #50570, .F. ) ;
#5242=DIRECTION ( 'NONE',  ( 0.000000000000000000, -1.000000000000000000, -0.000000000000000000 ) ) ;
#5245=DIRECTION ( 'NONE',  ( 0.000000000000000000, 0.000000000000000000, 1.000000000000000000 ) ) ;
#5248=LINE ( 'NONE', #1280, #11450 ) ;
#5249=VERTEX_POINT ( 'NONE', #32438 ) ;
#5250=EDGE_LOOP ( 'NONE', ( #33276, #26247, #50368, #36390 ) ) ;
#5252=CARTESIAN_POINT ( 'NONE',  ( -213.8817838414232426, -193.5000000000000000, 10.00000000000002842 ) ) ;
#5253=ORIENTED_EDGE ( 'NONE', *, *, #37515, .T. ) ;
#5254=ORIENTED_EDGE ( 'NONE', *, *, #20417, .F. ) ;
#5257=EDGE_CURVE ( 'NONE', #21902, #30065, #47547, .T. ) ;
#5262=ORIENTED_EDGE ( 'NONE', *, *, #51590, .F. ) ;
#5263=PLANE ( 'NONE',  #49320 ) ;
#5264=EDGE_CURVE ( 'NONE', #48345, #10459, #24037, .T. ) ;
#5267=CIRCLE ( 'NONE', #34613, 125.0000000000000000 ) ;
#5268=DIRECTION ( 'NONE',  ( -0.6068001458185945385, 0.000000000000000000, 0.7948544414133523750 ) ) ;
#5269=VERTEX_POINT ( 'NONE', #48219 ) ;
#5270=FACE_OUTER_BOUND ( 'NONE', #4332, .T. ) ;
#5271=AXIS2_PLACEMENT_3D ( 'NONE', #30114, #21720, #42185 ) ;
#5272=EDGE_CURVE ( 'NONE', #49114, #27618, #4783, .T. ) ;
#5273=CIRCLE ( 'NONE', #34619, 125.0000000000000000 ) ;
#5275=CARTESIAN_POINT ( 'NONE',  ( -145.4373324222574126, -193.5000000000000000, -78.89300572996837957 ) ) ;
#5276=ORIENTED_EDGE ( 'NONE', *, *, #36574, .T. ) ;
#5279=ORIENTED_EDGE ( 'NONE', *, *, #28788, .T. ) ;
#5281=DIRECTION ( 'NONE',  ( 0.000000000000000000, 0.000000000000000000, -1.000000000000000000 ) ) ;
#5283=ADVANCED_FACE ( 'NONE', ( #8266 ), #5115, .T. ) ;
#5285=VERTEX_POINT ( 'NONE', #4075 ) ;
#5286=CARTESIAN_POINT ( 'NONE',  ( -152.8876895714563773, -189.7472609257535510, 66.89437584437912676 ) ) ;
#5288=CARTESIAN_POINT ( 'NONE',  ( -149.3265790242249125, -193.5000000000000000, 72.15117186584558340 ) ) ;
#5289=ORIENTED_EDGE ( 'NONE', *, *, #47163, .T. ) ;
#5291=LINE ( 'NONE', #49173, #50959 ) ;
#5292=CARTESIAN_POINT ( 'NONE',  ( -129.3001299485802633, -189.7472609257535510, -94.04236105995799733 ) ) ;
#5293=ORIENTED_EDGE ( 'NONE', *, *, #31357, .T. ) ;
#5294=ORIENTED_EDGE ( 'NONE', *, *, #4156, .T. ) ;
#5295=AXIS2_PLACEMENT_3D ( 'NONE', #32308, #3678, #47329 ) ;
#5296=CARTESIAN_POINT ( 'NONE',  ( 27.50603775690334274, -189.7472609257535510, -99.25348746834811209 ) ) ;
#5297=DIRECTION ( 'NONE',  ( 0.000000000000000000, 0.000000000000000000, 1.000000000000000000 ) ) ;
#5298=DIRECTION ( 'NONE',  ( -0.000000000000000000, -1.000000000000000000, 0.000000000000000000 ) ) ;
#5299=EDGE_LOOP ( 'NONE', ( #8382, #39030, #44092, #3263 ) ) ;
#5300=DIRECTION ( 'NONE',  ( -0.9960498426152171181, 0.000000000000000000, 0.08879589532293157006 ) ) ;
#5301=CARTESIAN_POINT ( 'NONE',  ( -94.25732089370191602, -183.6283474603465606, 116.3157639405754935 ) ) ;
#5303=EDGE_LOOP ( 'NONE', ( #23409, #19625, #6002, #41668 ) ) ;
#5304=AXIS2_PLACEMENT_3D ( 'NONE', #26809, #27589, #15007 ) ;
#5305=CARTESIAN_POINT ( 'NONE',  ( -149.9407190013152160, -175.3837268820161057, -73.01058346660458653 ) ) ;
#5306=VECTOR ( 'NONE', #45460, 999.9999999999998863 ) ;
#5307=DIRECTION ( 'NONE',  ( -0.000000000000000000, 1.000000000000000000, -0.000000000000000000 ) ) ;
#5309=ORIENTED_EDGE ( 'NONE', *, *, #48392, .F. ) ;
#5312=CARTESIAN_POINT ( 'NONE',  ( -47.55243714407701816, -193.5000000000000000, -0.3758275821142288420 ) ) ;
#5317=DIRECTION ( 'NONE',  ( 0.000000000000000000, -1.000000000000000000, -0.000000000000000000 ) ) ;
#5321=PLANE ( 'NONE',  #31229 ) ;
#5324=EDGE_LOOP ( 'NONE', ( #6168, #51958, #1138, #12611 ) ) ;
#5325=LINE ( 'NONE', #9775, #25753 ) ;
#5326=ADVANCED_FACE ( 'NONE', ( #24814 ), #40830, .T. ) ;
#5327=EDGE_CURVE ( 'NONE', #41796, #265, #4581, .T. ) ;
#5330=PLANE ( 'NONE',  #36364 ) ;
#5331=CARTESIAN_POINT ( 'NONE',  ( -30.31202594373736403, -183.6283474603465606, -123.6727797384705951 ) ) ;
#5332=ORIENTED_EDGE ( 'NONE', *, *, #2505, .T. ) ;
#5333=VERTEX_POINT ( 'NONE', #24296 ) ;
#5335=EDGE_LOOP ( 'NONE', ( #36991, #42920, #19832, #29285 ) ) ;
#5336=CARTESIAN_POINT ( 'NONE',  ( -47.48307690889363641, -175.3837268820161057, 0.08879589532294547560 ) ) ;
#5338=DIRECTION ( 'NONE',  ( 0.000000000000000000, 1.000000000000000000, 0.000000000000000000 ) ) ;
#5339=ORIENTED_EDGE ( 'NONE', *, *, #20842, .F. ) ;
#5343=AXIS2_PLACEMENT_3D ( 'NONE', #35132, #51439, #3074 ) ;
#5345=ORIENTED_EDGE ( 'NONE', *, *, #24348, .F. ) ;
#5346=CARTESIAN_POINT ( 'NONE',  ( -48.47912675150885065, -183.6283474603465606, 6.938893903907228378E-15 ) ) ;
#5349=DIRECTION ( 'NONE',  ( 0.000000000000000000, 0.000000000000000000, 1.000000000000000000 ) ) ;
#5351=ORIENTED_EDGE ( 'NONE', *, *, #43170, .F. ) ;
#5353=DIRECTION ( 'NONE',  ( 0.000000000000000000, -1.000000000000000000, 0.000000000000000000 ) ) ;
#5354=CARTESIAN_POINT ( 'NONE',  ( 43.18784210722336780, -175.3837268820161057, -84.98333260264752198 ) ) ;
#5358=EDGE_LOOP ( 'NONE', ( #20860, #24051, #4052, #2729 ) ) ;
#5361=VECTOR ( 'NONE', #10453, 1000.000000000000000 ) ;
#5362=EDGE_LOOP ( 'NONE', ( #20699, #6750, #37266, #13609 ) ) ;
#5365=LINE ( 'NONE', #21382, #11134 ) ;
#5366=PLANE ( 'NONE',  #20302 ) ;
#5367=ORIENTED_EDGE ( 'NONE', *, *, #45780, .F. ) ;
#5368=ADVANCED_FACE ( 'NONE', ( #16936 ), #32695, .T. ) ;
#5371=CARTESIAN_POINT ( 'NONE',  ( -121.1142239062970418, -177.1207230881787780, 101.7307360698549132 ) ) ;
#5372=DIRECTION ( 'NONE',  ( 0.000000000000000000, 0.000000000000000000, -1.000000000000000000 ) ) ;
#5374=AXIS2_PLACEMENT_3D ( 'NONE', #13726, #45793, #9789 ) ;
#5375=PLANE ( 'NONE',  #42542 ) ;
#5377=FACE_OUTER_BOUND ( 'NONE', #10324, .T. ) ;
#5378=EDGE_LOOP ( 'NONE', ( #34765, #47494, #37205, #48118 ) ) ;
#5380=CARTESIAN_POINT ( 'NONE',  ( 67.04262753014327814, -175.3837268820161057, -47.74645837849745078 ) ) ;
#5381=LINE ( 'NONE', #50311, #38771 ) ;
#5382=ORIENTED_EDGE ( 'NONE', *, *, #23427, .F. ) ;
#5385=DIRECTION ( 'NONE',  ( 0.000000000000000000, 1.000000000000000000, 0.000000000000000000 ) ) ;
#5386=ADVANCED_FACE ( 'NONE', ( #15908 ), #1683, .T. ) ;
#5387=ADVANCED_FACE ( 'NONE', ( #26101 ), #33213, .T. ) ;
#5388=DIRECTION ( 'NONE',  ( -1.000000000000000000, 0.000000000000000000, 0.000000000000000000 ) ) ;
#5391=DIRECTION ( 'NONE',  ( 0.9473263538541923934, 0.000000000000000000, -0.3202698538628350744 ) ) ;
#5393=LINE ( 'NONE', #16961, #2358 ) ;
#5394=LINE ( 'NONE', #45600, #34231 ) ;
#5396=EDGE_CURVE ( 'NONE', #35024, #19199, #37937, .T. ) ;
#5397=CIRCLE ( 'NONE', #31405, 125.0000000000000000 ) ;
#5400=ORIENTED_EDGE ( 'NONE', *, *, #11730, .T. ) ;
#5402=VECTOR ( 'NONE', #24607, 1000.000000000000000 ) ;
#5405=FACE_OUTER_BOUND ( 'NONE', #51753, .T. ) ;
#5406=DIRECTION ( 'NONE',  ( 0.000000000000000000, -1.000000000000000000, 0.000000000000000000 ) ) ;
#5407=DIRECTION ( 'NONE',  ( 0.000000000000000000, 0.000000000000000000, 1.000000000000000000 ) ) ;
#5408=EDGE_LOOP ( 'NONE', ( #22235, #33553, #31997, #33040 ) ) ;
#5409=UNCERTAINTY_MEASURE_WITH_UNIT (LENGTH_MEASURE( 1.000000000000000082E-05 ), #30388, 'distance_accuracy_value', 'NONE');
#5410=AXIS2_PLACEMENT_3D ( 'NONE', #45356, #45104, #17229 ) ;
#5411=EDGE_CURVE ( 'NONE', #43356, #50666, #49781, .T. ) ;
#5412=VERTEX_POINT ( 'NONE', #18235 ) ;
#5414=ORIENTED_EDGE ( 'NONE', *, *, #50955, .F. ) ;
#5415=DIRECTION ( 'NONE',  ( 0.000000000000000000, 0.000000000000000000, 1.000000000000000000 ) ) ;
#5416=ORIENTED_EDGE ( 'NONE', *, *, #49738, .T. ) ;
#5417=LINE ( 'NONE', #37457, #600 ) ;
#5418=CARTESIAN_POINT ( 'NONE',  ( -114.9600645115007040, -193.5000000000000000, 105.8550183720738573 ) ) ;
#5420=FACE_OUTER_BOUND ( 'NONE', #30721, .T. ) ;
#5421=ORIENTED_EDGE ( 'NONE', *, *, #12784, .F. ) ;
#5422=LINE ( 'NONE', #5690, #1509 ) ;
#5423=ORIENTED_EDGE ( 'NONE', *, *, #8027, .F. ) ;
#5424=EDGE_CURVE ( 'NONE', #23290, #43364, #45832, .T. ) ;
#5425=ORIENTED_EDGE ( 'NONE', *, *, #41298, .T. ) ;
#5426=CYLINDRICAL_SURFACE ( 'NONE', #4448, 124.9999999999999858 ) ;
#5428=EDGE_LOOP ( 'NONE', ( #8463, #44744, #29369, #10462 ) ) ;
#5429=AXIS2_PLACEMENT_3D ( 'NONE', #37844, #48655, #17384 ) ;
#5430=AXIS2_PLACEMENT_3D ( 'NONE', #16273, #44126, #12051 ) ;
#5432=EDGE_CURVE ( 'NONE', #13401, #43754, #25580, .T. ) ;
#5433=DIRECTION ( 'NONE',  ( -0.000000000000000000, 1.000000000000000000, -0.000000000000000000 ) ) ;
#5434=EDGE_CURVE ( 'NONE', #43746, #8800, #49261, .T. ) ;
#5436=FACE_OUTER_BOUND ( 'NONE', #36883, .T. ) ;
#5437=EDGE_CURVE ( 'NONE', #32747, #5648, #13253, .T. ) ;
#5439=CIRCLE ( 'NONE', #12116, 125.0000000000000000 ) ;
#5440=EDGE_CURVE ( 'NONE', #10662, #41535, #38304, .T. ) ;
#5443=ORIENTED_EDGE ( 'NONE', *, *, #28532, .T. ) ;
#5444=EDGE_CURVE ( 'NONE', #8565, #25286, #13509, .T. ) ;
#5445=FACE_OUTER_BOUND ( 'NONE', #43971, .T. ) ;
#5447=FACE_OUTER_BOUND ( 'NONE', #9918, .T. ) ;
#5448=EDGE_CURVE ( 'NONE', #44462, #31730, #18215, .T. ) ;
#5451=EDGE_CURVE ( 'NONE', #11371, #27267, #50300, .T. ) ;
#5453=ADVANCED_FACE ( 'NONE', ( #14291 ), #21915, .F. ) ;
#5454=CARTESIAN_POINT ( 'NONE',  ( -29.73468717939733352, -183.6283474603465606, 123.5865930638411214 ) ) ;
#5455=CARTESIAN_POINT ( 'NONE',  ( -49.40581635894068313, -175.3837268820161057, -0.3758275821142418316 ) ) ;
#5456=ORIENTED_EDGE ( 'NONE', *, *, #9300, .F. ) ;
#5458=DIRECTION ( 'NONE',  ( 0.000000000000000000, 0.000000000000000000, 1.000000000000000000 ) ) ;
#5459=EDGE_LOOP ( 'NONE', ( #5048, #9096, #35272, #33423 ) ) ;
#5460=EDGE_LOOP ( 'NONE', ( #39614, #21710, #49628, #19288 ) ) ;
#5462=VERTEX_POINT ( 'NONE', #5898 ) ;
#5463=DIRECTION ( 'NONE',  ( 0.000000000000000000, 0.000000000000000000, 1.000000000000000000 ) ) ;
#5464=DIRECTION ( 'NONE',  ( -0.000000000000000000, 1.000000000000000000, -0.000000000000000000 ) ) ;
#5466=ORIENTED_EDGE ( 'NONE', *, *, #14048, .F. ) ;
#5468=AXIS2_PLACEMENT_3D ( 'NONE', #47416, #41727, #46923 ) ;
#5469=CARTESIAN_POINT ( 'NONE',  ( -5.732832253866456007, -189.7472609257535510, -117.4638425504666657 ) ) ;
#5470=DIRECTION ( 'NONE',  ( 0.000000000000000000, -1.000000000000000000, 0.000000000000000000 ) ) ;
#5471=ORIENTED_EDGE ( 'NONE', *, *, #18589, .F. ) ;
#5472=VECTOR ( 'NONE', #45970, 1000.000000000000000 ) ;
#5473=EDGE_CURVE ( 'NONE', #15110, #25409, #11631, .T. ) ;
#5474=VECTOR ( 'NONE', #23585, 1000.000000000000000 ) ;
#5475=EDGE_CURVE ( 'NONE', #12908, #49029, #23467, .T. ) ;
#5476=LINE ( 'NONE', #49364, #25652 ) ;
#5477=ORIENTED_EDGE ( 'NONE', *, *, #14101, .T. ) ;
#5481=VECTOR ( 'NONE', #50711, 1000.000000000000000 ) ;
#5482=EDGE_LOOP ( 'NONE', ( #32676, #1742, #46403, #31873 ) ) ;
#5483=CARTESIAN_POINT ( 'NONE',  ( 52.98246549829696050, -189.7472609257535510, 73.01058346660535392 ) ) ;
#5488=DIRECTION ( 'NONE',  ( 0.000000000000000000, -1.000000000000000000, 0.000000000000000000 ) ) ;
#5489=ORIENTED_EDGE ( 'NONE', *, *, #8679, .T. ) ;
#5490=PLANE ( 'NONE',  #32571 ) ;
#5491=AXIS2_PLACEMENT_3D ( 'NONE', #40733, #37060, #40218 ) ;
#5493=ORIENTED_EDGE ( 'NONE', *, *, #26912, .F. ) ;
#5494=CARTESIAN_POINT ( 'NONE',  ( 71.15591247552653442, -193.5000000000000000, 36.22785377504035154 ) ) ;
#5495=DIRECTION ( 'NONE',  ( 0.000000000000000000, 0.000000000000000000, 1.000000000000000000 ) ) ;
#5496=DIRECTION ( 'NONE',  ( -0.000000000000000000, 1.000000000000000000, -0.000000000000000000 ) ) ;
#5497=DIRECTION ( 'NONE',  ( 0.000000000000000000, 0.000000000000000000, -1.000000000000000000 ) ) ;
#5500=DIRECTION ( 'NONE',  ( -0.000000000000000000, 1.000000000000000000, -0.000000000000000000 ) ) ;
#5501=ADVANCED_FACE ( 'NONE', ( #10859 ), #23212, .T. ) ;
#5502=EDGE_CURVE ( 'NONE', #45026, #10698, #39229, .T. ) ;
#5504=DIRECTION ( 'NONE',  ( -0.5338233779648003940, 0.000000000000000000, 0.8455960035018199594 ) ) ;
#5505=ORIENTED_EDGE ( 'NONE', *, *, #16880, .T. ) ;
#5508=EDGE_CURVE ( 'NONE', #5830, #32508, #3237, .T. ) ;
#5509=DIRECTION ( 'NONE',  ( 0.000000000000000000, 0.000000000000000000, 1.000000000000000000 ) ) ;
#5510=ORIENTED_EDGE ( 'NONE', *, *, #9989, .T. ) ;
#5511=CIRCLE ( 'NONE', #1282, 125.0000000000000000 ) ;
#5512=VECTOR ( 'NONE', #2943, 1000.000000000000000 ) ;
#5514=CARTESIAN_POINT ( 'NONE',  ( -48.47912675150885065, -175.3837268820161057, 6.938893903907228378E-15 ) ) ;
#5515=DIRECTION ( 'NONE',  ( -0.9027978299657387629, 0.000000000000000000, -0.4300652022765304450 ) ) ;
#5517=ORIENTED_EDGE ( 'NONE', *, *, #14542, .T. ) ;
#5518=ORIENTED_EDGE ( 'NONE', *, *, #1824, .F. ) ;
#5519=VECTOR ( 'NONE', #35938, 1000.000000000000000 ) ;
#5521=DIRECTION ( 'NONE',  ( 0.5829794791144762289, 0.000000000000000000, -0.8124868780056783146 ) ) ;
#5522=VECTOR ( 'NONE', #15169, 1000.000000000000114 ) ;
#5524=FACE_OUTER_BOUND ( 'NONE', #36809, .T. ) ;
#5526=VECTOR ( 'NONE', #51236, 1000.000000000000227 ) ;
#5527=PLANE ( 'NONE',  #44497 ) ;
#5528=ORIENTED_EDGE ( 'NONE', *, *, #33302, .T. ) ;
#5529=EDGE_CURVE ( 'NONE', #47477, #47750, #46877, .T. ) ;
#5530=CARTESIAN_POINT ( 'NONE',  ( 74.60098876342242136, -177.1207230881787780, 21.82395850507348811 ) ) ;
#5532=CIRCLE ( 'NONE', #13043, 125.0000000000000000 ) ;
#5533=PLANE ( 'NONE',  #29241 ) ;
#5535=DIRECTION ( 'NONE',  ( 0.000000000000000000, -1.000000000000000000, 0.000000000000000000 ) ) ;
#5536=ORIENTED_EDGE ( 'NONE', *, *, #41761, .F. ) ;
#5537=CARTESIAN_POINT ( 'NONE',  ( -48.30223647638627682, -183.6283474603465606, -0.9842305779475897243 ) ) ;
#5541=ORIENTED_EDGE ( 'NONE', *, *, #2287, .T. ) ;
#5542=VECTOR ( 'NONE', #10519, 1000.000000000000000 ) ;
#5545=ORIENTED_EDGE ( 'NONE', *, *, #21761, .T. ) ;
#5549=CARTESIAN_POINT ( 'NONE',  ( -47.51449116960048968, -183.6283474603465606, 0.2635871660690785045 ) ) ;
#5551=CARTESIAN_POINT ( 'NONE',  ( -48.47912675150885065, -189.7472609257535510, 6.938893903907228378E-15 ) ) ;
#5553=ORIENTED_EDGE ( 'NONE', *, *, #49819, .T. ) ;
#5554=LINE ( 'NONE', #1067, #26549 ) ;
#5555=LINE ( 'NONE', #41269, #10217 ) ;
#5557=EDGE_LOOP ( 'NONE', ( #36293, #25069, #33914, #15885 ) ) ;
#5558=VECTOR ( 'NONE', #9093, 1000.000000000000000 ) ;
#5559=FACE_OUTER_BOUND ( 'NONE', #34033, .T. ) ;
#5561=DIRECTION ( 'NONE',  ( 0.000000000000000000, -1.000000000000000000, 0.000000000000000000 ) ) ;
#5562=VECTOR ( 'NONE', #22502, 1000.000000000000000 ) ;
#5563=LINE ( 'NONE', #33658, #14853 ) ;
#5564=ORIENTED_EDGE ( 'NONE', *, *, #8610, .T. ) ;
#5566=VECTOR ( 'NONE', #14978, 1000.000000000000000 ) ;
#5568=LINE ( 'NONE', #9245, #46615 ) ;
#5569=AXIS2_PLACEMENT_3D ( 'NONE', #4960, #48845, #20979 ) ;
#5572=CARTESIAN_POINT ( 'NONE',  ( 70.68712318874649725, -177.1207230881787780, -37.74128873232327663 ) ) ;
#5573=CYLINDRICAL_SURFACE ( 'NONE', #4292, 125.0000000000000000 ) ;
#5575=CARTESIAN_POINT ( 'NONE',  ( -48.47912675150885065, -175.3837268820161057, 6.938893903907228378E-15 ) ) ;
#5577=VECTOR ( 'NONE', #46162, 1000.000000000000000 ) ;
#5578=VECTOR ( 'NONE', #12460, 1000.000000000000000 ) ;
#5579=DIRECTION ( 'NONE',  ( 0.000000000000000000, 1.000000000000000000, -0.000000000000000000 ) ) ;
#5583=ORIENTED_EDGE ( 'NONE', *, *, #7892, .T. ) ;
#5584=CIRCLE ( 'NONE', #34919, 125.0000000000000000 ) ;
#5585=AXIS2_PLACEMENT_3D ( 'NONE', #22620, #38632, #47052 ) ;
#5586=VERTEX_POINT ( 'NONE', #43165 ) ;
#5587=CARTESIAN_POINT ( 'NONE',  ( -172.4422607493951318, -183.6283474603465606, 16.06677968424543579 ) ) ;
#5588=CARTESIAN_POINT ( 'NONE',  ( -47.60339180931321579, -175.3837268820161057, 0.4827922027307559594 ) ) ;
#5589=ORIENTED_EDGE ( 'NONE', *, *, #2595, .T. ) ;
#5590=AXIS2_PLACEMENT_3D ( 'NONE', #45310, #25070, #32681 ) ;
#5591=EDGE_LOOP ( 'NONE', ( #43211, #45296, #40113, #2197 ) ) ;
#5594=ADVANCED_FACE ( 'NONE', ( #2707 ), #7443, .T. ) ;
#5595=DIRECTION ( 'NONE',  ( -0.9960498426152165630, 0.000000000000000000, -0.08879589532293852283 ) ) ;
#5598=EDGE_CURVE ( 'NONE', #12133, #37972, #51327, .T. ) ;
#5599=DIRECTION ( 'NONE',  ( -0.000000000000000000, -0.000000000000000000, -1.000000000000000000 ) ) ;
#5600=CARTESIAN_POINT ( 'NONE',  ( -120.2975302769383177, -193.5000000000000000, 102.3089288139533863 ) ) ;
#5601=VERTEX_POINT ( 'NONE', #18745 ) ;
#5603=LINE ( 'NONE', #50772, #13497 ) ;
#5604=CARTESIAN_POINT ( 'NONE',  ( -0.6536498292959314060, -177.1207230881787780, 114.4068333132749160 ) ) ;
#5605=ORIENTED_EDGE ( 'NONE', *, *, #2319, .F. ) ;
#5606=CIRCLE ( 'NONE', #30625, 125.0000000000000000 ) ;
#5607=DIRECTION ( 'NONE',  ( 0.8124868780056783146, 0.000000000000000000, 0.5829794791144762289 ) ) ;
#5608=VERTEX_POINT ( 'NONE', #6914 ) ;
#5609=DIRECTION ( 'NONE',  ( 0.000000000000000000, -0.000000000000000000, 1.000000000000000000 ) ) ;
#5610=ORIENTED_EDGE ( 'NONE', *, *, #32127, .T. ) ;
#5611=CARTESIAN_POINT ( 'NONE',  ( -115.4536696835168641, -177.1207230881787780, -105.5434062319793185 ) ) ;
#5612=CARTESIAN_POINT ( 'NONE',  ( -47.82630463331833681, -193.5000000000000000, 0.7575112421616305713 ) ) ;
#5614=ADVANCED_FACE ( 'NONE', ( #47377 ), #18486, .T. ) ;
#5616=CIRCLE ( 'NONE', #34961, 125.0000000000000000 ) ;
#5617=ORIENTED_EDGE ( 'NONE', *, *, #17319, .F. ) ;
#5620=DIRECTION ( 'NONE',  ( 0.8757349421956345248, 0.000000000000000000, 0.4827922027307490205 ) ) ;
#5621=ORIENTED_EDGE ( 'NONE', *, *, #13741, .T. ) ;
#5622=CARTESIAN_POINT ( 'NONE',  ( 75.32224018181403835, -183.6283474603465606, 7.024906801079482399 ) ) ;
#5623=VECTOR ( 'NONE', #6841, 1000.000000000000000 ) ;
#5624=ORIENTED_EDGE ( 'NONE', *, *, #2149, .F. ) ;
#5625=EDGE_CURVE ( 'NONE', #14548, #37490, #43383, .T. ) ;
#5626=CARTESIAN_POINT ( 'NONE',  ( -96.30460367372252506, -177.1207230881787780, -114.4068333132746176 ) ) ;
#5629=EDGE_LOOP ( 'NONE', ( #22899, #38030, #37962, #5923, #47415, #25959, #8043, #1488 ) ) ;
#5630=LINE ( 'NONE', #14022, #24944 ) ;
#5632=AXIS2_PLACEMENT_3D ( 'NONE', #44312, #11716, #20637 ) ;
#5633=EDGE_CURVE ( 'NONE', #25704, #15236, #35029, .T. ) ;
#5634=CARTESIAN_POINT ( 'NONE',  ( -159.3947744408687868, -177.1207230881787780, -55.44293326708444880 ) ) ;
#5635=CIRCLE ( 'NONE', #3930, 125.0000000000000000 ) ;
#5637=EDGE_LOOP ( 'NONE', ( #37783, #3398, #18844, #15034 ) ) ;
#5641=FACE_OUTER_BOUND ( 'NONE', #4326, .T. ) ;
#5642=DIRECTION ( 'NONE',  ( 0.000000000000000000, 0.000000000000000000, 1.000000000000000000 ) ) ;
#5644=FACE_OUTER_BOUND ( 'NONE', #37064, .T. ) ;
#5645=ORIENTED_EDGE ( 'NONE', *, *, #19703, .T. ) ;
#5646=CARTESIAN_POINT ( 'NONE',  ( 10.73478887071927623, -193.5000000000000000, -110.0850225811106924 ) ) ;
#5648=VERTEX_POINT ( 'NONE', #10597 ) ;
#5649=EDGE_CURVE ( 'NONE', #27687, #38097, #26629, .T. ) ;
#5651=CARTESIAN_POINT ( 'NONE',  ( -148.6149069237406195, -177.1207230881787780, -74.81861753132355375 ) ) ;
#5652=VERTEX_POINT ( 'NONE', #15578 ) ;
#5654=CARTESIAN_POINT ( 'NONE',  ( -173.0003472773501301, -175.3837268820161057, 10.93003379476953363 ) ) ;
#5655=LINE ( 'NONE', #49010, #22906 ) ;
#5656=AXIS2_PLACEMENT_3D ( 'NONE', #2810, #50920, #14922 ) ;
#5657=VECTOR ( 'NONE', #42595, 1000.000000000000114 ) ;
#5658=ORIENTED_EDGE ( 'NONE', *, *, #8929, .F. ) ;
#5660=ORIENTED_EDGE ( 'NONE', *, *, #44539, .F. ) ;
#5661=DIRECTION ( 'NONE',  ( 0.000000000000000000, 0.000000000000000000, -1.000000000000000000 ) ) ;
#5662=LINE ( 'NONE', #30075, #45994 ) ;
#5663=AXIS2_PLACEMENT_3D ( 'NONE', #33160, #36853, #21078 ) ;
#5664=LINE ( 'NONE', #37706, #28615 ) ;
#5665=DIRECTION ( 'NONE',  ( 0.05924062789372142729, 0.000000000000000000, -0.9982437317643209074 ) ) ;
#5666=ORIENTED_EDGE ( 'NONE', *, *, #26885, .F. ) ;
#5670=DIRECTION ( 'NONE',  ( -0.08879589532294572540, 0.000000000000000000, 0.9960498426152160079 ) ) ;
#5672=VECTOR ( 'NONE', #3335, 1000.000000000000114 ) ;
#5673=CARTESIAN_POINT ( 'NONE',  ( -150.1390659022305840, -193.5000000000000000, 72.73415134496005408 ) ) ;
#5674=CARTESIAN_POINT ( 'NONE',  ( -173.4460699164830260, -189.7472609257535510, -2.874563619423225802 ) ) ;
#5676=EDGE_CURVE ( 'NONE', #22186, #47386, #40246, .T. ) ;
#5677=ADVANCED_FACE ( 'NONE', ( #15849 ), #57, .T. ) ;
#5680=VERTEX_POINT ( 'NONE', #23712 ) ;
#5681=CARTESIAN_POINT ( 'NONE',  ( 75.95066919219054569, -189.7472609257535510, -11.92584929509534852 ) ) ;
#5684=FACE_OUTER_BOUND ( 'NONE', #24849, .T. ) ;
#5686=LINE ( 'NONE', #50088, #17861 ) ;
#5687=DIRECTION ( 'NONE',  ( 0.000000000000000000, 1.000000000000000000, 0.000000000000000000 ) ) ;
#5688=EDGE_LOOP ( 'NONE', ( #17704, #42800, #33501, #1995 ) ) ;
#5690=CARTESIAN_POINT ( 'NONE',  ( 36.10886851198520731, -183.6283474603465606, 92.03190238880812046 ) ) ;
#5692=EDGE_CURVE ( 'NONE', #28453, #40339, #14849, .T. ) ;
#5699=EDGE_LOOP ( 'NONE', ( #23017, #27167, #41644, #2043 ) ) ;
#5700=AXIS2_PLACEMENT_3D ( 'NONE', #48762, #7769, #23797 ) ;
#5702=CARTESIAN_POINT ( 'NONE',  ( -48.47912675150885065, -189.7472609257535510, 6.938893903907228378E-15 ) ) ;
#5707=FACE_BOUND ( 'NONE', #317, .T. ) ;
#5708=EDGE_LOOP ( 'NONE', ( #4940, #41134, #29638, #12674 ) ) ;
#5711=ORIENTED_EDGE ( 'NONE', *, *, #27958, .F. ) ;
#5713=ORIENTED_EDGE ( 'NONE', *, *, #23669, .T. ) ;
#5714=CARTESIAN_POINT ( 'NONE',  ( -5.732832253866456007, -193.5000000000000000, -117.4638425504666657 ) ) ;
#5718=CARTESIAN_POINT ( 'NONE',  ( -49.25565061422690150, -193.5000000000000000, 0.6300878435817109935 ) ) ;
#5719=CARTESIAN_POINT ( 'NONE',  ( -139.0630283577175987, -177.1207230881787780, -86.13684908212448477 ) ) ;
#5720=ORIENTED_EDGE ( 'NONE', *, *, #6762, .T. ) ;
#5721=FACE_OUTER_BOUND ( 'NONE', #49848, .T. ) ;
#5722=ORIENTED_EDGE ( 'NONE', *, *, #45979, .F. ) ;
#5725=EDGE_CURVE ( 'NONE', #50565, #16442, #32367, .T. ) ;
#5726=CARTESIAN_POINT ( 'NONE',  ( -166.0019676197264005, -175.3837268820161057, 39.55227055146321646 ) ) ;
#5727=VECTOR ( 'NONE', #51066, 1000.000000000000000 ) ;
#5729=VECTOR ( 'NONE', #40351, 1000.000000000000000 ) ;
#5730=( NAMED_UNIT ( * ) SI_UNIT ( $, .STERADIAN. ) SOLID_ANGLE_UNIT ( ) );
#5731=CARTESIAN_POINT ( 'NONE',  ( -173.4190745413846457, -175.3837268820161057, -3.874202661594927211 ) ) ;
#5732=DIRECTION ( 'NONE',  ( 0.000000000000000000, 1.000000000000000000, -0.000000000000000000 ) ) ;
#5737=EDGE_CURVE ( 'NONE', #41712, #26081, #603, .T. ) ;
#5739=DIRECTION ( 'NONE',  ( 0.000000000000000000, 0.000000000000000000, -1.000000000000000000 ) ) ;
#5741=ORIENTED_EDGE ( 'NONE', *, *, #911, .F. ) ;
#5742=PLANE ( 'NONE',  #12203 ) ;
#5744=CIRCLE ( 'NONE', #44340, 125.0000000000000000 ) ;
#5745=ORIENTED_EDGE ( 'NONE', *, *, #39261, .F. ) ;
#5746=EDGE_CURVE ( 'NONE', #36146, #21174, #28421, .T. ) ;
#5747=VERTEX_POINT ( 'NONE', #48155 ) ;
#5748=DIRECTION ( 'NONE',  ( 0.000000000000000000, 0.000000000000000000, 1.000000000000000000 ) ) ;
#5751=DIRECTION ( 'NONE',  ( 0.000000000000000000, 0.000000000000000000, -1.000000000000000000 ) ) ;
#5752=CARTESIAN_POINT ( 'NONE',  ( 2.066935079424583765, -175.3837268820161057, -114.3245189510257802 ) ) ;
#5756=ORIENTED_EDGE ( 'NONE', *, *, #14737, .F. ) ;
#5760=CARTESIAN_POINT ( 'NONE',  ( -48.13092511607445800, -193.5000000000000000, 0.9374196611341301111 ) ) ;
#5763=LINE ( 'NONE', #28861, #36425 ) ;
#5768=ADVANCED_FACE ( 'NONE', ( #8207 ), #32636, .F. ) ;
#5771=DIRECTION ( 'NONE',  ( -0.000000000000000000, 1.000000000000000000, -0.000000000000000000 ) ) ;
#5772=ORIENTED_EDGE ( 'NONE', *, *, #19487, .F. ) ;
#5773=CARTESIAN_POINT ( 'NONE',  ( -48.88225018079680950, -189.7472609257535510, -0.9151456172430169067 ) ) ;
#5776=CARTESIAN_POINT ( 'NONE',  ( -169.9131040279660567, -183.6283474603465606, 29.64437826672833864 ) ) ;
#5779=ORIENTED_EDGE ( 'NONE', *, *, #27503, .F. ) ;
#5780=VECTOR ( 'NONE', #50346, 1000.000000000000000 ) ;
#5782=DIRECTION ( 'NONE',  ( 0.9473263538541923934, 0.000000000000000000, -0.3202698538628350744 ) ) ;
#5783=CIRCLE ( 'NONE', #14136, 125.0000000000000000 ) ;
#5785=DIRECTION ( 'NONE',  ( 0.000000000000000000, 0.000000000000000000, 1.000000000000000000 ) ) ;
#5787=LINE ( 'NONE', #46237, #8629 ) ;
#5788=ORIENTED_EDGE ( 'NONE', *, *, #37813, .T. ) ;
#5791=DIRECTION ( 'NONE',  ( 0.000000000000000000, -1.000000000000000000, 0.000000000000000000 ) ) ;
#5796=EDGE_LOOP ( 'NONE', ( #23948, #26673, #21207, #21353 ) ) ;
#5799=ORIENTED_EDGE ( 'NONE', *, *, #10845, .F. ) ;
#5800=DIRECTION ( 'NONE',  ( 0.000000000000000000, 1.000000000000000000, -0.000000000000000000 ) ) ;
#5802=LINE ( 'NONE', #21816, #49444 ) ;
#5804=VERTEX_POINT ( 'NONE', #18170 ) ;
#5805=EDGE_CURVE ( 'NONE', #12980, #23327, #50242, .T. ) ;
#5808=CARTESIAN_POINT ( 'NONE',  ( 46.40005841627164074, -177.1207230881787780, 81.38144888055276738 ) ) ;
#5810=ORIENTED_EDGE ( 'NONE', *, *, #23410, .F. ) ;
#5813=ORIENTED_EDGE ( 'NONE', *, *, #18036, .F. ) ;
#5814=AXIS2_PLACEMENT_3D ( 'NONE', #48143, #24227, #40236 ) ;
#5815=AXIS2_PLACEMENT_3D ( 'NONE', #33870, #5791, #29666 ) ;
#5816=CARTESIAN_POINT ( 'NONE',  ( 57.61256176024323139, -183.6283474603465606, -64.19309449102733822 ) ) ;
#5817=VERTEX_POINT ( 'NONE', #5845 ) ;
#5820=DIRECTION ( 'NONE',  ( 0.000000000000000000, -1.000000000000000000, 0.000000000000000000 ) ) ;
#5822=CYLINDRICAL_SURFACE ( 'NONE', #45160, 125.0000000000000000 ) ;
#5826=CARTESIAN_POINT ( 'NONE',  ( -44.48323084606168720, -177.1207230881787780, 123.9361149384469769 ) ) ;
#5828=CARTESIAN_POINT ( 'NONE',  ( -33.64434644548590825, -189.7472609257535510, -123.1094209424468033 ) ) ;
#5829=ADVANCED_FACE ( 'NONE', ( #25526 ), #49715, .T. ) ;
#5830=VERTEX_POINT ( 'NONE', #10034 ) ;
#5831=DIRECTION ( 'NONE',  ( 0.000000000000000000, 0.000000000000000000, 1.000000000000000000 ) ) ;
#5833=DIRECTION ( 'NONE',  ( 0.000000000000000000, -1.000000000000000000, 0.000000000000000000 ) ) ;
#5835=ORIENTED_EDGE ( 'NONE', *, *, #14105, .F. ) ;
#5836=DIRECTION ( 'NONE',  ( 0.9890401873221633666, 0.000000000000000000, 0.1476465640024850756 ) ) ;
#5837=CARTESIAN_POINT ( 'NONE',  ( -48.47912675150885065, -189.7472609257535510, 6.938893903907228378E-15 ) ) ;
#5838=EDGE_CURVE ( 'NONE', #23880, #49057, #26048, .T. ) ;
#5840=CARTESIAN_POINT ( 'NONE',  ( 0.7476021451244497795, -189.7472609257535510, -113.8100815915415609 ) ) ;
#5841=ORIENTED_EDGE ( 'NONE', *, *, #43762, .T. ) ;
#5843=CARTESIAN_POINT ( 'NONE',  ( 10.73478887071927623, -183.6283474603465606, -110.0850225811106924 ) ) ;
#5844=CARTESIAN_POINT ( 'NONE',  ( -22.44626007086657182, -177.1207230881787780, 122.2591094863196730 ) ) ;
#5845=CARTESIAN_POINT ( 'NONE',  ( -140.1460956102404509, -189.7472609257535510, 84.98333260264820410 ) ) ;
#5847=AXIS2_PLACEMENT_3D ( 'NONE', #28242, #44294, #36130 ) ;
#5848=DIRECTION ( 'NONE',  ( -0.05924062789372142729, 0.000000000000000000, 0.9982437317643209074 ) ) ;
#5849=LINE ( 'NONE', #28943, #30395 ) ;
#5850=FACE_OUTER_BOUND ( 'NONE', #15935, .T. ) ;
#5851=ORIENTED_EDGE ( 'NONE', *, *, #23597, .T. ) ;
#5852=VECTOR ( 'NONE', #3571, 1000.000000000000227 ) ;
#5855=DIRECTION ( 'NONE',  ( 0.000000000000000000, -0.000000000000000000, -1.000000000000000000 ) ) ;
#5856=VERTEX_POINT ( 'NONE', #49973 ) ;
#5858=ORIENTED_EDGE ( 'NONE', *, *, #25980, .F. ) ;
#5859=DIRECTION ( 'NONE',  ( 0.000000000000000000, -1.000000000000000000, 0.000000000000000000 ) ) ;
#5860=EDGE_CURVE ( 'NONE', #24862, #41328, #7332, .T. ) ;
#5862=CARTESIAN_POINT ( 'NONE',  ( 67.29303306501925874, -189.7472609257535510, 47.13604789772128356 ) ) ;
#5863=DIRECTION ( 'NONE',  ( 0.000000000000000000, 0.000000000000000000, -1.000000000000000000 ) ) ;
#5864=EDGE_LOOP ( 'NONE', ( #40634, #40989, #4096, #31975 ) ) ;
#5867=DIRECTION ( 'NONE',  ( -0.000000000000000000, -1.000000000000000000, 0.000000000000000000 ) ) ;
#5869=CARTESIAN_POINT ( 'NONE',  ( -48.88225018079680950, -175.3837268820161057, -0.9151456172430169067 ) ) ;
#5870=ORIENTED_EDGE ( 'NONE', *, *, #42970, .T. ) ;
#5871=CARTESIAN_POINT ( 'NONE',  ( 73.62243227112294619, -183.6283474603465606, 21.61797988633237821 ) ) ;
#5872=EDGE_LOOP ( 'NONE', ( #29122, #3420, #37191, #10143 ) ) ;
#5874=DIRECTION ( 'NONE',  ( -0.5586467658036594619, 0.000000000000000000, 0.8294056854501971054 ) ) ;
#5875=CARTESIAN_POINT ( 'NONE',  ( 12.12533326292401803, -183.6283474603465606, 109.3256576763158989 ) ) ;
#5876=ORIENTED_EDGE ( 'NONE', *, *, #25336, .F. ) ;
#5877=VERTEX_POINT ( 'NONE', #6088 ) ;
#5878=DIRECTION ( 'NONE',  ( -0.9646355819083614058, 0.000000000000000000, 0.2635871660690581320 ) ) ;
#5879=DIRECTION ( 'NONE',  ( -0.000000000000000000, 1.000000000000000000, 0.000000000000000000 ) ) ;
#5880=AXIS2_PLACEMENT_3D ( 'NONE', #46493, #21550, #25743 ) ;
#5883=PLANE ( 'NONE',  #1370 ) ;
#5885=FACE_OUTER_BOUND ( 'NONE', #25999, .T. ) ;
#5886=DIRECTION ( 'NONE',  ( 0.000000000000000000, 1.000000000000000000, -0.000000000000000000 ) ) ;
#5887=ADVANCED_FACE ( 'NONE', ( #38123 ), #17138, .T. ) ;
#5892=DIRECTION ( 'NONE',  ( -0.000000000000000000, 1.000000000000000000, 0.000000000000000000 ) ) ;
#5894=DIRECTION ( 'NONE',  ( 0.000000000000000000, 0.000000000000000000, 1.000000000000000000 ) ) ;
#5898=CARTESIAN_POINT ( 'NONE',  ( -171.5708553757489767, -183.6283474603465606, 14.98512977653254019 ) ) ;
#5899=ADVANCED_FACE ( 'NONE', ( #29464 ), #45514, .F. ) ;
#5902=EDGE_LOOP ( 'NONE', ( #16328, #46896, #49280, #41571 ) ) ;
#5903=CIRCLE ( 'NONE', #37878, 125.0000000000000000 ) ;
#5904=CARTESIAN_POINT ( 'NONE',  ( 38.46761263173351608, -193.5000000000000000, 89.80681772907068705 ) ) ;
#5905=ORIENTED_EDGE ( 'NONE', *, *, #13377, .F. ) ;
#5906=LINE ( 'NONE', #4868, #47117 ) ;
#5908=ORIENTED_EDGE ( 'NONE', *, *, #30592, .F. ) ;
#5909=EDGE_LOOP ( 'NONE', ( #34115, #14262, #26160, #23981 ) ) ;
#5910=EDGE_CURVE ( 'NONE', #512, #46176, #44239, .T. ) ;
#5912=ORIENTED_EDGE ( 'NONE', *, *, #22122, .T. ) ;
#5915=ORIENTED_EDGE ( 'NONE', *, *, #3695, .T. ) ;
#5919=EDGE_CURVE ( 'NONE', #15614, #10929, #20759, .T. ) ;
#5921=CYLINDRICAL_SURFACE ( 'NONE', #41664, 125.0000000000000000 ) ;
#5923=ORIENTED_EDGE ( 'NONE', *, *, #44958, .F. ) ;
#5924=ORIENTED_EDGE ( 'NONE', *, *, #41680, .T. ) ;
#5928=DIRECTION ( 'NONE',  ( -0.1182731709213523247, 0.000000000000000000, -0.9929810960135185827 ) ) ;
#5929=DIRECTION ( 'NONE',  ( -0.000000000000000000, 1.000000000000000000, -0.000000000000000000 ) ) ;
#5932=AXIS2_PLACEMENT_3D ( 'NONE', #38122, #25793, #49972 ) ;
#5933=ORIENTED_EDGE ( 'NONE', *, *, #41670, .F. ) ;
#5934=CARTESIAN_POINT ( 'NONE',  ( -170.6250538923603131, -189.7472609257535510, 26.55884942729648657 ) ) ;
#5945=DIRECTION ( 'NONE',  ( 0.6068001458185890984, 0.000000000000000000, 0.7948544414133565938 ) ) ;
#5946=CIRCLE ( 'NONE', #9278, 125.0000000000000000 ) ;
#5947=CARTESIAN_POINT ( 'NONE',  ( -49.47868758801764955, -175.3837268820161057, -0.02963332782256313663 ) ) ;
#5948=ORIENTED_EDGE ( 'NONE', *, *, #27503, .T. ) ;
#5949=CARTESIAN_POINT ( 'NONE',  ( -165.7578939544008847, -193.5000000000000000, -43.25148278810626579 ) ) ;
#5950=FACE_OUTER_BOUND ( 'NONE', #28430, .T. ) ;
#5951=CARTESIAN_POINT ( 'NONE',  ( -130.2106798473772642, -193.5000000000000000, 94.57776286494217288 ) ) ;
#5952=PLANE ( 'NONE',  #29069 ) ;
#5953=DIRECTION ( 'NONE',  ( 0.4031234292879730674, 0.000000000000000000, -0.9151456172430181280 ) ) ;
#5957=ORIENTED_EDGE ( 'NONE', *, *, #1216, .T. ) ;
#5958=AXIS2_PLACEMENT_3D ( 'NONE', #22107, #37867, #42321 ) ;
#5961=LINE ( 'NONE', #1493, #31322 ) ;
#5962=ORIENTED_EDGE ( 'NONE', *, *, #41022, .F. ) ;
#5963=CARTESIAN_POINT ( 'NONE',  ( -48.02249751411513756, -193.5000000000000000, -0.8896570909947397743 ) ) ;
#5965=DIRECTION ( 'NONE',  ( 0.000000000000000000, -1.000000000000000000, -0.000000000000000000 ) ) ;
#5966=ORIENTED_EDGE ( 'NONE', *, *, #24240, .F. ) ;
#5967=EDGE_CURVE ( 'NONE', #21665, #9485, #51517, .T. ) ;
#5971=ORIENTED_EDGE ( 'NONE', *, *, #23297, .T. ) ;
#5972=EDGE_CURVE ( 'NONE', #3044, #28776, #39209, .T. ) ;
#5973=ORIENTED_EDGE ( 'NONE', *, *, #11033, .T. ) ;
#5974=DIRECTION ( 'NONE',  ( 0.000000000000000000, 0.000000000000000000, -1.000000000000000000 ) ) ;
#5976=ADVANCED_FACE ( 'NONE', ( #2905 ), #43376, .T. ) ;
#5977=CIRCLE ( 'NONE', #45409, 125.0000000000000000 ) ;
#5978=LINE ( 'NONE', #49864, #13374 ) ;
#5980=CARTESIAN_POINT ( 'NONE',  ( 2.266533711611414148, -193.5000000000000000, 113.1409892739925596 ) ) ;
#5981=ORIENTED_EDGE ( 'NONE', *, *, #1517, .T. ) ;
#5982=DIRECTION ( 'NONE',  ( 0.000000000000000000, 0.000000000000000000, 1.000000000000000000 ) ) ;
#5983=ORIENTED_EDGE ( 'NONE', *, *, #47689, .F. ) ;
#5984=DIRECTION ( 'NONE',  ( -0.000000000000000000, 1.000000000000000000, 0.000000000000000000 ) ) ;
#5985=ORIENTED_EDGE ( 'NONE', *, *, #16336, .F. ) ;
#5986=ORIENTED_EDGE ( 'NONE', *, *, #22939, .F. ) ;
#5987=ORIENTED_EDGE ( 'NONE', *, *, #34275, .T. ) ;
#5989=VECTOR ( 'NONE', #6211, 1000.000000000000227 ) ;
#5990=VERTEX_POINT ( 'NONE', #51270 ) ;
#5992=CARTESIAN_POINT ( 'NONE',  ( 75.78974234412359579, -183.6283474603465606, 13.49993235881448861 ) ) ;
#5993=ORIENTED_EDGE ( 'NONE', *, *, #51545, .T. ) ;
#5995=ORIENTED_EDGE ( 'NONE', *, *, #13016, .T. ) ;
#5997=VERTEX_POINT ( 'NONE', #23404 ) ;
#5998=LINE ( 'NONE', #14405, #51429 ) ;
#6000=CARTESIAN_POINT ( 'NONE',  ( 116.9235303384055840, -213.5000000000000000, -9.999999999999971578 ) ) ;
#6002=ORIENTED_EDGE ( 'NONE', *, *, #38659, .T. ) ;
#6004=CARTESIAN_POINT ( 'NONE',  ( -48.47912675150885065, -189.7472609257535510, 6.938893903907228378E-15 ) ) ;
#6005=CARTESIAN_POINT ( 'NONE',  ( -150.5816505765687907, -177.1207230881787780, 70.36529243996407956 ) ) ;
#6007=ORIENTED_EDGE ( 'NONE', *, *, #34256, .T. ) ;
#6010=VECTOR ( 'NONE', #45986, 1000.000000000000000 ) ;
#6011=DIRECTION ( 'NONE',  ( 0.2348860457809707758, 0.000000000000000000, 0.9720229140804138579 ) ) ;
#6012=ORIENTED_EDGE ( 'NONE', *, *, #49755, .F. ) ;
#6013=ORIENTED_EDGE ( 'NONE', *, *, #28931, .F. ) ;
#6014=VECTOR ( 'NONE', #48439, 1000.000000000000114 ) ;
#6016=EDGE_CURVE ( 'NONE', #33758, #2870, #23148, .T. ) ;
#6017=DIRECTION ( 'NONE',  ( -0.000000000000000000, 1.000000000000000000, 0.000000000000000000 ) ) ;
#6018=LINE ( 'NONE', #41765, #46306 ) ;
#6019=EDGE_CURVE ( 'NONE', #44261, #1781, #31270, .T. ) ;
#6021=ADVANCED_FACE ( 'NONE', ( #3418 ), #10278, .F. ) ;
#6022=LINE ( 'NONE', #22042, #48060 ) ;
#6025=DIRECTION ( 'NONE',  ( -0.000000000000000000, 1.000000000000000000, -0.000000000000000000 ) ) ;
#6026=EDGE_CURVE ( 'NONE', #4313, #48860, #7113, .T. ) ;
#6028=CARTESIAN_POINT ( 'NONE',  ( -160.9694636715425702, -189.7472609257535510, 54.50618404931040573 ) ) ;
#6030=AXIS2_PLACEMENT_3D ( 'NONE', #9566, #25584, #37416 ) ;
#6032=EDGE_CURVE ( 'NONE', #25657, #19312, #15517, .T. ) ;
#6033=VECTOR ( 'NONE', #41412, 1000.000000000000000 ) ;
#6034=LINE ( 'NONE', #17615, #16793 ) ;
#6036=ADVANCED_FACE ( 'NONE', ( #26297 ), #6344, .T. ) ;
#6038=DIRECTION ( 'NONE',  ( 0.8124868780056863082, 0.000000000000000000, -0.5829794791144649047 ) ) ;
#6041=EDGE_CURVE ( 'NONE', #17251, #51869, #34448, .T. ) ;
#6042=ORIENTED_EDGE ( 'NONE', *, *, #35216, .F. ) ;
#6043=FACE_OUTER_BOUND ( 'NONE', #37908, .T. ) ;
#6045=VECTOR ( 'NONE', #17985, 1000.000000000000114 ) ;
#6046=CARTESIAN_POINT ( 'NONE',  ( -98.10897907742933910, -175.3837268820161057, 114.7252272087849434 ) ) ;
#6047=CARTESIAN_POINT ( 'NONE',  ( -172.2289551866394106, -189.7472609257535510, -17.63462396184710101 ) ) ;
#6051=VERTEX_POINT ( 'NONE', #47839 ) ;
#6052=AXIS2_PLACEMENT_3D ( 'NONE', #45526, #50253, #26315 ) ;
#6053=AXIS2_PLACEMENT_3D ( 'NONE', #10948, #19608, #2795 ) ;
#6054=FACE_OUTER_BOUND ( 'NONE', #49791, .T. ) ;
#6055=VERTEX_POINT ( 'NONE', #16286 ) ;
#6063=ORIENTED_EDGE ( 'NONE', *, *, #27934, .F. ) ;
#6064=CARTESIAN_POINT ( 'NONE',  ( -155.4465502054561057, -193.5000000000000000, 64.67588669375881238 ) ) ;
#6065=ORIENTED_EDGE ( 'NONE', *, *, #21870, .T. ) ;
#6067=LINE ( 'NONE', #42828, #45827 ) ;
#6068=ORIENTED_EDGE ( 'NONE', *, *, #245, .T. ) ;
#6069=FACE_OUTER_BOUND ( 'NONE', #5335, .T. ) ;
#6071=DIRECTION ( 'NONE',  ( -0.000000000000000000, -1.000000000000000000, 0.000000000000000000 ) ) ;
#6073=VECTOR ( 'NONE', #13512, 1000.000000000000227 ) ;
#6075=ORIENTED_EDGE ( 'NONE', *, *, #49419, .F. ) ;
#6077=DIRECTION ( 'NONE',  ( 0.000000000000000000, -1.000000000000000000, 0.000000000000000000 ) ) ;
#6078=CARTESIAN_POINT ( 'NONE',  ( -124.1938582159088327, -175.3837268820161057, -99.45993886622791536 ) ) ;
#6081=DIRECTION ( 'NONE',  ( 0.000000000000000000, 1.000000000000000000, -0.000000000000000000 ) ) ;
#6082=ORIENTED_EDGE ( 'NONE', *, *, #896, .T. ) ;
#6086=CYLINDRICAL_SURFACE ( 'NONE', #15979, 125.0000000000000000 ) ;
#6087=EDGE_CURVE ( 'NONE', #21890, #36336, #36785, .T. ) ;
#6088=CARTESIAN_POINT ( 'NONE',  ( -23.25236516653335528, -177.1207230881787780, -121.4073237908566654 ) ) ;
#6092=EDGE_CURVE ( 'NONE', #6218, #41928, #4207, .T. ) ;
#6094=CIRCLE ( 'NONE', #32065, 125.0000000000000000 ) ;
#6096=CARTESIAN_POINT ( 'NONE',  ( -149.3265790242249125, -189.7472609257535510, 72.15117186584561182 ) ) ;
#6098=PLANE ( 'NONE',  #3579 ) ;
#6099=FACE_OUTER_BOUND ( 'NONE', #5207, .T. ) ;
#6100=VERTEX_POINT ( 'NONE', #502 ) ;
#6103=ADVANCED_FACE ( 'NONE', ( #8657 ), #36004, .T. ) ;
#6104=CARTESIAN_POINT ( 'NONE',  ( -165.7578939544008847, -183.6283474603465606, -43.25148278810625868 ) ) ;
#6106=ORIENTED_EDGE ( 'NONE', *, *, #14754, .T. ) ;
#6107=ORIENTED_EDGE ( 'NONE', *, *, #32288, .T. ) ;
#6112=EDGE_CURVE ( 'NONE', #19096, #37383, #28094, .T. ) ;
#6113=CARTESIAN_POINT ( 'NONE',  ( 64.46023522152407281, -183.6283474603465606, -51.19472891551279758 ) ) ;
#6114=CARTESIAN_POINT ( 'NONE',  ( -55.71438232577004612, -189.7472609257535510, -124.7904286264580662 ) ) ;
#6115=EDGE_LOOP ( 'NONE', ( #44521, #33852, #47178, #1692 ) ) ;
#6116=ADVANCED_FACE ( 'NONE', ( #32575 ), #44667, .T. ) ;
#6117=VECTOR ( 'NONE', #4215, 1000.000000000000000 ) ;
#6124=EDGE_LOOP ( 'NONE', ( #18334, #13747, #35732, #49886 ) ) ;
#6126=VERTEX_POINT ( 'NONE', #40698 ) ;
#6128=LINE ( 'NONE', #34234, #20429 ) ;
#6129=DIRECTION ( 'NONE',  ( 0.000000000000000000, -0.000000000000000000, 1.000000000000000000 ) ) ;
#6130=AXIS2_PLACEMENT_3D ( 'NONE', #21216, #5196, #21735 ) ;
#6131=ADVANCED_FACE ( 'NONE', ( #2 ), #4722, .T. ) ;
#6132=AXIS2_PLACEMENT_3D ( 'NONE', #15393, #35873, #47718 ) ;
#6135=CIRCLE ( 'NONE', #42192, 125.0000000000000000 ) ;
#6136=CARTESIAN_POINT ( 'NONE',  ( -48.47912675150885065, -177.1207230881787780, 6.938893903907228378E-15 ) ) ;
#6137=CARTESIAN_POINT ( 'NONE',  ( 76.28370911321320591, -183.6283474603465606, -7.696413904697499753 ) ) ;
#6138=ORIENTED_EDGE ( 'NONE', *, *, #26102, .T. ) ;
#6140=ORIENTED_EDGE ( 'NONE', *, *, #5434, .T. ) ;
#6146=PLANE ( 'NONE',  #4626 ) ;
#6147=CARTESIAN_POINT ( 'NONE',  ( -48.47912675150885065, -183.6283474603465606, 6.938893903907228378E-15 ) ) ;
#6149=AXIS2_PLACEMENT_3D ( 'NONE', #11681, #15378, #27181 ) ;
#6151=DIRECTION ( 'NONE',  ( -0.000000000000000000, 1.000000000000000000, -0.000000000000000000 ) ) ;
#6152=CARTESIAN_POINT ( 'NONE',  ( -48.47912675150885065, -177.1207230881787780, 6.938893903907228378E-15 ) ) ;
#6153=DIRECTION ( 'NONE',  ( 0.000000000000000000, 1.000000000000000000, 0.000000000000000000 ) ) ;
#6154=EDGE_CURVE ( 'NONE', #2312, #16397, #49653, .T. ) ;
#6158=CARTESIAN_POINT ( 'NONE',  ( 26.52087324849106054, -198.5000000000000000, -80.00000000000002842 ) ) ;
#6159=LINE ( 'NONE', #18242, #23048 ) ;
#6160=CARTESIAN_POINT ( 'NONE',  ( -169.1033029113419559, -175.3837268820161057, 32.78426643622745473 ) ) ;
#6161=ORIENTED_EDGE ( 'NONE', *, *, #27908, .F. ) ;
#6163=DIRECTION ( 'NONE',  ( -0.1768902751225666370, 0.000000000000000000, -0.9842305779475979399 ) ) ;
#6165=AXIS2_PLACEMENT_3D ( 'NONE', #39032, #38263, #14117 ) ;
#6167=AXIS2_PLACEMENT_3D ( 'NONE', #25445, #5227, #17575 ) ;
#6168=ORIENTED_EDGE ( 'NONE', *, *, #51976, .T. ) ;
#6171=ORIENTED_EDGE ( 'NONE', *, *, #26989, .F. ) ;
#6172=DIRECTION ( 'NONE',  ( 0.9995608365087944591, 0.000000000000000000, -0.02963332782255633305 ) ) ;
#6174=AXIS2_PLACEMENT_3D ( 'NONE', #19339, #42979, #6989 ) ;
#6176=CARTESIAN_POINT ( 'NONE',  ( -48.18706998087187543, -193.5000000000000000, -0.9564009842765152092 ) ) ;
#6177=VERTEX_POINT ( 'NONE', #5252 ) ;
#6178=EDGE_LOOP ( 'NONE', ( #43143, #331, #21252, #28782 ) ) ;
#6180=ORIENTED_EDGE ( 'NONE', *, *, #18626, .F. ) ;
#6182=DIRECTION ( 'NONE',  ( 0.5586467658036535777, 0.000000000000000000, -0.8294056854502011022 ) ) ;
#6183=FACE_OUTER_BOUND ( 'NONE', #14576, .T. ) ;
#6184=DIRECTION ( 'NONE',  ( 0.9027978299657416494, 0.000000000000000000, 0.4300652022765245608 ) ) ;
#6186=ORIENTED_EDGE ( 'NONE', *, *, #15462, .F. ) ;
#6187=CARTESIAN_POINT ( 'NONE',  ( -48.47912675150885065, -177.1207230881787780, 6.938893903907228378E-15 ) ) ;
#6188=AXIS2_PLACEMENT_3D ( 'NONE', #13207, #29225, #45283 ) ;
#6194=DIRECTION ( 'NONE',  ( 0.000000000000000000, 0.000000000000000000, 1.000000000000000000 ) ) ;
#6196=ORIENTED_EDGE ( 'NONE', *, *, #47444, .T. ) ;
#6197=DIRECTION ( 'NONE',  ( -0.000000000000000000, 1.000000000000000000, -0.000000000000000000 ) ) ;
#6199=VERTEX_POINT ( 'NONE', #42006 ) ;
#6200=APPLICATION_CONTEXT ( 'automotive_design' ) ;
#6201=ORIENTED_EDGE ( 'NONE', *, *, #27233, .T. ) ;
#6203=CIRCLE ( 'NONE', #28826, 125.0000000000000000 ) ;
#6204=DIRECTION ( 'NONE',  ( -0.3482016354344059095, 0.000000000000000000, 0.9374196611341183427 ) ) ;
#6205=ORIENTED_EDGE ( 'NONE', *, *, #19554, .T. ) ;
#6206=LINE ( 'NONE', #30112, #38244 ) ;
#6207=DIRECTION ( 'NONE',  ( -0.000000000000000000, 1.000000000000000000, -0.000000000000000000 ) ) ;
#6208=CARTESIAN_POINT ( 'NONE',  ( -47.47956591500005885, -177.1207230881787780, -0.02963332782254939762 ) ) ;
#6209=EDGE_CURVE ( 'NONE', #28959, #36297, #22754, .T. ) ;
#6211=DIRECTION ( 'NONE',  ( -0.9473263538541876194, 0.000000000000000000, -0.3202698538628486746 ) ) ;
#6214=EDGE_LOOP ( 'NONE', ( #26053, #2053, #15278, #27777 ) ) ;
#6215=VECTOR ( 'NONE', #14669, 1000.000000000000000 ) ;
#6216=EDGE_LOOP ( 'NONE', ( #25405, #31444, #45804, #28110 ) ) ;
#6218=VERTEX_POINT ( 'NONE', #29402 ) ;
#6223=EDGE_CURVE ( 'NONE', #16369, #38638, #25731, .T. ) ;
#6224=ORIENTED_EDGE ( 'NONE', *, *, #73, .T. ) ;
#6230=ORIENTED_EDGE ( 'NONE', *, *, #43566, .F. ) ;
#6231=VERTEX_POINT ( 'NONE', #12855 ) ;
#6232=DIRECTION ( 'NONE',  ( -0.4031234292879600778, 0.000000000000000000, -0.9151456172430237901 ) ) ;
#6233=LINE ( 'NONE', #18327, #817 ) ;
#6234=FILL_AREA_STYLE_COLOUR ( '', #20076 ) ;
#6235=CYLINDRICAL_SURFACE ( 'NONE', #27005, 125.0000000000000000 ) ;
#6236=DIRECTION ( 'NONE',  ( 0.000000000000000000, 1.000000000000000000, 0.000000000000000000 ) ) ;
#6238=CARTESIAN_POINT ( 'NONE',  ( 32.49319223169170101, -175.3837268820161057, -95.22858582633061530 ) ) ;
#6239=ORIENTED_EDGE ( 'NONE', *, *, #28044, .T. ) ;
#6240=LINE ( 'NONE', #33578, #49143 ) ;
#6241=ORIENTED_EDGE ( 'NONE', *, *, #14748, .F. ) ;
#6242=VERTEX_POINT ( 'NONE', #9194 ) ;
#6243=DIRECTION ( 'NONE',  ( -0.000000000000000000, 1.000000000000000000, -0.000000000000000000 ) ) ;
#6244=EDGE_LOOP ( 'NONE', ( #2808, #40411, #9999, #22379 ) ) ;
#6248=CIRCLE ( 'NONE', #8747, 125.0000000000000000 ) ;
#6249=ADVANCED_FACE ( 'NONE', ( #21011 ), #4995, .T. ) ;
#6253=PLANE ( 'NONE',  #12378 ) ;
#6256=EDGE_CURVE ( 'NONE', #9002, #26704, #6018, .T. ) ;
#6258=LINE ( 'NONE', #2321, #27052 ) ;
#6259=DIRECTION ( 'NONE',  ( -0.000000000000000000, 1.000000000000000000, -0.000000000000000000 ) ) ;
#6260=CARTESIAN_POINT ( 'NONE',  ( -48.18706998087188254, -175.3837268820161057, 0.9564009842765313074 ) ) ;
#6261=ORIENTED_EDGE ( 'NONE', *, *, #33950, .F. ) ;
#6263=DIRECTION ( 'NONE',  ( 0.000000000000000000, 0.000000000000000000, -1.000000000000000000 ) ) ;
#6265=CARTESIAN_POINT ( 'NONE',  ( 63.54086012517504400, -193.5000000000000000, -53.17445600718543375 ) ) ;
#6267=ADVANCED_FACE ( 'NONE', ( #28877 ), #1559, .T. ) ;
#6268=EDGE_LOOP ( 'NONE', ( #46821, #26961, #16458, #9514 ) ) ;
#6270=DIRECTION ( 'NONE',  ( -0.000000000000000000, 1.000000000000000000, -0.000000000000000000 ) ) ;
#6272=EDGE_CURVE ( 'NONE', #49461, #3029, #33865, .T. ) ;
#6273=DIRECTION ( 'NONE',  ( 0.000000000000000000, -1.000000000000000000, -0.000000000000000000 ) ) ;
#6274=EDGE_LOOP ( 'NONE', ( #37030, #18109, #31849, #45930 ) ) ;
#6276=CARTESIAN_POINT ( 'NONE',  ( -172.4295958414655274, -175.3837268820161057, 3.504489105735777432 ) ) ;
#6278=DIRECTION ( 'NONE',  ( 0.9995608365087940150, 0.000000000000000000, 0.02963332782257007206 ) ) ;
#6279=ORIENTED_EDGE ( 'NONE', *, *, #45493, .T. ) ;
#6280=DIRECTION ( 'NONE',  ( 0.000000000000000000, 0.000000000000000000, 1.000000000000000000 ) ) ;
#6284=LINE ( 'NONE', #23085, #11987 ) ;
#6285=EDGE_CURVE ( 'NONE', #29184, #10769, #37053, .T. ) ;
#6287=VECTOR ( 'NONE', #5500, 1000.000000000000000 ) ;
#6292=DIRECTION ( 'NONE',  ( -0.000000000000000000, 1.000000000000000000, -0.000000000000000000 ) ) ;
#6293=EDGE_LOOP ( 'NONE', ( #40979, #41856, #10012, #10206 ) ) ;
#6294=CARTESIAN_POINT ( 'NONE',  ( -172.2289551866394106, -189.7472609257535510, -17.63462396184707970 ) ) ;
#6295=ORIENTED_EDGE ( 'NONE', *, *, #12471, .T. ) ;
#6296=AXIS2_PLACEMENT_3D ( 'NONE', #50977, #27031, #39624 ) ;
#6298=VECTOR ( 'NONE', #43472, 999.9999999999998863 ) ;
#6299=LINE ( 'NONE', #22317, #8258 ) ;
#6300=PRODUCT_DEFINITION_SHAPE ( 'NONE', 'NONE',  #34451 ) ;
#6302=VERTEX_POINT ( 'NONE', #49402 ) ;
#6304=CARTESIAN_POINT ( 'NONE',  ( 6.039888445539280504, -177.1207230881787780, 111.3726929437940498 ) ) ;
#6306=FACE_OUTER_BOUND ( 'NONE', #42503, .T. ) ;
#6307=ORIENTED_EDGE ( 'NONE', *, *, #12124, .F. ) ;
#6310=EDGE_CURVE ( 'NONE', #47750, #19173, #13386, .T. ) ;
#6311=EDGE_CURVE ( 'NONE', #15743, #32651, #21537, .T. ) ;
#6313=DIRECTION ( 'NONE',  ( 0.000000000000000000, 0.000000000000000000, 1.000000000000000000 ) ) ;
#6314=CARTESIAN_POINT ( 'NONE',  ( 56.77503207194101265, -189.7472609257535510, -67.42819922234311036 ) ) ;
#6316=ORIENTED_EDGE ( 'NONE', *, *, #807, .F. ) ;
#6318=ORIENTED_EDGE ( 'NONE', *, *, #31762, .F. ) ;
#6319=CARTESIAN_POINT ( 'NONE',  ( -147.6585554144535024, -177.1207230881787780, 76.08180419845386666 ) ) ;
#6320=VECTOR ( 'NONE', #25076, 1000.000000000000000 ) ;
#6321=LINE ( 'NONE', #34431, #18137 ) ;
#6322=ORIENTED_EDGE ( 'NONE', *, *, #26528, .F. ) ;
#6323=LINE ( 'NONE', #14726, #10436 ) ;
#6324=CARTESIAN_POINT ( 'NONE',  ( -49.32472275501067571, -183.6283474603465606, -0.5338233779647935107 ) ) ;
#6325=FACE_OUTER_BOUND ( 'NONE', #29148, .T. ) ;
#6326=DIRECTION ( 'NONE',  ( 0.000000000000000000, 1.000000000000000000, 0.000000000000000000 ) ) ;
#6327=CIRCLE ( 'NONE', #35678, 125.0000000000000000 ) ;
#6328=DIRECTION ( 'NONE',  ( 0.000000000000000000, 0.000000000000000000, 1.000000000000000000 ) ) ;
#6329=VERTEX_POINT ( 'NONE', #37807 ) ;
#6330=EDGE_CURVE ( 'NONE', #9868, #11130, #48820, .T. ) ;
#6331=DIRECTION ( 'NONE',  ( -0.000000000000000000, 1.000000000000000000, 0.000000000000000000 ) ) ;
#6332=CARTESIAN_POINT ( 'NONE',  ( -53.47502265695602119, -183.6283474603465606, -124.9001241957025883 ) ) ;
#6334=ADVANCED_FACE ( 'NONE', ( #48880 ), #39298, .T. ) ;
#6335=DIRECTION ( 'NONE',  ( 0.000000000000000000, 0.000000000000000000, 1.000000000000000000 ) ) ;
#6336=EDGE_LOOP ( 'NONE', ( #50130, #36327, #5345, #50659 ) ) ;
#6338=DIRECTION ( 'NONE',  ( -0.9720229140804107493, 0.000000000000000000, -0.2348860457809842095 ) ) ;
#6340=VECTOR ( 'NONE', #27225, 1000.000000000000000 ) ;
#6341=AXIS2_PLACEMENT_3D ( 'NONE', #31093, #35048, #7188 ) ;
#6343=DIRECTION ( 'NONE',  ( 0.000000000000000000, 0.000000000000000000, 1.000000000000000000 ) ) ;
#6344=CYLINDRICAL_SURFACE ( 'NONE', #31668, 125.0000000000000000 ) ;
#6346=VECTOR ( 'NONE', #5023, 1000.000000000000000 ) ;
#6347=CARTESIAN_POINT ( 'NONE',  ( -48.47912675150885065, -175.3837268820161057, 6.938893903907228378E-15 ) ) ;
#6349=DIRECTION ( 'NONE',  ( -0.000000000000000000, 1.000000000000000000, -0.000000000000000000 ) ) ;
#6350=CARTESIAN_POINT ( 'NONE',  ( -5.732832253866456007, -189.7472609257535510, -117.4638425504666657 ) ) ;
#6351=DIRECTION ( 'NONE',  ( 0.9266896074318343723, 0.000000000000000000, -0.3758275821142357809 ) ) ;
#6352=ORIENTED_EDGE ( 'NONE', *, *, #29349, .T. ) ;
#6354=LINE ( 'NONE', #14762, #47302 ) ;
#6356=ORIENTED_EDGE ( 'NONE', *, *, #6450, .F. ) ;
#6362=VECTOR ( 'NONE', #4256, 1000.000000000000000 ) ;
#6363=DIRECTION ( 'NONE',  ( 0.000000000000000000, 0.000000000000000000, 1.000000000000000000 ) ) ;
#6364=CARTESIAN_POINT ( 'NONE',  ( 75.78974234412359579, -177.1207230881787780, 13.49993235881448861 ) ) ;
#6366=EDGE_CURVE ( 'NONE', #20647, #17499, #16923, .T. ) ;
#6367=CARTESIAN_POINT ( 'NONE',  ( -145.4373324222574126, -175.3837268820161057, -78.89300572996837957 ) ) ;
#6368=LINE ( 'NONE', #50517, #30261 ) ;
#6369=CARTESIAN_POINT ( 'NONE',  ( -48.47912675150885065, -175.3837268820161057, 6.938893903907228378E-15 ) ) ;
#6372=AXIS2_PLACEMENT_3D ( 'NONE', #8181, #32862, #20791 ) ;
#6374=FACE_OUTER_BOUND ( 'NONE', #37032, .T. ) ;
#6376=CARTESIAN_POINT ( 'NONE',  ( -164.0008810331606526, -193.5000000000000000, 47.74645837849825369 ) ) ;
#6377=EDGE_LOOP ( 'NONE', ( #40567, #46089, #36199, #39281 ) ) ;
#6378=ADVANCED_FACE ( 'NONE', ( #30899 ), #43505, .T. ) ;
#6379=EDGE_CURVE ( 'NONE', #4823, #44074, #6985, .T. ) ;
#6381=DIRECTION ( 'NONE',  ( 0.000000000000000000, -1.000000000000000000, -0.000000000000000000 ) ) ;
#6382=VECTOR ( 'NONE', #27370, 1000.000000000000000 ) ;
#6384=PLANE ( 'NONE',  #41667 ) ;
#6385=EDGE_CURVE ( 'NONE', #41503, #11325, #3811, .T. ) ;
#6388=CARTESIAN_POINT ( 'NONE',  ( -47.87232660569025455, -183.6283474603465606, -0.7948544414133454916 ) ) ;
#6389=CARTESIAN_POINT ( 'NONE',  ( 45.36094686508022988, -193.5000000000000000, -82.57748230379237953 ) ) ;
#6393=DIRECTION ( 'NONE',  ( 0.000000000000000000, -1.000000000000000000, 0.000000000000000000 ) ) ;
#6396=EDGE_CURVE ( 'NONE', #11174, #15087, #2773, .T. ) ;
#6397=CARTESIAN_POINT ( 'NONE',  ( -134.7293151056888973, -193.5000000000000000, -89.08931047202574405 ) ) ;
#6398=EDGE_CURVE ( 'NONE', #23283, #41966, #3549, .T. ) ;
#6399=ORIENTED_EDGE ( 'NONE', *, *, #42488, .F. ) ;
#6402=VECTOR ( 'NONE', #27831, 1000.000000000000000 ) ;
#6404=ADVANCED_FACE ( 'NONE', ( #19582 ), #47193, .T. ) ;
#6405=DIRECTION ( 'NONE',  ( 0.000000000000000000, 0.000000000000000000, -1.000000000000000000 ) ) ;
#6406=CARTESIAN_POINT ( 'NONE',  ( -49.30901192927172616, -189.7472609257535510, -124.9972451320097093 ) ) ;
#6408=VECTOR ( 'NONE', #43149, 1000.000000000000000 ) ;
#6409=EDGE_CURVE ( 'NONE', #43249, #41296, #11694, .T. ) ;
#6412=DIRECTION ( 'NONE',  ( -0.5829794791144703447, 0.000000000000000000, -0.8124868780056825335 ) ) ;
#6413=ADVANCED_FACE ( 'NONE', ( #14887 ), #27194, .T. ) ;
#6414=ORIENTED_EDGE ( 'NONE', *, *, #22808, .F. ) ;
#6415=CARTESIAN_POINT ( 'NONE',  ( 75.37518750349086361, -183.6283474603465606, 6.025661128238926523 ) ) ;
#6416=EDGE_CURVE ( 'NONE', #12390, #46128, #35470, .T. ) ;
#6418=AXIS2_PLACEMENT_3D ( 'NONE', #31847, #294, #4512 ) ;
#6420=DIRECTION ( 'NONE',  ( 0.6068001458185945385, 0.000000000000000000, -0.7948544414133523750 ) ) ;
#6421=LINE ( 'NONE', #26638, #17788 ) ;
#6422=VERTEX_POINT ( 'NONE', #7242 ) ;
#6423=VECTOR ( 'NONE', #34502, 1000.000000000000114 ) ;
#6424=AXIS2_PLACEMENT_3D ( 'NONE', #46793, #7606, #19186 ) ;
#6427=AXIS2_PLACEMENT_3D ( 'NONE', #39897, #7854, #14990 ) ;
#6428=EDGE_CURVE ( 'NONE', #3536, #9877, #51155, .T. ) ;
#6429=AXIS2_PLACEMENT_3D ( 'NONE', #22203, #20444, #1248 ) ;
#6432=DIRECTION ( 'NONE',  ( 0.000000000000000000, 1.000000000000000000, 0.000000000000000000 ) ) ;
#6434=DIRECTION ( 'NONE',  ( -0.000000000000000000, 1.000000000000000000, -0.000000000000000000 ) ) ;
#6435=DIRECTION ( 'NONE',  ( -0.000000000000000000, 1.000000000000000000, -0.000000000000000000 ) ) ;
#6436=DIRECTION ( 'NONE',  ( -0.9995608365087942371, 0.000000000000000000, -0.02963332782256331357 ) ) ;
#6437=CARTESIAN_POINT ( 'NONE',  ( -172.3973245609188041, -189.7472609257535510, 4.503971736581616092 ) ) ;
#6439=EDGE_LOOP ( 'NONE', ( #30318, #20963, #36531, #51193 ) ) ;
#6441=CARTESIAN_POINT ( 'NONE',  ( -44.48323084606168720, -177.1207230881787780, 124.9361149384469769 ) ) ;
#6442=DIRECTION ( 'NONE',  ( -0.3758275821142357809, 0.000000000000000000, -0.9266896074318343723 ) ) ;
#6443=AXIS2_PLACEMENT_3D ( 'NONE', #8579, #37480, #40898 ) ;
#6444=AXIS2_PLACEMENT_3D ( 'NONE', #22947, #27390, #51575 ) ;
#6445=CARTESIAN_POINT ( 'NONE',  ( 22.03849146056077757, -189.7472609257535510, 103.2098131075567267 ) ) ;
#6446=CARTESIAN_POINT ( 'NONE',  ( -70.42295845586433245, -175.3837268820161057, -123.0587999703024877 ) ) ;
#6447=ORIENTED_EDGE ( 'NONE', *, *, #28497, .F. ) ;
#6448=VECTOR ( 'NONE', #8706, 1000.000000000000114 ) ;
#6450=EDGE_CURVE ( 'NONE', #23517, #17429, #10319, .T. ) ;
#6451=CARTESIAN_POINT ( 'NONE',  ( 116.9235303384055840, -213.5000000000000000, 2.819679052520814125E-14 ) ) ;
#6453=EDGE_CURVE ( 'NONE', #33588, #35501, #20897, .T. ) ;
#6454=ORIENTED_EDGE ( 'NONE', *, *, #30997, .T. ) ;
#6455=ORIENTED_EDGE ( 'NONE', *, *, #50367, .T. ) ;
#6456=VECTOR ( 'NONE', #19605, 1000.000000000000227 ) ;
#6457=LINE ( 'NONE', #30343, #36561 ) ;
#6458=DIRECTION ( 'NONE',  ( 0.000000000000000000, -0.000000000000000000, 1.000000000000000000 ) ) ;
#6459=VECTOR ( 'NONE', #27823, 1000.000000000000114 ) ;
#6460=FACE_OUTER_BOUND ( 'NONE', #23720, .T. ) ;
#6463=LINE ( 'NONE', #30597, #27069 ) ;
#6466=PLANE ( 'NONE',  #13292 ) ;
#6470=DIRECTION ( 'NONE',  ( -0.000000000000000000, 1.000000000000000000, -0.000000000000000000 ) ) ;
#6471=ADVANCED_FACE ( 'NONE', ( #48749 ), #20352, .T. ) ;
#6474=LINE ( 'NONE', #10138, #5562 ) ;
#6475=DIRECTION ( 'NONE',  ( 0.000000000000000000, -1.000000000000000000, 0.000000000000000000 ) ) ;
#6476=FACE_OUTER_BOUND ( 'NONE', #30900, .T. ) ;
#6478=EDGE_CURVE ( 'NONE', #51370, #43010, #26135, .T. ) ;
#6479=DIRECTION ( 'NONE',  ( -0.000000000000000000, 1.000000000000000000, -0.000000000000000000 ) ) ;
#6481=VECTOR ( 'NONE', #20889, 999.9999999999998863 ) ;
#6485=AXIS2_PLACEMENT_3D ( 'NONE', #7698, #23978, #28431 ) ;
#6486=ORIENTED_EDGE ( 'NONE', *, *, #11588, .F. ) ;
#6487=ORIENTED_EDGE ( 'NONE', *, *, #43277, .F. ) ;
#6489=VECTOR ( 'NONE', #6697, 1000.000000000000000 ) ;
#6490=ORIENTED_EDGE ( 'NONE', *, *, #13966, .T. ) ;
#6491=DIRECTION ( 'NONE',  ( 0.000000000000000000, 0.000000000000000000, -1.000000000000000000 ) ) ;
#6493=FACE_OUTER_BOUND ( 'NONE', #29403, .T. ) ;
#6494=VERTEX_POINT ( 'NONE', #29284 ) ;
#6495=DIRECTION ( 'NONE',  ( 0.000000000000000000, -0.000000000000000000, -1.000000000000000000 ) ) ;
#6496=AXIS2_PLACEMENT_3D ( 'NONE', #28127, #44179, #37527 ) ;
#6498=DIRECTION ( 'NONE',  ( -0.000000000000000000, 1.000000000000000000, -0.000000000000000000 ) ) ;
#6499=CARTESIAN_POINT ( 'NONE',  ( -50.83192613281184435, -177.1207230881787780, 123.9784823535113816 ) ) ;
#6500=VERTEX_POINT ( 'NONE', #45336 ) ;
#6503=AXIS2_PLACEMENT_3D ( 'NONE', #7087, #35192, #47299 ) ;
#6505=DIRECTION ( 'NONE',  ( 0.9374196611341231167, 0.000000000000000000, -0.3482016354343928088 ) ) ;
#6509=EDGE_LOOP ( 'NONE', ( #41874, #45923, #24253, #35591 ) ) ;
#6510=EDGE_CURVE ( 'NONE', #15990, #4438, #39557, .T. ) ;
#6512=ORIENTED_EDGE ( 'NONE', *, *, #33950, .T. ) ;
#6513=DIRECTION ( 'NONE',  ( 0.000000000000000000, 1.000000000000000000, 0.000000000000000000 ) ) ;
#6514=ORIENTED_EDGE ( 'NONE', *, *, #46798, .T. ) ;
#6515=AXIS2_PLACEMENT_3D ( 'NONE', #535, #31183, #6770 ) ;
#6517=AXIS2_PLACEMENT_3D ( 'NONE', #43081, #34927, #43852 ) ;
#6518=DIRECTION ( 'NONE',  ( -0.6528221181905119463, 0.000000000000000000, -0.7575112421616284619 ) ) ;
#6519=EDGE_LOOP ( 'NONE', ( #39329, #13051, #26272, #5545 ) ) ;
#6520=DIRECTION ( 'NONE',  ( -0.6965510290629882695, 0.000000000000000000, -0.7175072570443395970 ) ) ;
#6521=DIRECTION ( 'NONE',  ( 0.000000000000000000, 0.000000000000000000, -1.000000000000000000 ) ) ;
#6523=ORIENTED_EDGE ( 'NONE', *, *, #39098, .F. ) ;
#6524=LINE ( 'NONE', #10440, #3203 ) ;
#6525=ORIENTED_EDGE ( 'NONE', *, *, #19554, .F. ) ;
#6526=ORIENTED_EDGE ( 'NONE', *, *, #8789, .T. ) ;
#6528=AXIS2_PLACEMENT_3D ( 'NONE', #10874, #26893, #42924 ) ;
#6531=ADVANCED_FACE ( 'NONE', ( #40063 ), #32954, .T. ) ;
#6532=DIRECTION ( 'NONE',  ( 0.6749830015182038956, 0.000000000000000000, 0.7378332790417333475 ) ) ;
#6533=VERTEX_POINT ( 'NONE', #12979 ) ;
#6534=CIRCLE ( 'NONE', #8164, 125.0000000000000000 ) ;
#6535=DIRECTION ( 'NONE',  ( 0.9646355819083594074, 0.000000000000000000, -0.2635871660690647933 ) ) ;
#6536=DIRECTION ( 'NONE',  ( 0.4566292373937140270, 0.000000000000000000, -0.8896570909947467687 ) ) ;
#6537=CARTESIAN_POINT ( 'NONE',  ( -48.47912675150885065, -183.6283474603465606, 6.938893903907228378E-15 ) ) ;
#6538=LINE ( 'NONE', #49896, #9461 ) ;
#6540=ORIENTED_EDGE ( 'NONE', *, *, #33153, .F. ) ;
#6541=LINE ( 'NONE', #22566, #6215 ) ;
#6542=CARTESIAN_POINT ( 'NONE',  ( -47.57632892154311577, -189.7472609257535510, 0.4300652022765314997 ) ) ;
#6543=AXIS2_PLACEMENT_3D ( 'NONE', #48326, #24406, #12309 ) ;
#6544=CARTESIAN_POINT ( 'NONE',  ( -173.0563034899574859, -175.3837268820161057, -10.27263529369816908 ) ) ;
#6545=EDGE_LOOP ( 'NONE', ( #12020, #28109, #18932, #2744 ) ) ;
#6546=CARTESIAN_POINT ( 'NONE',  ( -172.5669052183642123, -183.6283474603465606, 15.07392567185546994 ) ) ;
#6547=FACE_OUTER_BOUND ( 'NONE', #42409, .T. ) ;
#6549=CARTESIAN_POINT ( 'NONE',  ( 46.40005841627164074, -193.5000000000000000, 81.38144888055276738 ) ) ;
#6550=EDGE_CURVE ( 'NONE', #38627, #9866, #36382, .T. ) ;
#6551=ORIENTED_EDGE ( 'NONE', *, *, #18064, .T. ) ;
#6552=AXIS2_PLACEMENT_3D ( 'NONE', #43986, #7732, #35574 ) ;
#6554=AXIS2_PLACEMENT_3D ( 'NONE', #9614, #37203, #21439 ) ;
#6557=VECTOR ( 'NONE', #12669, 1000.000000000000000 ) ;
#6559=CARTESIAN_POINT ( 'NONE',  ( -149.7090673587773040, -189.7472609257535510, -71.61357856150524981 ) ) ;
#6560=ORIENTED_EDGE ( 'NONE', *, *, #50850, .F. ) ;
#6562=EDGE_CURVE ( 'NONE', #49503, #30910, #4086, .T. ) ;
#6563=VERTEX_POINT ( 'NONE', #29007 ) ;
#6566=ORIENTED_EDGE ( 'NONE', *, *, #51638, .T. ) ;
#6567=DIRECTION ( 'NONE',  ( -0.000000000000000000, 1.000000000000000000, -0.000000000000000000 ) ) ;
#6568=EDGE_CURVE ( 'NONE', #19715, #48288, #42083, .T. ) ;
#6569=VECTOR ( 'NONE', #23607, 1000.000000000000114 ) ;
#6570=CARTESIAN_POINT ( 'NONE',  ( 26.52087324849106054, -198.5000000000000000, -70.00000000000002842 ) ) ;
#6575=EDGE_LOOP ( 'NONE', ( #15819, #43317, #50116, #14487 ) ) ;
#6577=CARTESIAN_POINT ( 'NONE',  ( 53.18081239921338010, -189.7472609257535510, -72.73415134495935774 ) ) ;
#6579=CARTESIAN_POINT ( 'NONE',  ( 9.336583202542589888, -189.7472609257535510, 110.8257356506556306 ) ) ;
#6580=ORIENTED_EDGE ( 'NONE', *, *, #35916, .F. ) ;
#6583=FACE_OUTER_BOUND ( 'NONE', #2062, .T. ) ;
#6584=ORIENTED_EDGE ( 'NONE', *, *, #113, .T. ) ;
#6585=ORIENTED_EDGE ( 'NONE', *, *, #37619, .F. ) ;
#6586=FACE_OUTER_BOUND ( 'NONE', #20715, .T. ) ;
#6589=VECTOR ( 'NONE', #23766, 1000.000000000000000 ) ;
#6590=LINE ( 'NONE', #30734, #32374 ) ;
#6596=CARTESIAN_POINT ( 'NONE',  ( 116.9235303384055840, -213.5000000000000000, 10.00000000000000000 ) ) ;
#6597=LINE ( 'NONE', #46284, #42758 ) ;
#6602=DIRECTION ( 'NONE',  ( -0.000000000000000000, 1.000000000000000000, -0.000000000000000000 ) ) ;
#6604=ORIENTED_EDGE ( 'NONE', *, *, #43586, .F. ) ;
#6605=AXIS2_PLACEMENT_3D ( 'NONE', #18055, #2017, #5463 ) ;
#6606=CARTESIAN_POINT ( 'NONE',  ( 141.7825277784304205, -213.5000000000000000, 10.00000000000000178 ) ) ;
#6607=DIRECTION ( 'NONE',  ( -0.000000000000000000, 1.000000000000000000, -0.000000000000000000 ) ) ;
#6608=DIRECTION ( 'NONE',  ( -0.000000000000000000, -1.000000000000000000, 0.000000000000000000 ) ) ;
#6612=CARTESIAN_POINT ( 'NONE',  ( -117.6101668435555325, -189.7472609257535510, -102.9412430821794686 ) ) ;
#6613=CARTESIAN_POINT ( 'NONE',  ( -37.67038537088846084, -177.1207230881787780, -124.5318076226586470 ) ) ;
#6615=ORIENTED_EDGE ( 'NONE', *, *, #42974, .T. ) ;
#6616=ADVANCED_FACE ( 'NONE', ( #44284 ), #37161, .T. ) ;
#6617=ADVANCED_FACE ( 'NONE', ( #36126 ), #33221, .T. ) ;
#6618=DIRECTION ( 'NONE',  ( -0.000000000000000000, 1.000000000000000000, -0.000000000000000000 ) ) ;
#6619=DIRECTION ( 'NONE',  ( 0.000000000000000000, -1.000000000000000000, 0.000000000000000000 ) ) ;
#6620=VERTEX_POINT ( 'NONE', #13262 ) ;
#6625=VERTEX_POINT ( 'NONE', #29534 ) ;
#6627=VECTOR ( 'NONE', #50701, 1000.000000000000000 ) ;
#6630=CARTESIAN_POINT ( 'NONE',  ( 66.73972540229262052, -189.7472609257535510, 45.83253885719641829 ) ) ;
#6631=ORIENTED_EDGE ( 'NONE', *, *, #19086, .T. ) ;
#6632=EDGE_CURVE ( 'NONE', #40491, #19552, #25588, .T. ) ;
#6633=CARTESIAN_POINT ( 'NONE',  ( -36.09284319799462537, -183.6283474603465606, 124.3848060646152476 ) ) ;
#6636=FACE_OUTER_BOUND ( 'NONE', #48462, .T. ) ;
#6638=ORIENTED_EDGE ( 'NONE', *, *, #29564, .T. ) ;
#6639=EDGE_CURVE ( 'NONE', #25286, #17442, #30064, .T. ) ;
#6640=DIRECTION ( 'NONE',  ( 0.000000000000000000, 0.000000000000000000, 1.000000000000000000 ) ) ;
#6641=ORIENTED_EDGE ( 'NONE', *, *, #15329, .T. ) ;
#6642=CARTESIAN_POINT ( 'NONE',  ( -117.6101668435555325, -175.3837268820161057, -102.9412430821794686 ) ) ;
#6643=EDGE_CURVE ( 'NONE', #31627, #47473, #5381, .T. ) ;
#6645=CARTESIAN_POINT ( 'NONE',  ( -161.4019114581580823, -193.5000000000000000, 53.60452120946281696 ) ) ;
#6648=EDGE_LOOP ( 'NONE', ( #40842, #31029, #9021, #50599 ) ) ;
#6652=CARTESIAN_POINT ( 'NONE',  ( -160.0666658415768211, -175.3837268820161057, 54.07611884703388228 ) ) ;
#6654=FACE_OUTER_BOUND ( 'NONE', #3331, .T. ) ;
#6656=EDGE_LOOP ( 'NONE', ( #47850, #42641, #27122, #35908 ) ) ;
#6659=ORIENTED_EDGE ( 'NONE', *, *, #8503, .F. ) ;
#6660=LINE ( 'NONE', #30045, #19054 ) ;
#6661=VERTEX_POINT ( 'NONE', #50044 ) ;
#6664=LINE ( 'NONE', #22683, #1745 ) ;
#6667=CARTESIAN_POINT ( 'NONE',  ( -171.9838957966129556, -193.5000000000000000, 19.27620354518722579 ) ) ;
#6669=VERTEX_POINT ( 'NONE', #49789 ) ;
#6670=DIRECTION ( 'NONE',  ( 0.000000000000000000, 0.000000000000000000, 1.000000000000000000 ) ) ;
#6673=CARTESIAN_POINT ( 'NONE',  ( -168.6933499419502596, -193.5000000000000000, 30.40954281680882687 ) ) ;
#6674=ORIENTED_EDGE ( 'NONE', *, *, #10581, .T. ) ;
#6678=ADVANCED_FACE ( 'NONE', ( #17482 ), #41891, .T. ) ;
#6683=ORIENTED_EDGE ( 'NONE', *, *, #26926, .T. ) ;
#6686=ORIENTED_EDGE ( 'NONE', *, *, #37088, .F. ) ;
#6687=CARTESIAN_POINT ( 'NONE',  ( -90.87721961371603641, -189.7472609257535510, 116.5264228893328777 ) ) ;
#6688=CARTESIAN_POINT ( 'NONE',  ( 71.87891646118019651, -193.5000000000000000, -33.74820638215424395 ) ) ;
#6689=ADVANCED_FACE ( 'NONE', ( #9571 ), #37692, .T. ) ;
#6690=ADVANCED_FACE ( 'NONE', ( #17731 ), #22445, .F. ) ;
#6693=ORIENTED_EDGE ( 'NONE', *, *, #51586, .T. ) ;
#6697=DIRECTION ( 'NONE',  ( -0.6965510290629882695, 0.000000000000000000, -0.7175072570443395970 ) ) ;
#6698=LINE ( 'NONE', #13799, #6752 ) ;
#6699=EDGE_CURVE ( 'NONE', #26523, #43006, #9839, .T. ) ;
#6700=VECTOR ( 'NONE', #46950, 1000.000000000000000 ) ;
#6701=LINE ( 'NONE', #51122, #10283 ) ;
#6702=DIRECTION ( 'NONE',  ( 0.000000000000000000, -1.000000000000000000, 0.000000000000000000 ) ) ;
#6703=VERTEX_POINT ( 'NONE', #1946 ) ;
#6704=EDGE_CURVE ( 'NONE', #14253, #48059, #22177, .T. ) ;
#6705=FACE_OUTER_BOUND ( 'NONE', #27629, .T. ) ;
#6706=FACE_OUTER_BOUND ( 'NONE', #30151, .T. ) ;
#6711=CARTESIAN_POINT ( 'NONE',  ( -47.97059563285963435, -193.5000000000000000, 0.8610436117673654355 ) ) ;
#6712=DIRECTION ( 'NONE',  ( -0.2348860457809775482, 0.000000000000000000, -0.9720229140804121926 ) ) ;
#6713=DIRECTION ( 'NONE',  ( -0.000000000000000000, 1.000000000000000000, 0.000000000000000000 ) ) ;
#6714=DIRECTION ( 'NONE',  ( -0.000000000000000000, 1.000000000000000000, -0.000000000000000000 ) ) ;
#6715=ORIENTED_EDGE ( 'NONE', *, *, #26481, .F. ) ;
#6718=AXIS2_PLACEMENT_3D ( 'NONE', #16189, #3321, #7265 ) ;
#6719=CIRCLE ( 'NONE', #4201, 125.0000000000000000 ) ;
#6720=ORIENTED_EDGE ( 'NONE', *, *, #11512, .T. ) ;
#6721=DIRECTION ( 'NONE',  ( 0.000000000000000000, -1.000000000000000000, 0.000000000000000000 ) ) ;
#6723=VERTEX_POINT ( 'NONE', #13518 ) ;
#6725=DIRECTION ( 'NONE',  ( 0.000000000000000000, 0.000000000000000000, -1.000000000000000000 ) ) ;
#6726=FACE_OUTER_BOUND ( 'NONE', #5460, .T. ) ;
#6727=CARTESIAN_POINT ( 'NONE',  ( -173.4291566779743050, -175.3837268820161057, 3.534122433558352760 ) ) ;
#6728=CARTESIAN_POINT ( 'NONE',  ( 66.36634345758743336, -175.3837268820161057, 46.76022031560704306 ) ) ;
#6730=ORIENTED_EDGE ( 'NONE', *, *, #18555, .F. ) ;
#6732=CARTESIAN_POINT ( 'NONE',  ( -63.43218022845228887, -193.5000000000000000, 124.1024020384604540 ) ) ;
#6736=EDGE_CURVE ( 'NONE', #47219, #3342, #6421, .T. ) ;
#6737=FACE_OUTER_BOUND ( 'NONE', #12223, .T. ) ;
#6738=EDGE_CURVE ( 'NONE', #13810, #44232, #15322, .T. ) ;
#6740=EDGE_CURVE ( 'NONE', #19788, #18322, #51334, .T. ) ;
#6742=EDGE_LOOP ( 'NONE', ( #15258, #51435, #24365, #22684 ) ) ;
#6743=DIRECTION ( 'NONE',  ( -0.2920567706369833760, 0.000000000000000000, 0.9564009842765202052 ) ) ;
#6748=LINE ( 'NONE', #51417, #15205 ) ;
#6750=ORIENTED_EDGE ( 'NONE', *, *, #50183, .F. ) ;
#6751=VERTEX_POINT ( 'NONE', #43172 ) ;
#6752=VECTOR ( 'NONE', #50579, 1000.000000000000000 ) ;
#6753=VECTOR ( 'NONE', #34194, 1000.000000000000114 ) ;
#6754=ORIENTED_EDGE ( 'NONE', *, *, #8851, .F. ) ;
#6755=DIRECTION ( 'NONE',  ( 0.000000000000000000, 0.000000000000000000, 1.000000000000000000 ) ) ;
#6756=CARTESIAN_POINT ( 'NONE',  ( -149.5539421794694022, -175.3837268820161057, 73.54509967498655953 ) ) ;
#6757=EDGE_CURVE ( 'NONE', #38633, #43006, #175, .T. ) ;
#6758=CARTESIAN_POINT ( 'NONE',  ( -32.98951909085346301, -175.3837268820161057, 123.0287672223653033 ) ) ;
#6759=FACE_OUTER_BOUND ( 'NONE', #14610, .T. ) ;
#6760=DIRECTION ( 'NONE',  ( 0.000000000000000000, -0.000000000000000000, 1.000000000000000000 ) ) ;
#6762=EDGE_CURVE ( 'NONE', #31203, #27852, #12736, .T. ) ;
#6763=EDGE_CURVE ( 'NONE', #27989, #1866, #37090, .T. ) ;
#6764=DIRECTION ( 'NONE',  ( 0.000000000000000000, 0.000000000000000000, -1.000000000000000000 ) ) ;
#6766=FACE_OUTER_BOUND ( 'NONE', #23483, .T. ) ;
#6767=ORIENTED_EDGE ( 'NONE', *, *, #17539, .F. ) ;
#6768=EDGE_LOOP ( 'NONE', ( #20772, #31362, #3501, #24923, #20227, #14783, #10605, #5835 ) ) ;
#6769=AXIS2_PLACEMENT_3D ( 'NONE', #26438, #18050, #21219 ) ;
#6770=DIRECTION ( 'NONE',  ( 0.000000000000000000, 0.000000000000000000, -1.000000000000000000 ) ) ;
#6773=PLANE ( 'NONE',  #13350 ) ;
#6774=ORIENTED_EDGE ( 'NONE', *, *, #44624, .T. ) ;
#6775=FACE_OUTER_BOUND ( 'NONE', #19206, .T. ) ;
#6776=VERTEX_POINT ( 'NONE', #31084 ) ;
#6780=FACE_OUTER_BOUND ( 'NONE', #23026, .T. ) ;
#6781=CARTESIAN_POINT ( 'NONE',  ( -163.6979789053106629, -193.5000000000000000, -45.83253885719559406 ) ) ;
#6782=CARTESIAN_POINT ( 'NONE',  ( 58.48829670243887335, -177.1207230881787780, -64.67588669375807342 ) ) ;
#6783=ORIENTED_EDGE ( 'NONE', *, *, #11482, .F. ) ;
#6785=CARTESIAN_POINT ( 'NONE',  ( -47.63353074800702558, -175.3837268820161057, -0.5338233779647817423 ) ) ;
#6786=VECTOR ( 'NONE', #28473, 1000.000000000000000 ) ;
#6787=DIRECTION ( 'NONE',  ( -0.000000000000000000, 1.000000000000000000, -0.000000000000000000 ) ) ;
#6791=CYLINDRICAL_SURFACE ( 'NONE', #8896, 124.9999999999999858 ) ;
#6793=AXIS2_PLACEMENT_3D ( 'NONE', #35217, #39657, #28093 ) ;
#6794=FACE_BOUND ( 'NONE', #36080, .T. ) ;
#6796=DIRECTION ( 'NONE',  ( 0.000000000000000000, 0.000000000000000000, -1.000000000000000000 ) ) ;
#6798=ORIENTED_EDGE ( 'NONE', *, *, #47021, .F. ) ;
#6800=EDGE_CURVE ( 'NONE', #6329, #13947, #47385, .T. ) ;
#6801=CARTESIAN_POINT ( 'NONE',  ( -49.45768324380835423, -189.7472609257535510, 0.2059786187410958813 ) ) ;
#6802=ORIENTED_EDGE ( 'NONE', *, *, #32429, .F. ) ;
#6803=CARTESIAN_POINT ( 'NONE',  ( -118.9967449635792462, -189.7472609257535510, -103.2098131075562009 ) ) ;
#6805=CARTESIAN_POINT ( 'NONE',  ( 48.06131630543706734, -175.3837268820161057, -79.40367028273054473 ) ) ;
#6806=DIRECTION ( 'NONE',  ( -0.000000000000000000, 1.000000000000000000, -0.000000000000000000 ) ) ;
#6809=ORIENTED_EDGE ( 'NONE', *, *, #6112, .T. ) ;
#6810=DIRECTION ( 'NONE',  ( -0.000000000000000000, 1.000000000000000000, -0.000000000000000000 ) ) ;
#6812=EDGE_CURVE ( 'NONE', #6055, #6703, #15855, .T. ) ;
#6813=LINE ( 'NONE', #46501, #27582 ) ;
#6814=VECTOR ( 'NONE', #24480, 1000.000000000000000 ) ;
#6815=EDGE_CURVE ( 'NONE', #39243, #503, #42118, .T. ) ;
#6819=VERTEX_POINT ( 'NONE', #27663 ) ;
#6820=DIRECTION ( 'NONE',  ( 0.000000000000000000, 1.000000000000000000, 0.000000000000000000 ) ) ;
#6821=DIRECTION ( 'NONE',  ( 0.05924062789371441901, 0.000000000000000000, -0.9982437317643214625 ) ) ;
#6822=EDGE_LOOP ( 'NONE', ( #15394, #15739, #12800, #39374 ) ) ;
#6824=ORIENTED_EDGE ( 'NONE', *, *, #572, .T. ) ;
#6825=CARTESIAN_POINT ( 'NONE',  ( -163.3872488209693756, -193.5000000000000000, -49.20491319441543254 ) ) ;
#6828=ORIENTED_EDGE ( 'NONE', *, *, #28558, .T. ) ;
#6829=DIRECTION ( 'NONE',  ( 0.000000000000000000, 0.000000000000000000, 1.000000000000000000 ) ) ;
#6830=LINE ( 'NONE', #18909, #11565 ) ;
#6832=ORIENTED_EDGE ( 'NONE', *, *, #24124, .T. ) ;
#6833=CARTESIAN_POINT ( 'NONE',  ( -26.71218532227686637, -193.5000000000000000, 122.0745693923550732 ) ) ;
#6834=VERTEX_POINT ( 'NONE', #15586 ) ;
#6836=PLANE ( 'NONE',  #51719 ) ;
#6840=LINE ( 'NONE', #14999, #32471 ) ;
#6841=DIRECTION ( 'NONE',  ( -0.000000000000000000, 1.000000000000000000, -0.000000000000000000 ) ) ;
#6842=ORIENTED_EDGE ( 'NONE', *, *, #39398, .F. ) ;
#6844=CARTESIAN_POINT ( 'NONE',  ( 32.99469856375238663, -175.3837268820161057, 94.79987230212020677 ) ) ;
#6846=DIRECTION ( 'NONE',  ( 0.000000000000000000, -0.000000000000000000, 1.000000000000000000 ) ) ;
#6847=ORIENTED_EDGE ( 'NONE', *, *, #5162, .T. ) ;
#6848=CARTESIAN_POINT ( 'NONE',  ( 73.80528149577283159, -189.7472609257535510, 25.91377046305970211 ) ) ;
#6849=CARTESIAN_POINT ( 'NONE',  ( 38.71172987070726634, -175.3837268820161057, -89.56983042009264295 ) ) ;
#6850=VECTOR ( 'NONE', #1213, 1000.000000000000000 ) ;
#6853=DIRECTION ( 'NONE',  ( 0.000000000000000000, 0.000000000000000000, 1.000000000000000000 ) ) ;
#6855=VERTEX_POINT ( 'NONE', #43695 ) ;
#6856=VECTOR ( 'NONE', #9366, 1000.000000000000000 ) ;
#6858=DIRECTION ( 'NONE',  ( -0.9929810960135185827, 0.000000000000000000, 0.1182731709213523247 ) ) ;
#6859=CARTESIAN_POINT ( 'NONE',  ( 14.37129481273059106, -175.3837268820161057, -108.0501018472328241 ) ) ;
#6860=DIRECTION ( 'NONE',  ( -0.000000000000000000, 1.000000000000000000, 0.000000000000000000 ) ) ;
#6862=CARTESIAN_POINT ( 'NONE',  ( -48.47912675150885065, -189.7472609257535510, 6.938893903907228378E-15 ) ) ;
#6863=ORIENTED_EDGE ( 'NONE', *, *, #51034, .T. ) ;
#6866=DIRECTION ( 'NONE',  ( 0.000000000000000000, 0.000000000000000000, 1.000000000000000000 ) ) ;
#6867=ORIENTED_EDGE ( 'NONE', *, *, #40944, .F. ) ;
#6870=ORIENTED_EDGE ( 'NONE', *, *, #1748, .T. ) ;
#6871=ADVANCED_FACE ( 'NONE', ( #7694 ), #50817, .T. ) ;
#6874=FACE_OUTER_BOUND ( 'NONE', #51382, .T. ) ;
#6875=VERTEX_POINT ( 'NONE', #51860 ) ;
#6878=CARTESIAN_POINT ( 'NONE',  ( -48.47912675150885065, -175.3837268820161057, 6.938893903907228378E-15 ) ) ;
#6881=DIRECTION ( 'NONE',  ( 0.000000000000000000, 0.000000000000000000, -1.000000000000000000 ) ) ;
#6885=ORIENTED_EDGE ( 'NONE', *, *, #41680, .F. ) ;
#6886=DIRECTION ( 'NONE',  ( 0.000000000000000000, -0.000000000000000000, 1.000000000000000000 ) ) ;
#6887=LINE ( 'NONE', #14525, #19611 ) ;
#6889=LINE ( 'NONE', #51059, #15687 ) ;
#6891=CIRCLE ( 'NONE', #28697, 124.9999999999999858 ) ;
#6892=VERTEX_POINT ( 'NONE', #31866 ) ;
#6894=DIRECTION ( 'NONE',  ( 0.000000000000000000, -0.000000000000000000, 1.000000000000000000 ) ) ;
#6895=ORIENTED_EDGE ( 'NONE', *, *, #10528, .T. ) ;
#6896=LINE ( 'NONE', #42889, #19047 ) ;
#6897=DIRECTION ( 'NONE',  ( -0.000000000000000000, 1.000000000000000000, -0.000000000000000000 ) ) ;
#6899=ORIENTED_EDGE ( 'NONE', *, *, #40521, .T. ) ;
#6902=CARTESIAN_POINT ( 'NONE',  ( -40.24578378811990831, -189.7472609257535510, 124.7285535218268251 ) ) ;
#6904=ORIENTED_EDGE ( 'NONE', *, *, #22236, .T. ) ;
#6905=CARTESIAN_POINT ( 'NONE',  ( 55.91309001144629320, -193.5000000000000000, 68.75510947788671956 ) ) ;
#6911=ORIENTED_EDGE ( 'NONE', *, *, #42681, .T. ) ;
#6912=CARTESIAN_POINT ( 'NONE',  ( -47.48307690889363641, -189.7472609257535510, 0.08879589532294547560 ) ) ;
#6914=CARTESIAN_POINT ( 'NONE',  ( -7.515176836080581957, -177.1207230881787780, 117.0391155081705250 ) ) ;
#6917=ORIENTED_EDGE ( 'NONE', *, *, #47378, .T. ) ;
#6918=LINE ( 'NONE', #38958, #51477 ) ;
#6919=EDGE_CURVE ( 'NONE', #20987, #12980, #44735, .T. ) ;
#6921=LINE ( 'NONE', #46112, #51216 ) ;
#6923=ORIENTED_EDGE ( 'NONE', *, *, #28724, .T. ) ;
#6925=EDGE_LOOP ( 'NONE', ( #39685, #30103, #23179, #46150 ) ) ;
#6926=CARTESIAN_POINT ( 'NONE',  ( 50.08808042611237710, -177.1207230881787780, -76.87330921200083367 ) ) ;
#6927=VECTOR ( 'NONE', #31280, 1000.000000000000227 ) ;
#6928=LINE ( 'NONE', #51339, #49784 ) ;
#6929=ORIENTED_EDGE ( 'NONE', *, *, #48371, .T. ) ;
#6931=CARTESIAN_POINT ( 'NONE',  ( -168.3100285466275636, -193.5000000000000000, -31.88354567334998535 ) ) ;
#6933=CARTESIAN_POINT ( 'NONE',  ( -238.7407812814481076, -213.5000000000000000, 10.00000000000000178 ) ) ;
#6934=CARTESIAN_POINT ( 'NONE',  ( -151.1459075827612537, -177.1207230881787780, 69.53890913632950799 ) ) ;
#6935=CARTESIAN_POINT ( 'NONE',  ( -84.82349129030166068, -175.3837268820161057, -119.5996955107802222 ) ) ;
#6936=LINE ( 'NONE', #3498, #8135 ) ;
#6937=EDGE_LOOP ( 'NONE', ( #25542, #14929, #6867, #28848 ) ) ;
#6939=VERTEX_POINT ( 'NONE', #48163 ) ;
#6940=VECTOR ( 'NONE', #35846, 1000.000000000000000 ) ;
#6941=ORIENTED_EDGE ( 'NONE', *, *, #42407, .T. ) ;
#6943=CARTESIAN_POINT ( 'NONE',  ( -139.0630283577175987, -177.1207230881787780, -86.13684908212449898 ) ) ;
#6947=DIRECTION ( 'NONE',  ( -0.8757349421956310831, 0.000000000000000000, -0.4827922027307550712 ) ) ;
#6948=DIRECTION ( 'NONE',  ( -0.6965510290629932655, 0.000000000000000000, -0.7175072570443347120 ) ) ;
#6949=ORIENTED_EDGE ( 'NONE', *, *, #5625, .F. ) ;
#6951=CARTESIAN_POINT ( 'NONE',  ( -169.2746641285359317, -193.5000000000000000, -32.14713283941905786 ) ) ;
#6952=DIRECTION ( 'NONE',  ( -0.000000000000000000, 1.000000000000000000, -0.000000000000000000 ) ) ;
#6953=EDGE_LOOP ( 'NONE', ( #23975, #31834, #26432, #41371 ) ) ;
#6954=EDGE_LOOP ( 'NONE', ( #30383, #29281, #15917, #28967 ) ) ;
#6955=DIRECTION ( 'NONE',  ( -0.5586467658036594619, 0.000000000000000000, 0.8294056854501971054 ) ) ;
#6956=CARTESIAN_POINT ( 'NONE',  ( 26.52087324849106054, -173.5000000000000284, -60.00000000000003553 ) ) ;
#6959=CIRCLE ( 'NONE', #35485, 125.0000000000000000 ) ;
#6960=DIRECTION ( 'NONE',  ( 0.8757349421956379665, 0.000000000000000000, -0.4827922027307427477 ) ) ;
#6961=EDGE_CURVE ( 'NONE', #24932, #34133, #40510, .T. ) ;
#6962=ADVANCED_FACE ( 'NONE', ( #40773 ), #27913, .T. ) ;
#6963=CARTESIAN_POINT ( 'NONE',  ( 20.93410174202488605, -175.3837268820161057, -102.7511748916624583 ) ) ;
#6964=ORIENTED_EDGE ( 'NONE', *, *, #50308, .T. ) ;
#6968=DIRECTION ( 'NONE',  ( 0.000000000000000000, 1.000000000000000000, -0.000000000000000000 ) ) ;
#6970=ORIENTED_EDGE ( 'NONE', *, *, #14480, .T. ) ;
#6971=EDGE_CURVE ( 'NONE', #471, #34929, #8722, .T. ) ;
#6972=DIRECTION ( 'NONE',  ( 0.000000000000000000, 0.000000000000000000, -1.000000000000000000 ) ) ;
#6974=CARTESIAN_POINT ( 'NONE',  ( -49.25565061422690150, -183.6283474603465606, 0.6300878435817109935 ) ) ;
#6976=AXIS2_PLACEMENT_3D ( 'NONE', #9760, #50237, #6335 ) ;
#6978=VECTOR ( 'NONE', #8856, 1000.000000000000000 ) ;
#6979=EDGE_CURVE ( 'NONE', #49449, #46206, #28427, .T. ) ;
#6981=EDGE_LOOP ( 'NONE', ( #31500, #43473, #28838, #9855 ) ) ;
#6983=EDGE_CURVE ( 'NONE', #28151, #33835, #36580, .T. ) ;
#6984=DIRECTION ( 'NONE',  ( -0.000000000000000000, 1.000000000000000000, -0.000000000000000000 ) ) ;
#6985=LINE ( 'NONE', #19336, #46415 ) ;
#6986=ORIENTED_EDGE ( 'NONE', *, *, #6209, .T. ) ;
#6987=EDGE_CURVE ( 'NONE', #6563, #602, #32372, .T. ) ;
#6988=ORIENTED_EDGE ( 'NONE', *, *, #5037, .F. ) ;
#6989=DIRECTION ( 'NONE',  ( 0.9266896074318370369, 0.000000000000000000, -0.3758275821142292306 ) ) ;
#6992=CARTESIAN_POINT ( 'NONE',  ( -164.3791542526839180, -193.5000000000000000, 46.82076062204521349 ) ) ;
#6993=VERTEX_POINT ( 'NONE', #11881 ) ;
#6995=CARTESIAN_POINT ( 'NONE',  ( 62.13187335169531167, -183.6283474603465606, -58.22548115875872554 ) ) ;
#6997=CARTESIAN_POINT ( 'NONE',  ( -105.4063847101409692, -175.3837268820161057, -111.2847127925096231 ) ) ;
#6998=AXIS2_PLACEMENT_3D ( 'NONE', #8254, #30244, #14734 ) ;
#6999=DIRECTION ( 'NONE',  ( -0.000000000000000000, 1.000000000000000000, -0.000000000000000000 ) ) ;
#7003=CIRCLE ( 'NONE', #11194, 124.9999999999999858 ) ;
#7007=LINE ( 'NONE', #26444, #47008 ) ;
#7008=PLANE ( 'NONE',  #21780 ) ;
#7010=DIRECTION ( 'NONE',  ( -0.000000000000000000, 1.000000000000000000, -0.000000000000000000 ) ) ;
#7011=ORIENTED_EDGE ( 'NONE', *, *, #16934, .T. ) ;
#7012=AXIS2_PLACEMENT_3D ( 'NONE', #35000, #41859, #26850 ) ;
#7014=ADVANCED_FACE ( 'NONE', ( #20824 ), #43947, .F. ) ;
#7016=LINE ( 'NONE', #23040, #6340 ) ;
#7017=EDGE_LOOP ( 'NONE', ( #40676, #47491, #15886, #28575 ) ) ;
#7019=CARTESIAN_POINT ( 'NONE',  ( 63.54086012517504400, -175.3837268820161057, -53.17445600718542664 ) ) ;
#7020=DIRECTION ( 'NONE',  ( 1.000000000000000000, 0.000000000000000000, -0.000000000000000000 ) ) ;
#7022=ADVANCED_FACE ( 'NONE', ( #16633 ), #28683, .T. ) ;
#7023=CARTESIAN_POINT ( 'NONE',  ( -81.14588623932559130, -177.1207230881787780, 120.6560517527618117 ) ) ;
#7024=EDGE_CURVE ( 'NONE', #26963, #19552, #7937, .T. ) ;
#7026=CARTESIAN_POINT ( 'NONE',  ( -171.5592422664403216, -183.6283474603465606, -21.82395850507258928 ) ) ;
#7029=ORIENTED_EDGE ( 'NONE', *, *, #31081, .T. ) ;
#7031=EDGE_LOOP ( 'NONE', ( #17174, #29421, #33522, #780 ) ) ;
#7033=CARTESIAN_POINT ( 'NONE',  ( -153.4237445717492392, -189.7472609257535510, 66.05018866041348247 ) ) ;
#7035=LINE ( 'NONE', #42241, #19660 ) ;
#7036=DIRECTION ( 'NONE',  ( -0.000000000000000000, 1.000000000000000000, -0.000000000000000000 ) ) ;
#7038=DIRECTION ( 'NONE',  ( 0.05924062789370748011, 0.000000000000000000, 0.9982437317643217956 ) ) ;
#7039=VECTOR ( 'NONE', #43295, 1000.000000000000000 ) ;
#7040=CARTESIAN_POINT ( 'NONE',  ( -130.7087404384255080, -189.7472609257535510, -94.14505102712755047 ) ) ;
#7041=CARTESIAN_POINT ( 'NONE',  ( -159.8192355313504152, -183.6283474603465606, -56.81883646197837834 ) ) ;
#7042=DIRECTION ( 'NONE',  ( 0.000000000000000000, -1.000000000000000000, 0.000000000000000000 ) ) ;
#7043=ADVANCED_FACE ( 'NONE', ( #50249 ), #29221, .T. ) ;
#7044=ORIENTED_EDGE ( 'NONE', *, *, #9704, .F. ) ;
#7045=DIRECTION ( 'NONE',  ( 0.000000000000000000, 0.000000000000000000, -1.000000000000000000 ) ) ;
#7046=DIRECTION ( 'NONE',  ( -0.4300652022765183435, 0.000000000000000000, -0.9027978299657446470 ) ) ;
#7049=DIRECTION ( 'NONE',  ( 0.000000000000000000, -1.000000000000000000, 0.000000000000000000 ) ) ;
#7050=EDGE_LOOP ( 'NONE', ( #22447, #33533, #14657, #2476 ) ) ;
#7051=EDGE_CURVE ( 'NONE', #13015, #23682, #33157, .T. ) ;
#7054=EDGE_CURVE ( 'NONE', #50634, #10587, #4348, .T. ) ;
#7056=LINE ( 'NONE', #34393, #45567 ) ;
#7058=VERTEX_POINT ( 'NONE', #21864 ) ;
#7059=ADVANCED_FACE ( 'NONE', ( #6099 ), #5321, .T. ) ;
#7061=FACE_BOUND ( 'NONE', #31927, .T. ) ;
#7062=CARTESIAN_POINT ( 'NONE',  ( -51.89154260666836649, -177.1207230881787780, 124.9534129907280828 ) ) ;
#7066=EDGE_CURVE ( 'NONE', #51627, #1228, #9259, .T. ) ;
#7067=ORIENTED_EDGE ( 'NONE', *, *, #12673, .F. ) ;
#7069=ORIENTED_EDGE ( 'NONE', *, *, #43461, .F. ) ;
#7070=CYLINDRICAL_SURFACE ( 'NONE', #19226, 125.0000000000000000 ) ;
#7071=CIRCLE ( 'NONE', #49877, 125.0000000000000000 ) ;
#7073=FACE_OUTER_BOUND ( 'NONE', #40219, .T. ) ;
#7075=ORIENTED_EDGE ( 'NONE', *, *, #44591, .T. ) ;
#7079=LINE ( 'NONE', #3134, #5526 ) ;
#7080=EDGE_LOOP ( 'NONE', ( #15158, #22484, #18835, #21624 ) ) ;
#7081=LINE ( 'NONE', #18654, #21358 ) ;
#7083=ADVANCED_FACE ( 'NONE', ( #33438 ), #33682, .T. ) ;
#7086=VERTEX_POINT ( 'NONE', #37631 ) ;
#7087=CARTESIAN_POINT ( 'NONE',  ( -149.9407190013152160, -193.5000000000000000, -73.01058346660458653 ) ) ;
#7089=CIRCLE ( 'NONE', #29733, 125.0000000000000000 ) ;
#7090=ORIENTED_EDGE ( 'NONE', *, *, #35313, .F. ) ;
#7092=ADVANCED_FACE ( 'NONE', ( #13710 ), #22372, .T. ) ;
#7095=DIRECTION ( 'NONE',  ( 0.000000000000000000, -1.000000000000000000, 0.000000000000000000 ) ) ;
#7098=CYLINDRICAL_SURFACE ( 'NONE', #15478, 125.0000000000000000 ) ;
#7102=ORIENTED_EDGE ( 'NONE', *, *, #45720, .T. ) ;
#7105=LINE ( 'NONE', #38637, #12858 ) ;
#7106=ORIENTED_EDGE ( 'NONE', *, *, #8083, .F. ) ;
#7112=DIRECTION ( 'NONE',  ( -0.000000000000000000, 1.000000000000000000, -0.000000000000000000 ) ) ;
#7113=LINE ( 'NONE', #14746, #26604 ) ;
#7115=CIRCLE ( 'NONE', #36460, 125.0000000000000000 ) ;
#7116=ADVANCED_FACE ( 'NONE', ( #5850 ), #37882, .T. ) ;
#7117=PLANE ( 'NONE',  #32963 ) ;
#7118=CARTESIAN_POINT ( 'NONE',  ( -148.0127667507368585, -177.1207230881787780, -75.61781872352626976 ) ) ;
#7121=DIRECTION ( 'NONE',  ( 0.000000000000000000, 1.000000000000000000, 0.000000000000000000 ) ) ;
#7122=ORIENTED_EDGE ( 'NONE', *, *, #13614, .T. ) ;
#7123=CIRCLE ( 'NONE', #49113, 124.9999999999999858 ) ;
#7127=ORIENTED_EDGE ( 'NONE', *, *, #23402, .T. ) ;
#7129=DIRECTION ( 'NONE',  ( 0.000000000000000000, 0.000000000000000000, 1.000000000000000000 ) ) ;
#7130=ORIENTED_EDGE ( 'NONE', *, *, #42614, .T. ) ;
#7133=LINE ( 'NONE', #2669, #50176 ) ;
#7134=CARTESIAN_POINT ( 'NONE',  ( 39.56636334395316368, -193.5000000000000000, -87.31661597576083977 ) ) ;
#7135=VERTEX_POINT ( 'NONE', #10040 ) ;
#7136=CIRCLE ( 'NONE', #33993, 125.0000000000000000 ) ;
#7137=PLANE ( 'NONE',  #38209 ) ;
#7138=CIRCLE ( 'NONE', #17240, 125.0000000000000000 ) ;
#7139=ORIENTED_EDGE ( 'NONE', *, *, #9639, .F. ) ;
#7140=LINE ( 'NONE', #34997, #51560 ) ;
#7142=VECTOR ( 'NONE', #38178, 1000.000000000000000 ) ;
#7143=EDGE_CURVE ( 'NONE', #4089, #44109, #26052, .T. ) ;
#7146=LINE ( 'NONE', #47355, #3018 ) ;
#7150=DIRECTION ( 'NONE',  ( 0.000000000000000000, -0.000000000000000000, -1.000000000000000000 ) ) ;
#7152=ORIENTED_EDGE ( 'NONE', *, *, #46733, .F. ) ;
#7153=VECTOR ( 'NONE', #23108, 1000.000000000000000 ) ;
#7154=PLANE ( 'NONE',  #37492 ) ;
#7155=CIRCLE ( 'NONE', #43234, 125.0000000000000000 ) ;
#7159=CIRCLE ( 'NONE', #5491, 125.0000000000000000 ) ;
#7160=DIRECTION ( 'NONE',  ( -0.000000000000000000, 1.000000000000000000, -0.000000000000000000 ) ) ;
#7162=ORIENTED_EDGE ( 'NONE', *, *, #47228, .T. ) ;
#7163=FACE_OUTER_BOUND ( 'NONE', #21012, .T. ) ;
#7165=PLANE ( 'NONE',  #31516 ) ;
#7169=CARTESIAN_POINT ( 'NONE',  ( -118.4510020108455706, -189.7472609257535510, 103.5805805771131105 ) ) ;
#7171=DIRECTION ( 'NONE',  ( 0.000000000000000000, 1.000000000000000000, 0.000000000000000000 ) ) ;
#7172=CARTESIAN_POINT ( 'NONE',  ( 38.46761263173353740, -175.3837268820161057, 89.80681772907070126 ) ) ;
#7174=CIRCLE ( 'NONE', #44964, 124.9999999999999858 ) ;
#7175=CARTESIAN_POINT ( 'NONE',  ( -146.0653709326077490, -189.7472609257535510, -78.11481899503409920 ) ) ;
#7179=CIRCLE ( 'NONE', #38231, 125.0000000000000000 ) ;
#7180=VECTOR ( 'NONE', #28154, 999.9999999999998863 ) ;
#7183=EDGE_CURVE ( 'NONE', #28621, #13545, #43831, .T. ) ;
#7184=CARTESIAN_POINT ( 'NONE',  ( 76.43863189440992301, -189.7472609257535510, -4.533605064403313456 ) ) ;
#7186=ORIENTED_EDGE ( 'NONE', *, *, #35206, .F. ) ;
#7187=ADVANCED_FACE ( 'NONE', ( #27076 ), #2652, .T. ) ;
#7188=DIRECTION ( 'NONE',  ( 0.000000000000000000, 0.000000000000000000, 1.000000000000000000 ) ) ;
#7189=AXIS2_PLACEMENT_3D ( 'NONE', #28522, #41918, #17234 ) ;
#7190=EDGE_LOOP ( 'NONE', ( #45835, #26788, #46611, #13586 ) ) ;
#7191=DIRECTION ( 'NONE',  ( -0.000000000000000000, 1.000000000000000000, -0.000000000000000000 ) ) ;
#7192=DIRECTION ( 'NONE',  ( 0.000000000000000000, 1.000000000000000000, -0.000000000000000000 ) ) ;
#7193=AXIS2_PLACEMENT_3D ( 'NONE', #9715, #45724, #5268 ) ;
#7194=CARTESIAN_POINT ( 'NONE',  ( 48.47907891923915003, -189.7472609257535510, 78.89300572996904748 ) ) ;
#7196=CARTESIAN_POINT ( 'NONE',  ( 63.31225588004632243, -193.5000000000000000, 55.92572546981597981 ) ) ;
#7198=ORIENTED_EDGE ( 'NONE', *, *, #25301, .F. ) ;
#7199=EDGE_LOOP ( 'NONE', ( #4781, #46901, #43427, #21591 ) ) ;
#7201=VECTOR ( 'NONE', #28325, 1000.000000000000000 ) ;
#7203=DIRECTION ( 'NONE',  ( 0.000000000000000000, -1.000000000000000000, 0.000000000000000000 ) ) ;
#7205=CARTESIAN_POINT ( 'NONE',  ( -172.7479958471414250, -193.5000000000000000, -13.49993235881364129 ) ) ;
#7207=VERTEX_POINT ( 'NONE', #26566 ) ;
#7210=CARTESIAN_POINT ( 'NONE',  ( -70.42295845586433245, -175.3837268820161057, -123.0587999703025019 ) ) ;
#7211=ADVANCED_FACE ( 'NONE', ( #47330 ), #10540, .T. ) ;
#7212=ORIENTED_EDGE ( 'NONE', *, *, #9952, .T. ) ;
#7214=EDGE_CURVE ( 'NONE', #37437, #46596, #34706, .T. ) ;
#7216=CARTESIAN_POINT ( 'NONE',  ( -92.78132261338707565, -193.5000000000000000, -116.8859077982276773 ) ) ;
#7220=CIRCLE ( 'NONE', #19809, 125.0000000000000000 ) ;
#7221=PLANE ( 'NONE',  #15308 ) ;
#7222=DIRECTION ( 'NONE',  ( 0.000000000000000000, 0.000000000000000000, -1.000000000000000000 ) ) ;
#7224=DIRECTION ( 'NONE',  ( 0.000000000000000000, -1.000000000000000000, 0.000000000000000000 ) ) ;
#7225=EDGE_LOOP ( 'NONE', ( #263, #22309, #3050, #45337 ) ) ;
#7226=CARTESIAN_POINT ( 'NONE',  ( -92.78132261338707565, -189.7472609257535510, -116.8859077982276773 ) ) ;
#7227=CIRCLE ( 'NONE', #21484, 125.0000000000000000 ) ;
#7232=LINE ( 'NONE', #23272, #17292 ) ;
#7234=DIRECTION ( 'NONE',  ( 0.8757349421956379665, 0.000000000000000000, -0.4827922027307427477 ) ) ;
#7235=VECTOR ( 'NONE', #21841, 1000.000000000000114 ) ;
#7236=DIRECTION ( 'NONE',  ( 0.000000000000000000, -1.000000000000000000, 0.000000000000000000 ) ) ;
#7238=AXIS2_PLACEMENT_3D ( 'NONE', #33544, #14098, #2515 ) ;
#7239=ORIENTED_EDGE ( 'NONE', *, *, #40386, .T. ) ;
#7240=ORIENTED_EDGE ( 'NONE', *, *, #48747, .F. ) ;
#7242=CARTESIAN_POINT ( 'NONE',  ( 72.14504940832448199, -189.7472609257535510, -32.78426643622660919 ) ) ;
#7243=EDGE_LOOP ( 'NONE', ( #46841, #31688, #51861, #45046 ) ) ;
#7244=ORIENTED_EDGE ( 'NONE', *, *, #26130, .T. ) ;
#7245=DIRECTION ( 'NONE',  ( 0.000000000000000000, 0.000000000000000000, -1.000000000000000000 ) ) ;
#7246=VERTEX_POINT ( 'NONE', #27340 ) ;
#7247=ADVANCED_FACE ( 'NONE', ( #22637 ), #43113, .T. ) ;
#7250=CIRCLE ( 'NONE', #1358, 125.0000000000000000 ) ;
#7251=ORIENTED_EDGE ( 'NONE', *, *, #22156, .F. ) ;
#7252=CARTESIAN_POINT ( 'NONE',  ( 31.84037011350117297, -193.5000000000000000, -94.47107458416898851 ) ) ;
#7255=CARTESIAN_POINT ( 'NONE',  ( -48.47912675150885065, -189.7472609257535510, 6.938893903907228378E-15 ) ) ;
#7257=EDGE_CURVE ( 'NONE', #43502, #18318, #3425, .T. ) ;
#7259=DIRECTION ( 'NONE',  ( -0.000000000000000000, 1.000000000000000000, -0.000000000000000000 ) ) ;
#7261=ORIENTED_EDGE ( 'NONE', *, *, #22182, .T. ) ;
#7262=ORIENTED_EDGE ( 'NONE', *, *, #16746, .F. ) ;
#7265=DIRECTION ( 'NONE',  ( 0.000000000000000000, -0.000000000000000000, -1.000000000000000000 ) ) ;
#7268=AXIS2_PLACEMENT_3D ( 'NONE', #39594, #11233, #23342 ) ;
#7269=PLANE ( 'NONE',  #1012 ) ;
#7273=EDGE_CURVE ( 'NONE', #22800, #9678, #35475, .T. ) ;
#7276=VECTOR ( 'NONE', #49234, 1000.000000000000227 ) ;
#7277=DIRECTION ( 'NONE',  ( 0.9785564922995032555, 0.000000000000000000, 0.2059786187411021818 ) ) ;
#7279=DIRECTION ( 'NONE',  ( 0.000000000000000000, 0.000000000000000000, 1.000000000000000000 ) ) ;
#7280=ORIENTED_EDGE ( 'NONE', *, *, #13146, .T. ) ;
#7282=ADVANCED_FACE ( 'NONE', ( #26822 ), #42853, .T. ) ;
#7283=DIRECTION ( 'NONE',  ( -0.000000000000000000, 1.000000000000000000, -0.000000000000000000 ) ) ;
#7284=CARTESIAN_POINT ( 'NONE',  ( -144.8751831225492595, -189.7472609257535510, 77.99872144864770007 ) ) ;
#7288=DIRECTION ( 'NONE',  ( 0.000000000000000000, 0.000000000000000000, -1.000000000000000000 ) ) ;
#7290=EDGE_CURVE ( 'NONE', #45084, #18433, #39669, .T. ) ;
#7291=ORIENTED_EDGE ( 'NONE', *, *, #37033, .F. ) ;
#7292=CARTESIAN_POINT ( 'NONE',  ( 54.18765407974403558, -177.1207230881787780, -69.53890913632879744 ) ) ;
#7293=VECTOR ( 'NONE', #28230, 1000.000000000000114 ) ;
#7294=LINE ( 'NONE', #3082, #28088 ) ;
#7295=VECTOR ( 'NONE', #17472, 1000.000000000000000 ) ;
#7297=DIRECTION ( 'NONE',  ( -0.000000000000000000, 1.000000000000000000, -0.000000000000000000 ) ) ;
#7299=VECTOR ( 'NONE', #40514, 1000.000000000000114 ) ;
#7300=CARTESIAN_POINT ( 'NONE',  ( -2.700932609314997457, -183.6283474603465606, -116.3157639405751809 ) ) ;
#7301=FACE_OUTER_BOUND ( 'NONE', #42002, .T. ) ;
#7303=CARTESIAN_POINT ( 'NONE',  ( -125.5794209599708751, -177.1207230881787780, 97.11716833071891131 ) ) ;
#7305=DIRECTION ( 'NONE',  ( -0.000000000000000000, 1.000000000000000000, -0.000000000000000000 ) ) ;
#7306=ORIENTED_EDGE ( 'NONE', *, *, #27782, .T. ) ;
#7308=VECTOR ( 'NONE', #19433, 1000.000000000000114 ) ;
#7309=DIRECTION ( 'NONE',  ( -0.9995608365087944591, 0.000000000000000000, 0.02963332782255633305 ) ) ;
#7310=CIRCLE ( 'NONE', #30783, 125.0000000000000000 ) ;
#7312=LINE ( 'NONE', #18864, #29465 ) ;
#7314=PLANE ( 'NONE',  #3604 ) ;
#7315=AXIS2_PLACEMENT_3D ( 'NONE', #1108, #5338, #21352 ) ;
#7316=ORIENTED_EDGE ( 'NONE', *, *, #127, .F. ) ;
#7317=VECTOR ( 'NONE', #48914, 1000.000000000000000 ) ;
#7318=CARTESIAN_POINT ( 'NONE',  ( 12.99855592850622443, -193.5000000000000000, 108.8370090194294875 ) ) ;
#7319=FACE_BOUND ( 'NONE', #20636, .T. ) ;
#7320=ADVANCED_FACE ( 'NONE', ( #34968 ), #15022, .T. ) ;
#7321=LINE ( 'NONE', #14683, #41367 ) ;
#7322=ORIENTED_EDGE ( 'NONE', *, *, #31324, .T. ) ;
#7323=ADVANCED_FACE ( 'NONE', ( #19708 ), #24191, .T. ) ;
#7324=EDGE_CURVE ( 'NONE', #26956, #20647, #7881, .T. ) ;
#7326=FACE_OUTER_BOUND ( 'NONE', #50786, .T. ) ;
#7327=ORIENTED_EDGE ( 'NONE', *, *, #2986, .T. ) ;
#7328=ADVANCED_FACE ( 'NONE', ( #4471 ), #48100, .T. ) ;
#7329=VERTEX_POINT ( 'NONE', #12342 ) ;
#7330=DIRECTION ( 'NONE',  ( 0.7765238627180437447, 0.000000000000000000, -0.6300878435817094392 ) ) ;
#7331=CIRCLE ( 'NONE', #22451, 125.0000000000000000 ) ;
#7332=CIRCLE ( 'NONE', #10664, 125.0000000000000000 ) ;
#7335=DIRECTION ( 'NONE',  ( 0.000000000000000000, 0.000000000000000000, -1.000000000000000000 ) ) ;
#7337=EDGE_CURVE ( 'NONE', #7798, #24942, #15306, .T. ) ;
#7340=LINE ( 'NONE', #19663, #29814 ) ;
#7343=LINE ( 'NONE', #34914, #18039 ) ;
#7345=CIRCLE ( 'NONE', #14893, 125.0000000000000000 ) ;
#7346=EDGE_CURVE ( 'NONE', #51078, #33364, #20235, .T. ) ;
#7347=AXIS2_PLACEMENT_3D ( 'NONE', #20308, #25298, #8479 ) ;
#7348=AXIS2_PLACEMENT_3D ( 'NONE', #11210, #51438, #40105 ) ;
#7349=PLANE ( 'NONE',  #10534 ) ;
#7352=ORIENTED_EDGE ( 'NONE', *, *, #32645, .F. ) ;
#7355=CARTESIAN_POINT ( 'NONE',  ( -8.461066480258370603, -183.6283474603465606, 117.3655938605930231 ) ) ;
#7356=ORIENTED_EDGE ( 'NONE', *, *, #48637, .T. ) ;
#7363=ORIENTED_EDGE ( 'NONE', *, *, #34386, .T. ) ;
#7364=CARTESIAN_POINT ( 'NONE',  ( -48.36085358058748085, -193.5000000000000000, -0.9929810960135100339 ) ) ;
#7366=CARTESIAN_POINT ( 'NONE',  ( -171.7300019102062265, -183.6283474603465606, -20.83798868929513759 ) ) ;
#7368=CARTESIAN_POINT ( 'NONE',  ( -98.10897907742933910, -189.7472609257535510, 114.7252272087849434 ) ) ;
#7369=CARTESIAN_POINT ( 'NONE',  ( -103.4012653778457320, -177.1207230881787780, -112.2878385610366649 ) ) ;
#7370=VERTEX_POINT ( 'NONE', #16296 ) ;
#7372=CARTESIAN_POINT ( 'NONE',  ( -49.21696003055058810, -175.3837268820161057, 0.6749830015182108900 ) ) ;
#7373=ADVANCED_FACE ( 'NONE', ( #9 ), #48360, .T. ) ;
#7374=DIRECTION ( 'NONE',  ( 0.000000000000000000, 1.000000000000000000, 0.000000000000000000 ) ) ;
#7375=DIRECTION ( 'NONE',  ( -0.000000000000000000, 1.000000000000000000, -0.000000000000000000 ) ) ;
#7376=ORIENTED_EDGE ( 'NONE', *, *, #3632, .T. ) ;
#7378=CARTESIAN_POINT ( 'NONE',  ( -171.2727421180348415, -183.6283474603465606, 23.38221600314376047 ) ) ;
#7379=DIRECTION ( 'NONE',  ( -0.1768902751225802927, 0.000000000000000000, 0.9842305779475953864 ) ) ;
#7380=VECTOR ( 'NONE', #34279, 1000.000000000000000 ) ;
#7383=ORIENTED_EDGE ( 'NONE', *, *, #9598, .F. ) ;
#7385=ORIENTED_EDGE ( 'NONE', *, *, #911, .T. ) ;
#7386=EDGE_CURVE ( 'NONE', #40758, #12830, #26207, .T. ) ;
#7387=AXIS2_PLACEMENT_3D ( 'NONE', #33233, #49281, #5661 ) ;
#7391=CARTESIAN_POINT ( 'NONE',  ( 14.37129481273059106, -189.7472609257535510, -108.0501018472328241 ) ) ;
#7392=ORIENTED_EDGE ( 'NONE', *, *, #38552, .F. ) ;
#7394=EDGE_CURVE ( 'NONE', #15211, #30309, #44937, .T. ) ;
#7396=EDGE_CURVE ( 'NONE', #24085, #27896, #8580, .T. ) ;
#7397=VECTOR ( 'NONE', #14707, 1000.000000000000114 ) ;
#7398=EDGE_CURVE ( 'NONE', #25917, #14780, #36299, .T. ) ;
#7400=ORIENTED_EDGE ( 'NONE', *, *, #12054, .F. ) ;
#7405=DIRECTION ( 'NONE',  ( 0.7765238627180393038, 0.000000000000000000, 0.6300878435817147682 ) ) ;
#7407=CARTESIAN_POINT ( 'NONE',  ( -48.30223647638628393, -193.5000000000000000, 0.9842305779476049343 ) ) ;
#7416=PLANE ( 'NONE',  #12109 ) ;
#7417=VECTOR ( 'NONE', #28111, 1000.000000000000000 ) ;
#7419=EDGE_CURVE ( 'NONE', #29336, #9008, #11947, .T. ) ;
#7420=FACE_OUTER_BOUND ( 'NONE', #2762, .T. ) ;
#7421=DIRECTION ( 'NONE',  ( -0.000000000000000000, 1.000000000000000000, -0.000000000000000000 ) ) ;
#7422=DIRECTION ( 'NONE',  ( -0.000000000000000000, 1.000000000000000000, 0.000000000000000000 ) ) ;
#7423=CARTESIAN_POINT ( 'NONE',  ( -138.3664773286545824, -177.1207230881787780, -85.41934182508016704 ) ) ;
#7426=VECTOR ( 'NONE', #6810, 1000.000000000000000 ) ;
#7427=CARTESIAN_POINT ( 'NONE',  ( -132.6364218684650211, -177.1207230881787780, 92.42591454022807795 ) ) ;
#7428=CARTESIAN_POINT ( 'NONE',  ( -48.47912675150885065, -177.1207230881787780, 6.938893903907228378E-15 ) ) ;
#7429=VERTEX_POINT ( 'NONE', #40985 ) ;
#7430=DIRECTION ( 'NONE',  ( -0.4031234292879600778, 0.000000000000000000, -0.9151456172430237901 ) ) ;
#7431=LINE ( 'NONE', #19491, #20645 ) ;
#7432=EDGE_LOOP ( 'NONE', ( #14473, #11227, #18639, #30654 ) ) ;
#7433=DIRECTION ( 'NONE',  ( -0.000000000000000000, 1.000000000000000000, -0.000000000000000000 ) ) ;
#7434=LINE ( 'NONE', #2694, #51679 ) ;
#7435=AXIS2_PLACEMENT_3D ( 'NONE', #3647, #39128, #16013 ) ;
#7438=VERTEX_POINT ( 'NONE', #50191 ) ;
#7439=DIRECTION ( 'NONE',  ( 0.000000000000000000, 0.000000000000000000, 1.000000000000000000 ) ) ;
#7442=CARTESIAN_POINT ( 'NONE',  ( -86.93810158023208601, -193.5000000000000000, 117.8859915627477193 ) ) ;
#7443=PLANE ( 'NONE',  #29070 ) ;
#7444=CARTESIAN_POINT ( 'NONE',  ( -82.43766229206461560, -193.5000000000000000, -119.2602935412679841 ) ) ;
#7445=AXIS2_PLACEMENT_3D ( 'NONE', #26681, #26925, #11408 ) ;
#7447=DIRECTION ( 'NONE',  ( 0.4827922027307490205, 0.000000000000000000, -0.8757349421956345248 ) ) ;
#7449=DIRECTION ( 'NONE',  ( 0.000000000000000000, 0.000000000000000000, -1.000000000000000000 ) ) ;
#7452=ORIENTED_EDGE ( 'NONE', *, *, #22331, .T. ) ;
#7454=EDGE_CURVE ( 'NONE', #11814, #5285, #16171, .T. ) ;
#7455=CARTESIAN_POINT ( 'NONE',  ( 64.44365795514079309, -175.3837268820161057, -53.60452120946194299 ) ) ;
#7456=PLANE ( 'NONE',  #17889 ) ;
#7459=DIRECTION ( 'NONE',  ( 0.000000000000000000, 0.000000000000000000, -1.000000000000000000 ) ) ;
#7460=VERTEX_POINT ( 'NONE', #17092 ) ;
#7463=DIRECTION ( 'NONE',  ( 0.3482016354343928088, 0.000000000000000000, 0.9374196611341231167 ) ) ;
#7465=VERTEX_POINT ( 'NONE', #25224 ) ;
#7466=VERTEX_POINT ( 'NONE', #49415 ) ;
#7467=VERTEX_POINT ( 'NONE', #30202 ) ;
#7468=CIRCLE ( 'NONE', #50278, 125.0000000000000000 ) ;
#7469=CARTESIAN_POINT ( 'NONE',  ( -155.4465502054561057, -177.1207230881787780, 64.67588669375881238 ) ) ;
#7471=PLANE ( 'NONE',  #33297 ) ;
#7473=CARTESIAN_POINT ( 'NONE',  ( -1.771278280434274155, -183.6283474603465606, -115.9455772817710226 ) ) ;
#7474=DIRECTION ( 'NONE',  ( 0.000000000000000000, 1.000000000000000000, 0.000000000000000000 ) ) ;
#7477=CARTESIAN_POINT ( 'NONE',  ( -49.13194886969938580, -183.6283474603465606, 0.7575112421616214675 ) ) ;
#7479=EDGE_CURVE ( 'NONE', #14630, #563, #22882, .T. ) ;
#7482=ORIENTED_EDGE ( 'NONE', *, *, #16794, .T. ) ;
#7483=DIRECTION ( 'NONE',  ( -0.000000000000000000, 1.000000000000000000, -0.000000000000000000 ) ) ;
#7486=EDGE_LOOP ( 'NONE', ( #17888, #47227, #7625, #15498 ) ) ;
#7490=CARTESIAN_POINT ( 'NONE',  ( -82.43766229206461560, -177.1207230881787780, -119.2602935412679983 ) ) ;
#7492=CARTESIAN_POINT ( 'NONE',  ( 76.28370911321320591, -183.6283474603465606, -7.696413904697499753 ) ) ;
#7493=ORIENTED_EDGE ( 'NONE', *, *, #3836, .T. ) ;
#7494=LINE ( 'NONE', #47179, #42245 ) ;
#7495=CARTESIAN_POINT ( 'NONE',  ( -121.0298553105864414, -177.1207230881787780, -100.5610240384919081 ) ) ;
#7498=PLANE ( 'NONE',  #38124 ) ;
#7499=CARTESIAN_POINT ( 'NONE',  ( -172.1767935149754294, -193.5000000000000000, 8.665274887906335266 ) ) ;
#7500=DIRECTION ( 'NONE',  ( -0.6528221181905280446, 0.000000000000000000, 0.7575112421616145841 ) ) ;
#7504=ORIENTED_EDGE ( 'NONE', *, *, #50052, .F. ) ;
#7505=VERTEX_POINT ( 'NONE', #45716 ) ;
#7506=DIRECTION ( 'NONE',  ( 0.000000000000000000, 0.000000000000000000, 1.000000000000000000 ) ) ;
#7510=DIRECTION ( 'NONE',  ( 0.000000000000000000, -1.000000000000000000, 0.000000000000000000 ) ) ;
#7511=EDGE_CURVE ( 'NONE', #16448, #12506, #46243, .T. ) ;
#7512=CARTESIAN_POINT ( 'NONE',  ( -47.74129347246713451, -177.1207230881787780, 0.6749830015182212151 ) ) ;
#7513=EDGE_CURVE ( 'NONE', #20061, #11975, #13397, .T. ) ;
#7515=AXIS2_PLACEMENT_3D ( 'NONE', #20167, #36186, #40914 ) ;
#7520=DIRECTION ( 'NONE',  ( -0.000000000000000000, 1.000000000000000000, -0.000000000000000000 ) ) ;
#7521=CIRCLE ( 'NONE', #36891, 125.0000000000000000 ) ;
#7523=CARTESIAN_POINT ( 'NONE',  ( -162.9896759831412965, -177.1207230881787780, -50.12318939043961308 ) ) ;
#7525=ORIENTED_EDGE ( 'NONE', *, *, #6272, .F. ) ;
#7527=DIRECTION ( 'NONE',  ( 0.000000000000000000, 0.000000000000000000, 1.000000000000000000 ) ) ;
#7529=EDGE_CURVE ( 'NONE', #29784, #17455, #43021, .T. ) ;
#7531=PLANE ( 'NONE',  #6053 ) ;
#7533=VERTEX_POINT ( 'NONE', #9709 ) ;
#7534=VECTOR ( 'NONE', #32787, 1000.000000000000114 ) ;
#7535=CARTESIAN_POINT ( 'NONE',  ( -49.17567778057185990, -183.6283474603465606, 0.7175072570443320474 ) ) ;
#7536=ORIENTED_EDGE ( 'NONE', *, *, #24433, .F. ) ;
#7538=ORIENTED_EDGE ( 'NONE', *, *, #33519, .T. ) ;
#7539=EDGE_LOOP ( 'NONE', ( #22858, #5471, #13616, #44308 ) ) ;
#7540=FACE_OUTER_BOUND ( 'NONE', #41794, .T. ) ;
#7542=LINE ( 'NONE', #31713, #42267 ) ;
#7546=VERTEX_POINT ( 'NONE', #21548 ) ;
#7548=DIRECTION ( 'NONE',  ( 0.6068001458185890984, 0.000000000000000000, 0.7948544414133565938 ) ) ;
#7549=PLANE ( 'NONE',  #40691 ) ;
#7551=DIRECTION ( 'NONE',  ( 0.9929810960135161402, 0.000000000000000000, 0.1182731709213730997 ) ) ;
#7553=DIRECTION ( 'NONE',  ( 0.6068001458185945385, 0.000000000000000000, -0.7948544414133523750 ) ) ;
#7554=EDGE_CURVE ( 'NONE', #49617, #16076, #17611, .T. ) ;
#7556=CARTESIAN_POINT ( 'NONE',  ( -131.9398708394020332, -193.5000000000000000, 91.70840728318374602 ) ) ;
#7560=CARTESIAN_POINT ( 'NONE',  ( -48.47912675150885065, -175.3837268820161057, 6.938893903907228378E-15 ) ) ;
#7562=CARTESIAN_POINT ( 'NONE',  ( -173.4190745413846741, -189.7472609257535510, -3.874202661595026687 ) ) ;
#7563=FACE_OUTER_BOUND ( 'NONE', #22219, .T. ) ;
#7566=ADVANCED_FACE ( 'NONE', ( #1814 ), #34140, .T. ) ;
#7567=ORIENTED_EDGE ( 'NONE', *, *, #39485, .T. ) ;
#7568=EDGE_CURVE ( 'NONE', #25658, #40221, #33371, .T. ) ;
#7569=EDGE_CURVE ( 'NONE', #20596, #32896, #42014, .T. ) ;
#7570=AXIS2_PLACEMENT_3D ( 'NONE', #37377, #21091, #12676 ) ;
#7571=VECTOR ( 'NONE', #10666, 1000.000000000000000 ) ;
#7573=ADVANCED_FACE ( 'NONE', ( #25477 ), #46753, .T. ) ;
#7574=FACE_BOUND ( 'NONE', #43085, .T. ) ;
#7576=DIRECTION ( 'NONE',  ( 0.000000000000000000, 1.000000000000000000, 0.000000000000000000 ) ) ;
#7578=EDGE_LOOP ( 'NONE', ( #11648, #40783, #16733, #14126 ) ) ;
#7579=CARTESIAN_POINT ( 'NONE',  ( 116.9235303384055840, -193.5000000000000000, 2.819679052520814125E-14 ) ) ;
#7580=VECTOR ( 'NONE', #40383, 1000.000000000000000 ) ;
#7581=ORIENTED_EDGE ( 'NONE', *, *, #2266, .T. ) ;
#7582=LINE ( 'NONE', #19928, #16690 ) ;
#7584=DIRECTION ( 'NONE',  ( 0.1182731709213660498, 0.000000000000000000, -0.9929810960135169173 ) ) ;
#7585=ORIENTED_EDGE ( 'NONE', *, *, #43170, .T. ) ;
#7589=ORIENTED_EDGE ( 'NONE', *, *, #32049, .T. ) ;
#7590=CARTESIAN_POINT ( 'NONE',  ( -48.47912675150885065, -177.1207230881787780, 6.938893903907228378E-15 ) ) ;
#7592=CARTESIAN_POINT ( 'NONE',  ( -169.6719064342497632, -193.5000000000000000, 30.61552143554992256 ) ) ;
#7596=FACE_OUTER_BOUND ( 'NONE', #9269, .T. ) ;
#7597=DIRECTION ( 'NONE',  ( 0.000000000000000000, 0.000000000000000000, 1.000000000000000000 ) ) ;
#7600=CIRCLE ( 'NONE', #21034, 125.0000000000000000 ) ;
#7603=CARTESIAN_POINT ( 'NONE',  ( 53.18081239921338721, -193.5000000000000000, -72.73415134495935774 ) ) ;
#7604=DIRECTION ( 'NONE',  ( 0.1476465640024851034, 0.000000000000000000, -0.9890401873221634776 ) ) ;
#7606=DIRECTION ( 'NONE',  ( 0.000000000000000000, -1.000000000000000000, -0.000000000000000000 ) ) ;
#7607=LINE ( 'NONE', #48337, #24078 ) ;
#7610=EDGE_CURVE ( 'NONE', #19801, #34735, #46489, .T. ) ;
#7611=ORIENTED_EDGE ( 'NONE', *, *, #36528, .F. ) ;
#7612=EDGE_CURVE ( 'NONE', #47296, #8540, #34400, .T. ) ;
#7616=EDGE_CURVE ( 'NONE', #33685, #37521, #42187, .T. ) ;
#7618=ORIENTED_EDGE ( 'NONE', *, *, #24791, .F. ) ;
#7619=AXIS2_PLACEMENT_3D ( 'NONE', #49018, #28254, #43766 ) ;
#7620=FACE_OUTER_BOUND ( 'NONE', #29471, .T. ) ;
#7621=EDGE_CURVE ( 'NONE', #49340, #1605, #249, .T. ) ;
#7622=FACE_OUTER_BOUND ( 'NONE', #36688, .T. ) ;
#7624=ORIENTED_EDGE ( 'NONE', *, *, #44298, .F. ) ;
#7625=ORIENTED_EDGE ( 'NONE', *, *, #31760, .F. ) ;
#7626=EDGE_CURVE ( 'NONE', #12568, #44736, #6284, .T. ) ;
#7628=EDGE_CURVE ( 'NONE', #36353, #43146, #10741, .T. ) ;
#7630=EDGE_CURVE ( 'NONE', #3016, #34125, #19397, .T. ) ;
#7631=CARTESIAN_POINT ( 'NONE',  ( -105.4063847101409692, -193.5000000000000000, -111.2847127925096231 ) ) ;
#7634=VECTOR ( 'NONE', #14741, 1000.000000000000000 ) ;
#7635=EDGE_CURVE ( 'NONE', #8800, #31552, #7321, .T. ) ;
#7639=VERTEX_POINT ( 'NONE', #30699 ) ;
#7640=EDGE_LOOP ( 'NONE', ( #9583, #33327, #8863, #351 ) ) ;
#7641=VERTEX_POINT ( 'NONE', #18873 ) ;
#7642=CARTESIAN_POINT ( 'NONE',  ( -47.92047998570519951, -175.3837268820161057, -0.8294056854501942189 ) ) ;
#7643=ORIENTED_EDGE ( 'NONE', *, *, #31432, .F. ) ;
#7645=LINE ( 'NONE', #272, #33449 ) ;
#7646=LINE ( 'NONE', #11316, #39476 ) ;
#7647=LINE ( 'NONE', #19469, #38404 ) ;
#7648=LINE ( 'NONE', #31556, #2280 ) ;
#7649=VERTEX_POINT ( 'NONE', #38334 ) ;
#7650=VECTOR ( 'NONE', #39252, 1000.000000000000114 ) ;
#7651=LINE ( 'NONE', #23670, #43237 ) ;
#7653=PLANE ( 'NONE',  #39830 ) ;
#7654=ORIENTED_EDGE ( 'NONE', *, *, #12911, .F. ) ;
#7655=CARTESIAN_POINT ( 'NONE',  ( -48.88225018079683082, -175.3837268820161057, 0.9151456172430223468 ) ) ;
#7657=DIRECTION ( 'NONE',  ( 0.4566292373937140270, 0.000000000000000000, -0.8896570909947467687 ) ) ;
#7659=ORIENTED_EDGE ( 'NONE', *, *, #19340, .T. ) ;
#7660=ADVANCED_FACE ( 'NONE', ( #15468 ), #50963, .T. ) ;
#7664=CARTESIAN_POINT ( 'NONE',  ( -98.31070548515600649, -175.3837268820161057, -113.5465278748093283 ) ) ;
#7667=CARTESIAN_POINT ( 'NONE',  ( 24.07160180756802248, -177.1207230881787780, 100.5610240384924481 ) ) ;
#7668=EDGE_CURVE ( 'NONE', #33506, #13423, #50444, .T. ) ;
#7671=ORIENTED_EDGE ( 'NONE', *, *, #33572, .F. ) ;
#7672=EDGE_CURVE ( 'NONE', #37490, #2274, #35165, .T. ) ;
#7673=CARTESIAN_POINT ( 'NONE',  ( -111.8989814360438828, -175.3837268820161057, -107.7168604805787027 ) ) ;
#7679=ORIENTED_EDGE ( 'NONE', *, *, #14775, .F. ) ;
#7683=PLANE ( 'NONE',  #50430 ) ;
#7684=DIRECTION ( 'NONE',  ( 0.000000000000000000, 0.000000000000000000, 1.000000000000000000 ) ) ;
#7685=DIRECTION ( 'NONE',  ( 0.000000000000000000, 1.000000000000000000, -0.000000000000000000 ) ) ;
#7687=AXIS2_PLACEMENT_3D ( 'NONE', #37291, #8919, #33361 ) ;
#7691=EDGE_CURVE ( 'NONE', #47822, #40259, #35951, .T. ) ;
#7693=LINE ( 'NONE', #4018, #30576 ) ;
#7694=FACE_OUTER_BOUND ( 'NONE', #20998, .T. ) ;
#7696=EDGE_CURVE ( 'NONE', #11813, #50878, #27538, .T. ) ;
#7698=CARTESIAN_POINT ( 'NONE',  ( -48.47912675150885065, -177.1207230881787780, 6.938893903907228378E-15 ) ) ;
#7699=EDGE_CURVE ( 'NONE', #30689, #22103, #8353, .T. ) ;
#7700=DIRECTION ( 'NONE',  ( -0.000000000000000000, 1.000000000000000000, -0.000000000000000000 ) ) ;
#7701=EDGE_LOOP ( 'NONE', ( #43956, #43100, #44629, #42896 ) ) ;
#7703=CARTESIAN_POINT ( 'NONE',  ( -17.07133635870350474, -193.5000000000000000, -119.9572859573364809 ) ) ;
#7705=CARTESIAN_POINT ( 'NONE',  ( -171.4559849729830603, -177.1207230881787780, 22.39848972532370297 ) ) ;
#7706=CARTESIAN_POINT ( 'NONE',  ( 24.63024857337166296, -183.6283474603465606, 101.3904297239426597 ) ) ;
#7710=VECTOR ( 'NONE', #29326, 1000.000000000000114 ) ;
#7712=ORIENTED_EDGE ( 'NONE', *, *, #23677, .F. ) ;
#7716=DIRECTION ( 'NONE',  ( 0.000000000000000000, 0.000000000000000000, 1.000000000000000000 ) ) ;
#7718=DIRECTION ( 'NONE',  ( 0.000000000000000000, 0.000000000000000000, 1.000000000000000000 ) ) ;
#7719=DIRECTION ( 'NONE',  ( -0.000000000000000000, 1.000000000000000000, -0.000000000000000000 ) ) ;
#7720=DIRECTION ( 'NONE',  ( 0.000000000000000000, 0.000000000000000000, -1.000000000000000000 ) ) ;
#7722=LINE ( 'NONE', #44244, #17162 ) ;
#7725=VECTOR ( 'NONE', #41042, 1000.000000000000000 ) ;
#7730=VECTOR ( 'NONE', #26394, 1000.000000000000114 ) ;
#7731=DIRECTION ( 'NONE',  ( 0.000000000000000000, 0.000000000000000000, 1.000000000000000000 ) ) ;
#7732=DIRECTION ( 'NONE',  ( 0.2059786187411021818, 0.000000000000000000, -0.9785564922995032555 ) ) ;
#7736=ADVANCED_FACE ( 'NONE', ( #28042 ), #4399, .T. ) ;
#7738=ADVANCED_FACE ( 'NONE', ( #23851 ), #48034, .T. ) ;
#7739=VERTEX_POINT ( 'NONE', #12014 ) ;
#7740=DIRECTION ( 'NONE',  ( 0.3482016354343928088, 0.000000000000000000, 0.9374196611341231167 ) ) ;
#7741=VERTEX_POINT ( 'NONE', #40381 ) ;
#7742=DIRECTION ( 'NONE',  ( 0.000000000000000000, -1.000000000000000000, 0.000000000000000000 ) ) ;
#7743=PLANE ( 'NONE',  #12725 ) ;
#7744=ORIENTED_EDGE ( 'NONE', *, *, #31762, .T. ) ;
#7746=LINE ( 'NONE', #44273, #33104 ) ;
#7747=CARTESIAN_POINT ( 'NONE',  ( -60.86541030502398542, -193.5000000000000000, -124.3848060646151623 ) ) ;
#7749=EDGE_LOOP ( 'NONE', ( #39788, #5617, #9091, #44000 ) ) ;
#7752=VERTEX_POINT ( 'NONE', #51729 ) ;
#7753=ADVANCED_FACE ( 'NONE', ( #28566 ), #15738, .F. ) ;
#7754=DIRECTION ( 'NONE',  ( 0.000000000000000000, 0.000000000000000000, 1.000000000000000000 ) ) ;
#7756=VERTEX_POINT ( 'NONE', #8089 ) ;
#7758=AXIS2_PLACEMENT_3D ( 'NONE', #28101, #8153, #28372 ) ;
#7759=VECTOR ( 'NONE', #40814, 1000.000000000000000 ) ;
#7760=ADVANCED_FACE ( 'NONE', ( #20425 ), #12278, .T. ) ;
#7766=CARTESIAN_POINT ( 'NONE',  ( -145.6517069852672535, -175.3837268820161057, 78.62880929222946236 ) ) ;
#7767=ORIENTED_EDGE ( 'NONE', *, *, #10184, .F. ) ;
#7768=CARTESIAN_POINT ( 'NONE',  ( -48.47912675150885065, -173.5000000000000284, 6.938893903907228378E-15 ) ) ;
#7769=DIRECTION ( 'NONE',  ( 0.000000000000000000, -1.000000000000000000, 0.000000000000000000 ) ) ;
#7772=ORIENTED_EDGE ( 'NONE', *, *, #39805, .F. ) ;
#7773=ORIENTED_EDGE ( 'NONE', *, *, #50142, .F. ) ;
#7774=EDGE_LOOP ( 'NONE', ( #9567, #13765, #29041, #7306 ) ) ;
#7775=CARTESIAN_POINT ( 'NONE',  ( -49.47868758801764955, -183.6283474603465606, 0.02963332782255607284 ) ) ;
#7776=PLANE ( 'NONE',  #18452 ) ;
#7777=CARTESIAN_POINT ( 'NONE',  ( 12.12533326292403935, -177.1207230881787780, 109.3256576763158989 ) ) ;
#7778=DIRECTION ( 'NONE',  ( -0.000000000000000000, 1.000000000000000000, 0.000000000000000000 ) ) ;
#7779=CARTESIAN_POINT ( 'NONE',  ( -49.44376233341721161, -189.7472609257535510, 0.2635871660690650709 ) ) ;
#7780=VECTOR ( 'NONE', #15705, 1000.000000000000114 ) ;
#7781=ORIENTED_EDGE ( 'NONE', *, *, #1926, .F. ) ;
#7782=AXIS2_PLACEMENT_3D ( 'NONE', #21547, #9451, #1567 ) ;
#7783=LINE ( 'NONE', #44041, #26567 ) ;
#7789=CARTESIAN_POINT ( 'NONE',  ( -171.5592422664403216, -177.1207230881787780, -21.82395850507255730 ) ) ;
#7792=DIRECTION ( 'NONE',  ( 0.7948544414133481562, 0.000000000000000000, 0.6068001458186002006 ) ) ;
#7793=EDGE_LOOP ( 'NONE', ( #12139, #28740, #44840, #9937 ) ) ;
#7794=DIRECTION ( 'NONE',  ( -0.2920567706369628924, 0.000000000000000000, -0.9564009842765264224 ) ) ;
#7795=AXIS2_PLACEMENT_3D ( 'NONE', #29986, #17658, #26554 ) ;
#7796=ORIENTED_EDGE ( 'NONE', *, *, #27978, .T. ) ;
#7798=VERTEX_POINT ( 'NONE', #32521 ) ;
#7800=CIRCLE ( 'NONE', #252, 125.0000000000000000 ) ;
#7801=CARTESIAN_POINT ( 'NONE',  ( -171.9838957966129556, -175.3837268820161057, 19.27620354518722579 ) ) ;
#7802=PLANE ( 'NONE',  #26520 ) ;
#7803=DIRECTION ( 'NONE',  ( -0.000000000000000000, 1.000000000000000000, 0.000000000000000000 ) ) ;
#7804=FACE_OUTER_BOUND ( 'NONE', #35519, .T. ) ;
#7806=ORIENTED_EDGE ( 'NONE', *, *, #26435, .F. ) ;
#7807=DIRECTION ( 'NONE',  ( 0.000000000000000000, 0.000000000000000000, -1.000000000000000000 ) ) ;
#7809=FACE_BOUND ( 'NONE', #36195, .T. ) ;
#7811=ADVANCED_FACE ( 'NONE', ( #31747 ), #19917, .T. ) ;
#7815=ORIENTED_EDGE ( 'NONE', *, *, #28313, .T. ) ;
#7818=VECTOR ( 'NONE', #11116, 1000.000000000000000 ) ;
#7820=FACE_OUTER_BOUND ( 'NONE', #2838, .T. ) ;
#7821=FACE_BOUND ( 'NONE', #51422, .T. ) ;
#7822=CARTESIAN_POINT ( 'NONE',  ( -118.4510020108455137, -175.3837268820161057, 103.5805805771131674 ) ) ;
#7823=DIRECTION ( 'NONE',  ( 0.000000000000000000, 1.000000000000000000, 0.000000000000000000 ) ) ;
#7824=AXIS2_PLACEMENT_3D ( 'NONE', #16735, #32741, #49495 ) ;
#7825=ORIENTED_EDGE ( 'NONE', *, *, #25536, .T. ) ;
#7826=ORIENTED_EDGE ( 'NONE', *, *, #20880, .F. ) ;
#7830=DIRECTION ( 'NONE',  ( 0.000000000000000000, 0.000000000000000000, 1.000000000000000000 ) ) ;
#7831=CYLINDRICAL_SURFACE ( 'NONE', #35581, 124.9999999999999858 ) ;
#7832=EDGE_CURVE ( 'NONE', #43249, #29810, #4664, .T. ) ;
#7833=VECTOR ( 'NONE', #13841, 1000.000000000000114 ) ;
#7836=CARTESIAN_POINT ( 'NONE',  ( -238.7407812814481076, -193.5000000000000000, 41.45482488023466772 ) ) ;
#7837=EDGE_LOOP ( 'NONE', ( #44372, #24003, #15933, #3287 ) ) ;
#7840=ORIENTED_EDGE ( 'NONE', *, *, #42644, .T. ) ;
#7841=ORIENTED_EDGE ( 'NONE', *, *, #6568, .F. ) ;
#7842=CARTESIAN_POINT ( 'NONE',  ( 74.49773146996547268, -193.5000000000000000, -22.39848972532282190 ) ) ;
#7845=AXIS2_PLACEMENT_3D ( 'NONE', #9437, #24951, #49127 ) ;
#7846=ORIENTED_EDGE ( 'NONE', *, *, #51029, .F. ) ;
#7849=VERTEX_POINT ( 'NONE', #45922 ) ;
#7850=FACE_OUTER_BOUND ( 'NONE', #46171, .T. ) ;
#7853=VECTOR ( 'NONE', #9958, 1000.000000000000000 ) ;
#7854=DIRECTION ( 'NONE',  ( 0.000000000000000000, 1.000000000000000000, 0.000000000000000000 ) ) ;
#7855=EDGE_LOOP ( 'NONE', ( #14842, #46364, #9836, #22020 ) ) ;
#7856=CYLINDRICAL_SURFACE ( 'NONE', #23673, 125.0000000000000000 ) ;
#7858=FACE_OUTER_BOUND ( 'NONE', #27571, .T. ) ;
#7859=DIRECTION ( 'NONE',  ( -0.000000000000000000, 1.000000000000000000, -0.000000000000000000 ) ) ;
#7865=AXIS2_PLACEMENT_3D ( 'NONE', #40931, #5470, #17294 ) ;
#7867=DIRECTION ( 'NONE',  ( 0.8294056854501971054, 0.000000000000000000, 0.5586467658036594619 ) ) ;
#7872=EDGE_CURVE ( 'NONE', #43059, #34819, #12795, .T. ) ;
#7873=DIRECTION ( 'NONE',  ( -0.6068001458185834363, 0.000000000000000000, -0.7948544414133608127 ) ) ;
#7874=DIRECTION ( 'NONE',  ( 0.000000000000000000, -0.000000000000000000, 1.000000000000000000 ) ) ;
#7876=EDGE_LOOP ( 'NONE', ( #28812, #8689, #30986, #23421 ) ) ;
#7877=ORIENTED_EDGE ( 'NONE', *, *, #31260, .F. ) ;
#7879=CARTESIAN_POINT ( 'NONE',  ( -128.2395503755045638, -193.5000000000000000, -96.24590808611419845 ) ) ;
#7880=CARTESIAN_POINT ( 'NONE',  ( -123.6678354051270361, -175.3837268820161057, 99.85818990449065780 ) ) ;
#7881=LINE ( 'NONE', #51796, #10279 ) ;
#7883=EDGE_LOOP ( 'NONE', ( #30706, #18480, #34853, #9386 ) ) ;
#7884=VECTOR ( 'NONE', #31790, 1000.000000000000114 ) ;
#7886=AXIS2_PLACEMENT_3D ( 'NONE', #33543, #17000, #49322 ) ;
#7887=VERTEX_POINT ( 'NONE', #28818 ) ;
#7889=ORIENTED_EDGE ( 'NONE', *, *, #24198, .F. ) ;
#7890=DIRECTION ( 'NONE',  ( 0.000000000000000000, -1.000000000000000000, 0.000000000000000000 ) ) ;
#7891=EDGE_CURVE ( 'NONE', #50412, #4631, #33810, .T. ) ;
#7892=EDGE_CURVE ( 'NONE', #38978, #177, #48826, .T. ) ;
#7895=CARTESIAN_POINT ( 'NONE',  ( 52.59568867645217694, -175.3837268820161057, -73.54509967498590584 ) ) ;
#7899=VERTEX_POINT ( 'NONE', #45656 ) ;
#7900=CARTESIAN_POINT ( 'NONE',  ( -167.8725343822893308, -189.7472609257535510, 33.48461921608600278 ) ) ;
#7903=ORIENTED_EDGE ( 'NONE', *, *, #32107, .F. ) ;
#7907=CARTESIAN_POINT ( 'NONE',  ( -5.113431607746556473, -175.3837268820161057, 117.2365833888819537 ) ) ;
#7908=DIRECTION ( 'NONE',  ( -0.000000000000000000, 1.000000000000000000, -0.000000000000000000 ) ) ;
#7910=DIRECTION ( 'NONE',  ( -0.000000000000000000, 1.000000000000000000, -0.000000000000000000 ) ) ;
#7913=EDGE_LOOP ( 'NONE', ( #14974, #46672, #40570, #40143 ) ) ;
#7915=DIRECTION ( 'NONE',  ( 0.000000000000000000, -1.000000000000000000, 0.000000000000000000 ) ) ;
#7916=AXIS2_PLACEMENT_3D ( 'NONE', #34165, #49941, #2091 ) ;
#7917=DIRECTION ( 'NONE',  ( 0.000000000000000000, 0.000000000000000000, 1.000000000000000000 ) ) ;
#7918=EDGE_CURVE ( 'NONE', #4861, #47386, #9911, .T. ) ;
#7919=AXIS2_PLACEMENT_3D ( 'NONE', #47573, #11555, #24172 ) ;
#7920=ORIENTED_EDGE ( 'NONE', *, *, #42864, .F. ) ;
#7921=CARTESIAN_POINT ( 'NONE',  ( -48.47912675150885065, -183.6283474603465606, 6.938893903907228378E-15 ) ) ;
#7922=LINE ( 'NONE', #40237, #9697 ) ;
#7923=VECTOR ( 'NONE', #26628, 1000.000000000000000 ) ;
#7925=CARTESIAN_POINT ( 'NONE',  ( -112.1919339979530150, -193.5000000000000000, 107.5438431188761683 ) ) ;
#7926=ORIENTED_EDGE ( 'NONE', *, *, #5015, .T. ) ;
#7927=EDGE_CURVE ( 'NONE', #19399, #34600, #8612, .T. ) ;
#7928=CARTESIAN_POINT ( 'NONE',  ( 62.86098202833237281, -177.1207230881787780, 56.81883646197908178 ) ) ;
#7929=DIRECTION ( 'NONE',  ( 0.000000000000000000, 0.000000000000000000, 1.000000000000000000 ) ) ;
#7933=VECTOR ( 'NONE', #5929, 1000.000000000000000 ) ;
#7935=CARTESIAN_POINT ( 'NONE',  ( -173.3968853974275817, -193.5000000000000000, 4.533605064404221174 ) ) ;
#7937=LINE ( 'NONE', #16359, #34570 ) ;
#7938=ORIENTED_EDGE ( 'NONE', *, *, #22212, .T. ) ;
#7939=EDGE_LOOP ( 'NONE', ( #47860, #40135, #36916, #37177 ) ) ;
#7940=LINE ( 'NONE', #48167, #38346 ) ;
#7943=EDGE_LOOP ( 'NONE', ( #45610, #39335, #1304, #15720 ) ) ;
#7944=ORIENTED_EDGE ( 'NONE', *, *, #7635, .T. ) ;
#7948=CARTESIAN_POINT ( 'NONE',  ( -151.4272465800706016, -193.5000000000000000, 70.89911581792887318 ) ) ;
#7949=AXIS2_PLACEMENT_3D ( 'NONE', #23873, #28336, #35439 ) ;
#7951=EDGE_CURVE ( 'NONE', #44345, #13008, #41951, .T. ) ;
#7952=EDGE_CURVE ( 'NONE', #3318, #6819, #37991, .T. ) ;
#7953=EDGE_CURVE ( 'NONE', #49860, #44109, #15346, .T. ) ;
#7954=CARTESIAN_POINT ( 'NONE',  ( -33.64434644548592246, -193.5000000000000000, -123.1094209424468033 ) ) ;
#7958=VECTOR ( 'NONE', #51574, 1000.000000000000000 ) ;
#7959=EDGE_CURVE ( 'NONE', #13211, #3068, #33562, .T. ) ;
#7960=ORIENTED_EDGE ( 'NONE', *, *, #22546, .T. ) ;
#7961=LINE ( 'NONE', #27682, #47641 ) ;
#7962=FACE_OUTER_BOUND ( 'NONE', #51343, .T. ) ;
#7964=EDGE_CURVE ( 'NONE', #36635, #34754, #35469, .T. ) ;
#7965=CIRCLE ( 'NONE', #33147, 125.0000000000000000 ) ;
#7966=CARTESIAN_POINT ( 'NONE',  ( 71.09073365861578964, -193.5000000000000000, 32.84887689123991095 ) ) ;
#7968=DIRECTION ( 'NONE',  ( 0.000000000000000000, -1.000000000000000000, 0.000000000000000000 ) ) ;
#7969=ORIENTED_EDGE ( 'NONE', *, *, #28044, .F. ) ;
#7970=CARTESIAN_POINT ( 'NONE',  ( -69.77312546433407192, -189.7472609257535510, 123.1729094355500109 ) ) ;
#7973=AXIS2_PLACEMENT_3D ( 'NONE', #1656, #30529, #6640 ) ;
#7974=LINE ( 'NONE', #51614, #21460 ) ;
#7975=PLANE ( 'NONE',  #2257 ) ;
#7976=EDGE_CURVE ( 'NONE', #43746, #18062, #2281, .T. ) ;
#7977=VECTOR ( 'NONE', #15752, 1000.000000000000000 ) ;
#7978=ORIENTED_EDGE ( 'NONE', *, *, #47786, .T. ) ;
#7979=ORIENTED_EDGE ( 'NONE', *, *, #21, .T. ) ;
#7981=CARTESIAN_POINT ( 'NONE',  ( 54.46899307705341187, -183.6283474603465606, -70.89911581792813422 ) ) ;
#7983=CARTESIAN_POINT ( 'NONE',  ( -47.92047998570520662, -193.5000000000000000, 0.8294056854502119824 ) ) ;
#7984=ORIENTED_EDGE ( 'NONE', *, *, #11823, .F. ) ;
#7987=FACE_OUTER_BOUND ( 'NONE', #34257, .T. ) ;
#7988=CARTESIAN_POINT ( 'NONE',  ( -147.0463339291295881, -193.5000000000000000, 76.87330921200150158 ) ) ;
#7989=VERTEX_POINT ( 'NONE', #46175 ) ;
#7990=DIRECTION ( 'NONE',  ( -0.000000000000000000, 1.000000000000000000, -0.000000000000000000 ) ) ;
#7993=CARTESIAN_POINT ( 'NONE',  ( -56.71246971489870958, -175.3837268820161057, -124.7285535218267682 ) ) ;
#7994=ORIENTED_EDGE ( 'NONE', *, *, #39488, .T. ) ;
#7996=AXIS2_PLACEMENT_3D ( 'NONE', #6078, #22872, #30750 ) ;
#7997=CARTESIAN_POINT ( 'NONE',  ( -48.30223647638627682, -189.7472609257535510, -0.9842305779475897243 ) ) ;
#8000=VECTOR ( 'NONE', #32498, 1000.000000000000000 ) ;
#8003=CARTESIAN_POINT ( 'NONE',  ( -48.47912675150885065, -189.7472609257535510, 6.938893903907228378E-15 ) ) ;
#8006=AXIS2_PLACEMENT_3D ( 'NONE', #48813, #51989, #48286 ) ;
#8007=ORIENTED_EDGE ( 'NONE', *, *, #1732, .T. ) ;
#8009=ORIENTED_EDGE ( 'NONE', *, *, #20558, .T. ) ;
#8010=ORIENTED_EDGE ( 'NONE', *, *, #3104, .F. ) ;
#8011=AXIS2_PLACEMENT_3D ( 'NONE', #51183, #34854, #3067 ) ;
#8012=FACE_OUTER_BOUND ( 'NONE', #36713, .T. ) ;
#8013=CARTESIAN_POINT ( 'NONE',  ( 37.77106160267053525, -193.5000000000000000, 89.08931047202635511 ) ) ;
#8014=ORIENTED_EDGE ( 'NONE', *, *, #8574, .F. ) ;
#8015=VECTOR ( 'NONE', #4480, 1000.000000000000114 ) ;
#8016=ORIENTED_EDGE ( 'NONE', *, *, #15519, .T. ) ;
#8017=DIRECTION ( 'NONE',  ( 1.000000000000000000, 0.000000000000000000, -0.000000000000000000 ) ) ;
#8018=CIRCLE ( 'NONE', #37387, 125.0000000000000000 ) ;
#8019=CIRCLE ( 'NONE', #37391, 125.0000000000000000 ) ;
#8020=DIRECTION ( 'NONE',  ( -0.9266896074318291543, 0.000000000000000000, -0.3758275821142488260 ) ) ;
#8023=DIRECTION ( 'NONE',  ( 0.000000000000000000, 0.000000000000000000, -1.000000000000000000 ) ) ;
#8025=CARTESIAN_POINT ( 'NONE',  ( 66.03142248012326831, -183.6283474603465606, 50.12318939044041599 ) ) ;
#8026=DIRECTION ( 'NONE',  ( -0.4566292373937140270, 0.000000000000000000, 0.8896570909947467687 ) ) ;
#8027=EDGE_CURVE ( 'NONE', #10828, #25168, #51165, .T. ) ;
#8028=ADVANCED_FACE ( 'NONE', ( #6493 ), #46426, .T. ) ;
#8029=DIRECTION ( 'NONE',  ( 0.000000000000000000, 0.000000000000000000, -1.000000000000000000 ) ) ;
#8031=ORIENTED_EDGE ( 'NONE', *, *, #26186, .T. ) ;
#8034=ORIENTED_EDGE ( 'NONE', *, *, #32087, .F. ) ;
#8035=EDGE_CURVE ( 'NONE', #2659, #10865, #28787, .T. ) ;
#8036=LINE ( 'NONE', #36147, #20731 ) ;
#8038=CIRCLE ( 'NONE', #30684, 125.0000000000000000 ) ;
#8039=CARTESIAN_POINT ( 'NONE',  ( 54.46899307705341187, -193.5000000000000000, -70.89911581792813422 ) ) ;
#8040=CIRCLE ( 'NONE', #50819, 125.0000000000000000 ) ;
#8042=LINE ( 'NONE', #31951, #38956 ) ;
#8043=ORIENTED_EDGE ( 'NONE', *, *, #4735, .F. ) ;
#8044=AXIS2_PLACEMENT_3D ( 'NONE', #44466, #40502, #28934 ) ;
#8046=ORIENTED_EDGE ( 'NONE', *, *, #35315, .T. ) ;
#8047=CARTESIAN_POINT ( 'NONE',  ( -17.07133635870349408, -177.1207230881787780, -119.9572859573364809 ) ) ;
#8049=ORIENTED_EDGE ( 'NONE', *, *, #42031, .F. ) ;
#8050=EDGE_CURVE ( 'NONE', #29948, #19322, #18317, .T. ) ;
#8051=FACE_OUTER_BOUND ( 'NONE', #18446, .T. ) ;
#8053=LINE ( 'NONE', #23323, #5672 ) ;
#8054=CIRCLE ( 'NONE', #3858, 125.0000000000000000 ) ;
#8056=CARTESIAN_POINT ( 'NONE',  ( -37.14819544345410662, -177.1207230881787780, 123.4817304940907263 ) ) ;
#8058=LINE ( 'NONE', #36417, #31744 ) ;
#8060=VERTEX_POINT ( 'NONE', #50375 ) ;
#8065=CYLINDRICAL_SURFACE ( 'NONE', #42930, 125.0000000000000000 ) ;
#8066=DIRECTION ( 'NONE',  ( 0.000000000000000000, 1.000000000000000000, 0.000000000000000000 ) ) ;
#8068=DIRECTION ( 'NONE',  ( -0.3758275821142488260, 0.000000000000000000, 0.9266896074318291543 ) ) ;
#8069=FACE_OUTER_BOUND ( 'NONE', #26209, .T. ) ;
#8070=ORIENTED_EDGE ( 'NONE', *, *, #13172, .F. ) ;
#8071=CARTESIAN_POINT ( 'NONE',  ( -105.7090724259148118, -193.5000000000000000, 111.1293539894142839 ) ) ;
#8072=CARTESIAN_POINT ( 'NONE',  ( -91.22542124915045747, -193.5000000000000000, 117.4638425504669783 ) ) ;
#8073=FACE_BOUND ( 'NONE', #16567, .T. ) ;
#8074=ORIENTED_EDGE ( 'NONE', *, *, #44106, .T. ) ;
#8075=AXIS2_PLACEMENT_3D ( 'NONE', #46998, #7046, #2336 ) ;
#8076=AXIS2_PLACEMENT_3D ( 'NONE', #28537, #8066, #44843 ) ;
#8077=CARTESIAN_POINT ( 'NONE',  ( -165.7578939544008847, -193.5000000000000000, -43.25148278810626579 ) ) ;
#8078=VECTOR ( 'NONE', #29195, 1000.000000000000114 ) ;
#8079=AXIS2_PLACEMENT_3D ( 'NONE', #18989, #26610, #35013 ) ;
#8080=DIRECTION ( 'NONE',  ( 0.000000000000000000, 0.000000000000000000, 1.000000000000000000 ) ) ;
#8081=ORIENTED_EDGE ( 'NONE', *, *, #44416, .T. ) ;
#8082=PLANE ( 'NONE',  #32147 ) ;
#8083=EDGE_CURVE ( 'NONE', #28733, #15796, #30631, .T. ) ;
#8085=PLANE ( 'NONE',  #15922 ) ;
#8086=VECTOR ( 'NONE', #51622, 1000.000000000000000 ) ;
#8087=FACE_BOUND ( 'NONE', #16262, .T. ) ;
#8089=CARTESIAN_POINT ( 'NONE',  ( -154.5708152632604993, -177.1207230881787780, 64.19309449102807719 ) ) ;
#8090=CIRCLE ( 'NONE', #7268, 125.0000000000000000 ) ;
#8091=CIRCLE ( 'NONE', #40827, 125.0000000000000000 ) ;
#8093=AXIS2_PLACEMENT_3D ( 'NONE', #41268, #16605, #48663 ) ;
#8094=DIRECTION ( 'NONE',  ( 0.000000000000000000, -0.000000000000000000, -1.000000000000000000 ) ) ;
#8095=ORIENTED_EDGE ( 'NONE', *, *, #6396, .T. ) ;
#8096=ORIENTED_EDGE ( 'NONE', *, *, #28607, .T. ) ;
#8097=VECTOR ( 'NONE', #1393, 1000.000000000000000 ) ;
#8098=FACE_OUTER_BOUND ( 'NONE', #8374, .T. ) ;
#8099=ORIENTED_EDGE ( 'NONE', *, *, #4844, .F. ) ;
#8100=CARTESIAN_POINT ( 'NONE',  ( -49.17567778057185990, -177.1207230881787780, 0.7175072570443320474 ) ) ;
#8101=PLANE ( 'NONE',  #28868 ) ;
#8103=CARTESIAN_POINT ( 'NONE',  ( -85.48706473349324142, -189.7472609257535510, -118.3487137068146637 ) ) ;
#8106=VERTEX_POINT ( 'NONE', #34830 ) ;
#8108=ORIENTED_EDGE ( 'NONE', *, *, #26620, .F. ) ;
#8109=VECTOR ( 'NONE', #29526, 1000.000000000000000 ) ;
#8110=EDGE_CURVE ( 'NONE', #40799, #3837, #8662, .T. ) ;
#8111=DIRECTION ( 'NONE',  ( 0.6528221181905119463, 0.000000000000000000, 0.7575112421616284619 ) ) ;
#8113=DIRECTION ( 'NONE',  ( 0.000000000000000000, -1.000000000000000000, 0.000000000000000000 ) ) ;
#8116=DIRECTION ( 'NONE',  ( -0.000000000000000000, -1.000000000000000000, 0.000000000000000000 ) ) ;
#8117=ORIENTED_EDGE ( 'NONE', *, *, #28561, .T. ) ;
#8118=DIRECTION ( 'NONE',  ( -0.000000000000000000, 1.000000000000000000, -0.000000000000000000 ) ) ;
#8120=ORIENTED_EDGE ( 'NONE', *, *, #41424, .F. ) ;
#8123=DIRECTION ( 'NONE',  ( 0.9720229140804123036, 0.000000000000000000, -0.2348860457809775759 ) ) ;
#8124=VECTOR ( 'NONE', #11085, 1000.000000000000000 ) ;
#8128=CARTESIAN_POINT ( 'NONE',  ( -40.30502441601360886, -175.3837268820161057, 123.7303097900624920 ) ) ;
#8129=CARTESIAN_POINT ( 'NONE',  ( 76.04209377433251404, -175.3837268820161057, -10.93003379476866854 ) ) ;
#8132=DIRECTION ( 'NONE',  ( 0.000000000000000000, 0.000000000000000000, 1.000000000000000000 ) ) ;
#8135=VECTOR ( 'NONE', #43709, 1000.000000000000000 ) ;
#8137=FACE_OUTER_BOUND ( 'NONE', #6124, .T. ) ;
#8138=VECTOR ( 'NONE', #50215, 999.9999999999998863 ) ;
#8139=DIRECTION ( 'NONE',  ( -0.6300878435817203194, 0.000000000000000000, 0.7765238627180349740 ) ) ;
#8140=VERTEX_POINT ( 'NONE', #43243 ) ;
#8141=DIRECTION ( 'NONE',  ( 0.000000000000000000, -1.000000000000000000, 0.000000000000000000 ) ) ;
#8146=ORIENTED_EDGE ( 'NONE', *, *, #22460, .F. ) ;
#8148=CIRCLE ( 'NONE', #6515, 125.0000000000000000 ) ;
#8149=CARTESIAN_POINT ( 'NONE',  ( 27.50603775690333563, -175.3837268820161057, -99.25348746834811209 ) ) ;
#8151=LINE ( 'NONE', #24189, #9377 ) ;
#8152=DIRECTION ( 'NONE',  ( 0.5085311186492273983, 0.000000000000000000, -0.8610436117673514467 ) ) ;
#8153=DIRECTION ( 'NONE',  ( 0.000000000000000000, -1.000000000000000000, -0.000000000000000000 ) ) ;
#8154=VERTEX_POINT ( 'NONE', #3560 ) ;
#8155=ADVANCED_FACE ( 'NONE', ( #131 ), #27729, .T. ) ;
#8156=LINE ( 'NONE', #4738, #25186 ) ;
#8159=VECTOR ( 'NONE', #4546, 1000.000000000000114 ) ;
#8160=EDGE_CURVE ( 'NONE', #27933, #44506, #34572, .T. ) ;
#8161=AXIS2_PLACEMENT_3D ( 'NONE', #50269, #5867, #17938 ) ;
#8162=EDGE_LOOP ( 'NONE', ( #22713, #15772, #42847, #13116 ) ) ;
#8163=LINE ( 'NONE', #43394, #2390 ) ;
#8164=AXIS2_PLACEMENT_3D ( 'NONE', #51965, #28011, #15953 ) ;
#8165=AXIS2_PLACEMENT_3D ( 'NONE', #36332, #13214, #29237 ) ;
#8167=CIRCLE ( 'NONE', #40039, 125.0000000000000000 ) ;
#8168=DIRECTION ( 'NONE',  ( 0.000000000000000000, -0.000000000000000000, -1.000000000000000000 ) ) ;
#8170=CARTESIAN_POINT ( 'NONE',  ( -136.1415351158078408, -175.3837268820161057, -89.10837311819175000 ) ) ;
#8172=ORIENTED_EDGE ( 'NONE', *, *, #23994, .F. ) ;
#8173=EDGE_CURVE ( 'NONE', #2222, #32491, #3521, .T. ) ;
#8175=ORIENTED_EDGE ( 'NONE', *, *, #27236, .F. ) ;
#8176=DIRECTION ( 'NONE',  ( -0.000000000000000000, 1.000000000000000000, -0.000000000000000000 ) ) ;
#8180=CARTESIAN_POINT ( 'NONE',  ( 73.87536152799695799, -193.5000000000000000, -25.58083653558413317 ) ) ;
#8181=CARTESIAN_POINT ( 'NONE',  ( 1.755575411425465360, -175.3837268820161057, 114.4616734920527392 ) ) ;
#8184=DIRECTION ( 'NONE',  ( -0.000000000000000000, 1.000000000000000000, -0.000000000000000000 ) ) ;
#8185=AXIS2_PLACEMENT_3D ( 'NONE', #38739, #18785, #51132 ) ;
#8187=AXIS2_PLACEMENT_3D ( 'NONE', #40950, #28070, #4972 ) ;
#8190=CARTESIAN_POINT ( 'NONE',  ( -91.84482189527193441, -193.5000000000000000, -117.2365833888816695 ) ) ;
#8193=CARTESIAN_POINT ( 'NONE',  ( 57.31108707223381060, -189.7472609257535510, -66.58401203837752291 ) ) ;
#8194=EDGE_LOOP ( 'NONE', ( #11014, #12159, #4864, #50373 ) ) ;
#8198=DIRECTION ( 'NONE',  ( -0.8124868780056863082, 0.000000000000000000, 0.5829794791144649047 ) ) ;
#8200=VECTOR ( 'NONE', #46123, 1000.000000000000000 ) ;
#8201=CARTESIAN_POINT ( 'NONE',  ( -145.6517069852672535, -193.5000000000000000, 78.62880929222943394 ) ) ;
#8202=CYLINDRICAL_SURFACE ( 'NONE', #13529, 124.9999999999999858 ) ;
#8203=VECTOR ( 'NONE', #1402, 1000.000000000000114 ) ;
#8205=ADVANCED_FACE ( 'NONE', ( #36133 ), #35613, .T. ) ;
#8206=CARTESIAN_POINT ( 'NONE',  ( -49.40581635894068313, -193.5000000000000000, -0.3758275821142418316 ) ) ;
#8207=FACE_OUTER_BOUND ( 'NONE', #9170, .T. ) ;
#8208=EDGE_CURVE ( 'NONE', #20769, #11778, #20109, .T. ) ;
#8209=CARTESIAN_POINT ( 'NONE',  ( -58.17235712592530916, -177.1207230881787780, 123.6213615703899649 ) ) ;
#8212=CARTESIAN_POINT ( 'NONE',  ( -48.47912675150885065, -193.5000000000000000, 6.938893903907228378E-15 ) ) ;
#8213=EDGE_LOOP ( 'NONE', ( #12974, #17160, #67, #17538 ) ) ;
#8217=EDGE_CURVE ( 'NONE', #15211, #12738, #35405, .T. ) ;
#8218=LINE ( 'NONE', #36589, #3617 ) ;
#8220=CIRCLE ( 'NONE', #51051, 125.0000000000000000 ) ;
#8224=CARTESIAN_POINT ( 'NONE',  ( -141.2664123866436512, -193.5000000000000000, -83.75869879877495805 ) ) ;
#8225=AXIS2_PLACEMENT_3D ( 'NONE', #49492, #21084, #9011 ) ;
#8226=CARTESIAN_POINT ( 'NONE',  ( -12.13476221271688260, -189.7472609257535510, 119.5996955107804780 ) ) ;
#8228=ORIENTED_EDGE ( 'NONE', *, *, #4343, .F. ) ;
#8229=ORIENTED_EDGE ( 'NONE', *, *, #32211, .F. ) ;
#8230=EDGE_LOOP ( 'NONE', ( #19883, #10481, #10224, #23120 ) ) ;
#8231=DIRECTION ( 'NONE',  ( -0.000000000000000000, 1.000000000000000000, -0.000000000000000000 ) ) ;
#8232=LINE ( 'NONE', #31108, #17677 ) ;
#8235=CARTESIAN_POINT ( 'NONE',  ( -123.5870580700902366, -175.3837268820161057, -98.66508442481458019 ) ) ;
#8238=DIRECTION ( 'NONE',  ( 0.000000000000000000, -1.000000000000000000, 0.000000000000000000 ) ) ;
#8240=CARTESIAN_POINT ( 'NONE',  ( -48.47912675150885065, -183.6283474603465606, 6.938893903907228378E-15 ) ) ;
#8241=ORIENTED_EDGE ( 'NONE', *, *, #31605, .T. ) ;
#8242=ORIENTED_EDGE ( 'NONE', *, *, #33940, .F. ) ;
#8244=DIRECTION ( 'NONE',  ( 0.000000000000000000, 1.000000000000000000, -0.000000000000000000 ) ) ;
#8246=VERTEX_POINT ( 'NONE', #7766 ) ;
#8248=LINE ( 'NONE', #877, #50575 ) ;
#8249=EDGE_LOOP ( 'NONE', ( #3458, #50058, #49167, #30850 ) ) ;
#8251=EDGE_LOOP ( 'NONE', ( #24730, #42056, #19032, #9996 ) ) ;
#8252=CARTESIAN_POINT ( 'NONE',  ( -161.4184887245413904, -193.5000000000000000, 51.19472891551360050 ) ) ;
#8254=CARTESIAN_POINT ( 'NONE',  ( 59.00260725618640123, -193.5000000000000000, -63.81752780152988436 ) ) ;
#8255=FACE_BOUND ( 'NONE', #39558, .T. ) ;
#8258=VECTOR ( 'NONE', #48312, 999.9999999999998863 ) ;
#8259=CARTESIAN_POINT ( 'NONE',  ( 75.47134233844786877, -175.3837268820161057, -3.504489105734901244 ) ) ;
#8260=VERTEX_POINT ( 'NONE', #17150 ) ;
#8261=AXIS2_PLACEMENT_3D ( 'NONE', #11586, #20243, #35484 ) ;
#8266=FACE_OUTER_BOUND ( 'NONE', #35311, .T. ) ;
#8267=ADVANCED_FACE ( 'NONE', ( #43515 ), #33162, .T. ) ;
#8268=DIRECTION ( 'NONE',  ( 0.08879589532293853671, 0.000000000000000000, -0.9960498426152166740 ) ) ;
#8270=ORIENTED_EDGE ( 'NONE', *, *, #9616, .T. ) ;
#8271=LINE ( 'NONE', #39787, #34521 ) ;
#8272=VERTEX_POINT ( 'NONE', #24062 ) ;
#8275=EDGE_CURVE ( 'NONE', #41080, #47094, #47458, .T. ) ;
#8277=DIRECTION ( 'NONE',  ( 0.000000000000000000, 0.000000000000000000, -1.000000000000000000 ) ) ;
#8278=VERTEX_POINT ( 'NONE', #41302 ) ;
#8279=ADVANCED_FACE ( 'NONE', ( #15407 ), #35356, .T. ) ;
#8281=CARTESIAN_POINT ( 'NONE',  ( -172.6359455740846158, -183.6283474603465606, -14.49428645563797069 ) ) ;
#8285=EDGE_CURVE ( 'NONE', #40286, #2431, #21162, .T. ) ;
#8287=ORIENTED_EDGE ( 'NONE', *, *, #48841, .T. ) ;
#8288=EDGE_CURVE ( 'NONE', #33417, #9630, #25540, .T. ) ;
#8289=CARTESIAN_POINT ( 'NONE',  ( -48.18706998087187543, -177.1207230881787780, -0.9564009842765152092 ) ) ;
#8290=DIRECTION ( 'NONE',  ( -0.000000000000000000, 1.000000000000000000, 0.000000000000000000 ) ) ;
#8291=EDGE_LOOP ( 'NONE', ( #34473, #50256, #32578, #44678 ) ) ;
#8292=DIRECTION ( 'NONE',  ( 0.000000000000000000, -1.000000000000000000, 0.000000000000000000 ) ) ;
#8293=DIRECTION ( 'NONE',  ( 0.5586467658036415873, 0.000000000000000000, 0.8294056854502090959 ) ) ;
#8294=EDGE_CURVE ( 'NONE', #28453, #26725, #29735, .T. ) ;
#8295=LINE ( 'NONE', #12220, #46241 ) ;
#8296=CYLINDRICAL_SURFACE ( 'NONE', #25734, 125.0000000000000000 ) ;
#8297=ORIENTED_EDGE ( 'NONE', *, *, #45031, .T. ) ;
#8298=ORIENTED_EDGE ( 'NONE', *, *, #47801, .F. ) ;
#8299=ORIENTED_EDGE ( 'NONE', *, *, #48263, .F. ) ;
#8300=CARTESIAN_POINT ( 'NONE',  ( -161.8276685539205744, -183.6283474603465606, 50.28156562190587664 ) ) ;
#8301=ORIENTED_EDGE ( 'NONE', *, *, #24208, .F. ) ;
#8302=CARTESIAN_POINT ( 'NONE',  ( 52.16997862029128186, -189.7472609257535510, 72.42760398749086903 ) ) ;
#8303=AXIS2_PLACEMENT_3D ( 'NONE', #14161, #10196, #21779 ) ;
#8305=DIRECTION ( 'NONE',  ( -0.000000000000000000, 1.000000000000000000, -0.000000000000000000 ) ) ;
#8307=DIRECTION ( 'NONE',  ( 0.000000000000000000, 0.000000000000000000, 1.000000000000000000 ) ) ;
#8308=EDGE_LOOP ( 'NONE', ( #49001, #38988, #46261, #6941 ) ) ;
#8310=EDGE_CURVE ( 'NONE', #35696, #28453, #2135, .T. ) ;
#8312=PLANE ( 'NONE',  #29840 ) ;
#8313=EDGE_LOOP ( 'NONE', ( #25244, #17307, #3130, #45504 ) ) ;
#8314=VECTOR ( 'NONE', #40640, 1000.000000000000000 ) ;
#8316=CARTESIAN_POINT ( 'NONE',  ( -151.4272465800706016, -183.6283474603465606, 70.89911581792887318 ) ) ;
#8317=CARTESIAN_POINT ( 'NONE',  ( 73.09196206113300320, -177.1207230881787780, 29.07697310430963356 ) ) ;
#8318=DIRECTION ( 'NONE',  ( 0.000000000000000000, -1.000000000000000000, -0.000000000000000000 ) ) ;
#8323=CIRCLE ( 'NONE', #36869, 125.0000000000000000 ) ;
#8324=ADVANCED_FACE ( 'NONE', ( #17680 ), #25808, .T. ) ;
#8325=ORIENTED_EDGE ( 'NONE', *, *, #43908, .T. ) ;
#8326=CARTESIAN_POINT ( 'NONE',  ( -158.3442440847887269, -193.5000000000000000, -59.62093586438114556 ) ) ;
#8327=DIRECTION ( 'NONE',  ( 0.1182731709213730997, 0.000000000000000000, -0.9929810960135161402 ) ) ;
#8330=ADVANCED_FACE ( 'NONE', ( #13465 ), #38133, .F. ) ;
#8331=EDGE_CURVE ( 'NONE', #16064, #9382, #1368, .T. ) ;
#8333=DIRECTION ( 'NONE',  ( 0.000000000000000000, 1.000000000000000000, -0.000000000000000000 ) ) ;
#8334=EDGE_CURVE ( 'NONE', #27228, #29227, #37093, .T. ) ;
#8336=DIRECTION ( 'NONE',  ( -0.000000000000000000, 1.000000000000000000, -0.000000000000000000 ) ) ;
#8337=CARTESIAN_POINT ( 'NONE',  ( -82.43766229206461560, -183.6283474603465606, -119.2602935412679983 ) ) ;
#8339=DIRECTION ( 'NONE',  ( 0.000000000000000000, 0.000000000000000000, -1.000000000000000000 ) ) ;
#8340=FACE_BOUND ( 'NONE', #41562, .T. ) ;
#8341=ORIENTED_EDGE ( 'NONE', *, *, #13203, .T. ) ;
#8344=CIRCLE ( 'NONE', #12538, 125.0000000000000000 ) ;
#8345=DIRECTION ( 'NONE',  ( -0.6068001458185834363, 0.000000000000000000, -0.7948544414133608127 ) ) ;
#8347=CARTESIAN_POINT ( 'NONE',  ( 68.59638248015004081, -193.5000000000000000, -43.79868877201405297 ) ) ;
#8348=EDGE_CURVE ( 'NONE', #29932, #38087, #37637, .T. ) ;
#8351=EDGE_CURVE ( 'NONE', #8740, #9394, #13981, .T. ) ;
#8353=LINE ( 'NONE', #32781, #43881 ) ;
#8355=CARTESIAN_POINT ( 'NONE',  ( -56.65322908700500193, -175.3837268820161057, -123.7303097900624351 ) ) ;
#8356=ORIENTED_EDGE ( 'NONE', *, *, #19828, .T. ) ;
#8358=VECTOR ( 'NONE', #29304, 1000.000000000000114 ) ;
#8359=VERTEX_POINT ( 'NONE', #33446 ) ;
#8360=PLANE ( 'NONE',  #17525 ) ;
#8362=PLANE ( 'NONE',  #35157 ) ;
#8363=DIRECTION ( 'NONE',  ( 0.9646355819083556327, 0.000000000000000000, 0.2635871660690782825 ) ) ;
#8364=FACE_OUTER_BOUND ( 'NONE', #7199, .T. ) ;
#8367=CARTESIAN_POINT ( 'NONE',  ( -74.51199343215203896, -193.5000000000000000, -122.2591094863194598 ) ) ;
#8369=FACE_OUTER_BOUND ( 'NONE', #1971, .T. ) ;
#8370=CARTESIAN_POINT ( 'NONE',  ( 5.542374969221969039, -177.1207230881787780, 112.7238987608088365 ) ) ;
#8371=ORIENTED_EDGE ( 'NONE', *, *, #7214, .T. ) ;
#8373=LINE ( 'NONE', #13089, #13078 ) ;
#8374=EDGE_LOOP ( 'NONE', ( #20452, #20229, #20508, #30138 ) ) ;
#8375=DIRECTION ( 'NONE',  ( 0.000000000000000000, 0.000000000000000000, -1.000000000000000000 ) ) ;
#8378=DIRECTION ( 'NONE',  ( 0.000000000000000000, 1.000000000000000000, 0.000000000000000000 ) ) ;
#8379=ORIENTED_EDGE ( 'NONE', *, *, #14673, .F. ) ;
#8382=ORIENTED_EDGE ( 'NONE', *, *, #48522, .F. ) ;
#8385=LINE ( 'NONE', #48863, #29785 ) ;
#8386=DIRECTION ( 'NONE',  ( -0.5085311186492154079, 0.000000000000000000, -0.8610436117673585521 ) ) ;
#8387=CARTESIAN_POINT ( 'NONE',  ( -157.4685091425930921, -193.5000000000000000, -59.13814366165038905 ) ) ;
#8388=DIRECTION ( 'NONE',  ( -0.000000000000000000, 1.000000000000000000, 0.000000000000000000 ) ) ;
#8389=DIRECTION ( 'NONE',  ( 0.000000000000000000, -0.000000000000000000, 1.000000000000000000 ) ) ;
#8390=EDGE_LOOP ( 'NONE', ( #30265, #3329, #30716, #50538 ) ) ;
#8391=EDGE_CURVE ( 'NONE', #20806, #26640, #37928, .T. ) ;
#8397=VECTOR ( 'NONE', #2467, 1000.000000000000000 ) ;
#8398=DIRECTION ( 'NONE',  ( -0.5085311186492094127, 0.000000000000000000, -0.8610436117673619938 ) ) ;
#8399=ORIENTED_EDGE ( 'NONE', *, *, #26340, .F. ) ;
#8400=CARTESIAN_POINT ( 'NONE',  ( 35.67816836544800907, -193.5000000000000000, -92.42591454022745268 ) ) ;
#8401=CARTESIAN_POINT ( 'NONE',  ( -140.1460956102404509, -189.7472609257535510, 84.98333260264821831 ) ) ;
#8404=ORIENTED_EDGE ( 'NONE', *, *, #5508, .T. ) ;
#8405=ORIENTED_EDGE ( 'NONE', *, *, #48204, .T. ) ;
#8406=FACE_OUTER_BOUND ( 'NONE', #47307, .T. ) ;
#8408=CARTESIAN_POINT ( 'NONE',  ( -119.6907301311197216, -193.5000000000000000, 101.5140743725400370 ) ) ;
#8411=CARTESIAN_POINT ( 'NONE',  ( -19.51863976943889512, -193.5000000000000000, 120.5706864261537419 ) ) ;
#8413=DIRECTION ( 'NONE',  ( 0.000000000000000000, -1.000000000000000000, 0.000000000000000000 ) ) ;
#8415=EDGE_CURVE ( 'NONE', #19199, #25045, #4986, .T. ) ;
#8417=ORIENTED_EDGE ( 'NONE', *, *, #40235, .T. ) ;
#8418=CARTESIAN_POINT ( 'NONE',  ( -114.1105527140175155, -193.5000000000000000, 106.3838142112217611 ) ) ;
#8420=AXIS2_PLACEMENT_3D ( 'NONE', #17412, #25274, #21331 ) ;
#8421=CARTESIAN_POINT ( 'NONE',  ( 75.27070168362158142, -175.3837268820161057, 17.63462396184792169 ) ) ;
#8422=CARTESIAN_POINT ( 'NONE',  ( -143.3583119192899460, -183.6283474603465606, -81.38144888055207105 ) ) ;
#8426=CARTESIAN_POINT ( 'NONE',  ( -143.3583119192899744, -193.5000000000000000, -81.38144888055202841 ) ) ;
#8427=VERTEX_POINT ( 'NONE', #41217 ) ;
#8428=DIRECTION ( 'NONE',  ( 0.000000000000000000, -0.000000000000000000, 1.000000000000000000 ) ) ;
#8429=DIRECTION ( 'NONE',  ( 0.6068001458185890984, 0.000000000000000000, 0.7948544414133565938 ) ) ;
#8430=EDGE_LOOP ( 'NONE', ( #23671, #13574, #38798, #38663 ) ) ;
#8431=DIRECTION ( 'NONE',  ( 0.000000000000000000, 0.000000000000000000, -1.000000000000000000 ) ) ;
#8432=DIRECTION ( 'NONE',  ( 0.000000000000000000, -0.000000000000000000, -1.000000000000000000 ) ) ;
#8434=DIRECTION ( 'NONE',  ( 0.000000000000000000, 0.000000000000000000, -1.000000000000000000 ) ) ;
#8435=EDGE_LOOP ( 'NONE', ( #24960, #49116, #51788, #41986 ) ) ;
#8437=DIRECTION ( 'NONE',  ( -0.000000000000000000, 0.000000000000000000, 1.000000000000000000 ) ) ;
#8438=DIRECTION ( 'NONE',  ( 1.000000000000000000, 0.000000000000000000, 0.000000000000000000 ) ) ;
#8445=ADVANCED_FACE ( 'NONE', ( #16814 ), #45197, .F. ) ;
#8446=DIRECTION ( 'NONE',  ( 0.000000000000000000, 0.000000000000000000, -1.000000000000000000 ) ) ;
#8447=LINE ( 'NONE', #3466, #49989 ) ;
#8448=ORIENTED_EDGE ( 'NONE', *, *, #16890, .T. ) ;
#8450=ORIENTED_EDGE ( 'NONE', *, *, #38060, .F. ) ;
#8452=LINE ( 'NONE', #48413, #6814 ) ;
#8453=AXIS2_PLACEMENT_3D ( 'NONE', #30553, #13505, #46604 ) ;
#8455=FACE_OUTER_BOUND ( 'NONE', #1291, .T. ) ;
#8457=VECTOR ( 'NONE', #21602, 1000.000000000000114 ) ;
#8458=DIRECTION ( 'NONE',  ( 0.000000000000000000, -1.000000000000000000, 0.000000000000000000 ) ) ;
#8459=LINE ( 'NONE', #24489, #42110 ) ;
#8460=EDGE_CURVE ( 'NONE', #31552, #7207, #32887, .T. ) ;
#8461=CARTESIAN_POINT ( 'NONE',  ( -149.7090673587772756, -193.5000000000000000, -71.61357856150526402 ) ) ;
#8463=ORIENTED_EDGE ( 'NONE', *, *, #12016, .F. ) ;
#8465=CARTESIAN_POINT ( 'NONE',  ( -131.9398708394020332, -183.6283474603465606, 91.70840728318374602 ) ) ;
#8466=CARTESIAN_POINT ( 'NONE',  ( -48.47912675150885065, -175.3837268820161057, 6.938893903907228378E-15 ) ) ;
#8468=EDGE_LOOP ( 'NONE', ( #45154, #28487, #18067, #35387 ) ) ;
#8471=DIRECTION ( 'NONE',  ( 0.6749830015182142207, 0.000000000000000000, -0.7378332790417239107 ) ) ;
#8472=DIRECTION ( 'NONE',  ( 0.000000000000000000, -1.000000000000000000, 0.000000000000000000 ) ) ;
#8478=CARTESIAN_POINT ( 'NONE',  ( -112.7586829773731267, -175.3837268820161057, -107.2060569716373521 ) ) ;
#8479=DIRECTION ( 'NONE',  ( -0.8757349421956345248, 0.000000000000000000, -0.4827922027307490205 ) ) ;
#8480=ORIENTED_EDGE ( 'NONE', *, *, #799, .F. ) ;
#8483=ORIENTED_EDGE ( 'NONE', *, *, #47021, .T. ) ;
#8484=CARTESIAN_POINT ( 'NONE',  ( -108.5723883981724640, -183.6283474603465606, 109.6074810615846076 ) ) ;
#8485=AXIS2_PLACEMENT_3D ( 'NONE', #2961, #27903, #19268 ) ;
#8486=ADVANCED_FACE ( 'NONE', ( #8906 ), #16553, .F. ) ;
#8488=DIRECTION ( 'NONE',  ( 0.000000000000000000, -0.000000000000000000, -1.000000000000000000 ) ) ;
#8489=DIRECTION ( 'NONE',  ( -0.000000000000000000, 1.000000000000000000, -0.000000000000000000 ) ) ;
#8490=AXIS2_PLACEMENT_3D ( 'NONE', #51721, #31737, #47777 ) ;
#8491=ADVANCED_FACE ( 'NONE', ( #41477 ), #33079, .T. ) ;
#8492=ORIENTED_EDGE ( 'NONE', *, *, #11730, .F. ) ;
#8494=FACE_OUTER_BOUND ( 'NONE', #33566, .T. ) ;
#8495=DIRECTION ( 'NONE',  ( 0.000000000000000000, 0.000000000000000000, -1.000000000000000000 ) ) ;
#8496=VECTOR ( 'NONE', #47961, 1000.000000000000114 ) ;
#8497=ORIENTED_EDGE ( 'NONE', *, *, #40903, .F. ) ;
#8498=CARTESIAN_POINT ( 'NONE',  ( -49.44376233341721161, -183.6283474603465606, 0.2635871660690650709 ) ) ;
#8499=LINE ( 'NONE', #44260, #18688 ) ;
#8501=ADVANCED_FACE ( 'NONE', ( #32819 ), #48871, .T. ) ;
#8502=DIRECTION ( 'NONE',  ( -0.7175072570443299380, 0.000000000000000000, -0.6965510290629983725 ) ) ;
#8503=EDGE_CURVE ( 'NONE', #23398, #6329, #4451, .T. ) ;
#8504=DIRECTION ( 'NONE',  ( -0.3482016354343995812, 0.000000000000000000, 0.9374196611341205632 ) ) ;
#8507=ORIENTED_EDGE ( 'NONE', *, *, #2663, .F. ) ;
#8509=VECTOR ( 'NONE', #13213, 1000.000000000000114 ) ;
#8512=DIRECTION ( 'NONE',  ( -0.3202698538628350744, 0.000000000000000000, -0.9473263538541923934 ) ) ;
#8513=CARTESIAN_POINT ( 'NONE',  ( -26.53529504715431031, -193.5000000000000000, 123.0587999703026725 ) ) ;
#8515=CARTESIAN_POINT ( 'NONE',  ( -49.47517659412407198, -175.3837268820161057, 0.08879589532293177823 ) ) ;
#8517=LINE ( 'NONE', #40836, #6073 ) ;
#8518=ORIENTED_EDGE ( 'NONE', *, *, #17626, .T. ) ;
#8521=CARTESIAN_POINT ( 'NONE',  ( -135.4258661347518853, -193.5000000000000000, -89.80681772907007598 ) ) ;
#8522=DIRECTION ( 'NONE',  ( 0.000000000000000000, 1.000000000000000000, -0.000000000000000000 ) ) ;
#8523=VERTEX_POINT ( 'NONE', #37285 ) ;
#8524=AXIS2_PLACEMENT_3D ( 'NONE', #30614, #22750, #49842 ) ;
#8525=EDGE_LOOP ( 'NONE', ( #40994, #10149, #26892, #49175 ) ) ;
#8526=DIRECTION ( 'NONE',  ( -0.9151456172430181280, 0.000000000000000000, -0.4031234292879730674 ) ) ;
#8527=VECTOR ( 'NONE', #14875, 1000.000000000000000 ) ;
#8528=AXIS2_PLACEMENT_3D ( 'NONE', #40248, #20287, #36315 ) ;
#8529=CARTESIAN_POINT ( 'NONE',  ( 23.33927677392130917, -193.5000000000000000, -102.3089288139528747 ) ) ;
#8530=CARTESIAN_POINT ( 'NONE',  ( -48.02249751411513756, -189.7472609257535510, -0.8896570909947397743 ) ) ;
#8531=ORIENTED_EDGE ( 'NONE', *, *, #23912, .F. ) ;
#8532=DIRECTION ( 'NONE',  ( -0.000000000000000000, -1.000000000000000000, 0.000000000000000000 ) ) ;
#8533=ORIENTED_EDGE ( 'NONE', *, *, #14962, .T. ) ;
#8534=CARTESIAN_POINT ( 'NONE',  ( 4.109287492203100634, -183.6283474603465606, -113.3995532942336979 ) ) ;
#8535=CARTESIAN_POINT ( 'NONE',  ( -49.03777351731249468, -193.5000000000000000, -0.8294056854502022125 ) ) ;
#8537=CARTESIAN_POINT ( 'NONE',  ( 39.56636334395317789, -183.6283474603465606, -87.31661597576083977 ) ) ;
#8538=ORIENTED_EDGE ( 'NONE', *, *, #28433, .F. ) ;
#8539=AXIS2_PLACEMENT_3D ( 'NONE', #8212, #36849, #4268 ) ;
#8540=VERTEX_POINT ( 'NONE', #24420 ) ;
#8541=EDGE_LOOP ( 'NONE', ( #43932, #25950, #38914, #7840 ) ) ;
#8543=PLANE ( 'NONE',  #12589 ) ;
#8545=CIRCLE ( 'NONE', #973, 125.0000000000000000 ) ;
#8546=DIRECTION ( 'NONE',  ( 0.000000000000000000, 0.000000000000000000, -1.000000000000000000 ) ) ;
#8548=DIRECTION ( 'NONE',  ( 0.000000000000000000, 1.000000000000000000, 0.000000000000000000 ) ) ;
#8549=ORIENTED_EDGE ( 'NONE', *, *, #31719, .F. ) ;
#8550=ADVANCED_FACE ( 'NONE', ( #33352 ), #4712, .T. ) ;
#8553=DIRECTION ( 'NONE',  ( 0.000000000000000000, 1.000000000000000000, 0.000000000000000000 ) ) ;
#8557=CARTESIAN_POINT ( 'NONE',  ( -155.4465502054561057, -183.6283474603465606, 64.67588669375881238 ) ) ;
#8558=AXIS2_PLACEMENT_3D ( 'NONE', #13428, #42053, #21842 ) ;
#8563=DIRECTION ( 'NONE',  ( 0.000000000000000000, 0.000000000000000000, -1.000000000000000000 ) ) ;
#8564=VECTOR ( 'NONE', #1413, 1000.000000000000000 ) ;
#8565=VERTEX_POINT ( 'NONE', #1547 ) ;
#8566=EDGE_CURVE ( 'NONE', #45141, #22586, #50172, .T. ) ;
#8569=FACE_OUTER_BOUND ( 'NONE', #18680, .T. ) ;
#8572=CARTESIAN_POINT ( 'NONE',  ( -48.71401279728984690, -177.1207230881787780, 0.9720229140804159673 ) ) ;
#8574=EDGE_CURVE ( 'NONE', #2935, #23376, #10200, .T. ) ;
#8575=CYLINDRICAL_SURFACE ( 'NONE', #46505, 125.0000000000000000 ) ;
#8579=CARTESIAN_POINT ( 'NONE',  ( -47.87232660569025455, -175.3837268820161057, -0.7948544414133454916 ) ) ;
#8580=CIRCLE ( 'NONE', #27892, 125.0000000000000000 ) ;
#8583=FACE_BOUND ( 'NONE', #10195, .T. ) ;
#8585=AXIS2_PLACEMENT_3D ( 'NONE', #5588, #34212, #1643 ) ;
#8586=AXIS2_PLACEMENT_3D ( 'NONE', #24847, #15939, #31950 ) ;
#8590=CARTESIAN_POINT ( 'NONE',  ( -47.66663987350317910, -189.7472609257535510, 0.5829794791144832233 ) ) ;
#8593=LINE ( 'NONE', #8854, #4176 ) ;
#8595=DIRECTION ( 'NONE',  ( 0.8294056854501971054, 0.000000000000000000, 0.5586467658036594619 ) ) ;
#8597=VECTOR ( 'NONE', #14722, 1000.000000000000227 ) ;
#8598=DIRECTION ( 'NONE',  ( -0.000000000000000000, 1.000000000000000000, -0.000000000000000000 ) ) ;
#8599=ORIENTED_EDGE ( 'NONE', *, *, #4550, .T. ) ;
#8600=AXIS2_PLACEMENT_3D ( 'NONE', #18872, #30698, #12479 ) ;
#8601=ORIENTED_EDGE ( 'NONE', *, *, #20326, .T. ) ;
#8603=CARTESIAN_POINT ( 'NONE',  ( 26.89923761108473954, -175.3837268820161057, -98.45863302693476271 ) ) ;
#8604=ORIENTED_EDGE ( 'NONE', *, *, #15065, .T. ) ;
#8605=CARTESIAN_POINT ( 'NONE',  ( -26.53529504715431031, -189.7472609257535510, 123.0587999703026725 ) ) ;
#8610=EDGE_CURVE ( 'NONE', #19842, #28928, #50672, .T. ) ;
#8611=EDGE_CURVE ( 'NONE', #16275, #32338, #6538, .T. ) ;
#8612=CIRCLE ( 'NONE', #21233, 125.0000000000000000 ) ;
#8613=EDGE_CURVE ( 'NONE', #49730, #41086, #34382, .T. ) ;
#8614=CYLINDRICAL_SURFACE ( 'NONE', #30957, 125.0000000000000000 ) ;
#8615=CARTESIAN_POINT ( 'NONE',  ( -169.7849785064912282, -175.3837268820161057, -25.70779184431770048 ) ) ;
#8619=ORIENTED_EDGE ( 'NONE', *, *, #7891, .F. ) ;
#8620=AXIS2_PLACEMENT_3D ( 'NONE', #6208, #17775, #41416 ) ;
#8621=AXIS2_PLACEMENT_3D ( 'NONE', #39165, #22885, #10799 ) ;
#8625=VERTEX_POINT ( 'NONE', #26480 ) ;
#8626=DIRECTION ( 'NONE',  ( 0.000000000000000000, -0.000000000000000000, -1.000000000000000000 ) ) ;
#8628=CARTESIAN_POINT ( 'NONE',  ( -79.88691714431334390, -183.6283474603465606, 119.9572859573367367 ) ) ;
#8629=VECTOR ( 'NONE', #1290, 1000.000000000000227 ) ;
#8630=DIRECTION ( 'NONE',  ( 0.000000000000000000, 0.000000000000000000, 1.000000000000000000 ) ) ;
#8631=ORIENTED_EDGE ( 'NONE', *, *, #8110, .T. ) ;
#8634=CARTESIAN_POINT ( 'NONE',  ( 17.44316424268006926, -183.6283474603465606, -105.0256126866231625 ) ) ;
#8635=EDGE_LOOP ( 'NONE', ( #32225, #9024, #42874, #37415 ) ) ;
#8636=EDGE_CURVE ( 'NONE', #10170, #27297, #42251, .T. ) ;
#8638=DIRECTION ( 'NONE',  ( 0.000000000000000000, 0.000000000000000000, -1.000000000000000000 ) ) ;
#8639=FACE_OUTER_BOUND ( 'NONE', #19296, .T. ) ;
#8641=DIRECTION ( 'NONE',  ( -0.000000000000000000, 1.000000000000000000, 0.000000000000000000 ) ) ;
#8644=CIRCLE ( 'NONE', #1935, 125.0000000000000000 ) ;
#8645=CARTESIAN_POINT ( 'NONE',  ( 39.56636334395317789, -177.1207230881787780, -87.31661597576083977 ) ) ;
#8646=EDGE_CURVE ( 'NONE', #10667, #42459, #50423, .T. ) ;
#8648=DIRECTION ( 'NONE',  ( -0.000000000000000000, 1.000000000000000000, -0.000000000000000000 ) ) ;
#8649=CARTESIAN_POINT ( 'NONE',  ( -173.0003472773501301, -175.3837268820161057, 10.93003379476953363 ) ) ;
#8650=EDGE_CURVE ( 'NONE', #7741, #32981, #9690, .T. ) ;
#8652=CARTESIAN_POINT ( 'NONE',  ( -48.41988612361514299, -183.6283474603465606, -0.9982437317643144681 ) ) ;
#8657=FACE_OUTER_BOUND ( 'NONE', #40917, .T. ) ;
#8659=EDGE_LOOP ( 'NONE', ( #17682, #40453, #44384, #6809 ) ) ;
#8661=ORIENTED_EDGE ( 'NONE', *, *, #35871, .T. ) ;
#8662=CIRCLE ( 'NONE', #19575, 125.0000000000000000 ) ;
#8663=EDGE_CURVE ( 'NONE', #10734, #1781, #18856, .T. ) ;
#8664=EDGE_CURVE ( 'NONE', #49035, #3976, #43802, .T. ) ;
#8667=DIRECTION ( 'NONE',  ( -0.9151456172430181280, 0.000000000000000000, -0.4031234292879730674 ) ) ;
#8671=CARTESIAN_POINT ( 'NONE',  ( 26.89923761108473599, -193.5000000000000000, -98.45863302693476271 ) ) ;
#8672=ORIENTED_EDGE ( 'NONE', *, *, #48690, .T. ) ;
#8673=LINE ( 'NONE', #792, #2985 ) ;
#8676=CARTESIAN_POINT ( 'NONE',  ( 66.73972540229263473, -193.5000000000000000, 45.83253885719642540 ) ) ;
#8677=VECTOR ( 'NONE', #36774, 1000.000000000000000 ) ;
#8679=EDGE_CURVE ( 'NONE', #33832, #44506, #51708, .T. ) ;
#8682=EDGE_CURVE ( 'NONE', #23051, #43457, #15352, .T. ) ;
#8683=DIRECTION ( 'NONE',  ( 0.000000000000000000, 0.000000000000000000, 1.000000000000000000 ) ) ;
#8686=CARTESIAN_POINT ( 'NONE',  ( -48.47912675150885065, -175.3837268820161057, 6.938893903907228378E-15 ) ) ;
#8687=EDGE_LOOP ( 'NONE', ( #21149, #11882, #22361, #41646 ) ) ;
#8689=ORIENTED_EDGE ( 'NONE', *, *, #51713, .F. ) ;
#8690=DIRECTION ( 'NONE',  ( -0.9027978299657477557, 0.000000000000000000, 0.4300652022765115712 ) ) ;
#8691=CARTESIAN_POINT ( 'NONE',  ( -166.9790462269951661, -193.5000000000000000, 36.52255268223138529 ) ) ;
#8692=VERTEX_POINT ( 'NONE', #23835 ) ;
#8693=FACE_OUTER_BOUND ( 'NONE', #35553, .T. ) ;
#8695=DIRECTION ( 'NONE',  ( 0.000000000000000000, 0.000000000000000000, 1.000000000000000000 ) ) ;
#8696=DIRECTION ( 'NONE',  ( 0.000000000000000000, -0.000000000000000000, 1.000000000000000000 ) ) ;
#8697=CIRCLE ( 'NONE', #39728, 125.0000000000000000 ) ;
#8698=ORIENTED_EDGE ( 'NONE', *, *, #33560, .T. ) ;
#8699=DIRECTION ( 'NONE',  ( -0.2059786187410953262, 0.000000000000000000, -0.9785564922995046988 ) ) ;
#8700=VECTOR ( 'NONE', #29317, 1000.000000000000000 ) ;
#8701=CARTESIAN_POINT ( 'NONE',  ( -170.2790847791494855, -193.5000000000000000, -28.10285082451569494 ) ) ;
#8706=DIRECTION ( 'NONE',  ( 0.7765238627180393038, 0.000000000000000000, 0.6300878435817147682 ) ) ;
#8707=ORIENTED_EDGE ( 'NONE', *, *, #46418, .T. ) ;
#8708=DIRECTION ( 'NONE',  ( -0.4639789333096864810, 0.000000000000000000, 0.8858462335218260097 ) ) ;
#8710=ORIENTED_EDGE ( 'NONE', *, *, #3625, .F. ) ;
#8712=VERTEX_POINT ( 'NONE', #30949 ) ;
#8714=VECTOR ( 'NONE', #8336, 1000.000000000000000 ) ;
#8715=DIRECTION ( 'NONE',  ( -0.3758275821142357809, 0.000000000000000000, -0.9266896074318343723 ) ) ;
#8718=AXIS2_PLACEMENT_3D ( 'NONE', #7300, #51707, #24356 ) ;
#8722=LINE ( 'NONE', #47903, #46342 ) ;
#8724=ORIENTED_EDGE ( 'NONE', *, *, #25830, .T. ) ;
#8725=CARTESIAN_POINT ( 'NONE',  ( -74.51199343215201054, -183.6283474603465606, -122.2591094863194883 ) ) ;
#8728=ORIENTED_EDGE ( 'NONE', *, *, #37827, .F. ) ;
#8729=ORIENTED_EDGE ( 'NONE', *, *, #40693, .F. ) ;
#8731=CARTESIAN_POINT ( 'NONE',  ( -12.76653800058364574, -189.7472609257535510, -119.7898618611244927 ) ) ;
#8733=DIRECTION ( 'NONE',  ( 0.000000000000000000, 0.000000000000000000, 1.000000000000000000 ) ) ;
#8735=ORIENTED_EDGE ( 'NONE', *, *, #36276, .T. ) ;
#8736=ORIENTED_EDGE ( 'NONE', *, *, #51700, .F. ) ;
#8737=CARTESIAN_POINT ( 'NONE',  ( -55.71438232577009586, -193.5000000000000000, -124.7904286264580804 ) ) ;
#8739=PLANE ( 'NONE',  #36715 ) ;
#8740=VERTEX_POINT ( 'NONE', #35397 ) ;
#8742=CARTESIAN_POINT ( 'NONE',  ( -47.48307690889363641, -193.5000000000000000, 0.08879589532294547560 ) ) ;
#8743=CIRCLE ( 'NONE', #38119, 125.0000000000000000 ) ;
#8744=ORIENTED_EDGE ( 'NONE', *, *, #22642, .F. ) ;
#8746=EDGE_LOOP ( 'NONE', ( #13809, #15390, #45727, #4872 ) ) ;
#8747=AXIS2_PLACEMENT_3D ( 'NONE', #2824, #26740, #30670 ) ;
#8751=CIRCLE ( 'NONE', #381, 125.0000000000000000 ) ;
#8753=ORIENTED_EDGE ( 'NONE', *, *, #22934, .T. ) ;
#8754=VERTEX_POINT ( 'NONE', #3872 ) ;
#8756=DIRECTION ( 'NONE',  ( 0.000000000000000000, -1.000000000000000000, 0.000000000000000000 ) ) ;
#8758=EDGE_CURVE ( 'NONE', #49289, #28894, #15967, .T. ) ;
#8759=LINE ( 'NONE', #37135, #46696 ) ;
#8763=AXIS2_PLACEMENT_3D ( 'NONE', #50332, #10369, #26395 ) ;
#8764=DIRECTION ( 'NONE',  ( -0.000000000000000000, 1.000000000000000000, -0.000000000000000000 ) ) ;
#8765=ORIENTED_EDGE ( 'NONE', *, *, #10900, .T. ) ;
#8766=LINE ( 'NONE', #9306, #23221 ) ;
#8767=ORIENTED_EDGE ( 'NONE', *, *, #42322, .F. ) ;
#8769=CARTESIAN_POINT ( 'NONE',  ( -63.43218022845230308, -189.7472609257535510, 124.1024020384604540 ) ) ;
#8770=ORIENTED_EDGE ( 'NONE', *, *, #27023, .T. ) ;
#8771=CARTESIAN_POINT ( 'NONE',  ( 63.31225588004632243, -193.5000000000000000, 55.92572546981597981 ) ) ;
#8775=DIRECTION ( 'NONE',  ( 0.000000000000000000, 1.000000000000000000, -0.000000000000000000 ) ) ;
#8776=ORIENTED_EDGE ( 'NONE', *, *, #44358, .F. ) ;
#8778=ORIENTED_EDGE ( 'NONE', *, *, #6812, .F. ) ;
#8780=ADVANCED_FACE ( 'NONE', ( #34876 ), #39589, .T. ) ;
#8782=DIRECTION ( 'NONE',  ( 0.8757349421956345248, 0.000000000000000000, 0.4827922027307490205 ) ) ;
#8783=EDGE_LOOP ( 'NONE', ( #17579, #25725, #2681, #7280 ) ) ;
#8784=CIRCLE ( 'NONE', #28925, 125.0000000000000000 ) ;
#8787=CARTESIAN_POINT ( 'NONE',  ( 65.12862465015750502, -193.5000000000000000, 49.69312418816386412 ) ) ;
#8789=EDGE_CURVE ( 'NONE', #47477, #11775, #50941, .T. ) ;
#8790=DIRECTION ( 'NONE',  ( 0.000000000000000000, 0.000000000000000000, -1.000000000000000000 ) ) ;
#8791=ORIENTED_EDGE ( 'NONE', *, *, #44089, .F. ) ;
#8794=DIRECTION ( 'NONE',  ( -0.000000000000000000, 1.000000000000000000, -0.000000000000000000 ) ) ;
#8796=ADVANCED_FACE ( 'NONE', ( #46995 ), #19896, .T. ) ;
#8797=LINE ( 'NONE', #20909, #19365 ) ;
#8798=AXIS2_PLACEMENT_3D ( 'NONE', #19727, #15286, #43656 ) ;
#8799=PLANE ( 'NONE',  #4761 ) ;
#8800=VERTEX_POINT ( 'NONE', #10975 ) ;
#8802=EDGE_CURVE ( 'NONE', #26457, #10145, #47504, .T. ) ;
#8803=ORIENTED_EDGE ( 'NONE', *, *, #6919, .T. ) ;
#8805=CARTESIAN_POINT ( 'NONE',  ( 52.59568867645218404, -175.3837268820161057, -73.54509967498589162 ) ) ;
#8806=EDGE_CURVE ( 'NONE', #7086, #21227, #43839, .T. ) ;
#8807=DIRECTION ( 'NONE',  ( 0.9785564922995017012, 0.000000000000000000, 0.2059786187411094538 ) ) ;
#8810=ORIENTED_EDGE ( 'NONE', *, *, #48536, .F. ) ;
#8811=ORIENTED_EDGE ( 'NONE', *, *, #18487, .F. ) ;
#8812=CARTESIAN_POINT ( 'NONE',  ( 8.294189685504184339, -175.3837268820161057, -110.2396968984190977 ) ) ;
#8813=VERTEX_POINT ( 'NONE', #35146 ) ;
#8814=DIRECTION ( 'NONE',  ( 0.000000000000000000, -1.000000000000000000, 0.000000000000000000 ) ) ;
#8815=ORIENTED_EDGE ( 'NONE', *, *, #46036, .T. ) ;
#8816=VECTOR ( 'NONE', #14020, 1000.000000000000000 ) ;
#8817=CARTESIAN_POINT ( 'NONE',  ( -49.08592689732743963, -189.7472609257535510, -0.7948544414133539293 ) ) ;
#8818=EDGE_CURVE ( 'NONE', #10133, #38089, #15190, .T. ) ;
#8819=DIRECTION ( 'NONE',  ( 0.000000000000000000, -0.000000000000000000, 1.000000000000000000 ) ) ;
#8820=AXIS2_PLACEMENT_3D ( 'NONE', #45178, #37528, #8626 ) ;
#8821=AXIS2_PLACEMENT_3D ( 'NONE', #4137, #20150, #36172 ) ;
#8822=CARTESIAN_POINT ( 'NONE',  ( -164.0008810331606526, -189.7472609257535510, 47.74645837849825369 ) ) ;
#8823=CARTESIAN_POINT ( 'NONE',  ( -152.0588566364587848, -177.1207230881787780, -68.17212999877148150 ) ) ;
#8826=EDGE_LOOP ( 'NONE', ( #5293, #45850, #48432, #46718 ) ) ;
#8827=ADVANCED_FACE ( 'NONE', ( #7301 ), #28293, .T. ) ;
#8828=AXIS2_PLACEMENT_3D ( 'NONE', #24885, #36717, #28034 ) ;
#8830=FACE_OUTER_BOUND ( 'NONE', #37164, .T. ) ;
#8831=CYLINDRICAL_SURFACE ( 'NONE', #11041, 125.0000000000000000 ) ;
#8834=CARTESIAN_POINT ( 'NONE',  ( -55.99477380783403646, -193.5000000000000000, 123.7720294769269600 ) ) ;
#8835=FACE_OUTER_BOUND ( 'NONE', #27952, .T. ) ;
#8836=DIRECTION ( 'NONE',  ( 0.000000000000000000, -0.000000000000000000, -1.000000000000000000 ) ) ;
#8837=DIRECTION ( 'NONE',  ( 0.000000000000000000, 0.000000000000000000, 1.000000000000000000 ) ) ;
#8838=VERTEX_POINT ( 'NONE', #24113 ) ;
#8839=VECTOR ( 'NONE', #3975, 1000.000000000000000 ) ;
#8843=AXIS2_PLACEMENT_3D ( 'NONE', #12360, #44435, #48903 ) ;
#8844=FACE_BOUND ( 'NONE', #5459, .T. ) ;
#8845=ORIENTED_EDGE ( 'NONE', *, *, #35940, .F. ) ;
#8846=CARTESIAN_POINT ( 'NONE',  ( -20.16057156355606139, -193.5000000000000000, -120.7230919990158782 ) ) ;
#8847=ORIENTED_EDGE ( 'NONE', *, *, #37281, .T. ) ;
#8848=CARTESIAN_POINT ( 'NONE',  ( -23.99795575808071035, -193.5000000000000000, -122.5792489240757703 ) ) ;
#8849=EDGE_CURVE ( 'NONE', #32529, #9666, #48553, .T. ) ;
#8850=ORIENTED_EDGE ( 'NONE', *, *, #49403, .F. ) ;
#8851=EDGE_CURVE ( 'NONE', #28628, #51319, #20669, .T. ) ;
#8853=ORIENTED_EDGE ( 'NONE', *, *, #46117, .T. ) ;
#8854=CARTESIAN_POINT ( 'NONE',  ( 66.03142248012325410, -177.1207230881787780, 50.12318939044039467 ) ) ;
#8856=DIRECTION ( 'NONE',  ( 0.9266896074318343723, 0.000000000000000000, -0.3758275821142357809 ) ) ;
#8857=ORIENTED_EDGE ( 'NONE', *, *, #23774, .F. ) ;
#8858=CIRCLE ( 'NONE', #2141, 125.0000000000000000 ) ;
#8860=EDGE_CURVE ( 'NONE', #17733, #20353, #36963, .T. ) ;
#8863=ORIENTED_EDGE ( 'NONE', *, *, #10537, .T. ) ;
#8864=EDGE_CURVE ( 'NONE', #48760, #10162, #32760, .T. ) ;
#8865=VERTEX_POINT ( 'NONE', #4918 ) ;
#8868=CARTESIAN_POINT ( 'NONE',  ( -130.2106798473772642, -175.3837268820161057, 94.57776286494217288 ) ) ;
#8869=EDGE_CURVE ( 'NONE', #27646, #39413, #5177, .T. ) ;
#8871=VECTOR ( 'NONE', #45107, 1000.000000000000227 ) ;
#8872=DIRECTION ( 'NONE',  ( -0.000000000000000000, 1.000000000000000000, -0.000000000000000000 ) ) ;
#8873=VECTOR ( 'NONE', #4916, 1000.000000000000000 ) ;
#8874=CARTESIAN_POINT ( 'NONE',  ( 56.28386853063362594, -175.3837268820161057, 66.33788548805519270 ) ) ;
#8875=DIRECTION ( 'NONE',  ( -0.000000000000000000, 1.000000000000000000, -0.000000000000000000 ) ) ;
#8876=ADVANCED_FACE ( 'NONE', ( #8069 ), #9115, .T. ) ;
#8878=CIRCLE ( 'NONE', #2169, 125.0000000000000000 ) ;
#8881=VERTEX_POINT ( 'NONE', #40121 ) ;
#8883=DIRECTION ( 'NONE',  ( 0.000000000000000000, -0.000000000000000000, -1.000000000000000000 ) ) ;
#8884=EDGE_LOOP ( 'NONE', ( #8229, #6447, #10253, #9230 ) ) ;
#8886=DIRECTION ( 'NONE',  ( 0.000000000000000000, 0.000000000000000000, -1.000000000000000000 ) ) ;
#8889=DIRECTION ( 'NONE',  ( -0.000000000000000000, 1.000000000000000000, -0.000000000000000000 ) ) ;
#8891=ORIENTED_EDGE ( 'NONE', *, *, #15136, .T. ) ;
#8894=VERTEX_POINT ( 'NONE', #20153 ) ;
#8896=AXIS2_PLACEMENT_3D ( 'NONE', #34123, #38830, #50175 ) ;
#8897=CARTESIAN_POINT ( 'NONE',  ( -134.9506378406916838, -175.3837268820161057, 90.26448786734087548 ) ) ;
#8899=DIRECTION ( 'NONE',  ( 0.000000000000000000, -0.000000000000000000, -1.000000000000000000 ) ) ;
#8901=ORIENTED_EDGE ( 'NONE', *, *, #22111, .T. ) ;
#8902=AXIS2_PLACEMENT_3D ( 'NONE', #27577, #39643, #3656 ) ;
#8903=CARTESIAN_POINT ( 'NONE',  ( -48.93575598890257794, -177.1207230881787780, 0.8896570909947506545 ) ) ;
#8904=CIRCLE ( 'NONE', #8079, 125.0000000000000000 ) ;
#8906=FACE_OUTER_BOUND ( 'NONE', #22726, .T. ) ;
#8909=DIRECTION ( 'NONE',  ( -0.000000000000000000, 1.000000000000000000, -0.000000000000000000 ) ) ;
#8910=ORIENTED_EDGE ( 'NONE', *, *, #6453, .T. ) ;
#8912=CARTESIAN_POINT ( 'NONE',  ( -28.86423599357335590, -177.1207230881787780, 122.4396006697296144 ) ) ;
#8913=AXIS2_PLACEMENT_3D ( 'NONE', #23950, #16082, #16613 ) ;
#8914=EDGE_CURVE ( 'NONE', #44523, #14995, #36175, .T. ) ;
#8915=CIRCLE ( 'NONE', #38277, 125.0000000000000000 ) ;
#8916=VECTOR ( 'NONE', #12049, 1000.000000000000000 ) ;
#8917=ADVANCED_FACE ( 'NONE', ( #49056 ), #20943, .T. ) ;
#8918=FACE_OUTER_BOUND ( 'NONE', #19122, .T. ) ;
#8919=DIRECTION ( 'NONE',  ( 0.000000000000000000, -1.000000000000000000, 0.000000000000000000 ) ) ;
#8920=EDGE_CURVE ( 'NONE', #246, #16275, #48898, .T. ) ;
#8921=VERTEX_POINT ( 'NONE', #40894 ) ;
#8925=ORIENTED_EDGE ( 'NONE', *, *, #34601, .T. ) ;
#8926=ADVANCED_FACE ( 'NONE', ( #29062 ), #12258, .T. ) ;
#8927=VECTOR ( 'NONE', #46666, 1000.000000000000000 ) ;
#8929=EDGE_CURVE ( 'NONE', #49151, #14954, #20406, .T. ) ;
#8930=PLANE ( 'NONE',  #42142 ) ;
#8932=DIRECTION ( 'NONE',  ( 0.000000000000000000, -1.000000000000000000, 0.000000000000000000 ) ) ;
#8933=ORIENTED_EDGE ( 'NONE', *, *, #15183, .T. ) ;
#8935=EDGE_CURVE ( 'NONE', #43736, #10566, #25144, .T. ) ;
#8937=ORIENTED_EDGE ( 'NONE', *, *, #48831, .T. ) ;
#8939=FACE_OUTER_BOUND ( 'NONE', #9823, .T. ) ;
#8940=ORIENTED_EDGE ( 'NONE', *, *, #20215, .T. ) ;
#8941=CARTESIAN_POINT ( 'NONE',  ( 59.80284513346456521, -183.6283474603465606, 62.45009659481583242 ) ) ;
#8942=AXIS2_PLACEMENT_3D ( 'NONE', #15970, #19384, #19135 ) ;
#8943=AXIS2_PLACEMENT_3D ( 'NONE', #12195, #44274, #47954 ) ;
#8945=ORIENTED_EDGE ( 'NONE', *, *, #8986, .T. ) ;
#8946=DIRECTION ( 'NONE',  ( 0.000000000000000000, 0.000000000000000000, -1.000000000000000000 ) ) ;
#8947=AXIS2_PLACEMENT_3D ( 'NONE', #18066, #14642, #5982 ) ;
#8948=ADVANCED_FACE ( 'NONE', ( #17261 ), #41937, .F. ) ;
#8949=EDGE_CURVE ( 'NONE', #19112, #24906, #43025, .T. ) ;
#8950=CARTESIAN_POINT ( 'NONE',  ( -130.7087404384255080, -189.7472609257535510, -94.14505102712755047 ) ) ;
#8953=ORIENTED_EDGE ( 'NONE', *, *, #47659, .T. ) ;
#8954=CIRCLE ( 'NONE', #5632, 125.0000000000000000 ) ;
#8956=VECTOR ( 'NONE', #24787, 1000.000000000000000 ) ;
#8958=AXIS2_PLACEMENT_3D ( 'NONE', #15900, #50418, #38307 ) ;
#8959=EDGE_LOOP ( 'NONE', ( #30667, #5756, #15138, #1029 ) ) ;
#8960=CARTESIAN_POINT ( 'NONE',  ( -48.47912675150885065, -183.6283474603465606, 6.938893903907228378E-15 ) ) ;
#8962=ORIENTED_EDGE ( 'NONE', *, *, #24967, .F. ) ;
#8967=VERTEX_POINT ( 'NONE', #18299 ) ;
#8968=VECTOR ( 'NONE', #12687, 999.9999999999998863 ) ;
#8970=CARTESIAN_POINT ( 'NONE',  ( 73.66680038934278230, -189.7472609257535510, -26.55884942729568365 ) ) ;
#8971=FACE_OUTER_BOUND ( 'NONE', #39132, .T. ) ;
#8972=ORIENTED_EDGE ( 'NONE', *, *, #49555, .F. ) ;
#8973=CARTESIAN_POINT ( 'NONE',  ( -150.5215542367829471, -175.3837268820161057, -72.19655804061974891 ) ) ;
#8974=CARTESIAN_POINT ( 'NONE',  ( 5.139251539934009294, -183.6283474603465606, 111.8087531435657951 ) ) ;
#8975=DIRECTION ( 'NONE',  ( 0.9564009842765244240, 0.000000000000000000, -0.2920567706369695538 ) ) ;
#8976=ORIENTED_EDGE ( 'NONE', *, *, #42064, .T. ) ;
#8977=DIRECTION ( 'NONE',  ( -0.000000000000000000, 1.000000000000000000, -0.000000000000000000 ) ) ;
#8978=ADVANCED_FACE ( 'NONE', ( #9892 ), #2264, .T. ) ;
#8979=DIRECTION ( 'NONE',  ( -0.000000000000000000, 1.000000000000000000, -0.000000000000000000 ) ) ;
#8980=ORIENTED_EDGE ( 'NONE', *, *, #21333, .F. ) ;
#8982=AXIS2_PLACEMENT_3D ( 'NONE', #2965, #7685, #50553 ) ;
#8983=CARTESIAN_POINT ( 'NONE',  ( -27.36201831380532923, -175.3837268820161057, -122.1886788576022411 ) ) ;
#8984=CARTESIAN_POINT ( 'NONE',  ( -48.47912675150885065, -175.3837268820161057, 6.938893903907228378E-15 ) ) ;
#8986=EDGE_CURVE ( 'NONE', #28248, #19289, #34617, .T. ) ;
#8990=EDGE_CURVE ( 'NONE', #44410, #1407, #41330, .T. ) ;
#8992=EDGE_CURVE ( 'NONE', #1774, #14215, #40500, .T. ) ;
#8993=FACE_OUTER_BOUND ( 'NONE', #1890, .T. ) ;
#8996=DIRECTION ( 'NONE',  ( 0.000000000000000000, 1.000000000000000000, 0.000000000000000000 ) ) ;
#8997=CARTESIAN_POINT ( 'NONE',  ( -49.45768324380835423, -193.5000000000000000, 0.2059786187410958813 ) ) ;
#9000=AXIS2_PLACEMENT_3D ( 'NONE', #2677, #43412, #18462 ) ;
#9001=VECTOR ( 'NONE', #3229, 1000.000000000000114 ) ;
#9002=VERTEX_POINT ( 'NONE', #41677 ) ;
#9004=AXIS2_PLACEMENT_3D ( 'NONE', #27152, #51352, #20051 ) ;
#9005=VECTOR ( 'NONE', #5030, 1000.000000000000114 ) ;
#9007=VERTEX_POINT ( 'NONE', #46161 ) ;
#9008=VERTEX_POINT ( 'NONE', #45899 ) ;
#9010=EDGE_LOOP ( 'NONE', ( #29529, #41628, #34097, #18581 ) ) ;
#9011=DIRECTION ( 'NONE',  ( 0.000000000000000000, 0.000000000000000000, -1.000000000000000000 ) ) ;
#9012=EDGE_CURVE ( 'NONE', #31844, #17957, #31275, .T. ) ;
#9014=CYLINDRICAL_SURFACE ( 'NONE', #50986, 125.0000000000000000 ) ;
#9015=ORIENTED_EDGE ( 'NONE', *, *, #48758, .T. ) ;
#9016=ORIENTED_EDGE ( 'NONE', *, *, #19984, .T. ) ;
#9017=EDGE_CURVE ( 'NONE', #22760, #4153, #37995, .T. ) ;
#9018=CARTESIAN_POINT ( 'NONE',  ( -169.0136227435421006, -175.3837268820161057, -33.11246405730811659 ) ) ;
#9020=PLANE ( 'NONE',  #33344 ) ;
#9021=ORIENTED_EDGE ( 'NONE', *, *, #22438, .F. ) ;
#9023=CARTESIAN_POINT ( 'NONE',  ( 26.52087324849106054, -198.5000000000000000, -70.00000000000002842 ) ) ;
#9024=ORIENTED_EDGE ( 'NONE', *, *, #2553, .F. ) ;
#9025=CARTESIAN_POINT ( 'NONE',  ( 46.40005841627163363, -183.6283474603465606, 81.38144888055276738 ) ) ;
#9027=ORIENTED_EDGE ( 'NONE', *, *, #34491, .T. ) ;
#9028=FACE_OUTER_BOUND ( 'NONE', #35033, .T. ) ;
#9034=CARTESIAN_POINT ( 'NONE',  ( 55.03325008324586776, -193.5000000000000000, -70.07273251429357686 ) ) ;
#9035=FACE_OUTER_BOUND ( 'NONE', #46857, .T. ) ;
#9037=ORIENTED_EDGE ( 'NONE', *, *, #2923, .F. ) ;
#9038=CARTESIAN_POINT ( 'NONE',  ( -48.47912675150885065, -189.7472609257535510, 6.938893903907228378E-15 ) ) ;
#9040=CARTESIAN_POINT ( 'NONE',  ( -19.28375372365792728, -175.3837268820161057, 121.5427093402341541 ) ) ;
#9041=EDGE_LOOP ( 'NONE', ( #31740, #27869, #4933, #6970 ) ) ;
#9042=LINE ( 'NONE', #21649, #40138 ) ;
#9043=AXIS2_PLACEMENT_3D ( 'NONE', #49457, #9492, #25512 ) ;
#9045=CIRCLE ( 'NONE', #26634, 125.0000000000000000 ) ;
#9047=CARTESIAN_POINT ( 'NONE',  ( 8.750818922897904528, -193.5000000000000000, -111.1293539894138434 ) ) ;
#9049=DIRECTION ( 'NONE',  ( -0.000000000000000000, 1.000000000000000000, -0.000000000000000000 ) ) ;
#9050=CARTESIAN_POINT ( 'NONE',  ( -141.2664123866436796, -175.3837268820161057, -83.75869879877495805 ) ) ;
#9052=DIRECTION ( 'NONE',  ( 0.000000000000000000, -1.000000000000000000, -0.000000000000000000 ) ) ;
#9053=CARTESIAN_POINT ( 'NONE',  ( -118.9967449635792320, -189.7472609257535510, -103.2098131075562009 ) ) ;
#9055=ADVANCED_FACE ( 'NONE', ( #21454 ), #22224, .T. ) ;
#9056=ADVANCED_FACE ( 'NONE', ( #5436 ), #38517, .T. ) ;
#9057=CARTESIAN_POINT ( 'NONE',  ( -85.14888725715766782, -189.7472609257535510, 119.5003291395398719 ) ) ;
#9059=CARTESIAN_POINT ( 'NONE',  ( -144.0067397530739584, -183.6283474603465606, -80.61932246194587037 ) ) ;
#9064=DIRECTION ( 'NONE',  ( -0.05924062789370006937, 0.000000000000000000, -0.9982437317643222396 ) ) ;
#9067=CIRCLE ( 'NONE', #25010, 125.0000000000000000 ) ;
#9074=PLANE ( 'NONE',  #28102 ) ;
#9075=EDGE_CURVE ( 'NONE', #46251, #51992, #14349, .T. ) ;
#9076=EDGE_LOOP ( 'NONE', ( #23271, #45182, #36020, #9292 ) ) ;
#9077=DIRECTION ( 'NONE',  ( 0.000000000000000000, 0.000000000000000000, 1.000000000000000000 ) ) ;
#9080=CARTESIAN_POINT ( 'NONE',  ( 33.75048693540708911, -175.3837268820161057, 94.14505102712816154 ) ) ;
#9081=ORIENTED_EDGE ( 'NONE', *, *, #38469, .F. ) ;
#9082=EDGE_LOOP ( 'NONE', ( #42264, #16111, #21183, #1903 ) ) ;
#9083=ADVANCED_FACE ( 'NONE', ( #6476 ), #37479, .T. ) ;
#9086=DIRECTION ( 'NONE',  ( 0.6528221181905174975, 0.000000000000000000, 0.7575112421616236880 ) ) ;
#9087=DIRECTION ( 'NONE',  ( 0.4031234292879792847, 0.000000000000000000, -0.9151456172430153524 ) ) ;
#9088=DIRECTION ( 'NONE',  ( 0.000000000000000000, -0.000000000000000000, -1.000000000000000000 ) ) ;
#9091=ORIENTED_EDGE ( 'NONE', *, *, #49922, .T. ) ;
#9092=VERTEX_POINT ( 'NONE', #47185 ) ;
#9093=DIRECTION ( 'NONE',  ( -0.9473263538541946138, 0.000000000000000000, 0.3202698538628279690 ) ) ;
#9095=DIRECTION ( 'NONE',  ( -0.000000000000000000, 1.000000000000000000, -0.000000000000000000 ) ) ;
#9096=ORIENTED_EDGE ( 'NONE', *, *, #37233, .F. ) ;
#9097=CIRCLE ( 'NONE', #25042, 125.0000000000000000 ) ;
#9098=DIRECTION ( 'NONE',  ( -0.000000000000000000, 1.000000000000000000, -0.000000000000000000 ) ) ;
#9099=AXIS2_PLACEMENT_3D ( 'NONE', #40467, #20504, #12616 ) ;
#9101=VECTOR ( 'NONE', #16897, 1000.000000000000000 ) ;
#9103=DIRECTION ( 'NONE',  ( 0.000000000000000000, 0.000000000000000000, 1.000000000000000000 ) ) ;
#9104=CARTESIAN_POINT ( 'NONE',  ( -165.5546359831674295, -193.5000000000000000, 43.79868877201493405 ) ) ;
#9106=CARTESIAN_POINT ( 'NONE',  ( 40.26790151320557953, -183.6283474603465606, -86.60307583628355133 ) ) ;
#9108=EDGE_CURVE ( 'NONE', #15949, #33758, #35771, .T. ) ;
#9109=ORIENTED_EDGE ( 'NONE', *, *, #9328, .T. ) ;
#9110=PLANE ( 'NONE',  #27086 ) ;
#9114=PLANE ( 'NONE',  #23839 ) ;
#9115=CYLINDRICAL_SURFACE ( 'NONE', #35435, 125.0000000000000000 ) ;
#9116=EDGE_CURVE ( 'NONE', #32483, #31844, #35861, .T. ) ;
#9117=EDGE_LOOP ( 'NONE', ( #43077, #31071, #6107, #28256 ) ) ;
#9119=CARTESIAN_POINT ( 'NONE',  ( 29.27398957514435196, -183.6283474603465606, -97.87467957287998388 ) ) ;
#9120=AXIS2_PLACEMENT_3D ( 'NONE', #28850, #44903, #24931 ) ;
#9122=FACE_BOUND ( 'NONE', #38135, .T. ) ;
#9123=ORIENTED_EDGE ( 'NONE', *, *, #18876, .T. ) ;
#9125=CYLINDRICAL_SURFACE ( 'NONE', #38199, 125.0000000000000000 ) ;
#9126=ORIENTED_EDGE ( 'NONE', *, *, #41799, .T. ) ;
#9127=FACE_OUTER_BOUND ( 'NONE', #51157, .T. ) ;
#9128=ORIENTED_EDGE ( 'NONE', *, *, #14380, .T. ) ;
#9130=ORIENTED_EDGE ( 'NONE', *, *, #6366, .T. ) ;
#9131=DIRECTION ( 'NONE',  ( -0.000000000000000000, 1.000000000000000000, 0.000000000000000000 ) ) ;
#9133=VECTOR ( 'NONE', #7990, 1000.000000000000000 ) ;
#9134=AXIS2_PLACEMENT_3D ( 'NONE', #47023, #14451, #14197 ) ;
#9137=EDGE_LOOP ( 'NONE', ( #25847, #16592, #36005, #15858 ) ) ;
#9139=CIRCLE ( 'NONE', #22574, 125.0000000000000000 ) ;
#9140=PLANE ( 'NONE',  #39 ) ;
#9141=ORIENTED_EDGE ( 'NONE', *, *, #2243, .F. ) ;
#9143=EDGE_LOOP ( 'NONE', ( #19156, #42009, #40980, #2493 ) ) ;
#9144=CARTESIAN_POINT ( 'NONE',  ( 64.86941505090324256, -193.5000000000000000, -50.28156562190505241 ) ) ;
#9145=AXIS2_PLACEMENT_3D ( 'NONE', #49862, #13067, #45665 ) ;
#9146=CARTESIAN_POINT ( 'NONE',  ( -88.78924379339714790, -193.5000000000000000, -118.3219948448692520 ) ) ;
#9147=ORIENTED_EDGE ( 'NONE', *, *, #38153, .F. ) ;
#9148=DIRECTION ( 'NONE',  ( -0.000000000000000000, 1.000000000000000000, -0.000000000000000000 ) ) ;
#9151=ORIENTED_EDGE ( 'NONE', *, *, #5451, .T. ) ;
#9152=AXIS2_PLACEMENT_3D ( 'NONE', #40108, #45114, #16742 ) ;
#9153=LINE ( 'NONE', #21235, #35116 ) ;
#9154=DIRECTION ( 'NONE',  ( -0.000000000000000000, 1.000000000000000000, -0.000000000000000000 ) ) ;
#9155=ORIENTED_EDGE ( 'NONE', *, *, #8990, .T. ) ;
#9157=CARTESIAN_POINT ( 'NONE',  ( -73.94077438226447896, -193.5000000000000000, 122.3793467049372481 ) ) ;
#9158=ORIENTED_EDGE ( 'NONE', *, *, #12826, .T. ) ;
#9159=ORIENTED_EDGE ( 'NONE', *, *, #32175, .T. ) ;
#9160=CARTESIAN_POINT ( 'NONE',  ( 60.58466639580034041, -189.7472609257535510, -61.07445476073405644 ) ) ;
#9163=ADVANCED_FACE ( 'NONE', ( #27711 ), #27186, .T. ) ;
#9164=EDGE_LOOP ( 'NONE', ( #48066, #26868, #5553, #40969 ) ) ;
#9165=EDGE_CURVE ( 'NONE', #33115, #49764, #19068, .T. ) ;
#9167=CARTESIAN_POINT ( 'NONE',  ( -170.9669310976187830, -189.7472609257535510, -24.93467037017130394 ) ) ;
#9169=CARTESIAN_POINT ( 'NONE',  ( -48.47912675150885065, -213.5000000000000000, 6.938893903907228378E-15 ) ) ;
#9170=EDGE_LOOP ( 'NONE', ( #11886, #947, #34394, #15486 ) ) ;
#9171=EDGE_CURVE ( 'NONE', #9853, #20140, #23520, .T. ) ;
#9173=DIRECTION ( 'NONE',  ( -0.000000000000000000, 1.000000000000000000, -0.000000000000000000 ) ) ;
#9174=DIRECTION ( 'NONE',  ( 0.000000000000000000, 1.000000000000000000, 0.000000000000000000 ) ) ;
#9177=FACE_OUTER_BOUND ( 'NONE', #6768, .T. ) ;
#9178=EDGE_LOOP ( 'NONE', ( #22589, #10495, #21375, #29223 ) ) ;
#9179=VECTOR ( 'NONE', #4413, 1000.000000000000000 ) ;
#9182=CARTESIAN_POINT ( 'NONE',  ( -47.92047998570520662, -193.5000000000000000, 0.8294056854502119824 ) ) ;
#9184=EDGE_CURVE ( 'NONE', #21155, #40815, #49192, .T. ) ;
#9187=ADVANCED_FACE ( 'NONE', ( #46938 ), #39290, .F. ) ;
#9188=EDGE_CURVE ( 'NONE', #34792, #18880, #23274, .T. ) ;
#9190=ORIENTED_EDGE ( 'NONE', *, *, #9604, .T. ) ;
#9194=CARTESIAN_POINT ( 'NONE',  ( 28.02885774092382221, -175.3837268820161057, 98.85104101073332572 ) ) ;
#9195=ORIENTED_EDGE ( 'NONE', *, *, #32175, .F. ) ;
#9196=CARTESIAN_POINT ( 'NONE',  ( -91.84482189527184914, -189.7472609257535510, -117.2365833888816837 ) ) ;
#9199=PLANE ( 'NONE',  #37677 ) ;
#9200=DIRECTION ( 'NONE',  ( 0.2348860457809911206, 0.000000000000000000, -0.9720229140804089729 ) ) ;
#9201=LINE ( 'NONE', #33096, #50601 ) ;
#9202=DIRECTION ( 'NONE',  ( 0.000000000000000000, 0.000000000000000000, -1.000000000000000000 ) ) ;
#9203=VERTEX_POINT ( 'NONE', #27456 ) ;
#9211=CARTESIAN_POINT ( 'NONE',  ( -48.47912675150885065, -189.7472609257535510, 6.938893903907228378E-15 ) ) ;
#9213=CARTESIAN_POINT ( 'NONE',  ( 53.56330073376472001, -193.5000000000000000, 72.19655804062048787 ) ) ;
#9215=ORIENTED_EDGE ( 'NONE', *, *, #2243, .T. ) ;
#9217=CARTESIAN_POINT ( 'NONE',  ( -48.02249751411513756, -177.1207230881787780, -0.8896570909947397743 ) ) ;
#9218=ORIENTED_EDGE ( 'NONE', *, *, #37420, .T. ) ;
#9219=DIRECTION ( 'NONE',  ( 0.000000000000000000, 0.000000000000000000, 1.000000000000000000 ) ) ;
#9220=ORIENTED_EDGE ( 'NONE', *, *, #39204, .F. ) ;
#9221=DIRECTION ( 'NONE',  ( -0.5586467658036415873, 0.000000000000000000, -0.8294056854502090959 ) ) ;
#9224=EDGE_CURVE ( 'NONE', #40095, #43678, #43498, .T. ) ;
#9225=EDGE_CURVE ( 'NONE', #38326, #19688, #41626, .T. ) ;
#9226=EDGE_CURVE ( 'NONE', #14956, #47094, #37428, .T. ) ;
#9227=DIRECTION ( 'NONE',  ( 0.000000000000000000, -1.000000000000000000, 0.000000000000000000 ) ) ;
#9229=LINE ( 'NONE', #28131, #11373 ) ;
#9230=ORIENTED_EDGE ( 'NONE', *, *, #2705, .F. ) ;
#9231=ORIENTED_EDGE ( 'NONE', *, *, #30769, .F. ) ;
#9233=CARTESIAN_POINT ( 'NONE',  ( -119.6907301311197216, -177.1207230881787780, 101.5140743725400370 ) ) ;
#9234=LINE ( 'NONE', #21585, #19443 ) ;
#9236=ORIENTED_EDGE ( 'NONE', *, *, #24401, .T. ) ;
#9238=DIRECTION ( 'NONE',  ( -0.000000000000000000, 1.000000000000000000, -0.000000000000000000 ) ) ;
#9239=ADVANCED_FACE ( 'NONE', ( #47709 ), #11687, .T. ) ;
#9240=CYLINDRICAL_SURFACE ( 'NONE', #4164, 125.0000000000000000 ) ;
#9241=FACE_OUTER_BOUND ( 'NONE', #27295, .T. ) ;
#9242=VERTEX_POINT ( 'NONE', #39783 ) ;
#9243=ADVANCED_FACE ( 'NONE', ( #6726 ), #38756, .T. ) ;
#9245=CARTESIAN_POINT ( 'NONE',  ( 76.21810084846656252, -193.5000000000000000, -8.694908215727984668 ) ) ;
#9247=DIRECTION ( 'NONE',  ( 0.000000000000000000, 1.000000000000000000, 0.000000000000000000 ) ) ;
#9252=FACE_OUTER_BOUND ( 'NONE', #50515, .T. ) ;
#9253=ADVANCED_FACE ( 'NONE', ( #24648 ), #48588, .F. ) ;
#9254=FACE_OUTER_BOUND ( 'NONE', #33706, .T. ) ;
#9256=LINE ( 'NONE', #836, #22924 ) ;
#9257=CARTESIAN_POINT ( 'NONE',  ( -49.46816693883101834, -189.7472609257535510, 0.1476465640024780257 ) ) ;
#9259=LINE ( 'NONE', #29469, #44681 ) ;
#9261=ORIENTED_EDGE ( 'NONE', *, *, #40126, .F. ) ;
#9262=PLANE ( 'NONE',  #49283 ) ;
#9264=VECTOR ( 'NONE', #42937, 1000.000000000000114 ) ;
#9265=DIRECTION ( 'NONE',  ( 0.000000000000000000, 0.000000000000000000, -1.000000000000000000 ) ) ;
#9266=DIRECTION ( 'NONE',  ( 0.000000000000000000, -0.000000000000000000, -1.000000000000000000 ) ) ;
#9267=EDGE_LOOP ( 'NONE', ( #47806, #33139, #33785, #7261 ) ) ;
#9269=EDGE_LOOP ( 'NONE', ( #21273, #37369, #37330, #46943 ) ) ;
#9270=DIRECTION ( 'NONE',  ( 0.000000000000000000, 0.000000000000000000, -1.000000000000000000 ) ) ;
#9271=DIRECTION ( 'NONE',  ( -0.000000000000000000, 1.000000000000000000, -0.000000000000000000 ) ) ;
#9276=CARTESIAN_POINT ( 'NONE',  ( -47.64924157374594671, -189.7472609257535510, 123.9972451320097377 ) ) ;
#9277=VERTEX_POINT ( 'NONE', #12814 ) ;
#9278=AXIS2_PLACEMENT_3D ( 'NONE', #46431, #10159, #37500 ) ;
#9280=ORIENTED_EDGE ( 'NONE', *, *, #20182, .T. ) ;
#9282=EDGE_LOOP ( 'NONE', ( #36969, #14937, #10155, #15798 ) ) ;
#9283=ADVANCED_FACE ( 'NONE', ( #28839 ), #42428, .T. ) ;
#9284=EDGE_CURVE ( 'NONE', #42609, #17165, #39924, .T. ) ;
#9285=ADVANCED_FACE ( 'NONE', ( #44891 ), #2237, .T. ) ;
#9287=DIRECTION ( 'NONE',  ( 0.000000000000000000, 1.000000000000000000, 0.000000000000000000 ) ) ;
#9291=ORIENTED_EDGE ( 'NONE', *, *, #47852, .T. ) ;
#9292=ORIENTED_EDGE ( 'NONE', *, *, #41933, .T. ) ;
#9293=DIRECTION ( 'NONE',  ( 0.8455960035018311727, 0.000000000000000000, -0.5338233779647826305 ) ) ;
#9295=ORIENTED_EDGE ( 'NONE', *, *, #41824, .T. ) ;
#9296=EDGE_CURVE ( 'NONE', #37279, #39766, #18278, .T. ) ;
#9297=DIRECTION ( 'NONE',  ( -0.000000000000000000, 1.000000000000000000, -0.000000000000000000 ) ) ;
#9300=EDGE_CURVE ( 'NONE', #29184, #29691, #464, .T. ) ;
#9304=VECTOR ( 'NONE', #23147, 1000.000000000000000 ) ;
#9305=ORIENTED_EDGE ( 'NONE', *, *, #37685, .T. ) ;
#9306=CARTESIAN_POINT ( 'NONE',  ( 51.05451324771861721, -183.6283474603465606, 75.61781872352699452 ) ) ;
#9307=VERTEX_POINT ( 'NONE', #33050 ) ;
#9308=CARTESIAN_POINT ( 'NONE',  ( 76.04209377433248562, -175.3837268820161057, -10.93003379476866677 ) ) ;
#9309=EDGE_CURVE ( 'NONE', #19466, #46209, #29366, .T. ) ;
#9312=ADVANCED_FACE ( 'NONE', ( #41192 ), #46139, .T. ) ;
#9314=DIRECTION ( 'NONE',  ( -0.02963332782257007553, 0.000000000000000000, 0.9995608365087941261 ) ) ;
#9315=DIRECTION ( 'NONE',  ( 0.000000000000000000, 1.000000000000000000, -0.000000000000000000 ) ) ;
#9316=DIRECTION ( 'NONE',  ( 0.000000000000000000, 0.000000000000000000, -1.000000000000000000 ) ) ;
#9317=EDGE_CURVE ( 'NONE', #43356, #17362, #13080, .T. ) ;
#9318=ORIENTED_EDGE ( 'NONE', *, *, #39642, .T. ) ;
#9320=ORIENTED_EDGE ( 'NONE', *, *, #2432, .T. ) ;
#9321=ORIENTED_EDGE ( 'NONE', *, *, #12756, .F. ) ;
#9322=VECTOR ( 'NONE', #31163, 1000.000000000000000 ) ;
#9325=VERTEX_POINT ( 'NONE', #39267 ) ;
#9326=VERTEX_POINT ( 'NONE', #42699 ) ;
#9328=EDGE_CURVE ( 'NONE', #25619, #46012, #26669, .T. ) ;
#9329=CARTESIAN_POINT ( 'NONE',  ( 8.879953965148883910, -175.3837268820161057, 109.9360785596608707 ) ) ;
#9331=CARTESIAN_POINT ( 'NONE',  ( -48.47912675150885065, -183.6283474603465606, 6.938893903907228378E-15 ) ) ;
#9332=EDGE_LOOP ( 'NONE', ( #22287, #14899, #13291, #16461 ) ) ;
#9334=DIRECTION ( 'NONE',  ( -0.000000000000000000, 1.000000000000000000, -0.000000000000000000 ) ) ;
#9336=DIRECTION ( 'NONE',  ( -0.000000000000000000, 1.000000000000000000, 0.000000000000000000 ) ) ;
#9342=PLANE ( 'NONE',  #15091 ) ;
#9344=DIRECTION ( 'NONE',  ( -0.000000000000000000, 1.000000000000000000, -0.000000000000000000 ) ) ;
#9345=ORIENTED_EDGE ( 'NONE', *, *, #13552, .F. ) ;
#9347=EDGE_CURVE ( 'NONE', #19097, #44141, #46915, .T. ) ;
#9348=EDGE_CURVE ( 'NONE', #20876, #13540, #3274, .T. ) ;
#9350=FACE_OUTER_BOUND ( 'NONE', #13777, .T. ) ;
#9352=CARTESIAN_POINT ( 'NONE',  ( -48.30223647638627682, -193.5000000000000000, -0.9842305779475897243 ) ) ;
#9353=VERTEX_POINT ( 'NONE', #51126 ) ;
#9354=AXIS2_PLACEMENT_3D ( 'NONE', #40007, #27677, #32385 ) ;
#9357=FACE_OUTER_BOUND ( 'NONE', #5591, .T. ) ;
#9359=DIRECTION ( 'NONE',  ( -0.8757349421956379665, 0.000000000000000000, 0.4827922027307427477 ) ) ;
#9360=VERTEX_POINT ( 'NONE', #18521 ) ;
#9362=ORIENTED_EDGE ( 'NONE', *, *, #8949, .F. ) ;
#9363=ORIENTED_EDGE ( 'NONE', *, *, #31220, .T. ) ;
#9366=DIRECTION ( 'NONE',  ( -0.000000000000000000, 1.000000000000000000, -0.000000000000000000 ) ) ;
#9367=VERTEX_POINT ( 'NONE', #43201 ) ;
#9368=VECTOR ( 'NONE', #50613, 1000.000000000000000 ) ;
#9372=DIRECTION ( 'NONE',  ( 0.000000000000000000, 0.000000000000000000, 1.000000000000000000 ) ) ;
#9373=CARTESIAN_POINT ( 'NONE',  ( -48.47912675150885065, -175.3837268820161057, 6.938893903907228378E-15 ) ) ;
#9374=CIRCLE ( 'NONE', #31191, 125.0000000000000000 ) ;
#9375=DIRECTION ( 'NONE',  ( -0.000000000000000000, -1.000000000000000000, 0.000000000000000000 ) ) ;
#9376=ADVANCED_FACE ( 'NONE', ( #6706 ), #35317, .T. ) ;
#9377=VECTOR ( 'NONE', #31023, 1000.000000000000114 ) ;
#9378=CARTESIAN_POINT ( 'NONE',  ( -47.70260288879081401, -183.6283474603465606, 0.6300878435817218737 ) ) ;
#9379=FACE_BOUND ( 'NONE', #51928, .T. ) ;
#9380=EDGE_LOOP ( 'NONE', ( #8175, #18014, #5541, #43730 ) ) ;
#9381=CARTESIAN_POINT ( 'NONE',  ( -48.71401279728984690, -193.5000000000000000, 0.9720229140804159673 ) ) ;
#9382=VERTEX_POINT ( 'NONE', #15113 ) ;
#9383=CARTESIAN_POINT ( 'NONE',  ( -155.9155026329808607, -193.5000000000000000, -61.91627321685031404 ) ) ;
#9386=ORIENTED_EDGE ( 'NONE', *, *, #18590, .T. ) ;
#9387=AXIS2_PLACEMENT_3D ( 'NONE', #40841, #24307, #16945 ) ;
#9388=FACE_OUTER_BOUND ( 'NONE', #15131, .T. ) ;
#9390=CYLINDRICAL_SURFACE ( 'NONE', #10013, 124.9999999999999858 ) ;
#9393=CARTESIAN_POINT ( 'NONE',  ( -68.21229068036657850, -183.6283474603465606, -123.4325817657429809 ) ) ;
#9394=VERTEX_POINT ( 'NONE', #51615 ) ;
#9397=CARTESIAN_POINT ( 'NONE',  ( -48.47912675150885065, -177.1207230881787780, 6.938893903907228378E-15 ) ) ;
#9399=ORIENTED_EDGE ( 'NONE', *, *, #10221, .T. ) ;
#9400=DIRECTION ( 'NONE',  ( 0.000000000000000000, 1.000000000000000000, 0.000000000000000000 ) ) ;
#9403=AXIS2_PLACEMENT_3D ( 'NONE', #37852, #20796, #5297 ) ;
#9404=VERTEX_POINT ( 'NONE', #23500 ) ;
#9405=EDGE_CURVE ( 'NONE', #42603, #23736, #35737, .T. ) ;
#9408=CARTESIAN_POINT ( 'NONE',  ( -151.4272465800706300, -177.1207230881787780, 70.89911581792885897 ) ) ;
#9409=LINE ( 'NONE', #26668, #39878 ) ;
#9410=VERTEX_POINT ( 'NONE', #51368 ) ;
#9414=EDGE_LOOP ( 'NONE', ( #49689, #23648, #33869, #7352 ) ) ;
#9415=DIRECTION ( 'NONE',  ( -0.9995608365087940150, 0.000000000000000000, -0.02963332782257007206 ) ) ;
#9416=ORIENTED_EDGE ( 'NONE', *, *, #2516, .T. ) ;
#9418=DIRECTION ( 'NONE',  ( 0.000000000000000000, 0.000000000000000000, -1.000000000000000000 ) ) ;
#9419=ORIENTED_EDGE ( 'NONE', *, *, #10706, .F. ) ;
#9422=VECTOR ( 'NONE', #6351, 1000.000000000000000 ) ;
#9425=AXIS2_PLACEMENT_3D ( 'NONE', #48238, #16178, #8023 ) ;
#9426=DIRECTION ( 'NONE',  ( 1.000000000000000000, 0.000000000000000000, -6.978251959525016136E-17 ) ) ;
#9427=AXIS2_PLACEMENT_3D ( 'NONE', #48452, #28191, #4288 ) ;
#9428=ADVANCED_FACE ( 'NONE', ( #31117 ), #11141, .T. ) ;
#9429=CARTESIAN_POINT ( 'NONE',  ( 67.64905612629584652, -183.6283474603465606, -43.47841891815124882 ) ) ;
#9430=CARTESIAN_POINT ( 'NONE',  ( -48.59739992243020623, -177.1207230881787780, -0.9929810960135115883 ) ) ;
#9432=CARTESIAN_POINT ( 'NONE',  ( 48.47907891923915713, -193.5000000000000000, 78.89300572996904748 ) ) ;
#9433=CARTESIAN_POINT ( 'NONE',  ( -108.5723883981723930, -177.1207230881787780, 109.6074810615846360 ) ) ;
#9437=CARTESIAN_POINT ( 'NONE',  ( -48.98765787015805984, -193.5000000000000000, -0.8610436117673551104 ) ) ;
#9438=LINE ( 'NONE', #4714, #24842 ) ;
#9440=VERTEX_POINT ( 'NONE', #7210 ) ;
#9441=AXIS2_PLACEMENT_3D ( 'NONE', #21773, #13367, #8638 ) ;
#9442=DIRECTION ( 'NONE',  ( 0.000000000000000000, 0.000000000000000000, 1.000000000000000000 ) ) ;
#9444=EDGE_LOOP ( 'NONE', ( #1456, #3063, #5912, #2097 ) ) ;
#9445=EDGE_LOOP ( 'NONE', ( #49110, #38253, #26388, #9719 ) ) ;
#9447=ORIENTED_EDGE ( 'NONE', *, *, #18087, .F. ) ;
#9449=DIRECTION ( 'NONE',  ( 0.000000000000000000, 0.000000000000000000, 1.000000000000000000 ) ) ;
#9450=LINE ( 'NONE', #4469, #34595 ) ;
#9451=DIRECTION ( 'NONE',  ( 0.000000000000000000, -1.000000000000000000, 0.000000000000000000 ) ) ;
#9453=DIRECTION ( 'NONE',  ( -0.4827922027307551267, 0.000000000000000000, 0.8757349421956311941 ) ) ;
#9456=CIRCLE ( 'NONE', #1040, 125.0000000000000000 ) ;
#9458=ADVANCED_FACE ( 'NONE', ( #31371 ), #47413, .T. ) ;
#9460=FACE_OUTER_BOUND ( 'NONE', #20499, .T. ) ;
#9461=VECTOR ( 'NONE', #26219, 1000.000000000000000 ) ;
#9463=ORIENTED_EDGE ( 'NONE', *, *, #2532, .F. ) ;
#9467=AXIS2_PLACEMENT_3D ( 'NONE', #6549, #42790, #2591 ) ;
#9468=EDGE_CURVE ( 'NONE', #47944, #46596, #38495, .T. ) ;
#9471=ORIENTED_EDGE ( 'NONE', *, *, #21164, .F. ) ;
#9472=DIRECTION ( 'NONE',  ( 0.000000000000000000, 0.000000000000000000, 1.000000000000000000 ) ) ;
#9474=ORIENTED_EDGE ( 'NONE', *, *, #33047, .F. ) ;
#9478=CARTESIAN_POINT ( 'NONE',  ( -47.64924157374594671, -175.3837268820161057, 124.9972451320097377 ) ) ;
#9479=AXIS2_PLACEMENT_3D ( 'NONE', #1730, #14874, #38749 ) ;
#9480=EDGE_LOOP ( 'NONE', ( #6824, #44894, #27882, #9917 ) ) ;
#9481=DIRECTION ( 'NONE',  ( 0.000000000000000000, 0.000000000000000000, -1.000000000000000000 ) ) ;
#9482=CARTESIAN_POINT ( 'NONE',  ( -160.2705093830644216, -183.6283474603465606, -55.92572546981521242 ) ) ;
#9484=ORIENTED_EDGE ( 'NONE', *, *, #43337, .F. ) ;
#9485=VERTEX_POINT ( 'NONE', #36351 ) ;
#9486=CIRCLE ( 'NONE', #22046, 125.0000000000000000 ) ;
#9488=DIRECTION ( 'NONE',  ( -0.9785564922995060311, 0.000000000000000000, 0.2059786187410889424 ) ) ;
#9491=ADVANCED_FACE ( 'NONE', ( #23753 ), #36881, .T. ) ;
#9492=DIRECTION ( 'NONE',  ( -0.5829794791144820021, 0.000000000000000000, 0.8124868780056742068 ) ) ;
#9494=DIRECTION ( 'NONE',  ( 0.000000000000000000, 0.000000000000000000, -1.000000000000000000 ) ) ;
#9495=DIRECTION ( 'NONE',  ( 0.000000000000000000, 0.000000000000000000, 1.000000000000000000 ) ) ;
#9496=AXIS2_PLACEMENT_3D ( 'NONE', #24423, #19965, #23893 ) ;
#9498=VECTOR ( 'NONE', #13055, 1000.000000000000227 ) ;
#9499=CARTESIAN_POINT ( 'NONE',  ( 73.50869128264334051, -183.6283474603465606, -22.25084316132034701 ) ) ;
#9502=CIRCLE ( 'NONE', #29627, 125.0000000000000000 ) ;
#9504=CARTESIAN_POINT ( 'NONE',  ( -49.45768324380835423, -193.5000000000000000, 0.2059786187410958813 ) ) ;
#9506=CARTESIAN_POINT ( 'NONE',  ( -151.9915035862630646, -193.5000000000000000, 70.07273251429430161 ) ) ;
#9507=AXIS2_PLACEMENT_3D ( 'NONE', #25921, #33554, #14109 ) ;
#9508=PLANE ( 'NONE',  #36342 ) ;
#9513=VECTOR ( 'NONE', #34440, 1000.000000000000114 ) ;
#9514=ORIENTED_EDGE ( 'NONE', *, *, #46911, .T. ) ;
#9516=EDGE_CURVE ( 'NONE', #34486, #46012, #4048, .T. ) ;
#9517=DIRECTION ( 'NONE',  ( 0.8455960035018272869, 0.000000000000000000, -0.5338233779647886257 ) ) ;
#9518=AXIS2_PLACEMENT_3D ( 'NONE', #43699, #12137, #4537 ) ;
#9519=CARTESIAN_POINT ( 'NONE',  ( 141.7825277784304205, -213.5000000000000000, 10.00000000000000178 ) ) ;
#9520=ORIENTED_EDGE ( 'NONE', *, *, #1622, .F. ) ;
#9521=ORIENTED_EDGE ( 'NONE', *, *, #28568, .F. ) ;
#9522=ORIENTED_EDGE ( 'NONE', *, *, #661, .F. ) ;
#9524=ADVANCED_FACE ( 'NONE', ( #36615 ), #7975, .F. ) ;
#9525=CARTESIAN_POINT ( 'NONE',  ( -4.176930889631405464, -175.3837268820161057, 116.8859077982279615 ) ) ;
#9526=FACE_OUTER_BOUND ( 'NONE', #48847, .T. ) ;
#9527=AXIS2_PLACEMENT_3D ( 'NONE', #21638, #37658, #49507 ) ;
#9528=ORIENTED_EDGE ( 'NONE', *, *, #29096, .T. ) ;
#9529=EDGE_CURVE ( 'NONE', #3419, #20713, #1382, .T. ) ;
#9530=DIRECTION ( 'NONE',  ( 0.000000000000000000, 1.000000000000000000, 0.000000000000000000 ) ) ;
#9531=DIRECTION ( 'NONE',  ( 0.000000000000000000, -0.000000000000000000, 1.000000000000000000 ) ) ;
#9534=EDGE_CURVE ( 'NONE', #18514, #4438, #16912, .T. ) ;
#9535=PLANE ( 'NONE',  #41507 ) ;
#9539=ORIENTED_EDGE ( 'NONE', *, *, #17297, .T. ) ;
#9540=CARTESIAN_POINT ( 'NONE',  ( -48.47912675150885065, -189.7472609257535510, 6.938893903907228378E-15 ) ) ;
#9541=DIRECTION ( 'NONE',  ( 0.8757349421956379665, 0.000000000000000000, -0.4827922027307427477 ) ) ;
#9542=DIRECTION ( 'NONE',  ( 0.000000000000000000, 1.000000000000000000, 0.000000000000000000 ) ) ;
#9543=ORIENTED_EDGE ( 'NONE', *, *, #5162, .F. ) ;
#9544=ORIENTED_EDGE ( 'NONE', *, *, #36762, .F. ) ;
#9545=DIRECTION ( 'NONE',  ( 0.000000000000000000, -1.000000000000000000, 0.000000000000000000 ) ) ;
#9546=CARTESIAN_POINT ( 'NONE',  ( -49.08592689732743963, -183.6283474603465606, -0.7948544414133539293 ) ) ;
#9548=DIRECTION ( 'NONE',  ( 0.000000000000000000, 0.000000000000000000, 1.000000000000000000 ) ) ;
#9551=DIRECTION ( 'NONE',  ( -0.000000000000000000, 1.000000000000000000, -0.000000000000000000 ) ) ;
#9553=VECTOR ( 'NONE', #2414, 1000.000000000000000 ) ;
#9556=VERTEX_POINT ( 'NONE', #24008 ) ;
#9557=FACE_OUTER_BOUND ( 'NONE', #31945, .T. ) ;
#9559=ORIENTED_EDGE ( 'NONE', *, *, #36762, .T. ) ;
#9561=DIRECTION ( 'NONE',  ( -0.000000000000000000, 1.000000000000000000, -0.000000000000000000 ) ) ;
#9563=AXIS2_PLACEMENT_3D ( 'NONE', #21488, #37768, #1240 ) ;
#9564=DIRECTION ( 'NONE',  ( 0.000000000000000000, 0.000000000000000000, -1.000000000000000000 ) ) ;
#9566=CARTESIAN_POINT ( 'NONE',  ( 75.67769207106684348, -177.1207230881787780, 14.49428645563876650 ) ) ;
#9567=ORIENTED_EDGE ( 'NONE', *, *, #2800, .F. ) ;
#9568=EDGE_CURVE ( 'NONE', #9092, #12643, #11910, .T. ) ;
#9569=ORIENTED_EDGE ( 'NONE', *, *, #27978, .F. ) ;
#9570=CARTESIAN_POINT ( 'NONE',  ( -48.47912675150885065, -175.3837268820161057, 6.938893903907228378E-15 ) ) ;
#9571=FACE_OUTER_BOUND ( 'NONE', #46588, .T. ) ;
#9572=VERTEX_POINT ( 'NONE', #16667 ) ;
#9573=EDGE_CURVE ( 'NONE', #10121, #33538, #44769, .T. ) ;
#9574=ORIENTED_EDGE ( 'NONE', *, *, #29160, .F. ) ;
#9577=ADVANCED_FACE ( 'NONE', ( #40541 ), #39757, .T. ) ;
#9578=EDGE_CURVE ( 'NONE', #1828, #22639, #4297, .T. ) ;
#9579=DIRECTION ( 'NONE',  ( -0.000000000000000000, 1.000000000000000000, -0.000000000000000000 ) ) ;
#9580=EDGE_LOOP ( 'NONE', ( #29487, #24304, #7581, #22511 ) ) ;
#9581=LINE ( 'NONE', #13525, #17219 ) ;
#9583=ORIENTED_EDGE ( 'NONE', *, *, #29374, .F. ) ;
#9584=DIRECTION ( 'NONE',  ( 0.5085311186492273983, 0.000000000000000000, -0.8610436117673514467 ) ) ;
#9585=DIRECTION ( 'NONE',  ( -0.000000000000000000, 1.000000000000000000, -0.000000000000000000 ) ) ;
#9586=AXIS2_PLACEMENT_3D ( 'NONE', #44589, #39348, #3353 ) ;
#9587=CIRCLE ( 'NONE', #22190, 125.0000000000000000 ) ;
#9589=CARTESIAN_POINT ( 'NONE',  ( -153.7737137892885073, -193.5000000000000000, -65.49088066501643368 ) ) ;
#9590=DIRECTION ( 'NONE',  ( -0.4566292373937200777, 0.000000000000000000, 0.8896570909947436601 ) ) ;
#9591=VERTEX_POINT ( 'NONE', #31893 ) ;
#9592=ORIENTED_EDGE ( 'NONE', *, *, #13850, .F. ) ;
#9593=AXIS2_PLACEMENT_3D ( 'NONE', #32759, #27519, #43555 ) ;
#9594=ADVANCED_FACE ( 'NONE', ( #40804 ), #24790, .T. ) ;
#9595=ORIENTED_EDGE ( 'NONE', *, *, #33546, .F. ) ;
#9596=DIRECTION ( 'NONE',  ( -0.000000000000000000, 1.000000000000000000, -0.000000000000000000 ) ) ;
#9597=DIRECTION ( 'NONE',  ( 0.9151456172430153524, 0.000000000000000000, 0.4031234292879792847 ) ) ;
#9598=EDGE_CURVE ( 'NONE', #8921, #33930, #43723, .T. ) ;
#9600=CARTESIAN_POINT ( 'NONE',  ( -77.03256798524175508, -189.7472609257535510, 121.6951149130964893 ) ) ;
#9601=VERTEX_POINT ( 'NONE', #41585 ) ;
#9603=CIRCLE ( 'NONE', #9637, 125.0000000000000000 ) ;
#9604=EDGE_CURVE ( 'NONE', #1758, #36353, #4765, .T. ) ;
#9605=ORIENTED_EDGE ( 'NONE', *, *, #3695, .F. ) ;
#9607=ORIENTED_EDGE ( 'NONE', *, *, #42109, .F. ) ;
#9608=ORIENTED_EDGE ( 'NONE', *, *, #16992, .T. ) ;
#9609=DIRECTION ( 'NONE',  ( -0.000000000000000000, 1.000000000000000000, -0.000000000000000000 ) ) ;
#9611=DIRECTION ( 'NONE',  ( 0.000000000000000000, 0.000000000000000000, 1.000000000000000000 ) ) ;
#9614=CARTESIAN_POINT ( 'NONE',  ( -48.47912675150885065, -183.6283474603465606, 6.938893903907228378E-15 ) ) ;
#9616=EDGE_CURVE ( 'NONE', #22071, #38204, #46080, .T. ) ;
#9618=CARTESIAN_POINT ( 'NONE',  ( -157.1522883217072604, -175.3837268820161057, 59.71720175837172206 ) ) ;
#9619=DIRECTION ( 'NONE',  ( 0.05924062789371441901, 0.000000000000000000, -0.9982437317643214625 ) ) ;
#9621=VECTOR ( 'NONE', #8176, 1000.000000000000000 ) ;
#9622=CIRCLE ( 'NONE', #45718, 125.0000000000000000 ) ;
#9623=DIRECTION ( 'NONE',  ( -1.000000000000000000, -0.000000000000000000, 4.884776371667511665E-16 ) ) ;
#9624=DIRECTION ( 'NONE',  ( -0.000000000000000000, 1.000000000000000000, -0.000000000000000000 ) ) ;
#9629=DIRECTION ( 'NONE',  ( 0.8124868780056783146, 0.000000000000000000, 0.5829794791144762289 ) ) ;
#9630=VERTEX_POINT ( 'NONE', #13743 ) ;
#9632=EDGE_LOOP ( 'NONE', ( #1543, #42137, #37905, #8270 ) ) ;
#9633=EDGE_CURVE ( 'NONE', #21582, #24818, #33710, .T. ) ;
#9637=AXIS2_PLACEMENT_3D ( 'NONE', #50583, #14583, #10631 ) ;
#9639=EDGE_CURVE ( 'NONE', #27923, #895, #45038, .T. ) ;
#9640=ADVANCED_FACE ( 'NONE', ( #17170 ), #13229, .T. ) ;
#9642=DIRECTION ( 'NONE',  ( -0.000000000000000000, -1.000000000000000000, 0.000000000000000000 ) ) ;
#9645=DIRECTION ( 'NONE',  ( -0.8757349421956345248, 0.000000000000000000, -0.4827922027307490205 ) ) ;
#9647=ORIENTED_EDGE ( 'NONE', *, *, #13325, .T. ) ;
#9648=ORIENTED_EDGE ( 'NONE', *, *, #29663, .F. ) ;
#9649=CARTESIAN_POINT ( 'NONE',  ( -48.41988612361515010, -175.3837268820161057, 0.9982437317643287900 ) ) ;
#9650=FACE_OUTER_BOUND ( 'NONE', #7883, .T. ) ;
#9655=VECTOR ( 'NONE', #43480, 1000.000000000000000 ) ;
#9657=CARTESIAN_POINT ( 'NONE',  ( -141.2664123866436512, -189.7472609257535510, -83.75869879877495805 ) ) ;
#9658=VERTEX_POINT ( 'NONE', #5875 ) ;
#9659=VECTOR ( 'NONE', #19389, 1000.000000000000000 ) ;
#9660=EDGE_CURVE ( 'NONE', #16711, #29476, #22147, .T. ) ;
#9662=DIRECTION ( 'NONE',  ( 0.000000000000000000, 0.000000000000000000, -1.000000000000000000 ) ) ;
#9664=DIRECTION ( 'NONE',  ( 0.1768902751225666370, 0.000000000000000000, 0.9842305779475979399 ) ) ;
#9665=VERTEX_POINT ( 'NONE', #49752 ) ;
#9666=VERTEX_POINT ( 'NONE', #28972 ) ;
#9669=CARTESIAN_POINT ( 'NONE',  ( 76.52053249983501360, -183.6283474603465606, -0.2918682030015273265 ) ) ;
#9675=ORIENTED_EDGE ( 'NONE', *, *, #50392, .F. ) ;
#9676=CARTESIAN_POINT ( 'NONE',  ( -48.47912675150885065, -177.1207230881787780, 6.938893903907228378E-15 ) ) ;
#9678=VERTEX_POINT ( 'NONE', #17448 ) ;
#9681=CARTESIAN_POINT ( 'NONE',  ( 75.78974234412359579, -193.5000000000000000, 13.49993235881449394 ) ) ;
#9682=CARTESIAN_POINT ( 'NONE',  ( -155.4121128832437364, -183.6283474603465606, -62.78108192021942813 ) ) ;
#9684=DIRECTION ( 'NONE',  ( 0.000000000000000000, -1.000000000000000000, 0.000000000000000000 ) ) ;
#9685=VERTEX_POINT ( 'NONE', #37912 ) ;
#9686=DIRECTION ( 'NONE',  ( -0.000000000000000000, 1.000000000000000000, -0.000000000000000000 ) ) ;
#9687=CARTESIAN_POINT ( 'NONE',  ( 51.78320179844649118, -175.3837268820161057, -72.96212019587142095 ) ) ;
#9690=LINE ( 'NONE', #25718, #36306 ) ;
#9691=ORIENTED_EDGE ( 'NONE', *, *, #27934, .T. ) ;
#9693=CYLINDRICAL_SURFACE ( 'NONE', #32369, 125.0000000000000000 ) ;
#9694=CARTESIAN_POINT ( 'NONE',  ( -48.47912675150885065, -189.7472609257535510, 6.938893903907228378E-15 ) ) ;
#9695=EDGE_LOOP ( 'NONE', ( #33515, #5351, #11078, #37850 ) ) ;
#9696=EDGE_LOOP ( 'NONE', ( #49892, #26792, #6641, #12551 ) ) ;
#9697=VECTOR ( 'NONE', #11620, 999.9999999999998863 ) ;
#9698=AXIS2_PLACEMENT_3D ( 'NONE', #9034, #41589, #9293 ) ;
#9700=CARTESIAN_POINT ( 'NONE',  ( 64.29733702426837283, -193.5000000000000000, 53.91167979418564471 ) ) ;
#9704=EDGE_CURVE ( 'NONE', #885, #32675, #17951, .T. ) ;
#9705=DIRECTION ( 'NONE',  ( 0.000000000000000000, 0.000000000000000000, 1.000000000000000000 ) ) ;
#9706=ORIENTED_EDGE ( 'NONE', *, *, #19143, .T. ) ;
#9708=AXIS2_PLACEMENT_3D ( 'NONE', #18833, #43011, #14917 ) ;
#9709=CARTESIAN_POINT ( 'NONE',  ( -85.48706473349324142, -175.3837268820161057, -118.3487137068146637 ) ) ;
#9711=CARTESIAN_POINT ( 'NONE',  ( 76.28370911321319170, -177.1207230881787780, -7.696413904697508634 ) ) ;
#9713=CARTESIAN_POINT ( 'NONE',  ( -48.47912675150885065, -183.6283474603465606, 6.938893903907228378E-15 ) ) ;
#9714=EDGE_LOOP ( 'NONE', ( #44688, #36971, #15457, #40672 ) ) ;
#9715=CARTESIAN_POINT ( 'NONE',  ( -124.4642912599203726, -193.5000000000000000, 99.25348746834863789 ) ) ;
#9717=AXIS2_PLACEMENT_3D ( 'NONE', #1246, #17303, #41450 ) ;
#9718=CARTESIAN_POINT ( 'NONE',  ( -78.00521078983979351, -175.3837268820161057, 121.4627941443857111 ) ) ;
#9719=ORIENTED_EDGE ( 'NONE', *, *, #51956, .T. ) ;
#9721=DIRECTION ( 'NONE',  ( 0.000000000000000000, 0.000000000000000000, -1.000000000000000000 ) ) ;
#9722=ORIENTED_EDGE ( 'NONE', *, *, #26254, .F. ) ;
#9723=ADVANCED_FACE ( 'NONE', ( #33960 ), #41073, .T. ) ;
#9724=DIRECTION ( 'NONE',  ( 0.6068001458185834363, 0.000000000000000000, 0.7948544414133608127 ) ) ;
#9729=ORIENTED_EDGE ( 'NONE', *, *, #13010, .F. ) ;
#9730=AXIS2_PLACEMENT_3D ( 'NONE', #8649, #48873, #36775 ) ;
#9731=PLANE ( 'NONE',  #16392 ) ;
#9732=VECTOR ( 'NONE', #2105, 1000.000000000000227 ) ;
#9734=LINE ( 'NONE', #29182, #28051 ) ;
#9736=AXIS2_PLACEMENT_3D ( 'NONE', #12851, #28875, #4992 ) ;
#9738=DIRECTION ( 'NONE',  ( -0.000000000000000000, 1.000000000000000000, -0.000000000000000000 ) ) ;
#9740=PLANE ( 'NONE',  #37569 ) ;
#9741=ORIENTED_EDGE ( 'NONE', *, *, #9660, .F. ) ;
#9742=ORIENTED_EDGE ( 'NONE', *, *, #15996, .F. ) ;
#9743=DIRECTION ( 'NONE',  ( -0.2059786187411094538, 0.000000000000000000, 0.9785564922995017012 ) ) ;
#9744=PLANE ( 'NONE',  #8558 ) ;
#9746=VERTEX_POINT ( 'NONE', #11076 ) ;
#9747=AXIS2_PLACEMENT_3D ( 'NONE', #48126, #12893, #8696 ) ;
#9750=CARTESIAN_POINT ( 'NONE',  ( -173.4787860028527007, -177.1207230881787780, 0.2918682030023981300 ) ) ;
#9751=AXIS2_PLACEMENT_3D ( 'NONE', #43741, #39531, #32172 ) ;
#9752=FACE_OUTER_BOUND ( 'NONE', #42762, .T. ) ;
#9755=CIRCLE ( 'NONE', #39101, 125.0000000000000000 ) ;
#9756=DIRECTION ( 'NONE',  ( -0.6068001458185834363, 0.000000000000000000, -0.7948544414133608127 ) ) ;
#9757=DIRECTION ( 'NONE',  ( 0.000000000000000000, -1.000000000000000000, 0.000000000000000000 ) ) ;
#9759=VECTOR ( 'NONE', #10635, 1000.000000000000114 ) ;
#9760=CARTESIAN_POINT ( 'NONE',  ( -48.47912675150885065, -189.7472609257535510, 6.938893903907228378E-15 ) ) ;
#9762=CARTESIAN_POINT ( 'NONE',  ( -29.73468717939733708, -183.6283474603465606, 123.5865930638411214 ) ) ;
#9764=LINE ( 'NONE', #34447, #5062 ) ;
#9765=ADVANCED_FACE ( 'NONE', ( #47354 ), #6384, .F. ) ;
#9767=ADVANCED_FACE ( 'NONE', ( #46850 ), #14526, .T. ) ;
#9768=CIRCLE ( 'NONE', #34111, 125.0000000000000000 ) ;
#9769=AXIS2_PLACEMENT_3D ( 'NONE', #27517, #3600, #35143 ) ;
#9770=CARTESIAN_POINT ( 'NONE',  ( 70.68712318874649725, -183.6283474603465606, -37.74128873232327663 ) ) ;
#9771=LINE ( 'NONE', #48684, #22834 ) ;
#9773=EDGE_LOOP ( 'NONE', ( #6767, #30032, #25661, #50425 ) ) ;
#9774=VERTEX_POINT ( 'NONE', #18979 ) ;
#9775=CARTESIAN_POINT ( 'NONE',  ( -154.2693405752510500, -175.3837268820161057, 66.58401203837830451 ) ) ;
#9778=ORIENTED_EDGE ( 'NONE', *, *, #28211, .T. ) ;
#9779=VECTOR ( 'NONE', #27698, 1000.000000000000000 ) ;
#9780=ORIENTED_EDGE ( 'NONE', *, *, #47286, .F. ) ;
#9782=VERTEX_POINT ( 'NONE', #22666 ) ;
#9784=LINE ( 'NONE', #29480, #9101 ) ;
#9785=AXIS2_PLACEMENT_3D ( 'NONE', #25916, #37224, #1214 ) ;
#9786=AXIS2_PLACEMENT_3D ( 'NONE', #27964, #42242, #35855 ) ;
#9787=LINE ( 'NONE', #37374, #19395 ) ;
#9788=AXIS2_PLACEMENT_3D ( 'NONE', #23800, #19348, #15414 ) ;
#9789=DIRECTION ( 'NONE',  ( 0.000000000000000000, -0.000000000000000000, 1.000000000000000000 ) ) ;
#9790=ORIENTED_EDGE ( 'NONE', *, *, #8849, .T. ) ;
#9792=DIRECTION ( 'NONE',  ( -0.000000000000000000, 1.000000000000000000, 0.000000000000000000 ) ) ;
#9794=ORIENTED_EDGE ( 'NONE', *, *, #48323, .F. ) ;
#9796=DIRECTION ( 'NONE',  ( 0.000000000000000000, 0.000000000000000000, 1.000000000000000000 ) ) ;
#9800=CARTESIAN_POINT ( 'NONE',  ( 74.31448861501726810, -183.6283474603465606, -23.38221600314288651 ) ) ;
#9801=LINE ( 'NONE', #26598, #33868 ) ;
#9803=ORIENTED_EDGE ( 'NONE', *, *, #48887, .F. ) ;
#9804=VECTOR ( 'NONE', #7500, 1000.000000000000114 ) ;
#9808=CARTESIAN_POINT ( 'NONE',  ( -169.3144491972411458, -177.1207230881787780, -27.83926365844663664 ) ) ;
#9809=ORIENTED_EDGE ( 'NONE', *, *, #51347, .T. ) ;
#9810=CARTESIAN_POINT ( 'NONE',  ( -70.58093260035830951, -189.7472609257535510, 122.0143860769388908 ) ) ;
#9811=VECTOR ( 'NONE', #10610, 1000.000000000000114 ) ;
#9816=ORIENTED_EDGE ( 'NONE', *, *, #25590, .T. ) ;
#9818=EDGE_LOOP ( 'NONE', ( #49940, #12789, #23230, #912 ) ) ;
#9819=VECTOR ( 'NONE', #15834, 1000.000000000000114 ) ;
#9822=PLANE ( 'NONE',  #43793 ) ;
#9823=EDGE_LOOP ( 'NONE', ( #13671, #26887, #46861, #19077 ) ) ;
#9824=AXIS2_PLACEMENT_3D ( 'NONE', #7655, #2437, #47352 ) ;
#9825=CIRCLE ( 'NONE', #4802, 125.0000000000000000 ) ;
#9826=CARTESIAN_POINT ( 'NONE',  ( -48.47912675150885065, -175.3837268820161057, 6.938893903907228378E-15 ) ) ;
#9829=EDGE_CURVE ( 'NONE', #12249, #46797, #6889, .T. ) ;
#9830=AXIS2_PLACEMENT_3D ( 'NONE', #23949, #40488, #36551 ) ;
#9831=CARTESIAN_POINT ( 'NONE',  ( -41.24387117724851493, -175.3837268820161057, 124.7904286264581231 ) ) ;
#9832=ADVANCED_FACE ( 'NONE', ( #43414 ), #10316, .T. ) ;
#9833=ORIENTED_EDGE ( 'NONE', *, *, #28832, .T. ) ;
#9835=AXIS2_PLACEMENT_3D ( 'NONE', #1329, #29967, #1063 ) ;
#9836=ORIENTED_EDGE ( 'NONE', *, *, #34328, .T. ) ;
#9839=LINE ( 'NONE', #6160, #28676 ) ;
#9840=ORIENTED_EDGE ( 'NONE', *, *, #45895, .T. ) ;
#9843=AXIS2_PLACEMENT_3D ( 'NONE', #20135, #27753, #48258 ) ;
#9845=ORIENTED_EDGE ( 'NONE', *, *, #16746, .T. ) ;
#9846=DIRECTION ( 'NONE',  ( 0.000000000000000000, 0.000000000000000000, 1.000000000000000000 ) ) ;
#9847=EDGE_LOOP ( 'NONE', ( #20899, #23804, #1109, #49467 ) ) ;
#9849=LINE ( 'NONE', #1702, #36742 ) ;
#9851=CARTESIAN_POINT ( 'NONE',  ( -48.47912675150885065, -189.7472609257535510, 6.938893903907228378E-15 ) ) ;
#9853=VERTEX_POINT ( 'NONE', #26599 ) ;
#9855=ORIENTED_EDGE ( 'NONE', *, *, #32706, .T. ) ;
#9856=CARTESIAN_POINT ( 'NONE',  ( -133.8011377042516301, -177.1207230881787780, -91.35181687837437892 ) ) ;
#9857=LINE ( 'NONE', #25881, #35236 ) ;
#9858=AXIS2_PLACEMENT_3D ( 'NONE', #18515, #30583, #46642 ) ;
#9860=AXIS2_PLACEMENT_3D ( 'NONE', #10959, #15174, #24857 ) ;
#9863=ORIENTED_EDGE ( 'NONE', *, *, #30162, .F. ) ;
#9866=VERTEX_POINT ( 'NONE', #38932 ) ;
#9868=VERTEX_POINT ( 'NONE', #31308 ) ;
#9869=ORIENTED_EDGE ( 'NONE', *, *, #47522, .T. ) ;
#9870=CARTESIAN_POINT ( 'NONE',  ( -173.4190745413846457, -175.3837268820161057, -3.874202661594927211 ) ) ;
#9871=PLANE ( 'NONE',  #51849 ) ;
#9872=EDGE_CURVE ( 'NONE', #14916, #48059, #3064, .T. ) ;
#9874=EDGE_CURVE ( 'NONE', #9242, #14212, #47578, .T. ) ;
#9875=ADVANCED_FACE ( 'NONE', ( #19242 ), #38432, .T. ) ;
#9877=VERTEX_POINT ( 'NONE', #35504 ) ;
#9878=DIRECTION ( 'NONE',  ( -0.000000000000000000, -1.000000000000000000, 0.000000000000000000 ) ) ;
#9880=EDGE_CURVE ( 'NONE', #41928, #25092, #36648, .T. ) ;
#9881=ORIENTED_EDGE ( 'NONE', *, *, #13872, .T. ) ;
#9882=CARTESIAN_POINT ( 'NONE',  ( -62.43888699632653783, -175.3837268820161057, 124.2180546213279371 ) ) ;
#9883=CIRCLE ( 'NONE', #30020, 125.0000000000000000 ) ;
#9885=ADVANCED_FACE ( 'NONE', ( #2680 ), #18720, .T. ) ;
#9888=EDGE_CURVE ( 'NONE', #13637, #1466, #51552, .T. ) ;
#9889=CIRCLE ( 'NONE', #19153, 125.0000000000000000 ) ;
#9892=FACE_OUTER_BOUND ( 'NONE', #50399, .T. ) ;
#9893=EDGE_CURVE ( 'NONE', #35294, #26421, #45071, .T. ) ;
#9895=EDGE_CURVE ( 'NONE', #9685, #23874, #43370, .T. ) ;
#9896=DIRECTION ( 'NONE',  ( 0.000000000000000000, 1.000000000000000000, 0.000000000000000000 ) ) ;
#9897=FACE_BOUND ( 'NONE', #19852, .T. ) ;
#9898=ADVANCED_FACE ( 'NONE', ( #20006 ), #543, .F. ) ;
#9900=AXIS2_PLACEMENT_3D ( 'NONE', #33509, #913, #9584 ) ;
#9905=ORIENTED_EDGE ( 'NONE', *, *, #22043, .T. ) ;
#9906=DIRECTION ( 'NONE',  ( 0.9266896074318291543, 0.000000000000000000, 0.3758275821142488260 ) ) ;
#9909=DIRECTION ( 'NONE',  ( 0.000000000000000000, 1.000000000000000000, 0.000000000000000000 ) ) ;
#9910=DIRECTION ( 'NONE',  ( 0.000000000000000000, 0.000000000000000000, 1.000000000000000000 ) ) ;
#9911=LINE ( 'NONE', #25926, #6978 ) ;
#9912=VERTEX_POINT ( 'NONE', #32085 ) ;
#9914=CARTESIAN_POINT ( 'NONE',  ( -2.700932609314997457, -177.1207230881787780, -116.3157639405751809 ) ) ;
#9917=ORIENTED_EDGE ( 'NONE', *, *, #31161, .T. ) ;
#9918=EDGE_LOOP ( 'NONE', ( #32684, #50827, #24457, #11066 ) ) ;
#9919=DIRECTION ( 'NONE',  ( -0.000000000000000000, 1.000000000000000000, -0.000000000000000000 ) ) ;
#9920=AXIS2_PLACEMENT_3D ( 'NONE', #1400, #8756, #17706 ) ;
#9923=DIRECTION ( 'NONE',  ( -0.000000000000000000, 1.000000000000000000, -0.000000000000000000 ) ) ;
#9924=DIRECTION ( 'NONE',  ( -0.000000000000000000, 1.000000000000000000, -0.000000000000000000 ) ) ;
#9925=DIRECTION ( 'NONE',  ( 0.9266896074318343723, 0.000000000000000000, -0.3758275821142357809 ) ) ;
#9926=ORIENTED_EDGE ( 'NONE', *, *, #48142, .T. ) ;
#9927=DIRECTION ( 'NONE',  ( 0.7378332790417239107, 0.000000000000000000, 0.6749830015182142207 ) ) ;
#9928=EDGE_CURVE ( 'NONE', #4219, #27267, #47876, .T. ) ;
#9930=DIRECTION ( 'NONE',  ( -0.6965510290630033685, 0.000000000000000000, 0.7175072570443249420 ) ) ;
#9931=VERTEX_POINT ( 'NONE', #28399 ) ;
#9932=AXIS2_PLACEMENT_3D ( 'NONE', #6294, #49153, #25484 ) ;
#9933=VERTEX_POINT ( 'NONE', #40741 ) ;
#9934=ORIENTED_EDGE ( 'NONE', *, *, #3598, .T. ) ;
#9935=LINE ( 'NONE', #18838, #11533 ) ;
#9936=LINE ( 'NONE', #51374, #36498 ) ;
#9937=ORIENTED_EDGE ( 'NONE', *, *, #33060, .T. ) ;
#9938=EDGE_CURVE ( 'NONE', #30058, #10177, #3900, .T. ) ;
#9939=EDGE_CURVE ( 'NONE', #5079, #3221, #36035, .T. ) ;
#9941=ADVANCED_FACE ( 'NONE', ( #31568 ), #20260, .T. ) ;
#9943=FACE_OUTER_BOUND ( 'NONE', #41355, .T. ) ;
#9944=EDGE_LOOP ( 'NONE', ( #27550, #19519, #2572, #7327 ) ) ;
#9945=FACE_OUTER_BOUND ( 'NONE', #43815, .T. ) ;
#9946=ORIENTED_EDGE ( 'NONE', *, *, #40048, .F. ) ;
#9949=ORIENTED_EDGE ( 'NONE', *, *, #3980, .F. ) ;
#9951=LINE ( 'NONE', #14157, #25586 ) ;
#9952=EDGE_CURVE ( 'NONE', #8894, #14662, #11606, .T. ) ;
#9954=LINE ( 'NONE', #1272, #29086 ) ;
#9955=EDGE_LOOP ( 'NONE', ( #36006, #32432, #20944, #38901 ) ) ;
#9956=PLANE ( 'NONE',  #13103 ) ;
#9958=DIRECTION ( 'NONE',  ( -0.000000000000000000, 1.000000000000000000, -0.000000000000000000 ) ) ;
#9959=CARTESIAN_POINT ( 'NONE',  ( 48.69345348225014192, -189.7472609257535510, -78.62880929222870918 ) ) ;
#9961=ORIENTED_EDGE ( 'NONE', *, *, #36828, .T. ) ;
#9962=PLANE ( 'NONE',  #51526 ) ;
#9965=CARTESIAN_POINT ( 'NONE',  ( -155.4121128832437364, -193.5000000000000000, -62.78108192021939971 ) ) ;
#9967=ORIENTED_EDGE ( 'NONE', *, *, #24844, .F. ) ;
#9968=VECTOR ( 'NONE', #17962, 1000.000000000000114 ) ;
#9971=CYLINDRICAL_SURFACE ( 'NONE', #20568, 125.0000000000000000 ) ;
#9972=VECTOR ( 'NONE', #6567, 1000.000000000000000 ) ;
#9975=DIRECTION ( 'NONE',  ( 0.000000000000000000, 0.000000000000000000, 1.000000000000000000 ) ) ;
#9977=LINE ( 'NONE', #13643, #44730 ) ;
#9978=ORIENTED_EDGE ( 'NONE', *, *, #20866, .T. ) ;
#9980=VECTOR ( 'NONE', #10945, 1000.000000000000114 ) ;
#9981=DIRECTION ( 'NONE',  ( 0.000000000000000000, 1.000000000000000000, 0.000000000000000000 ) ) ;
#9983=CARTESIAN_POINT ( 'NONE',  ( -48.47912675150885065, -189.7472609257535510, 6.938893903907228378E-15 ) ) ;
#9986=ORIENTED_EDGE ( 'NONE', *, *, #23100, .T. ) ;
#9987=VECTOR ( 'NONE', #4628, 1000.000000000000000 ) ;
#9988=DIRECTION ( 'NONE',  ( 0.000000000000000000, 1.000000000000000000, 0.000000000000000000 ) ) ;
#9989=EDGE_CURVE ( 'NONE', #42327, #1307, #50133, .T. ) ;
#9990=ORIENTED_EDGE ( 'NONE', *, *, #47852, .F. ) ;
#9991=DIRECTION ( 'NONE',  ( -0.000000000000000000, 1.000000000000000000, -0.000000000000000000 ) ) ;
#9995=LINE ( 'NONE', #17872, #36523 ) ;
#9996=ORIENTED_EDGE ( 'NONE', *, *, #37697, .T. ) ;
#9999=ORIENTED_EDGE ( 'NONE', *, *, #44612, .T. ) ;
#10001=PLANE ( 'NONE',  #1302 ) ;
#10002=EDGE_LOOP ( 'NONE', ( #13414, #17926, #29895, #20660 ) ) ;
#10004=AXIS2_PLACEMENT_3D ( 'NONE', #45471, #25487, #24710 ) ;
#10006=EDGE_CURVE ( 'NONE', #20725, #46128, #29438, .T. ) ;
#10007=EDGE_CURVE ( 'NONE', #13237, #4441, #49447, .T. ) ;
#10008=FACE_OUTER_BOUND ( 'NONE', #31019, .T. ) ;
#10009=CARTESIAN_POINT ( 'NONE',  ( -164.8312043469690593, -177.1207230881787780, -42.87565520599202529 ) ) ;
#10011=ORIENTED_EDGE ( 'NONE', *, *, #39163, .F. ) ;
#10012=ORIENTED_EDGE ( 'NONE', *, *, #3995, .T. ) ;
#10013=AXIS2_PLACEMENT_3D ( 'NONE', #27473, #35355, #10676 ) ;
#10014=CARTESIAN_POINT ( 'NONE',  ( -168.1141659785444915, -183.6283474603465606, -36.22785377503947046 ) ) ;
#10015=ORIENTED_EDGE ( 'NONE', *, *, #32402, .T. ) ;
#10016=CARTESIAN_POINT ( 'NONE',  ( 54.54686566053560881, -183.6283474603465606, 69.00559874123592863 ) ) ;
#10017=DIRECTION ( 'NONE',  ( -0.000000000000000000, 1.000000000000000000, -0.000000000000000000 ) ) ;
#10018=EDGE_LOOP ( 'NONE', ( #44712, #44178, #28716, #50511 ) ) ;
#10020=FACE_OUTER_BOUND ( 'NONE', #26093, .T. ) ;
#10021=CARTESIAN_POINT ( 'NONE',  ( -114.9600645115007040, -177.1207230881787780, 105.8550183720738431 ) ) ;
#10022=DIRECTION ( 'NONE',  ( 0.000000000000000000, 0.000000000000000000, -1.000000000000000000 ) ) ;
#10023=DIRECTION ( 'NONE',  ( 0.000000000000000000, 0.000000000000000000, 1.000000000000000000 ) ) ;
#10024=ORIENTED_EDGE ( 'NONE', *, *, #17021, .F. ) ;
#10026=CARTESIAN_POINT ( 'NONE',  ( -169.2746641285359317, -193.5000000000000000, -32.14713283941905786 ) ) ;
#10028=DIRECTION ( 'NONE',  ( 0.9646355819083576311, 0.000000000000000000, 0.2635871660690715101 ) ) ;
#10029=VERTEX_POINT ( 'NONE', #33407 ) ;
#10030=CARTESIAN_POINT ( 'NONE',  ( 6.443011874827243801, -193.5000000000000000, 112.2878385610370771 ) ) ;
#10033=CARTESIAN_POINT ( 'NONE',  ( 3.652658254809380445, -193.5000000000000000, -112.5098962032389522 ) ) ;
#10034=CARTESIAN_POINT ( 'NONE',  ( 75.51463005422468200, -183.6283474603465606, -1.322128892811231360 ) ) ;
#10038=LINE ( 'NONE', #2129, #5214 ) ;
#10039=FACE_OUTER_BOUND ( 'NONE', #43050, .T. ) ;
#10040=CARTESIAN_POINT ( 'NONE',  ( -6.081033889300858419, -189.7472609257535510, -116.5264228893325651 ) ) ;
#10041=STYLED_ITEM ( 'NONE', ( #34349 ), #35805 ) ;
#10043=CARTESIAN_POINT ( 'NONE',  ( 1.150725574412429175, -175.3837268820161057, -114.7252272087845739 ) ) ;
#10044=LINE ( 'NONE', #6104, #10373 ) ;
#10045=DIRECTION ( 'NONE',  ( 1.000000000000000000, 0.000000000000000000, 6.978251959525016136E-17 ) ) ;
#10047=VERTEX_POINT ( 'NONE', #10009 ) ;
#10048=EDGE_LOOP ( 'NONE', ( #19144, #51750, #6923, #5788 ) ) ;
#10049=DIRECTION ( 'NONE',  ( -0.8757349421956379665, 0.000000000000000000, 0.4827922027307427477 ) ) ;
#10050=CARTESIAN_POINT ( 'NONE',  ( -47.70260288879080690, -193.5000000000000000, -0.6300878435817026668 ) ) ;
#10051=CYLINDRICAL_SURFACE ( 'NONE', #24675, 125.0000000000000000 ) ;
#10055=CARTESIAN_POINT ( 'NONE',  ( 20.10322172534453244, -189.7472609257535510, -103.3076327631962954 ) ) ;
#10057=ORIENTED_EDGE ( 'NONE', *, *, #13683, .T. ) ;
#10059=VERTEX_POINT ( 'NONE', #13420 ) ;
#10061=ORIENTED_EDGE ( 'NONE', *, *, #4135, .T. ) ;
#10063=DIRECTION ( 'NONE',  ( -0.6068001458185890984, 0.000000000000000000, -0.7948544414133565938 ) ) ;
#10066=ORIENTED_EDGE ( 'NONE', *, *, #40048, .T. ) ;
#10067=EDGE_LOOP ( 'NONE', ( #22010, #32577, #19119, #35112 ) ) ;
#10069=DIRECTION ( 'NONE',  ( 0.2059786187410889424, 0.000000000000000000, 0.9785564922995060311 ) ) ;
#10070=CIRCLE ( 'NONE', #2521, 125.0000000000000000 ) ;
#10071=EDGE_LOOP ( 'NONE', ( #12466, #40388 ) ) ;
#10072=LINE ( 'NONE', #38166, #8203 ) ;
#10073=ORIENTED_EDGE ( 'NONE', *, *, #12722, .F. ) ;
#10074=CARTESIAN_POINT ( 'NONE',  ( -149.3265790242249125, -175.3837268820161057, 72.15117186584559761 ) ) ;
#10075=CARTESIAN_POINT ( 'NONE',  ( -48.47912675150885065, -183.6283474603465606, 6.938893903907228378E-15 ) ) ;
#10077=CARTESIAN_POINT ( 'NONE',  ( -132.6364218684650211, -177.1207230881787780, 92.42591454022807795 ) ) ;
#10079=DIRECTION ( 'NONE',  ( -0.9890401873221654760, 0.000000000000000000, 0.1476465640024710868 ) ) ;
#10080=FACE_OUTER_BOUND ( 'NONE', #5909, .T. ) ;
#10081=PLANE ( 'NONE',  #8453 ) ;
#10084=LINE ( 'NONE', #26099, #33607 ) ;
#10085=CARTESIAN_POINT ( 'NONE',  ( -124.1938582159088043, -189.7472609257535510, -99.45993886622794378 ) ) ;
#10086=CARTESIAN_POINT ( 'NONE',  ( -49.03777351731250889, -193.5000000000000000, 0.8294056854502042109 ) ) ;
#10088=ORIENTED_EDGE ( 'NONE', *, *, #30159, .F. ) ;
#10089=AXIS2_PLACEMENT_3D ( 'NONE', #38709, #50816, #14823 ) ;
#10092=FACE_OUTER_BOUND ( 'NONE', #29113, .T. ) ;
#10094=EDGE_LOOP ( 'NONE', ( #15296, #6686, #45387, #7262 ) ) ;
#10095=ORIENTED_EDGE ( 'NONE', *, *, #42716, .T. ) ;
#10096=CARTESIAN_POINT ( 'NONE',  ( 61.06976976088564157, -175.3837268820161057, -60.19999396110172540 ) ) ;
#10098=VERTEX_POINT ( 'NONE', #9482 ) ;
#10099=AXIS2_PLACEMENT_3D ( 'NONE', #17551, #46179, #26177 ) ;
#10100=CARTESIAN_POINT ( 'NONE',  ( -165.6791976657750354, -175.3837268820161057, 40.49875167739065773 ) ) ;
#10101=ORIENTED_EDGE ( 'NONE', *, *, #35030, .F. ) ;
#10103=CARTESIAN_POINT ( 'NONE',  ( -80.85382946868864451, -177.1207230881787780, 119.6996507684852844 ) ) ;
#10104=EDGE_CURVE ( 'NONE', #9678, #20898, #19061, .T. ) ;
#10107=ORIENTED_EDGE ( 'NONE', *, *, #6643, .F. ) ;
#10108=ORIENTED_EDGE ( 'NONE', *, *, #47440, .T. ) ;
#10111=DIRECTION ( 'NONE',  ( 0.000000000000000000, -1.000000000000000000, 0.000000000000000000 ) ) ;
#10112=DIRECTION ( 'NONE',  ( 0.000000000000000000, 0.000000000000000000, 1.000000000000000000 ) ) ;
#10113=CARTESIAN_POINT ( 'NONE',  ( -48.47912675150885065, -189.7472609257535510, 6.938893903907228378E-15 ) ) ;
#10117=CARTESIAN_POINT ( 'NONE',  ( -152.8713435144644848, -193.5000000000000000, -68.75510947788595217 ) ) ;
#10118=EDGE_CURVE ( 'NONE', #10459, #24955, #21307, .T. ) ;
#10119=AXIS2_PLACEMENT_3D ( 'NONE', #19231, #35239, #23172 ) ;
#10121=VERTEX_POINT ( 'NONE', #16858 ) ;
#10123=VERTEX_POINT ( 'NONE', #37066 ) ;
#10125=EDGE_CURVE ( 'NONE', #14296, #20982, #45489, .T. ) ;
#10126=CARTESIAN_POINT ( 'NONE',  ( -95.72791768350688812, -177.1207230881787780, -115.7261930397105232 ) ) ;
#10127=CARTESIAN_POINT ( 'NONE',  ( -23.01747912075237679, -183.6283474603465606, -122.3793467049370776 ) ) ;
#10130=VERTEX_POINT ( 'NONE', #28914 ) ;
#10131=FACE_OUTER_BOUND ( 'NONE', #35293, .T. ) ;
#10132=VERTEX_POINT ( 'NONE', #41521 ) ;
#10133=VERTEX_POINT ( 'NONE', #1603 ) ;
#10134=FACE_OUTER_BOUND ( 'NONE', #39211, .T. ) ;
#10135=PLANE ( 'NONE',  #11861 ) ;
#10137=ORIENTED_EDGE ( 'NONE', *, *, #13166, .F. ) ;
#10138=CARTESIAN_POINT ( 'NONE',  ( -103.4012653778457462, -183.6283474603465606, -112.2878385610366649 ) ) ;
#10139=CARTESIAN_POINT ( 'NONE',  ( -18.31235070009513777, -175.3837268820161057, 121.3052580173829824 ) ) ;
#10142=CARTESIAN_POINT ( 'NONE',  ( 75.43907105790114542, -175.3837268820161057, -4.503971736580769658 ) ) ;
#10143=ORIENTED_EDGE ( 'NONE', *, *, #28179, .F. ) ;
#10144=CARTESIAN_POINT ( 'NONE',  ( 38.71172987070728055, -175.3837268820161057, -89.56983042009262874 ) ) ;
#10145=VERTEX_POINT ( 'NONE', #41801 ) ;
#10147=VERTEX_POINT ( 'NONE', #21047 ) ;
#10148=CARTESIAN_POINT ( 'NONE',  ( 49.27559354810669845, -183.6283474603465606, -76.29032973288636299 ) ) ;
#10149=ORIENTED_EDGE ( 'NONE', *, *, #12695, .F. ) ;
#10150=AXIS2_PLACEMENT_3D ( 'NONE', #4459, #36784, #20476 ) ;
#10151=PLANE ( 'NONE',  #34372 ) ;
#10154=EDGE_LOOP ( 'NONE', ( #35297, #17908, #42733, #46513 ) ) ;
#10155=ORIENTED_EDGE ( 'NONE', *, *, #40831, .T. ) ;
#10156=DIRECTION ( 'NONE',  ( 0.7948544414133481562, 0.000000000000000000, 0.6068001458186002006 ) ) ;
#10157=EDGE_CURVE ( 'NONE', #42041, #45184, #5291, .T. ) ;
#10159=DIRECTION ( 'NONE',  ( 0.000000000000000000, -1.000000000000000000, -0.000000000000000000 ) ) ;
#10162=VERTEX_POINT ( 'NONE', #50720 ) ;
#10163=ORIENTED_EDGE ( 'NONE', *, *, #14322, .F. ) ;
#10164=PLANE ( 'NONE',  #15863 ) ;
#10165=DIRECTION ( 'NONE',  ( -0.9890401873221644768, 0.000000000000000000, 0.1476465640024779702 ) ) ;
#10166=AXIS2_PLACEMENT_3D ( 'NONE', #36596, #51598, #326 ) ;
#10169=LINE ( 'NONE', #5980, #30558 ) ;
#10170=VERTEX_POINT ( 'NONE', #18143 ) ;
#10171=ADVANCED_FACE ( 'NONE', ( #51243 ), #14209, .T. ) ;
#10172=EDGE_CURVE ( 'NONE', #30279, #39399, #45934, .T. ) ;
#10173=DIRECTION ( 'NONE',  ( 0.6300878435817038881, 0.000000000000000000, 0.7765238627180482966 ) ) ;
#10175=LINE ( 'NONE', #45674, #31486 ) ;
#10176=ORIENTED_EDGE ( 'NONE', *, *, #13884, .T. ) ;
#10177=VERTEX_POINT ( 'NONE', #10497 ) ;
#10178=ADVANCED_FACE ( 'NONE', ( #50989 ), #26530, .T. ) ;
#10180=VERTEX_POINT ( 'NONE', #11267 ) ;
#10182=CIRCLE ( 'NONE', #2643, 125.0000000000000000 ) ;
#10184=EDGE_CURVE ( 'NONE', #6892, #1866, #22855, .T. ) ;
#10185=DIRECTION ( 'NONE',  ( 0.000000000000000000, 0.000000000000000000, 1.000000000000000000 ) ) ;
#10186=CARTESIAN_POINT ( 'NONE',  ( -8.461066480258370603, -177.1207230881787780, 117.3655938605930231 ) ) ;
#10187=VERTEX_POINT ( 'NONE', #22076 ) ;
#10188=DIRECTION ( 'NONE',  ( -0.9720229140804139689, 0.000000000000000000, 0.2348860457809708036 ) ) ;
#10190=VECTOR ( 'NONE', #2710, 1000.000000000000000 ) ;
#10191=ORIENTED_EDGE ( 'NONE', *, *, #47518, .T. ) ;
#10192=DIRECTION ( 'NONE',  ( 0.4031234292879730674, 0.000000000000000000, -0.9151456172430181280 ) ) ;
#10193=PLANE ( 'NONE',  #19000 ) ;
#10194=CARTESIAN_POINT ( 'NONE',  ( -48.47912675150885065, -193.5000000000000000, 6.938893903907228378E-15 ) ) ;
#10195=EDGE_LOOP ( 'NONE', ( #32726, #50782, #19623, #13226 ) ) ;
#10196=DIRECTION ( 'NONE',  ( 0.1476465640024710868, 0.000000000000000000, 0.9890401873221654760 ) ) ;
#10197=FACE_OUTER_BOUND ( 'NONE', #37361, .T. ) ;
#10200=LINE ( 'NONE', #37795, #18650 ) ;
#10201=EDGE_LOOP ( 'NONE', ( #8728, #36120, #4406, #20556 ) ) ;
#10205=CARTESIAN_POINT ( 'NONE',  ( -48.47912675150885065, -177.1207230881787780, 6.938893903907228378E-15 ) ) ;
#10206=ORIENTED_EDGE ( 'NONE', *, *, #7612, .T. ) ;
#10207=VECTOR ( 'NONE', #21749, 1000.000000000000114 ) ;
#10208=DIRECTION ( 'NONE',  ( 0.000000000000000000, 0.000000000000000000, 1.000000000000000000 ) ) ;
#10209=DIRECTION ( 'NONE',  ( 0.000000000000000000, -0.000000000000000000, 1.000000000000000000 ) ) ;
#10210=VERTEX_POINT ( 'NONE', #38874 ) ;
#10212=ORIENTED_EDGE ( 'NONE', *, *, #19759, .T. ) ;
#10213=EDGE_CURVE ( 'NONE', #25533, #47448, #39188, .T. ) ;
#10215=LINE ( 'NONE', #34398, #49707 ) ;
#10217=VECTOR ( 'NONE', #17393, 1000.000000000000000 ) ;
#10220=LINE ( 'NONE', #10743, #24971 ) ;
#10221=EDGE_CURVE ( 'NONE', #9326, #6776, #31246, .T. ) ;
#10223=CARTESIAN_POINT ( 'NONE',  ( -47.64924157374594671, -193.5000000000000000, 124.9972451320097377 ) ) ;
#10224=ORIENTED_EDGE ( 'NONE', *, *, #14789, .F. ) ;
#10226=CIRCLE ( 'NONE', #39582, 125.0000000000000000 ) ;
#10227=DIRECTION ( 'NONE',  ( 0.5829794791144650157, 0.000000000000000000, 0.8124868780056864193 ) ) ;
#10232=CARTESIAN_POINT ( 'NONE',  ( -41.30311180514221547, -193.5000000000000000, 123.7921848946937899 ) ) ;
#10235=EDGE_CURVE ( 'NONE', #42695, #37425, #29971, .T. ) ;
#10240=LINE ( 'NONE', #1317, #36511 ) ;
#10241=EDGE_LOOP ( 'NONE', ( #32459, #44604, #31159, #47780 ) ) ;
#10242=AXIS2_PLACEMENT_3D ( 'NONE', #39801, #19344, #35884 ) ;
#10244=EDGE_CURVE ( 'NONE', #36752, #20294, #1425, .T. ) ;
#10245=DIRECTION ( 'NONE',  ( 0.000000000000000000, 1.000000000000000000, 0.000000000000000000 ) ) ;
#10246=ORIENTED_EDGE ( 'NONE', *, *, #18740, .F. ) ;
#10248=ORIENTED_EDGE ( 'NONE', *, *, #41678, .F. ) ;
#10249=EDGE_CURVE ( 'NONE', #29042, #39776, #34672, .T. ) ;
#10250=DIRECTION ( 'NONE',  ( -0.000000000000000000, 1.000000000000000000, -0.000000000000000000 ) ) ;
#10252=FACE_OUTER_BOUND ( 'NONE', #35603, .T. ) ;
#10253=ORIENTED_EDGE ( 'NONE', *, *, #2819, .T. ) ;
#10254=ORIENTED_EDGE ( 'NONE', *, *, #26896, .F. ) ;
#10255=ADVANCED_FACE ( 'NONE', ( #39130 ), #43080, .F. ) ;
#10257=CARTESIAN_POINT ( 'NONE',  ( 53.18081239921338010, -189.7472609257535510, -72.73415134495935774 ) ) ;
#10260=CARTESIAN_POINT ( 'NONE',  ( -114.1105527140175155, -193.5000000000000000, 106.3838142112217611 ) ) ;
#10262=DIRECTION ( 'NONE',  ( -0.000000000000000000, 1.000000000000000000, -0.000000000000000000 ) ) ;
#10266=VECTOR ( 'NONE', #30415, 1000.000000000000227 ) ;
#10267=DIRECTION ( 'NONE',  ( 0.000000000000000000, 0.000000000000000000, -1.000000000000000000 ) ) ;
#10268=ORIENTED_EDGE ( 'NONE', *, *, #20343, .T. ) ;
#10269=CARTESIAN_POINT ( 'NONE',  ( 51.65665342072240662, -183.6283474603465606, 74.81861753132422166 ) ) ;
#10270=EDGE_CURVE ( 'NONE', #34518, #18747, #33309, .T. ) ;
#10271=PLANE ( 'NONE',  #13101 ) ;
#10272=VECTOR ( 'NONE', #10469, 1000.000000000000114 ) ;
#10273=FACE_OUTER_BOUND ( 'NONE', #7837, .T. ) ;
#10275=LINE ( 'NONE', #6848, #24811 ) ;
#10277=PLANE ( 'NONE',  #14359 ) ;
#10278=PLANE ( 'NONE',  #42543 ) ;
#10279=VECTOR ( 'NONE', #40452, 1000.000000000000000 ) ;
#10281=DIRECTION ( 'NONE',  ( -0.000000000000000000, 1.000000000000000000, -0.000000000000000000 ) ) ;
#10283=VECTOR ( 'NONE', #30586, 1000.000000000000000 ) ;
#10285=CARTESIAN_POINT ( 'NONE',  ( 71.87891646118019651, -175.3837268820161057, -33.74820638215424395 ) ) ;
#10288=EDGE_CURVE ( 'NONE', #44335, #4324, #36224, .T. ) ;
#10289=ADVANCED_FACE ( 'NONE', ( #7596 ), #39893, .F. ) ;
#10290=LINE ( 'NONE', #26311, #45343 ) ;
#10291=ADVANCED_FACE ( 'NONE', ( #7850 ), #16263, .T. ) ;
#10296=ORIENTED_EDGE ( 'NONE', *, *, #25440, .T. ) ;
#10297=ORIENTED_EDGE ( 'NONE', *, *, #10584, .T. ) ;
#10298=DIRECTION ( 'NONE',  ( -0.000000000000000000, 1.000000000000000000, -0.000000000000000000 ) ) ;
#10299=AXIS2_PLACEMENT_3D ( 'NONE', #40886, #16994, #33002 ) ;
#10300=CARTESIAN_POINT ( 'NONE',  ( -49.47868758801764955, -189.7472609257535510, -0.02963332782256313663 ) ) ;
#10301=DIRECTION ( 'NONE',  ( 0.2348860457809911206, 0.000000000000000000, -0.9720229140804089729 ) ) ;
#10304=DIRECTION ( 'NONE',  ( 0.9027978299657416494, 0.000000000000000000, 0.4300652022765245608 ) ) ;
#10305=DIRECTION ( 'NONE',  ( -0.9785564922995060311, 0.000000000000000000, 0.2059786187410889424 ) ) ;
#10307=PLANE ( 'NONE',  #3132 ) ;
#10308=VERTEX_POINT ( 'NONE', #39386 ) ;
#10310=DIRECTION ( 'NONE',  ( 0.000000000000000000, 0.000000000000000000, -1.000000000000000000 ) ) ;
#10312=DIRECTION ( 'NONE',  ( -0.000000000000000000, 1.000000000000000000, -0.000000000000000000 ) ) ;
#10313=ORIENTED_EDGE ( 'NONE', *, *, #26481, .T. ) ;
#10315=LINE ( 'NONE', #50528, #23778 ) ;
#10316=CYLINDRICAL_SURFACE ( 'NONE', #44185, 125.0000000000000000 ) ;
#10317=VECTOR ( 'NONE', #44365, 1000.000000000000000 ) ;
#10319=CIRCLE ( 'NONE', #1084, 125.0000000000000000 ) ;
#10321=AXIS2_PLACEMENT_3D ( 'NONE', #31812, #51273, #34962 ) ;
#10322=CARTESIAN_POINT ( 'NONE',  ( -120.5074237604784457, -193.5000000000000000, 100.9358816284415639 ) ) ;
#10323=DIRECTION ( 'NONE',  ( 0.05924062789372142729, 0.000000000000000000, -0.9982437317643209074 ) ) ;
#10324=EDGE_LOOP ( 'NONE', ( #38651, #16401, #41665, #28171 ) ) ;
#10325=DIRECTION ( 'NONE',  ( -0.7948544414133608127, 0.000000000000000000, 0.6068001458185834363 ) ) ;
#10326=CARTESIAN_POINT ( 'NONE',  ( 74.18685885783125400, -175.3837268820161057, -18.13990644964003351 ) ) ;
#10330=ORIENTED_EDGE ( 'NONE', *, *, #34271, .T. ) ;
#10331=DIRECTION ( 'NONE',  ( -0.000000000000000000, 1.000000000000000000, -0.000000000000000000 ) ) ;
#10333=DIRECTION ( 'NONE',  ( 0.000000000000000000, 0.000000000000000000, -1.000000000000000000 ) ) ;
#10335=ORIENTED_EDGE ( 'NONE', *, *, #16828, .F. ) ;
#10337=CARTESIAN_POINT ( 'NONE',  ( -67.22356632362124174, -193.5000000000000000, -123.5865930638409509 ) ) ;
#10338=DIRECTION ( 'NONE',  ( 0.000000000000000000, -1.000000000000000000, -0.000000000000000000 ) ) ;
#10340=CIRCLE ( 'NONE', #17078, 125.0000000000000000 ) ;
#10341=ORIENTED_EDGE ( 'NONE', *, *, #35058, .F. ) ;
#10342=LINE ( 'NONE', #41615, #33799 ) ;
#10343=ORIENTED_EDGE ( 'NONE', *, *, #3239, .F. ) ;
#10344=FACE_OUTER_BOUND ( 'NONE', #46322, .T. ) ;
#10349=EDGE_CURVE ( 'NONE', #20987, #35554, #8167, .T. ) ;
#10350=CARTESIAN_POINT ( 'NONE',  ( 73.32083127613157103, -177.1207230881787780, 28.10285082451656535 ) ) ;
#10351=AXIS2_PLACEMENT_3D ( 'NONE', #21854, #6081, #42067 ) ;
#10352=CARTESIAN_POINT ( 'NONE',  ( -173.2765435274470178, -183.6283474603465606, -7.113702696401515979 ) ) ;
#10353=VECTOR ( 'NONE', #43691, 1000.000000000000000 ) ;
#10357=LINE ( 'NONE', #1958, #51844 ) ;
#10358=CARTESIAN_POINT ( 'NONE',  ( 48.33059356687145680, -193.5000000000000000, 77.48473115145309009 ) ) ;
#10359=VECTOR ( 'NONE', #49067, 1000.000000000000114 ) ;
#10360=FACE_OUTER_BOUND ( 'NONE', #15347, .T. ) ;
#10361=DIRECTION ( 'NONE',  ( 0.000000000000000000, 0.000000000000000000, 1.000000000000000000 ) ) ;
#10362=ORIENTED_EDGE ( 'NONE', *, *, #40743, .F. ) ;
#10364=ORIENTED_EDGE ( 'NONE', *, *, #40280, .F. ) ;
#10365=FACE_OUTER_BOUND ( 'NONE', #38556, .T. ) ;
#10366=DIRECTION ( 'NONE',  ( 0.000000000000000000, 0.000000000000000000, -1.000000000000000000 ) ) ;
#10368=CARTESIAN_POINT ( 'NONE',  ( -173.4190745413846741, -189.7472609257535510, -3.874202661595026687 ) ) ;
#10369=DIRECTION ( 'NONE',  ( 0.000000000000000000, 1.000000000000000000, 0.000000000000000000 ) ) ;
#10372=DIRECTION ( 'NONE',  ( -0.000000000000000000, 1.000000000000000000, -0.000000000000000000 ) ) ;
#10373=VECTOR ( 'NONE', #18182, 1000.000000000000114 ) ;
#10374=ORIENTED_EDGE ( 'NONE', *, *, #12712, .T. ) ;
#10376=CARTESIAN_POINT ( 'NONE',  ( -19.92568551777507224, -175.3837268820161057, -121.6951149130962904 ) ) ;
#10377=CARTESIAN_POINT ( 'NONE',  ( -128.2395503755045638, -193.5000000000000000, -96.24590808611419845 ) ) ;
#10378=DIRECTION ( 'NONE',  ( 0.000000000000000000, 1.000000000000000000, 0.000000000000000000 ) ) ;
#10379=LINE ( 'NONE', #1978, #1910 ) ;
#10381=VERTEX_POINT ( 'NONE', #15770 ) ;
#10383=EDGE_CURVE ( 'NONE', #9092, #14259, #35978, .T. ) ;
#10385=EDGE_LOOP ( 'NONE', ( #29483, #102, #51673, #51801 ) ) ;
#10386=DIRECTION ( 'NONE',  ( 0.1182731709213660498, 0.000000000000000000, -0.9929810960135169173 ) ) ;
#10387=ADVANCED_FACE ( 'NONE', ( #52029 ), #31779, .F. ) ;
#10390=PLANE ( 'NONE',  #31527 ) ;
#10392=CARTESIAN_POINT ( 'NONE',  ( -160.9694636715425702, -175.3837268820161057, 54.50618404931040573 ) ) ;
#10393=LINE ( 'NONE', #46669, #5577 ) ;
#10395=CARTESIAN_POINT ( 'NONE',  ( -83.89965873179622236, -193.5000000000000000, 118.8334608768482497 ) ) ;
#10396=ORIENTED_EDGE ( 'NONE', *, *, #49158, .T. ) ;
#10397=LINE ( 'NONE', #15140, #7571 ) ;
#10399=VECTOR ( 'NONE', #51205, 1000.000000000000000 ) ;
#10400=AXIS2_PLACEMENT_3D ( 'NONE', #9381, #36970, #17783 ) ;
#10403=EDGE_CURVE ( 'NONE', #15221, #13319, #46786, .T. ) ;
#10404=ORIENTED_EDGE ( 'NONE', *, *, #16599, .T. ) ;
#10405=AXIS2_PLACEMENT_3D ( 'NONE', #17774, #29329, #21719 ) ;
#10407=ADVANCED_FACE ( 'NONE', ( #40416 ), #20201, .T. ) ;
#10408=ORIENTED_EDGE ( 'NONE', *, *, #5860, .F. ) ;
#10411=ORIENTED_EDGE ( 'NONE', *, *, #45908, .T. ) ;
#10412=FACE_OUTER_BOUND ( 'NONE', #26476, .T. ) ;
#10414=AXIS2_PLACEMENT_3D ( 'NONE', #50641, #22000, #14912 ) ;
#10415=DIRECTION ( 'NONE',  ( -0.6068001458185834363, 0.000000000000000000, -0.7948544414133608127 ) ) ;
#10416=ORIENTED_EDGE ( 'NONE', *, *, #47228, .F. ) ;
#10417=ORIENTED_EDGE ( 'NONE', *, *, #50246, .T. ) ;
#10418=ORIENTED_EDGE ( 'NONE', *, *, #40655, .T. ) ;
#10419=CARTESIAN_POINT ( 'NONE',  ( -170.5806857741408180, -193.5000000000000000, -21.61797988633145451 ) ) ;
#10420=CARTESIAN_POINT ( 'NONE',  ( -173.4724443937511751, -177.1207230881787780, 1.292495564989516454 ) ) ;
#10421=EDGE_CURVE ( 'NONE', #45486, #19065, #20456, .T. ) ;
#10422=CARTESIAN_POINT ( 'NONE',  ( -48.47912675150885065, -177.1207230881787780, 6.938893903907228378E-15 ) ) ;
#10423=CARTESIAN_POINT ( 'NONE',  ( -20.16057156355605784, -189.7472609257535510, -120.7230919990158782 ) ) ;
#10424=ORIENTED_EDGE ( 'NONE', *, *, #29995, .T. ) ;
#10426=DIRECTION ( 'NONE',  ( 0.9646355819083614058, 0.000000000000000000, -0.2635871660690581320 ) ) ;
#10427=ORIENTED_EDGE ( 'NONE', *, *, #13019, .F. ) ;
#10431=LINE ( 'NONE', #26458, #4821 ) ;
#10435=ORIENTED_EDGE ( 'NONE', *, *, #50050, .T. ) ;
#10436=VECTOR ( 'NONE', #10781, 1000.000000000000000 ) ;
#10440=CARTESIAN_POINT ( 'NONE',  ( -95.72791768350688812, -193.5000000000000000, -115.7261930397105232 ) ) ;
#10446=CARTESIAN_POINT ( 'NONE',  ( -53.47502265695599277, -177.1207230881787780, -124.9001241957025883 ) ) ;
#10447=ORIENTED_EDGE ( 'NONE', *, *, #30104, .T. ) ;
#10453=DIRECTION ( 'NONE',  ( -0.000000000000000000, 1.000000000000000000, -0.000000000000000000 ) ) ;
#10454=CARTESIAN_POINT ( 'NONE',  ( 54.46899307705341187, -177.1207230881787780, -70.89911581792813422 ) ) ;
#10456=DIRECTION ( 'NONE',  ( 0.000000000000000000, 1.000000000000000000, -0.000000000000000000 ) ) ;
#10457=DIRECTION ( 'NONE',  ( -0.000000000000000000, 1.000000000000000000, 0.000000000000000000 ) ) ;
#10459=VERTEX_POINT ( 'NONE', #38922 ) ;
#10460=CARTESIAN_POINT ( 'NONE',  ( -170.8336150310144887, -193.5000000000000000, 25.58083653558494319 ) ) ;
#10461=DIRECTION ( 'NONE',  ( 0.000000000000000000, 0.000000000000000000, 1.000000000000000000 ) ) ;
#10462=ORIENTED_EDGE ( 'NONE', *, *, #42711, .T. ) ;
#10465=EDGE_LOOP ( 'NONE', ( #38724, #20304, #21029, #24277 ) ) ;
#10466=EDGE_CURVE ( 'NONE', #7849, #51485, #14907, .T. ) ;
#10469=DIRECTION ( 'NONE',  ( -0.7765238627180482966, 0.000000000000000000, 0.6300878435817038881 ) ) ;
#10470=CARTESIAN_POINT ( 'NONE',  ( -47.53180039765465636, -183.6283474603465606, -0.3202698538628280800 ) ) ;
#10471=VECTOR ( 'NONE', #51819, 999.9999999999998863 ) ;
#10474=LINE ( 'NONE', #34141, #40891 ) ;
#10481=ORIENTED_EDGE ( 'NONE', *, *, #12788, .F. ) ;
#10482=VECTOR ( 'NONE', #28059, 1000.000000000000114 ) ;
#10483=PLANE ( 'NONE',  #4941 ) ;
#10484=AXIS2_PLACEMENT_3D ( 'NONE', #50056, #21406, #1437 ) ;
#10485=AXIS2_PLACEMENT_3D ( 'NONE', #9023, #41578, #48453 ) ;
#10486=LINE ( 'NONE', #6046, #12454 ) ;
#10489=LINE ( 'NONE', #18897, #13281 ) ;
#10490=DIRECTION ( 'NONE',  ( 0.000000000000000000, 0.000000000000000000, 1.000000000000000000 ) ) ;
#10491=ORIENTED_EDGE ( 'NONE', *, *, #27428, .T. ) ;
#10495=ORIENTED_EDGE ( 'NONE', *, *, #21766, .F. ) ;
#10496=DIRECTION ( 'NONE',  ( 0.000000000000000000, -1.000000000000000000, 0.000000000000000000 ) ) ;
#10497=CARTESIAN_POINT ( 'NONE',  ( -152.0588566364587848, -183.6283474603465606, -68.17212999877148150 ) ) ;
#10498=CARTESIAN_POINT ( 'NONE',  ( -48.30901192927175458, -193.5000000000000000, -124.9998842437354227 ) ) ;
#10499=VERTEX_POINT ( 'NONE', #30792 ) ;
#10500=EDGE_LOOP ( 'NONE', ( #48122, #16460, #43190, #2038 ) ) ;
#10501=LINE ( 'NONE', #34428, #16471 ) ;
#10503=FACE_OUTER_BOUND ( 'NONE', #38385, .T. ) ;
#10505=CARTESIAN_POINT ( 'NONE',  ( 35.67816836544800907, -193.5000000000000000, -92.42591454022745268 ) ) ;
#10509=FACE_OUTER_BOUND ( 'NONE', #13877, .T. ) ;
#10510=DIRECTION ( 'NONE',  ( 0.000000000000000000, 0.000000000000000000, 1.000000000000000000 ) ) ;
#10512=FACE_OUTER_BOUND ( 'NONE', #32584, .T. ) ;
#10513=AXIS2_PLACEMENT_3D ( 'NONE', #6785, #2049, #26478 ) ;
#10514=EDGE_CURVE ( 'NONE', #40054, #18957, #43129, .T. ) ;
#10515=ADVANCED_FACE ( 'NONE', ( #6636 ), #23173, .F. ) ;
#10517=EDGE_CURVE ( 'NONE', #16252, #17485, #50773, .T. ) ;
#10519=DIRECTION ( 'NONE',  ( -0.000000000000000000, 1.000000000000000000, -0.000000000000000000 ) ) ;
#10520=AXIS2_PLACEMENT_3D ( 'NONE', #22753, #39020, #26423 ) ;
#10523=ORIENTED_EDGE ( 'NONE', *, *, #20230, .F. ) ;
#10524=CARTESIAN_POINT ( 'NONE',  ( -145.0195698084541505, -175.3837268820161057, 79.40367028273126948 ) ) ;
#10525=EDGE_CURVE ( 'NONE', #37576, #45084, #9045, .T. ) ;
#10526=CARTESIAN_POINT ( 'NONE',  ( 43.12693905415815010, -175.3837268820161057, -83.57229767764155781 ) ) ;
#10527=VECTOR ( 'NONE', #41140, 1000.000000000000000 ) ;
#10528=EDGE_CURVE ( 'NONE', #50173, #10187, #7133, .T. ) ;
#10529=AXIS2_PLACEMENT_3D ( 'NONE', #27408, #43456, #35545 ) ;
#10530=DIRECTION ( 'NONE',  ( 0.000000000000000000, -1.000000000000000000, 0.000000000000000000 ) ) ;
#10531=CARTESIAN_POINT ( 'NONE',  ( -109.0835867659424565, -193.5000000000000000, -109.3256576763154726 ) ) ;
#10532=ORIENTED_EDGE ( 'NONE', *, *, #46549, .T. ) ;
#10533=EDGE_CURVE ( 'NONE', #34277, #15815, #1461, .T. ) ;
#10534=AXIS2_PLACEMENT_3D ( 'NONE', #10761, #23610, #15761 ) ;
#10537=EDGE_CURVE ( 'NONE', #32593, #8246, #3144, .T. ) ;
#10538=LINE ( 'NONE', #22888, #43795 ) ;
#10540=PLANE ( 'NONE',  #12776 ) ;
#10541=EDGE_CURVE ( 'NONE', #29842, #41150, #50993, .T. ) ;
#10542=ORIENTED_EDGE ( 'NONE', *, *, #14677, .T. ) ;
#10543=DIRECTION ( 'NONE',  ( 0.9995608365087942371, 0.000000000000000000, 0.02963332782256331357 ) ) ;
#10544=CARTESIAN_POINT ( 'NONE',  ( -170.2837019307126809, -177.1207230881787780, 23.23456943914128203 ) ) ;
#10545=ORIENTED_EDGE ( 'NONE', *, *, #27435, .F. ) ;
#10546=ORIENTED_EDGE ( 'NONE', *, *, #14754, .F. ) ;
#10547=CIRCLE ( 'NONE', #39084, 125.0000000000000000 ) ;
#10548=ORIENTED_EDGE ( 'NONE', *, *, #46483, .T. ) ;
#10550=AXIS2_PLACEMENT_3D ( 'NONE', #41333, #5353, #37394 ) ;
#10551=CIRCLE ( 'NONE', #2974, 125.0000000000000000 ) ;
#10552=DIRECTION ( 'NONE',  ( -0.000000000000000000, 1.000000000000000000, -0.000000000000000000 ) ) ;
#10553=CARTESIAN_POINT ( 'NONE',  ( -11.17913199888832843, -193.5000000000000000, 119.3051146910914326 ) ) ;
#10555=EDGE_CURVE ( 'NONE', #23501, #14662, #10823, .T. ) ;
#10558=CARTESIAN_POINT ( 'NONE',  ( -117.6201219941651601, -193.5000000000000000, 104.1370384486469902 ) ) ;
#10561=VERTEX_POINT ( 'NONE', #22909 ) ;
#10562=CIRCLE ( 'NONE', #50041, 125.0000000000000000 ) ;
#10563=DIRECTION ( 'NONE',  ( 0.000000000000000000, -1.000000000000000000, 0.000000000000000000 ) ) ;
#10564=ORIENTED_EDGE ( 'NONE', *, *, #13614, .F. ) ;
#10566=VERTEX_POINT ( 'NONE', #11317 ) ;
#10567=PLANE ( 'NONE',  #19053 ) ;
#10568=VECTOR ( 'NONE', #44979, 1000.000000000000000 ) ;
#10571=EDGE_CURVE ( 'NONE', #7135, #41798, #2928, .T. ) ;
#10572=ORIENTED_EDGE ( 'NONE', *, *, #39814, .F. ) ;
#10574=CARTESIAN_POINT ( 'NONE',  ( -65.65563056894596627, -183.6283474603465606, 123.8142468240612999 ) ) ;
#10577=LINE ( 'NONE', #22674, #13108 ) ;
#10581=EDGE_CURVE ( 'NONE', #23257, #22776, #35035, .T. ) ;
#10582=DIRECTION ( 'NONE',  ( 0.5586467658036535777, 0.000000000000000000, -0.8294056854502011022 ) ) ;
#10584=EDGE_CURVE ( 'NONE', #4360, #23329, #44436, .T. ) ;
#10585=ORIENTED_EDGE ( 'NONE', *, *, #32867, .F. ) ;
#10587=VERTEX_POINT ( 'NONE', #32600 ) ;
#10589=CIRCLE ( 'NONE', #14806, 125.0000000000000000 ) ;
#10590=CARTESIAN_POINT ( 'NONE',  ( -142.9772358822569629, -193.5000000000000000, 81.82363577055969017 ) ) ;
#10591=CARTESIAN_POINT ( 'NONE',  ( 64.01121016852529522, -193.5000000000000000, -54.50618404930953176 ) ) ;
#10593=VECTOR ( 'NONE', #21843, 1000.000000000000000 ) ;
#10596=CARTESIAN_POINT ( 'NONE',  ( -142.3192003680973130, -193.5000000000000000, 82.57748230379306165 ) ) ;
#10597=CARTESIAN_POINT ( 'NONE',  ( -46.12632737020501850, -183.6283474603465606, -123.9784823535113532 ) ) ;
#10598=VERTEX_POINT ( 'NONE', #11838 ) ;
#10599=CARTESIAN_POINT ( 'NONE',  ( -48.36085358058748085, -189.7472609257535510, -0.9929810960135100339 ) ) ;
#10600=ADVANCED_FACE ( 'NONE', ( #35493 ), #48374, .T. ) ;
#10601=CIRCLE ( 'NONE', #25727, 125.0000000000000000 ) ;
#10603=CARTESIAN_POINT ( 'NONE',  ( 75.02564229359539638, -189.7472609257535510, -19.27620354518634826 ) ) ;
#10605=ORIENTED_EDGE ( 'NONE', *, *, #47659, .F. ) ;
#10606=CIRCLE ( 'NONE', #51771, 125.0000000000000000 ) ;
#10610=DIRECTION ( 'NONE',  ( -0.8124868780056863082, 0.000000000000000000, 0.5829794791144649047 ) ) ;
#10611=VECTOR ( 'NONE', #15497, 1000.000000000000000 ) ;
#10612=ADVANCED_FACE ( 'NONE', ( #3698 ), #51814, .T. ) ;
#10613=VECTOR ( 'NONE', #8489, 1000.000000000000000 ) ;
#10614=CARTESIAN_POINT ( 'NONE',  ( -48.47912675150885065, -175.3837268820161057, 6.938893903907228378E-15 ) ) ;
#10615=ORIENTED_EDGE ( 'NONE', *, *, #47967, .T. ) ;
#10616=CARTESIAN_POINT ( 'NONE',  ( 8.750818922897904528, -193.5000000000000000, -111.1293539894138434 ) ) ;
#10617=ORIENTED_EDGE ( 'NONE', *, *, #15887, .T. ) ;
#10619=LINE ( 'NONE', #26650, #49361 ) ;
#10620=CARTESIAN_POINT ( 'NONE',  ( -159.5526844214375899, -183.6283474603465606, 57.33816169485221081 ) ) ;
#10621=DIRECTION ( 'NONE',  ( 0.000000000000000000, 1.000000000000000000, -0.000000000000000000 ) ) ;
#10622=ORIENTED_EDGE ( 'NONE', *, *, #6330, .T. ) ;
#10625=ADVANCED_FACE ( 'NONE', ( #11594 ), #27865, .T. ) ;
#10626=CARTESIAN_POINT ( 'NONE',  ( -166.1003692892502102, -193.5000000000000000, -42.31126686685032467 ) ) ;
#10630=LINE ( 'NONE', #19540, #2700 ) ;
#10631=DIRECTION ( 'NONE',  ( 0.000000000000000000, 0.000000000000000000, 1.000000000000000000 ) ) ;
#10633=CIRCLE ( 'NONE', #44203, 125.0000000000000000 ) ;
#10635=DIRECTION ( 'NONE',  ( 0.7765238627180437447, 0.000000000000000000, -0.6300878435817094392 ) ) ;
#10636=VERTEX_POINT ( 'NONE', #48116 ) ;
#10637=ORIENTED_EDGE ( 'NONE', *, *, #32859, .F. ) ;
#10641=AXIS2_PLACEMENT_3D ( 'NONE', #50734, #38887, #11277 ) ;
#10644=AXIS2_PLACEMENT_3D ( 'NONE', #43995, #34621, #50665 ) ;
#10645=DIRECTION ( 'NONE',  ( -0.000000000000000000, 1.000000000000000000, -0.000000000000000000 ) ) ;
#10650=DIRECTION ( 'NONE',  ( 0.000000000000000000, 0.000000000000000000, -1.000000000000000000 ) ) ;
#10653=ORIENTED_EDGE ( 'NONE', *, *, #1191, .F. ) ;
#10654=PLANE ( 'NONE',  #9479 ) ;
#10655=LINE ( 'NONE', #18793, #17777 ) ;
#10657=CARTESIAN_POINT ( 'NONE',  ( -148.7414553014637306, -193.5000000000000000, 72.96212019587208886 ) ) ;
#10659=DIRECTION ( 'NONE',  ( 0.000000000000000000, 1.000000000000000000, 0.000000000000000000 ) ) ;
#10661=DIRECTION ( 'NONE',  ( 0.4031234292879730674, 0.000000000000000000, -0.9151456172430181280 ) ) ;
#10662=VERTEX_POINT ( 'NONE', #24450 ) ;
#10663=AXIS2_PLACEMENT_3D ( 'NONE', #35130, #39572, #38560 ) ;
#10664=AXIS2_PLACEMENT_3D ( 'NONE', #46046, #21860, #33433 ) ;
#10666=DIRECTION ( 'NONE',  ( -0.000000000000000000, 1.000000000000000000, -0.000000000000000000 ) ) ;
#10667=VERTEX_POINT ( 'NONE', #4229 ) ;
#10668=VECTOR ( 'NONE', #41300, 1000.000000000000000 ) ;
#10670=DIRECTION ( 'NONE',  ( 0.6528221181905119463, 0.000000000000000000, 0.7575112421616284619 ) ) ;
#10673=CARTESIAN_POINT ( 'NONE',  ( -70.24606818074175862, -193.5000000000000000, -122.0745693923548885 ) ) ;
#10674=AXIS2_PLACEMENT_3D ( 'NONE', #27418, #79, #43467 ) ;
#10676=DIRECTION ( 'NONE',  ( 0.000000000000000000, 0.000000000000000000, 1.000000000000000000 ) ) ;
#10677=AXIS2_PLACEMENT_3D ( 'NONE', #16063, #40730, #4750 ) ;
#10678=DIRECTION ( 'NONE',  ( 0.000000000000000000, 0.000000000000000000, 1.000000000000000000 ) ) ;
#10679=ORIENTED_EDGE ( 'NONE', *, *, #50433, .T. ) ;
#10680=DIRECTION ( 'NONE',  ( 0.000000000000000000, 1.000000000000000000, 0.000000000000000000 ) ) ;
#10681=VECTOR ( 'NONE', #21087, 1000.000000000000000 ) ;
#10683=CARTESIAN_POINT ( 'NONE',  ( 28.02885774092381865, -189.7472609257535510, 98.85104101073331151 ) ) ;
#10684=VERTEX_POINT ( 'NONE', #8170 ) ;
#10685=EDGE_LOOP ( 'NONE', ( #32329, #50048, #50366, #30804 ) ) ;
#10686=EDGE_LOOP ( 'NONE', ( #47887, #14202, #1728, #624 ) ) ;
#10688=CARTESIAN_POINT ( 'NONE',  ( -129.9529520667707914, -175.3837268820161057, -94.79987230211959570 ) ) ;
#10689=DIRECTION ( 'NONE',  ( 0.000000000000000000, 1.000000000000000000, -0.000000000000000000 ) ) ;
#10693=ORIENTED_EDGE ( 'NONE', *, *, #10706, .T. ) ;
#10694=ADVANCED_FACE ( 'NONE', ( #4490 ), #28385, .T. ) ;
#10695=PLANE ( 'NONE',  #12269 ) ;
#10696=ORIENTED_EDGE ( 'NONE', *, *, #40919, .F. ) ;
#10698=VERTEX_POINT ( 'NONE', #20506 ) ;
#10699=VECTOR ( 'NONE', #51437, 1000.000000000000000 ) ;
#10700=ORIENTED_EDGE ( 'NONE', *, *, #48169, .T. ) ;
#10702=CARTESIAN_POINT ( 'NONE',  ( -173.2765435274470178, -193.5000000000000000, -7.113702696401505321 ) ) ;
#10703=CARTESIAN_POINT ( 'NONE',  ( 66.11593792271145276, -193.5000000000000000, -47.37063079638321739 ) ) ;
#10706=EDGE_CURVE ( 'NONE', #4089, #15087, #2337, .T. ) ;
#10707=FACE_OUTER_BOUND ( 'NONE', #34604, .T. ) ;
#10709=DIRECTION ( 'NONE',  ( -0.5085311186492094127, 0.000000000000000000, -0.8610436117673619938 ) ) ;
#10710=EDGE_LOOP ( 'NONE', ( #15511, #38258, #9539, #44044 ) ) ;
#10711=EDGE_LOOP ( 'NONE', ( #29105, #26734, #19944, #31314 ) ) ;
#10712=LINE ( 'NONE', #26737, #20339 ) ;
#10713=VECTOR ( 'NONE', #47728, 1000.000000000000227 ) ;
#10714=EDGE_CURVE ( 'NONE', #43197, #36214, #7647, .T. ) ;
#10716=CIRCLE ( 'NONE', #13236, 125.0000000000000000 ) ;
#10717=CARTESIAN_POINT ( 'NONE',  ( 65.52619748798558419, -177.1207230881787780, 48.77484799213969069 ) ) ;
#10718=ORIENTED_EDGE ( 'NONE', *, *, #971, .T. ) ;
#10720=LINE ( 'NONE', #39075, #42465 ) ;
#10722=CARTESIAN_POINT ( 'NONE',  ( -85.14888725715768203, -175.3837268820161057, 119.5003291395398577 ) ) ;
#10726=LINE ( 'NONE', #38829, #12035 ) ;
#10727=DIRECTION ( 'NONE',  ( 0.000000000000000000, 0.000000000000000000, 1.000000000000000000 ) ) ;
#10732=CARTESIAN_POINT ( 'NONE',  ( -172.0042974347349229, -189.7472609257535510, 10.84123789944660743 ) ) ;
#10733=CARTESIAN_POINT ( 'NONE',  ( -168.0489871616337325, -189.7472609257535510, -32.84887689123905830 ) ) ;
#10734=VERTEX_POINT ( 'NONE', #24 ) ;
#10737=AXIS2_PLACEMENT_3D ( 'NONE', #19806, #35841, #15890 ) ;
#10738=CARTESIAN_POINT ( 'NONE',  ( -49.30901192927175458, -189.7472609257535510, -124.9972451320097093 ) ) ;
#10739=CIRCLE ( 'NONE', #39284, 125.0000000000000000 ) ;
#10740=LINE ( 'NONE', #46752, #44673 ) ;
#10741=LINE ( 'NONE', #39096, #12809 ) ;
#10742=VECTOR ( 'NONE', #593, 1000.000000000000114 ) ;
#10743=CARTESIAN_POINT ( 'NONE',  ( -139.8555433305420195, -193.5000000000000000, -83.82333043185242616 ) ) ;
#10744=LINE ( 'NONE', #11509, #18505 ) ;
#10746=DIRECTION ( 'NONE',  ( -0.000000000000000000, 1.000000000000000000, -0.000000000000000000 ) ) ;
#10747=VERTEX_POINT ( 'NONE', #43405 ) ;
#10749=AXIS2_PLACEMENT_3D ( 'NONE', #22058, #38077, #18123 ) ;
#10750=ORIENTED_EDGE ( 'NONE', *, *, #42437, .F. ) ;
#10751=DIRECTION ( 'NONE',  ( -0.000000000000000000, 1.000000000000000000, -0.000000000000000000 ) ) ;
#10755=DIRECTION ( 'NONE',  ( 0.000000000000000000, 1.000000000000000000, 0.000000000000000000 ) ) ;
#10756=DIRECTION ( 'NONE',  ( 0.000000000000000000, -1.000000000000000000, 0.000000000000000000 ) ) ;
#10757=ORIENTED_EDGE ( 'NONE', *, *, #6450, .T. ) ;
#10758=CARTESIAN_POINT ( 'NONE',  ( -145.6517069852672535, -175.3837268820161057, 78.62880929222943394 ) ) ;
#10759=CARTESIAN_POINT ( 'NONE',  ( -48.47912675150885065, -189.7472609257535510, 6.938893903907228378E-15 ) ) ;
#10760=ORIENTED_EDGE ( 'NONE', *, *, #30207, .T. ) ;
#10761=CARTESIAN_POINT ( 'NONE',  ( -170.6250538923603131, -193.5000000000000000, 26.55884942729649723 ) ) ;
#10762=ORIENTED_EDGE ( 'NONE', *, *, #38603, .T. ) ;
#10763=CARTESIAN_POINT ( 'NONE',  ( 42.10477485469927927, -183.6283474603465606, 86.13684908212515268 ) ) ;
#10764=ORIENTED_EDGE ( 'NONE', *, *, #23748, .F. ) ;
#10766=DIRECTION ( 'NONE',  ( 0.000000000000000000, 0.000000000000000000, 1.000000000000000000 ) ) ;
#10767=DIRECTION ( 'NONE',  ( 0.000000000000000000, -1.000000000000000000, 0.000000000000000000 ) ) ;
#10768=DIRECTION ( 'NONE',  ( -0.000000000000000000, 1.000000000000000000, -0.000000000000000000 ) ) ;
#10769=VERTEX_POINT ( 'NONE', #12881 ) ;
#10770=ORIENTED_EDGE ( 'NONE', *, *, #17882, .F. ) ;
#10771=ADVANCED_FACE ( 'NONE', ( #20778 ), #45734, .T. ) ;
#10772=EDGE_CURVE ( 'NONE', #39548, #22041, #41253, .T. ) ;
#10773=DIRECTION ( 'NONE',  ( -0.000000000000000000, 1.000000000000000000, -0.000000000000000000 ) ) ;
#10775=FACE_OUTER_BOUND ( 'NONE', #40569, .T. ) ;
#10777=EDGE_CURVE ( 'NONE', #30392, #42165, #26671, .T. ) ;
#10778=FACE_OUTER_BOUND ( 'NONE', #35710, .T. ) ;
#10779=VERTEX_POINT ( 'NONE', #25494 ) ;
#10780=AXIS2_PLACEMENT_3D ( 'NONE', #37315, #12879, #17871 ) ;
#10781=DIRECTION ( 'NONE',  ( -0.000000000000000000, 1.000000000000000000, -0.000000000000000000 ) ) ;
#10782=DIRECTION ( 'NONE',  ( 0.9842305779475954974, 0.000000000000000000, 0.1768902751225803205 ) ) ;
#10784=CARTESIAN_POINT ( 'NONE',  ( -48.47912675150885065, -183.6283474603465606, 6.938893903907228378E-15 ) ) ;
#10786=DIRECTION ( 'NONE',  ( -0.000000000000000000, 1.000000000000000000, 0.000000000000000000 ) ) ;
#10793=FACE_OUTER_BOUND ( 'NONE', #22905, .T. ) ;
#10795=PLANE ( 'NONE',  #3081 ) ;
#10796=DIRECTION ( 'NONE',  ( -0.000000000000000000, 1.000000000000000000, -0.000000000000000000 ) ) ;
#10798=CIRCLE ( 'NONE', #9120, 124.9999999999999858 ) ;
#10799=DIRECTION ( 'NONE',  ( 0.000000000000000000, 0.000000000000000000, 1.000000000000000000 ) ) ;
#10801=FACE_OUTER_BOUND ( 'NONE', #22002, .T. ) ;
#10802=CARTESIAN_POINT ( 'NONE',  ( 7.991501969728830090, -193.5000000000000000, 110.3950557015152754 ) ) ;
#10803=ORIENTED_EDGE ( 'NONE', *, *, #48437, .T. ) ;
#10809=ORIENTED_EDGE ( 'NONE', *, *, #27902, .T. ) ;
#10810=AXIS2_PLACEMENT_3D ( 'NONE', #24645, #29363, #37256 ) ;
#10811=ORIENTED_EDGE ( 'NONE', *, *, #7054, .T. ) ;
#10812=CARTESIAN_POINT ( 'NONE',  ( -172.4792251663439231, -183.6283474603465606, 0.3215015308248941328 ) ) ;
#10813=VECTOR ( 'NONE', #8872, 1000.000000000000000 ) ;
#10817=LINE ( 'NONE', #30519, #51331 ) ;
#10818=CARTESIAN_POINT ( 'NONE',  ( -48.47912675150885065, -177.1207230881787780, 6.938893903907228378E-15 ) ) ;
#10821=DIRECTION ( 'NONE',  ( 0.000000000000000000, -0.000000000000000000, 1.000000000000000000 ) ) ;
#10823=LINE ( 'NONE', #51290, #23305 ) ;
#10825=ORIENTED_EDGE ( 'NONE', *, *, #7398, .F. ) ;
#10827=LINE ( 'NONE', #49742, #28940 ) ;
#10828=VERTEX_POINT ( 'NONE', #1833 ) ;
#10829=CARTESIAN_POINT ( 'NONE',  ( -93.85419746441394295, -183.6283474603465606, 115.4006183233324805 ) ) ;
#10830=ORIENTED_EDGE ( 'NONE', *, *, #1326, .F. ) ;
#10833=DIRECTION ( 'NONE',  ( -0.9890401873221623674, 0.000000000000000000, -0.1476465640024917925 ) ) ;
#10836=ADVANCED_FACE ( 'NONE', ( #17376 ), #33397, .T. ) ;
#10837=AXIS2_PLACEMENT_3D ( 'NONE', #33267, #34302, #2251 ) ;
#10839=CARTESIAN_POINT ( 'NONE',  ( -26.53529504715431031, -193.5000000000000000, 123.0587999703026725 ) ) ;
#10840=EDGE_CURVE ( 'NONE', #18322, #40221, #44311, .T. ) ;
#10842=EDGE_LOOP ( 'NONE', ( #14085, #39103, #43697, #21541 ) ) ;
#10843=DIRECTION ( 'NONE',  ( -0.5085311186492094127, 0.000000000000000000, -0.8610436117673619938 ) ) ;
#10845=EDGE_CURVE ( 'NONE', #43984, #41178, #21824, .T. ) ;
#10847=FACE_OUTER_BOUND ( 'NONE', #4061, .T. ) ;
#10848=CARTESIAN_POINT ( 'NONE',  ( -159.5526844214375615, -193.5000000000000000, 57.33816169485226055 ) ) ;
#10849=ORIENTED_EDGE ( 'NONE', *, *, #45256, .T. ) ;
#10850=FACE_OUTER_BOUND ( 'NONE', #3445, .T. ) ;
#10853=CARTESIAN_POINT ( 'NONE',  ( -47.53180039765466347, -193.5000000000000000, 0.3202698538628485636 ) ) ;
#10854=PLANE ( 'NONE',  #21141 ) ;
#10855=ORIENTED_EDGE ( 'NONE', *, *, #40831, .F. ) ;
#10859=FACE_OUTER_BOUND ( 'NONE', #23330, .T. ) ;
#10860=ORIENTED_EDGE ( 'NONE', *, *, #4659, .T. ) ;
#10863=CARTESIAN_POINT ( 'NONE',  ( -33.86391487983341619, -175.3837268820161057, 124.1426420773540542 ) ) ;
#10865=VERTEX_POINT ( 'NONE', #1052 ) ;
#10866=EDGE_LOOP ( 'NONE', ( #3272, #3394, #10981, #21368 ) ) ;
#10874=CARTESIAN_POINT ( 'NONE',  ( 43.18784210722336780, -193.5000000000000000, -84.98333260264752198 ) ) ;
#10876=EDGE_CURVE ( 'NONE', #8246, #31707, #42810, .T. ) ;
#10877=EDGE_CURVE ( 'NONE', #3069, #2708, #29953, .T. ) ;
#10878=EDGE_CURVE ( 'NONE', #15404, #47058, #15805, .T. ) ;
#10880=LINE ( 'NONE', #3497, #33692 ) ;
#10882=ORIENTED_EDGE ( 'NONE', *, *, #24362, .F. ) ;
#10883=ADVANCED_FACE ( 'NONE', ( #30981 ), #18131, .T. ) ;
#10884=EDGE_LOOP ( 'NONE', ( #26515, #1004, #34062, #25576 ) ) ;
#10887=CARTESIAN_POINT ( 'NONE',  ( 55.91309001144629320, -177.1207230881787780, 68.75510947788671956 ) ) ;
#10888=VECTOR ( 'NONE', #44361, 1000.000000000000000 ) ;
#10890=DIRECTION ( 'NONE',  ( 0.000000000000000000, 0.000000000000000000, 1.000000000000000000 ) ) ;
#10891=DIRECTION ( 'NONE',  ( 0.3482016354343995812, 0.000000000000000000, -0.9374196611341205632 ) ) ;
#10892=ORIENTED_EDGE ( 'NONE', *, *, #4906, .F. ) ;
#10893=EDGE_CURVE ( 'NONE', #51589, #16369, #51037, .T. ) ;
#10895=EDGE_CURVE ( 'NONE', #50975, #39853, #2086, .T. ) ;
#10896=ORIENTED_EDGE ( 'NONE', *, *, #9188, .F. ) ;
#10897=ORIENTED_EDGE ( 'NONE', *, *, #1191, .T. ) ;
#10899=DIRECTION ( 'NONE',  ( 0.000000000000000000, 0.000000000000000000, -1.000000000000000000 ) ) ;
#10900=EDGE_CURVE ( 'NONE', #50209, #28776, #10489, .T. ) ;
#10903=ADVANCED_FACE ( 'NONE', ( #26259 ), #42285, .T. ) ;
#10904=DIRECTION ( 'NONE',  ( 0.7175072570443249420, 0.000000000000000000, 0.6965510290630033685 ) ) ;
#10907=CARTESIAN_POINT ( 'NONE',  ( 43.86477233319989466, -175.3837268820161057, -84.24728067915975771 ) ) ;
#10909=VECTOR ( 'NONE', #36735, 1000.000000000000000 ) ;
#10910=VECTOR ( 'NONE', #38254, 1000.000000000000000 ) ;
#10912=CYLINDRICAL_SURFACE ( 'NONE', #11147, 125.0000000000000000 ) ;
#10913=LINE ( 'NONE', #20600, #15188 ) ;
#10914=ORIENTED_EDGE ( 'NONE', *, *, #19617, .T. ) ;
#10915=CARTESIAN_POINT ( 'NONE',  ( -158.0280232639029236, -175.3837268820161057, 60.19999396110247147 ) ) ;
#10916=CARTESIAN_POINT ( 'NONE',  ( 39.18328161278951427, -193.5000000000000000, 89.10837311819236106 ) ) ;
#10918=DIRECTION ( 'NONE',  ( 0.000000000000000000, 0.000000000000000000, 1.000000000000000000 ) ) ;
#10922=ORIENTED_EDGE ( 'NONE', *, *, #9872, .T. ) ;
#10923=VECTOR ( 'NONE', #39426, 1000.000000000000000 ) ;
#10925=CARTESIAN_POINT ( 'NONE',  ( 69.99104047056317768, -175.3837268820161057, -39.87254040532513244 ) ) ;
#10926=ORIENTED_EDGE ( 'NONE', *, *, #7616, .T. ) ;
#10927=EDGE_LOOP ( 'NONE', ( #26727, #7618, #15170, #28659 ) ) ;
#10929=VERTEX_POINT ( 'NONE', #11776 ) ;
#10934=ORIENTED_EDGE ( 'NONE', *, *, #47198, .T. ) ;
#10935=CARTESIAN_POINT ( 'NONE',  ( 71.87891646118019651, -189.7472609257535510, -33.74820638215424395 ) ) ;
#10936=EDGE_CURVE ( 'NONE', #38286, #46129, #31768, .T. ) ;
#10937=EDGE_CURVE ( 'NONE', #11500, #21582, #35697, .T. ) ;
#10938=CARTESIAN_POINT ( 'NONE',  ( -97.70585564814139445, -175.3837268820161057, 113.8100815915419162 ) ) ;
#10939=DIRECTION ( 'NONE',  ( -0.000000000000000000, 1.000000000000000000, -0.000000000000000000 ) ) ;
#10941=ORIENTED_EDGE ( 'NONE', *, *, #33375, .F. ) ;
#10945=DIRECTION ( 'NONE',  ( 0.2348860457809775482, 0.000000000000000000, 0.9720229140804121926 ) ) ;
#10947=CARTESIAN_POINT ( 'NONE',  ( 74.00867759460086859, -193.5000000000000000, 24.93467037017222410 ) ) ;
#10948=CARTESIAN_POINT ( 'NONE',  ( -19.92568551777507224, -189.7472609257535510, -121.6951149130962904 ) ) ;
#10949=CYLINDRICAL_SURFACE ( 'NONE', #50723, 125.0000000000000000 ) ;
#10950=ORIENTED_EDGE ( 'NONE', *, *, #42906, .T. ) ;
#10951=CARTESIAN_POINT ( 'NONE',  ( -163.3245969606054473, -189.7472609257535510, -46.76022031560624725 ) ) ;
#10952=VERTEX_POINT ( 'NONE', #16003 ) ;
#10953=DIRECTION ( 'NONE',  ( -0.000000000000000000, 1.000000000000000000, -0.000000000000000000 ) ) ;
#10954=EDGE_LOOP ( 'NONE', ( #34539, #5241, #44350, #22231 ) ) ;
#10955=ORIENTED_EDGE ( 'NONE', *, *, #15773, .F. ) ;
#10956=AXIS2_PLACEMENT_3D ( 'NONE', #22831, #47531, #27017 ) ;
#10957=PLANE ( 'NONE',  #1434 ) ;
#10959=CARTESIAN_POINT ( 'NONE',  ( -101.0675409952199999, -183.6283474603465606, 113.3995532942341100 ) ) ;
#10960=DIRECTION ( 'NONE',  ( 0.05924062789371441901, 0.000000000000000000, -0.9982437317643214625 ) ) ;
#10961=CARTESIAN_POINT ( 'NONE',  ( -41.24387117724851493, -193.5000000000000000, 124.7904286264581231 ) ) ;
#10965=EDGE_CURVE ( 'NONE', #36158, #38434, #11526, .T. ) ;
#10966=EDGE_LOOP ( 'NONE', ( #24045, #7069, #19342, #44588 ) ) ;
#10967=LINE ( 'NONE', #42239, #41307 ) ;
#10968=DIRECTION ( 'NONE',  ( 0.000000000000000000, 0.000000000000000000, 1.000000000000000000 ) ) ;
#10969=DIRECTION ( 'NONE',  ( -0.000000000000000000, 1.000000000000000000, -0.000000000000000000 ) ) ;
#10973=VECTOR ( 'NONE', #46101, 1000.000000000000000 ) ;
#10974=LINE ( 'NONE', #50940, #41429 ) ;
#10975=CARTESIAN_POINT ( 'NONE',  ( 40.30419662299490824, -177.1207230881787780, -87.99159897727903967 ) ) ;
#10976=EDGE_LOOP ( 'NONE', ( #15088, #29291, #1790, #48475 ) ) ;
#10977=CARTESIAN_POINT ( 'NONE',  ( -48.47912675150885065, -177.1207230881787780, 6.938893903907228378E-15 ) ) ;
#10979=AXIS2_PLACEMENT_3D ( 'NONE', #13640, #6017, #10209 ) ;
#10980=CARTESIAN_POINT ( 'NONE',  ( -49.03777351731249468, -177.1207230881787780, -0.8294056854502022125 ) ) ;
#10981=ORIENTED_EDGE ( 'NONE', *, *, #32750, .T. ) ;
#10983=DIRECTION ( 'NONE',  ( -0.000000000000000000, 1.000000000000000000, -0.000000000000000000 ) ) ;
#10986=VERTEX_POINT ( 'NONE', #11258 ) ;
#10988=VECTOR ( 'NONE', #2987, 1000.000000000000114 ) ;
#10989=FACE_BOUND ( 'NONE', #23552, .T. ) ;
#10991=EDGE_CURVE ( 'NONE', #1773, #38174, #12296, .T. ) ;
#10992=CARTESIAN_POINT ( 'NONE',  ( -48.47912675150885065, -189.7472609257535510, 6.938893903907228378E-15 ) ) ;
#10993=ORIENTED_EDGE ( 'NONE', *, *, #30751, .T. ) ;
#10994=ORIENTED_EDGE ( 'NONE', *, *, #48690, .F. ) ;
#10995=CARTESIAN_POINT ( 'NONE',  ( -118.4380981977755880, -175.3837268820161057, -102.3804074221059892 ) ) ;
#10997=DIRECTION ( 'NONE',  ( -0.000000000000000000, 1.000000000000000000, -0.000000000000000000 ) ) ;
#10998=DIRECTION ( 'NONE',  ( -0.000000000000000000, 1.000000000000000000, 0.000000000000000000 ) ) ;
#11000=ORIENTED_EDGE ( 'NONE', *, *, #28955, .T. ) ;
#11001=DIRECTION ( 'NONE',  ( 0.000000000000000000, 1.000000000000000000, 0.000000000000000000 ) ) ;
#11002=CARTESIAN_POINT ( 'NONE',  ( 33.25242634436025924, -189.7472609257535510, -94.57776286494160445 ) ) ;
#11003=ORIENTED_EDGE ( 'NONE', *, *, #11052, .F. ) ;
#11004=VECTOR ( 'NONE', #9064, 1000.000000000000114 ) ;
#11006=CARTESIAN_POINT ( 'NONE',  ( -120.2975302769383177, -177.1207230881787780, 102.3089288139533863 ) ) ;
#11007=ORIENTED_EDGE ( 'NONE', *, *, #2045, .F. ) ;
#11011=ORIENTED_EDGE ( 'NONE', *, *, #34614, .T. ) ;
#11012=DIRECTION ( 'NONE',  ( 0.000000000000000000, 0.000000000000000000, -1.000000000000000000 ) ) ;
#11013=FACE_OUTER_BOUND ( 'NONE', #3338, .T. ) ;
#11014=ORIENTED_EDGE ( 'NONE', *, *, #24124, .F. ) ;
#11015=ORIENTED_EDGE ( 'NONE', *, *, #16877, .F. ) ;
#11017=ORIENTED_EDGE ( 'NONE', *, *, #28579, .F. ) ;
#11018=DIRECTION ( 'NONE',  ( 0.000000000000000000, 0.000000000000000000, 1.000000000000000000 ) ) ;
#11019=DIRECTION ( 'NONE',  ( 0.000000000000000000, 0.000000000000000000, 1.000000000000000000 ) ) ;
#11020=AXIS2_PLACEMENT_3D ( 'NONE', #15868, #31878, #28180 ) ;
#11021=ORIENTED_EDGE ( 'NONE', *, *, #36288, .F. ) ;
#11022=DIRECTION ( 'NONE',  ( -0.000000000000000000, 1.000000000000000000, -0.000000000000000000 ) ) ;
#11024=FACE_OUTER_BOUND ( 'NONE', #27096, .T. ) ;
#11028=ADVANCED_FACE ( 'NONE', ( #31494 ), #15222, .T. ) ;
#11031=DIRECTION ( 'NONE',  ( -0.000000000000000000, 1.000000000000000000, 0.000000000000000000 ) ) ;
#11032=ORIENTED_EDGE ( 'NONE', *, *, #47437, .T. ) ;
#11033=EDGE_CURVE ( 'NONE', #28863, #10734, #51483, .T. ) ;
#11034=CARTESIAN_POINT ( 'NONE',  ( -173.1763543514842070, -183.6283474603465606, 8.694908215728872847 ) ) ;
#11035=DIRECTION ( 'NONE',  ( 0.000000000000000000, 0.000000000000000000, -1.000000000000000000 ) ) ;
#11038=LINE ( 'NONE', #15015, #38654 ) ;
#11040=ORIENTED_EDGE ( 'NONE', *, *, #22414, .T. ) ;
#11041=AXIS2_PLACEMENT_3D ( 'NONE', #17527, #29059, #32755 ) ;
#11044=LINE ( 'NONE', #39167, #24014 ) ;
#11045=CARTESIAN_POINT ( 'NONE',  ( -103.4012653778457462, -177.1207230881787780, -112.2878385610366649 ) ) ;
#11048=ORIENTED_EDGE ( 'NONE', *, *, #15998, .T. ) ;
#11052=EDGE_CURVE ( 'NONE', #47414, #6751, #3910, .T. ) ;
#11053=FACE_OUTER_BOUND ( 'NONE', #22633, .T. ) ;
#11057=CIRCLE ( 'NONE', #20286, 125.0000000000000000 ) ;
#11059=CARTESIAN_POINT ( 'NONE',  ( 58.48829670243887335, -183.6283474603465606, -64.67588669375807342 ) ) ;
#11062=DIRECTION ( 'NONE',  ( 0.000000000000000000, -0.000000000000000000, 1.000000000000000000 ) ) ;
#11065=CARTESIAN_POINT ( 'NONE',  ( -129.4514457347087557, -175.3837268820161057, 95.22858582633116953 ) ) ;
#11066=ORIENTED_EDGE ( 'NONE', *, *, #19737, .T. ) ;
#11067=ADVANCED_FACE ( 'NONE', ( #8369 ), #24392, .T. ) ;
#11071=AXIS2_PLACEMENT_3D ( 'NONE', #26276, #15237, #38625 ) ;
#11072=ORIENTED_EDGE ( 'NONE', *, *, #37619, .T. ) ;
#11075=VECTOR ( 'NONE', #27655, 1000.000000000000114 ) ;
#11076=CARTESIAN_POINT ( 'NONE',  ( -78.00521078983982193, -189.7472609257535510, 121.4627941443857111 ) ) ;
#11077=FACE_OUTER_BOUND ( 'NONE', #25365, .T. ) ;
#11078=ORIENTED_EDGE ( 'NONE', *, *, #28090, .F. ) ;
#11079=CIRCLE ( 'NONE', #47188, 125.0000000000000000 ) ;
#11081=VERTEX_POINT ( 'NONE', #45240 ) ;
#11084=ORIENTED_EDGE ( 'NONE', *, *, #34397, .T. ) ;
#11085=DIRECTION ( 'NONE',  ( 0.000000000000000000, 0.000000000000000000, -1.000000000000000000 ) ) ;
#11086=CARTESIAN_POINT ( 'NONE',  ( -158.0280232639029236, -193.5000000000000000, 60.19999396110247147 ) ) ;
#11087=ORIENTED_EDGE ( 'NONE', *, *, #30585, .T. ) ;
#11089=VECTOR ( 'NONE', #22117, 1000.000000000000000 ) ;
#11091=AXIS2_PLACEMENT_3D ( 'NONE', #26730, #30407, #5751 ) ;
#11093=CARTESIAN_POINT ( 'NONE',  ( -168.1141659785444915, -193.5000000000000000, -36.22785377503943494 ) ) ;
#11094=ORIENTED_EDGE ( 'NONE', *, *, #26470, .T. ) ;
#11095=VECTOR ( 'NONE', #33857, 1000.000000000000000 ) ;
#11097=CARTESIAN_POINT ( 'NONE',  ( 69.14211578623219623, -177.1207230881787780, 42.31126686685117733 ) ) ;
#11098=CARTESIAN_POINT ( 'NONE',  ( 24.63024857337165585, -177.1207230881787780, 101.3904297239426455 ) ) ;
#11099=EDGE_LOOP ( 'NONE', ( #37563, #25571, #47638, #32327 ) ) ;
#11101=ADVANCED_FACE ( 'NONE', ( #4501 ), #28398, .T. ) ;
#11102=CARTESIAN_POINT ( 'NONE',  ( -48.47912675150885065, -189.7472609257535510, 6.938893903907228378E-15 ) ) ;
#11103=CARTESIAN_POINT ( 'NONE',  ( 75.51463005422469621, -193.5000000000000000, -1.322128892811228251 ) ) ;
#11104=ADVANCED_FACE ( 'NONE', ( #20515 ), #542, .T. ) ;
#11109=ORIENTED_EDGE ( 'NONE', *, *, #4283, .F. ) ;
#11110=AXIS2_PLACEMENT_3D ( 'NONE', #39641, #44396, #35711 ) ;
#11111=VERTEX_POINT ( 'NONE', #813 ) ;
#11112=LINE ( 'NONE', #6926, #9811 ) ;
#11115=VECTOR ( 'NONE', #15801, 1000.000000000000000 ) ;
#11116=DIRECTION ( 'NONE',  ( -0.7378332790417333475, 0.000000000000000000, 0.6749830015182038956 ) ) ;
#11117=EDGE_LOOP ( 'NONE', ( #38271, #26151, #45224, #51145 ) ) ;
#11118=ORIENTED_EDGE ( 'NONE', *, *, #38741, .T. ) ;
#11119=EDGE_CURVE ( 'NONE', #44193, #32445, #21578, .T. ) ;
#11122=CARTESIAN_POINT ( 'NONE',  ( 24.63024857337166296, -183.6283474603465606, 101.3904297239426597 ) ) ;
#11123=CARTESIAN_POINT ( 'NONE',  ( -48.36085358058748085, -177.1207230881787780, -0.9929810960135100339 ) ) ;
#11125=LINE ( 'NONE', #35054, #4275 ) ;
#11127=ORIENTED_EDGE ( 'NONE', *, *, #36574, .F. ) ;
#11129=AXIS2_PLACEMENT_3D ( 'NONE', #32219, #48262, #9103 ) ;
#11130=VERTEX_POINT ( 'NONE', #12628 ) ;
#11131=LINE ( 'NONE', #6441, #38354 ) ;
#11132=VECTOR ( 'NONE', #43293, 1000.000000000000000 ) ;
#11133=DIRECTION ( 'NONE',  ( 0.2920567706369833760, 0.000000000000000000, -0.9564009842765202052 ) ) ;
#11134=VECTOR ( 'NONE', #1677, 1000.000000000000000 ) ;
#11135=CARTESIAN_POINT ( 'NONE',  ( 74.00867759460086859, -189.7472609257535510, 24.93467037017222410 ) ) ;
#11137=EDGE_LOOP ( 'NONE', ( #31718, #5986, #16957, #21885 ) ) ;
#11140=DIRECTION ( 'NONE',  ( 0.000000000000000000, 0.000000000000000000, 1.000000000000000000 ) ) ;
#11141=PLANE ( 'NONE',  #27369 ) ;
#11142=VERTEX_POINT ( 'NONE', #40479 ) ;
#11144=LINE ( 'NONE', #22987, #26447 ) ;
#11145=CARTESIAN_POINT ( 'NONE',  ( -118.4510020108455137, -193.5000000000000000, 103.5805805771131674 ) ) ;
#11147=AXIS2_PLACEMENT_3D ( 'NONE', #21714, #6470, #29839 ) ;
#11149=CARTESIAN_POINT ( 'NONE',  ( -171.4462109067799247, -193.5000000000000000, 15.97798378892250071 ) ) ;
#11151=DIRECTION ( 'NONE',  ( -0.000000000000000000, 1.000000000000000000, 0.000000000000000000 ) ) ;
#11152=AXIS2_PLACEMENT_3D ( 'NONE', #47136, #51104, #43176 ) ;
#11155=DIRECTION ( 'NONE',  ( 0.7575112421616236880, 0.000000000000000000, -0.6528221181905174975 ) ) ;
#11156=ORIENTED_EDGE ( 'NONE', *, *, #28500, .T. ) ;
#11157=ADVANCED_FACE ( 'NONE', ( #12371 ), #44447, .T. ) ;
#11161=CARTESIAN_POINT ( 'NONE',  ( 55.35935253854128746, -193.5000000000000000, 69.58857822035042773 ) ) ;
#11162=EDGE_CURVE ( 'NONE', #18433, #42344, #44974, .T. ) ;
#11163=VECTOR ( 'NONE', #300, 1000.000000000000000 ) ;
#11164=PLANE ( 'NONE',  #24057 ) ;
#11167=LINE ( 'NONE', #27190, #41234 ) ;
#11168=ORIENTED_EDGE ( 'NONE', *, *, #37505, .T. ) ;
#11169=AXIS2_PLACEMENT_3D ( 'NONE', #48682, #41290, #28941 ) ;
#11170=ADVANCED_FACE ( 'NONE', ( #12891 ), #29437, .T. ) ;
#11171=FACE_OUTER_BOUND ( 'NONE', #5708, .T. ) ;
#11172=CARTESIAN_POINT ( 'NONE',  ( 23.33927677392130917, -177.1207230881787780, -102.3089288139528747 ) ) ;
#11174=VERTEX_POINT ( 'NONE', #5029 ) ;
#11176=VECTOR ( 'NONE', #30621, 1000.000000000000114 ) ;
#11178=ORIENTED_EDGE ( 'NONE', *, *, #13550, .F. ) ;
#11179=EDGE_CURVE ( 'NONE', #19179, #46206, #34245, .T. ) ;
#11180=FACE_OUTER_BOUND ( 'NONE', #21346, .T. ) ;
#11183=DIRECTION ( 'NONE',  ( -0.000000000000000000, 1.000000000000000000, -0.000000000000000000 ) ) ;
#11185=ORIENTED_EDGE ( 'NONE', *, *, #37515, .F. ) ;
#11186=DIRECTION ( 'NONE',  ( -0.02963332782255633305, 0.000000000000000000, -0.9995608365087944591 ) ) ;
#11187=AXIS2_PLACEMENT_3D ( 'NONE', #34691, #47315, #11283 ) ;
#11188=EDGE_CURVE ( 'NONE', #41176, #24784, #21651, .T. ) ;
#11189=CARTESIAN_POINT ( 'NONE',  ( 60.90550954139437323, -189.7472609257535510, 60.49794494914088006 ) ) ;
#11190=DIRECTION ( 'NONE',  ( -0.000000000000000000, 1.000000000000000000, -0.000000000000000000 ) ) ;
#11191=ORIENTED_EDGE ( 'NONE', *, *, #4318, .F. ) ;
#11193=EDGE_CURVE ( 'NONE', #41557, #14780, #33645, .T. ) ;
#11194=AXIS2_PLACEMENT_3D ( 'NONE', #41836, #1887, #17924 ) ;
#11196=DIRECTION ( 'NONE',  ( -0.000000000000000000, 1.000000000000000000, -0.000000000000000000 ) ) ;
#11197=CARTESIAN_POINT ( 'NONE',  ( -146.0653709326077490, -193.5000000000000000, -78.11481899503411341 ) ) ;
#11198=CARTESIAN_POINT ( 'NONE',  ( -139.0630283577175987, -193.5000000000000000, -86.13684908212448477 ) ) ;
#11200=DIRECTION ( 'NONE',  ( 0.000000000000000000, 0.000000000000000000, 1.000000000000000000 ) ) ;
#11201=ORIENTED_EDGE ( 'NONE', *, *, #17617, .F. ) ;
#11203=DIRECTION ( 'NONE',  ( -0.000000000000000000, 1.000000000000000000, -0.000000000000000000 ) ) ;
#11204=ORIENTED_EDGE ( 'NONE', *, *, #38553, .F. ) ;
#11205=CARTESIAN_POINT ( 'NONE',  ( -1.578537454945990293, -177.1207230881787780, 114.7887733785766926 ) ) ;
#11206=EDGE_LOOP ( 'NONE', ( #8910, #13090, #30888, #38558 ) ) ;
#11207=VECTOR ( 'NONE', #51694, 1000.000000000000000 ) ;
#11210=CARTESIAN_POINT ( 'NONE',  ( -47.82630463331832971, -193.5000000000000000, -0.7575112421616121416 ) ) ;
#11211=DIRECTION ( 'NONE',  ( -0.000000000000000000, 1.000000000000000000, -0.000000000000000000 ) ) ;
#11213=ORIENTED_EDGE ( 'NONE', *, *, #21509, .F. ) ;
#11214=PLANE ( 'NONE',  #37607 ) ;
#11215=ORIENTED_EDGE ( 'NONE', *, *, #39035, .T. ) ;
#11216=EDGE_CURVE ( 'NONE', #33918, #21157, #41788, .T. ) ;
#11217=ORIENTED_EDGE ( 'NONE', *, *, #51911, .F. ) ;
#11218=DIRECTION ( 'NONE',  ( 0.000000000000000000, 0.000000000000000000, -1.000000000000000000 ) ) ;
#11219=DIRECTION ( 'NONE',  ( 0.000000000000000000, -1.000000000000000000, 0.000000000000000000 ) ) ;
#11220=LINE ( 'NONE', #35394, #36620 ) ;
#11221=AXIS2_PLACEMENT_3D ( 'NONE', #38316, #50674, #42784 ) ;
#11222=FACE_OUTER_BOUND ( 'NONE', #20239, .T. ) ;
#11225=FACE_OUTER_BOUND ( 'NONE', #30341, .T. ) ;
#11227=ORIENTED_EDGE ( 'NONE', *, *, #6087, .F. ) ;
#11229=FACE_OUTER_BOUND ( 'NONE', #7943, .T. ) ;
#11230=CIRCLE ( 'NONE', #26353, 125.0000000000000000 ) ;
#11232=EDGE_CURVE ( 'NONE', #29743, #37750, #34671, .T. ) ;
#11233=DIRECTION ( 'NONE',  ( 0.000000000000000000, 1.000000000000000000, -0.000000000000000000 ) ) ;
#11234=EDGE_LOOP ( 'NONE', ( #1218, #40669, #18444, #47972 ) ) ;
#11235=DIRECTION ( 'NONE',  ( 0.9995608365087942371, 0.000000000000000000, 0.02963332782256331357 ) ) ;
#11236=CARTESIAN_POINT ( 'NONE',  ( 57.12946453413545100, -193.5000000000000000, 66.87170886602000053 ) ) ;
#11237=ORIENTED_EDGE ( 'NONE', *, *, #11456, .T. ) ;
#11239=CIRCLE ( 'NONE', #10414, 125.0000000000000000 ) ;
#11240=ORIENTED_EDGE ( 'NONE', *, *, #44319, .T. ) ;
#11241=DIRECTION ( 'NONE',  ( 0.3482016354344059095, 0.000000000000000000, -0.9374196611341183427 ) ) ;
#11242=EDGE_CURVE ( 'NONE', #43197, #16239, #26735, .T. ) ;
#11243=FACE_BOUND ( 'NONE', #50206, .T. ) ;
#11245=EDGE_CURVE ( 'NONE', #12900, #34513, #25768, .T. ) ;
#11246=DIRECTION ( 'NONE',  ( 0.5829794791144650157, 0.000000000000000000, 0.8124868780056864193 ) ) ;
#11247=ORIENTED_EDGE ( 'NONE', *, *, #23092, .F. ) ;
#11248=EDGE_CURVE ( 'NONE', #41150, #10561, #26019, .T. ) ;
#11250=CARTESIAN_POINT ( 'NONE',  ( -169.0136227435421006, -193.5000000000000000, -33.11246405730811659 ) ) ;
#11253=AXIS2_PLACEMENT_3D ( 'NONE', #39902, #35989, #23627 ) ;
#11256=CARTESIAN_POINT ( 'NONE',  ( 75.12566530717464275, -193.5000000000000000, 18.62405380494841367 ) ) ;
#11257=EDGE_LOOP ( 'NONE', ( #49481, #40031, #39786, #26060 ) ) ;
#11258=CARTESIAN_POINT ( 'NONE',  ( -19.92568551777506869, -175.3837268820161057, -121.6951149130962904 ) ) ;
#11259=CARTESIAN_POINT ( 'NONE',  ( -147.0463339291296165, -183.6283474603465606, 76.87330921200147316 ) ) ;
#11260=ORIENTED_EDGE ( 'NONE', *, *, #27907, .T. ) ;
#11265=FACE_OUTER_BOUND ( 'NONE', #2520, .T. ) ;
#11267=CARTESIAN_POINT ( 'NONE',  ( -123.4791267515088435, -173.5000000000000284, 60.00000000000001421 ) ) ;
#11270=DIRECTION ( 'NONE',  ( -0.9785564922995060311, 0.000000000000000000, 0.2059786187410889424 ) ) ;
#11273=DIRECTION ( 'NONE',  ( 0.000000000000000000, -0.000000000000000000, 1.000000000000000000 ) ) ;
#11275=CARTESIAN_POINT ( 'NONE',  ( -168.4003408533108086, -193.5000000000000000, -35.26900067126609173 ) ) ;
#11276=LINE ( 'NONE', #42832, #40911 ) ;
#11277=DIRECTION ( 'NONE',  ( 0.000000000000000000, -0.000000000000000000, 1.000000000000000000 ) ) ;
#11279=ORIENTED_EDGE ( 'NONE', *, *, #23363, .F. ) ;
#11283=DIRECTION ( 'NONE',  ( 0.000000000000000000, 0.000000000000000000, -1.000000000000000000 ) ) ;
#11284=DIRECTION ( 'NONE',  ( -0.9473263538541876194, 0.000000000000000000, -0.3202698538628486746 ) ) ;
#11285=DIRECTION ( 'NONE',  ( 0.000000000000000000, 0.000000000000000000, -1.000000000000000000 ) ) ;
#11290=CIRCLE ( 'NONE', #42361, 125.0000000000000000 ) ;
#11291=PLANE ( 'NONE',  #22725 ) ;
#11292=DIRECTION ( 'NONE',  ( -0.000000000000000000, 1.000000000000000000, 0.000000000000000000 ) ) ;
#11293=ORIENTED_EDGE ( 'NONE', *, *, #39099, .F. ) ;
#11294=VERTEX_POINT ( 'NONE', #34421 ) ;
#11295=ORIENTED_EDGE ( 'NONE', *, *, #43639, .F. ) ;
#11296=VECTOR ( 'NONE', #43045, 1000.000000000000000 ) ;
#11298=DIRECTION ( 'NONE',  ( 0.000000000000000000, 0.000000000000000000, -1.000000000000000000 ) ) ;
#11299=DIRECTION ( 'NONE',  ( 0.000000000000000000, 0.000000000000000000, -1.000000000000000000 ) ) ;
#11300=CIRCLE ( 'NONE', #13871, 125.0000000000000000 ) ;
#11302=FACE_OUTER_BOUND ( 'NONE', #20053, .T. ) ;
#11303=DIRECTION ( 'NONE',  ( 0.000000000000000000, -0.000000000000000000, 1.000000000000000000 ) ) ;
#11304=ORIENTED_EDGE ( 'NONE', *, *, #17021, .T. ) ;
#11305=VECTOR ( 'NONE', #46323, 1000.000000000000000 ) ;
#11306=CARTESIAN_POINT ( 'NONE',  ( 50.70030191143631271, -177.1207230881787780, -76.08180419845319875 ) ) ;
#11307=EDGE_CURVE ( 'NONE', #42630, #12033, #46516, .T. ) ;
#11309=ORIENTED_EDGE ( 'NONE', *, *, #31059, .T. ) ;
#11310=ORIENTED_EDGE ( 'NONE', *, *, #41674, .F. ) ;
#11312=EDGE_CURVE ( 'NONE', #45236, #23329, #40990, .T. ) ;
#11314=VERTEX_POINT ( 'NONE', #33897 ) ;
#11315=DIRECTION ( 'NONE',  ( 0.000000000000000000, -1.000000000000000000, 0.000000000000000000 ) ) ;
#11316=CARTESIAN_POINT ( 'NONE',  ( 21.47984469475713354, -193.5000000000000000, 102.3804074221065292 ) ) ;
#11317=CARTESIAN_POINT ( 'NONE',  ( 71.18041382641612813, -175.3837268820161057, -32.52067927015754378 ) ) ;
#11319=ORIENTED_EDGE ( 'NONE', *, *, #16543, .T. ) ;
#11320=AXIS2_PLACEMENT_3D ( 'NONE', #45316, #33723, #30042 ) ;
#11321=CARTESIAN_POINT ( 'NONE',  ( 51.78320179844649118, -189.7472609257535510, -72.96212019587142095 ) ) ;
#11325=VERTEX_POINT ( 'NONE', #22606 ) ;
#11326=AXIS2_PLACEMENT_3D ( 'NONE', #6004, #2829, #18854 ) ;
#11330=DIRECTION ( 'NONE',  ( -0.000000000000000000, 1.000000000000000000, -0.000000000000000000 ) ) ;
#11331=CIRCLE ( 'NONE', #50825, 125.0000000000000000 ) ;
#11332=ORIENTED_EDGE ( 'NONE', *, *, #33687, .T. ) ;
#11334=CARTESIAN_POINT ( 'NONE',  ( -43.48323084606168720, -183.6283474603465606, 124.9001241957026167 ) ) ;
#11336=LINE ( 'NONE', #3456, #5512 ) ;
#11340=LINE ( 'NONE', #27112, #28263 ) ;
#11341=AXIS2_PLACEMENT_3D ( 'NONE', #41629, #21678, #26378 ) ;
#11342=LINE ( 'NONE', #46339, #487 ) ;
#11344=EDGE_CURVE ( 'NONE', #31867, #39679, #2374, .T. ) ;
#11345=LINE ( 'NONE', #27377, #24242 ) ;
#11346=AXIS2_PLACEMENT_3D ( 'NONE', #28121, #18972, #6881 ) ;
#11347=CARTESIAN_POINT ( 'NONE',  ( 73.80528149577284580, -175.3837268820161057, 25.91377046305969145 ) ) ;
#11350=DIRECTION ( 'NONE',  ( 0.3482016354343928088, 0.000000000000000000, 0.9374196611341231167 ) ) ;
#11351=ORIENTED_EDGE ( 'NONE', *, *, #8391, .F. ) ;
#11352=ADVANCED_FACE ( 'NONE', ( #10008 ), #2619, .T. ) ;
#11353=LINE ( 'NONE', #43435, #29831 ) ;
#11356=DIRECTION ( 'NONE',  ( 0.8455960035018234011, 0.000000000000000000, 0.5338233779647948429 ) ) ;
#11357=DIRECTION ( 'NONE',  ( 0.000000000000000000, -1.000000000000000000, 0.000000000000000000 ) ) ;
#11358=CARTESIAN_POINT ( 'NONE',  ( 76.48781641346532467, -175.3837268820161057, 2.874563619424056249 ) ) ;
#11359=CIRCLE ( 'NONE', #24807, 124.9999999999999858 ) ;
#11363=DIRECTION ( 'NONE',  ( -0.000000000000000000, 1.000000000000000000, 0.000000000000000000 ) ) ;
#11365=AXIS2_PLACEMENT_3D ( 'NONE', #6388, #26603, #47104 ) ;
#11366=AXIS2_PLACEMENT_3D ( 'NONE', #45511, #25790, #33430 ) ;
#11368=CARTESIAN_POINT ( 'NONE',  ( 44.58442300236217903, -183.6283474603465606, -81.94739446021065987 ) ) ;
#11369=FACE_OUTER_BOUND ( 'NONE', #13257, .T. ) ;
#11370=ORIENTED_EDGE ( 'NONE', *, *, #49702, .F. ) ;
#11371=VERTEX_POINT ( 'NONE', #15230 ) ;
#11372=PLANE ( 'NONE',  #10529 ) ;
#11373=VECTOR ( 'NONE', #37328, 1000.000000000000000 ) ;
#11374=ORIENTED_EDGE ( 'NONE', *, *, #2149, .T. ) ;
#11376=DIRECTION ( 'NONE',  ( 0.000000000000000000, 1.000000000000000000, -0.000000000000000000 ) ) ;
#11378=PLANE ( 'NONE',  #50442 ) ;
#11379=AXIS2_PLACEMENT_3D ( 'NONE', #27106, #8184, #32090 ) ;
#11381=ORIENTED_EDGE ( 'NONE', *, *, #23363, .T. ) ;
#11382=ORIENTED_EDGE ( 'NONE', *, *, #32604, .T. ) ;
#11384=VECTOR ( 'NONE', #48714, 999.9999999999998863 ) ;
#11385=CYLINDRICAL_SURFACE ( 'NONE', #10674, 125.0000000000000000 ) ;
#11389=CARTESIAN_POINT ( 'NONE',  ( 64.01121016852529522, -189.7472609257535510, -54.50618404930953176 ) ) ;
#11390=ORIENTED_EDGE ( 'NONE', *, *, #31050, .F. ) ;
#11392=DIRECTION ( 'NONE',  ( -0.000000000000000000, 1.000000000000000000, -0.000000000000000000 ) ) ;
#11393=CARTESIAN_POINT ( 'NONE',  ( 75.95066919219054569, -189.7472609257535510, -11.92584929509534852 ) ) ;
#11394=ORIENTED_EDGE ( 'NONE', *, *, #22257, .T. ) ;
#11395=VERTEX_POINT ( 'NONE', #7355 ) ;
#11397=ORIENTED_EDGE ( 'NONE', *, *, #31124, .F. ) ;
#11401=LINE ( 'NONE', #35844, #9779 ) ;
#11402=AXIS2_PLACEMENT_3D ( 'NONE', #16610, #32620, #17123 ) ;
#11405=LINE ( 'NONE', #38745, #46972 ) ;
#11408=DIRECTION ( 'NONE',  ( 0.000000000000000000, 0.000000000000000000, -1.000000000000000000 ) ) ;
#11409=ADVANCED_FACE ( 'NONE', ( #18906 ), #19674, .T. ) ;
#11411=DIRECTION ( 'NONE',  ( -0.000000000000000000, 1.000000000000000000, -0.000000000000000000 ) ) ;
#11412=ADVANCED_FACE ( 'NONE', ( #52026 ), #23616, .T. ) ;
#11413=VECTOR ( 'NONE', #44541, 1000.000000000000000 ) ;
#11414=LINE ( 'NONE', #15379, #48004 ) ;
#11416=CIRCLE ( 'NONE', #31559, 125.0000000000000000 ) ;
#11424=ORIENTED_EDGE ( 'NONE', *, *, #22331, .F. ) ;
#11425=VERTEX_POINT ( 'NONE', #22853 ) ;
#11429=EDGE_LOOP ( 'NONE', ( #18246, #25164, #3610, #16788 ) ) ;
#11430=CARTESIAN_POINT ( 'NONE',  ( -172.4195137048758681, -189.7472609257535510, -3.844569333772463793 ) ) ;
#11431=LINE ( 'NONE', #31411, #29338 ) ;
#11434=ORIENTED_EDGE ( 'NONE', *, *, #25960, .F. ) ;
#11436=DIRECTION ( 'NONE',  ( 0.000000000000000000, 0.000000000000000000, 1.000000000000000000 ) ) ;
#11439=CIRCLE ( 'NONE', #35791, 125.0000000000000000 ) ;
#11440=CARTESIAN_POINT ( 'NONE',  ( 62.59443091842027940, -183.6283474603465606, -57.33816169485142211 ) ) ;
#11443=ORIENTED_EDGE ( 'NONE', *, *, #7621, .F. ) ;
#11444=VERTEX_POINT ( 'NONE', #44112 ) ;
#11445=DIRECTION ( 'NONE',  ( 0.000000000000000000, 0.000000000000000000, -1.000000000000000000 ) ) ;
#11446=CARTESIAN_POINT ( 'NONE',  ( 62.43652093785069468, -183.6283474603465606, 55.44293326708522329 ) ) ;
#11447=AXIS2_PLACEMENT_3D ( 'NONE', #31378, #27440, #42951 ) ;
#11449=DIRECTION ( 'NONE',  ( -0.2635871660690783380, 0.000000000000000000, 0.9646355819083558547 ) ) ;
#11450=VECTOR ( 'NONE', #21267, 999.9999999999998863 ) ;
#11454=ORIENTED_EDGE ( 'NONE', *, *, #5633, .T. ) ;
#11456=EDGE_CURVE ( 'NONE', #35941, #33506, #40127, .T. ) ;
#11457=ADVANCED_FACE ( 'NONE', ( #11265 ), #34924, .T. ) ;
#11458=VECTOR ( 'NONE', #40085, 1000.000000000000114 ) ;
#11461=CARTESIAN_POINT ( 'NONE',  ( -164.6246685127424882, -193.5000000000000000, -46.20836643930983456 ) ) ;
#11463=DIRECTION ( 'NONE',  ( 0.000000000000000000, 0.000000000000000000, 1.000000000000000000 ) ) ;
#11465=ORIENTED_EDGE ( 'NONE', *, *, #25590, .F. ) ;
#11468=EDGE_CURVE ( 'NONE', #43678, #34495, #51757, .T. ) ;
#11469=PLANE ( 'NONE',  #14070 ) ;
#11470=CARTESIAN_POINT ( 'NONE',  ( 72.71365293123227502, -183.6283474603465606, -30.61552143554913030 ) ) ;
#11473=EDGE_CURVE ( 'NONE', #49349, #27618, #3139, .T. ) ;
#11477=ORIENTED_EDGE ( 'NONE', *, *, #32402, .F. ) ;
#11478=DIRECTION ( 'NONE',  ( -0.000000000000000000, 1.000000000000000000, 0.000000000000000000 ) ) ;
#11479=AXIS2_PLACEMENT_3D ( 'NONE', #51393, #35341, #11936 ) ;
#11480=DIRECTION ( 'NONE',  ( -0.08879589532293158394, 0.000000000000000000, -0.9960498426152172291 ) ) ;
#11482=EDGE_CURVE ( 'NONE', #48404, #19489, #11539, .T. ) ;
#11485=VECTOR ( 'NONE', #2206, 1000.000000000000341 ) ;
#11486=ADVANCED_FACE ( 'NONE', ( #27567 ), #43599, .T. ) ;
#11487=DIRECTION ( 'NONE',  ( -0.000000000000000000, 1.000000000000000000, 0.000000000000000000 ) ) ;
#11488=DIRECTION ( 'NONE',  ( 0.2348860457809775482, 0.000000000000000000, 0.9720229140804121926 ) ) ;
#11490=DIRECTION ( 'NONE',  ( -0.9027978299657477557, 0.000000000000000000, 0.4300652022765115712 ) ) ;
#11491=CARTESIAN_POINT ( 'NONE',  ( -47.78257572244586271, -189.7472609257535510, 0.7175072570443418174 ) ) ;
#11492=FACE_BOUND ( 'NONE', #31889, .T. ) ;
#11493=VERTEX_POINT ( 'NONE', #13362 ) ;
#11496=CARTESIAN_POINT ( 'NONE',  ( -47.78257572244585560, -183.6283474603465606, -0.7175072570443230546 ) ) ;
#11500=VERTEX_POINT ( 'NONE', #48598 ) ;
#11503=ORIENTED_EDGE ( 'NONE', *, *, #3518, .T. ) ;
#11504=EDGE_CURVE ( 'NONE', #45084, #46184, #36222, .T. ) ;
#11505=AXIS2_PLACEMENT_3D ( 'NONE', #18406, #18908, #6313 ) ;
#11506=DIRECTION ( 'NONE',  ( 0.000000000000000000, 1.000000000000000000, -0.000000000000000000 ) ) ;
#11507=FACE_BOUND ( 'NONE', #9380, .T. ) ;
#11508=CARTESIAN_POINT ( 'NONE',  ( -156.2577088867455473, -193.5000000000000000, -63.31490529818420754 ) ) ;
#11509=CARTESIAN_POINT ( 'NONE',  ( -162.3451783319732442, -183.6283474603465606, 51.57055649762783389 ) ) ;
#11511=ORIENTED_EDGE ( 'NONE', *, *, #50246, .F. ) ;
#11512=EDGE_CURVE ( 'NONE', #45026, #51761, #29376, .T. ) ;
#11514=VECTOR ( 'NONE', #36689, 1000.000000000000000 ) ;
#11515=AXIS2_PLACEMENT_3D ( 'NONE', #31018, #38392, #6853 ) ;
#11516=ORIENTED_EDGE ( 'NONE', *, *, #45011, .F. ) ;
#11518=VECTOR ( 'NONE', #42797, 1000.000000000000000 ) ;
#11519=EDGE_CURVE ( 'NONE', #48694, #29891, #47722, .T. ) ;
#11520=EDGE_CURVE ( 'NONE', #14560, #36987, #4091, .T. ) ;
#11521=EDGE_CURVE ( 'NONE', #4209, #17851, #42689, .T. ) ;
#11523=ADVANCED_FACE ( 'NONE', ( #49109 ), #17314, .F. ) ;
#11524=LINE ( 'NONE', #50974, #37356 ) ;
#11526=LINE ( 'NONE', #15754, #23341 ) ;
#11528=ORIENTED_EDGE ( 'NONE', *, *, #34594, .F. ) ;
#11531=EDGE_CURVE ( 'NONE', #39155, #47506, #36473, .T. ) ;
#11532=ADVANCED_FACE ( 'NONE', ( #5228 ), #13095, .T. ) ;
#11533=VECTOR ( 'NONE', #6520, 1000.000000000000000 ) ;
#11534=DIRECTION ( 'NONE',  ( 0.000000000000000000, 0.000000000000000000, 1.000000000000000000 ) ) ;
#11535=ORIENTED_EDGE ( 'NONE', *, *, #19546, .F. ) ;
#11537=EDGE_LOOP ( 'NONE', ( #25145, #40901, #37512, #20649 ) ) ;
#11538=AXIS2_PLACEMENT_3D ( 'NONE', #44912, #4704, #44123 ) ;
#11539=LINE ( 'NONE', #43343, #18353 ) ;
#11540=ORIENTED_EDGE ( 'NONE', *, *, #29236, .T. ) ;
#11541=EDGE_CURVE ( 'NONE', #30974, #40458, #24160, .T. ) ;
#11542=DIRECTION ( 'NONE',  ( 0.000000000000000000, 0.000000000000000000, 1.000000000000000000 ) ) ;
#11545=ADVANCED_FACE ( 'NONE', ( #40168 ), #48324, .T. ) ;
#11548=ORIENTED_EDGE ( 'NONE', *, *, #36200, .F. ) ;
#11549=PLANE ( 'NONE',  #16156 ) ;
#11551=EDGE_CURVE ( 'NONE', #1671, #37031, #48854, .T. ) ;
#11552=DIRECTION ( 'NONE',  ( 0.000000000000000000, 1.000000000000000000, 0.000000000000000000 ) ) ;
#11555=DIRECTION ( 'NONE',  ( 0.9151456172430210145, 0.000000000000000000, -0.4031234292879665171 ) ) ;
#11556=EDGE_CURVE ( 'NONE', #38180, #11142, #33336, .T. ) ;
#11557=EDGE_LOOP ( 'NONE', ( #38833, #5985, #35412, #12380, #28614, #11443 ) ) ;
#11560=DIRECTION ( 'NONE',  ( 0.000000000000000000, 0.000000000000000000, 1.000000000000000000 ) ) ;
#11561=EDGE_CURVE ( 'NONE', #41080, #1671, #41829, .T. ) ;
#11564=CIRCLE ( 'NONE', #44281, 125.0000000000000000 ) ;
#11565=VECTOR ( 'NONE', #47038, 1000.000000000000000 ) ;
#11567=DIRECTION ( 'NONE',  ( -0.000000000000000000, -1.000000000000000000, 0.000000000000000000 ) ) ;
#11568=CIRCLE ( 'NONE', #35086, 125.0000000000000000 ) ;
#11569=PLANE ( 'NONE',  #32811 ) ;
#11571=ORIENTED_EDGE ( 'NONE', *, *, #311, .F. ) ;
#11572=EDGE_LOOP ( 'NONE', ( #35040, #7139, #17604, #48088 ) ) ;
#11573=ORIENTED_EDGE ( 'NONE', *, *, #20922, .F. ) ;
#11574=EDGE_CURVE ( 'NONE', #21936, #46797, #754, .T. ) ;
#11575=VECTOR ( 'NONE', #6172, 1000.000000000000114 ) ;
#11577=CARTESIAN_POINT ( 'NONE',  ( 75.52097166332623601, -177.1207230881787780, -0.3215015308241039316 ) ) ;
#11579=CARTESIAN_POINT ( 'NONE',  ( -64.08700758308647494, -189.7472609257535510, -124.0217483183786840 ) ) ;
#11580=ORIENTED_EDGE ( 'NONE', *, *, #23885, .T. ) ;
#11586=CARTESIAN_POINT ( 'NONE',  ( -102.5006284722404502, -177.1207230881787780, -112.7238987608084386 ) ) ;
#11587=EDGE_CURVE ( 'NONE', #50750, #4539, #10798, .T. ) ;
#11588=EDGE_CURVE ( 'NONE', #41523, #41127, #49375, .T. ) ;
#11589=DIRECTION ( 'NONE',  ( 0.000000000000000000, -1.000000000000000000, -0.000000000000000000 ) ) ;
#11590=EDGE_LOOP ( 'NONE', ( #17710, #10427, #18377, #22184 ) ) ;
#11594=FACE_OUTER_BOUND ( 'NONE', #1911, .T. ) ;
#11595=DIRECTION ( 'NONE',  ( 0.000000000000000000, -1.000000000000000000, -0.000000000000000000 ) ) ;
#11599=CARTESIAN_POINT ( 'NONE',  ( -84.82349129030157542, -189.7472609257535510, -119.5996955107802364 ) ) ;
#11600=VERTEX_POINT ( 'NONE', #45181 ) ;
#11601=LINE ( 'NONE', #48383, #10471 ) ;
#11602=AXIS2_PLACEMENT_3D ( 'NONE', #7642, #7890, #23425 ) ;
#11606=LINE ( 'NONE', #7907, #27448 ) ;
#11609=VECTOR ( 'NONE', #18640, 1000.000000000000114 ) ;
#11610=CARTESIAN_POINT ( 'NONE',  ( -124.3803110981236273, -193.5000000000000000, -98.05618656931939370 ) ) ;
#11612=CARTESIAN_POINT ( 'NONE',  ( 47.04848625005566731, -177.1207230881787780, 80.61932246194658092 ) ) ;
#11614=EDGE_CURVE ( 'NONE', #42344, #14242, #45222, .T. ) ;
#11615=LINE ( 'NONE', #42642, #36674 ) ;
#11617=DIRECTION ( 'NONE',  ( 0.000000000000000000, -0.000000000000000000, 1.000000000000000000 ) ) ;
#11619=DIRECTION ( 'NONE',  ( -0.000000000000000000, 1.000000000000000000, -0.000000000000000000 ) ) ;
#11620=DIRECTION ( 'NONE',  ( 0.2348860457809842095, 0.000000000000000000, -0.9720229140804107493 ) ) ;
#11623=CARTESIAN_POINT ( 'NONE',  ( -137.2624501260119985, -183.6283474603465606, 87.99159897727967916 ) ) ;
#11625=FACE_OUTER_BOUND ( 'NONE', #30638, .T. ) ;
#11628=CARTESIAN_POINT ( 'NONE',  ( 62.59443091842029361, -177.1207230881787780, -57.33816169485141501 ) ) ;
#11631=LINE ( 'NONE', #27659, #25750 ) ;
#11632=CARTESIAN_POINT ( 'NONE',  ( 9.336583202542586335, -189.7472609257535510, 110.8257356506556164 ) ) ;
#11633=AXIS2_PLACEMENT_3D ( 'NONE', #29511, #9551, #45051 ) ;
#11634=AXIS2_PLACEMENT_3D ( 'NONE', #44888, #742, #5739 ) ;
#11636=DIRECTION ( 'NONE',  ( 0.000000000000000000, 0.000000000000000000, 1.000000000000000000 ) ) ;
#11637=DIRECTION ( 'NONE',  ( -0.000000000000000000, 1.000000000000000000, -0.000000000000000000 ) ) ;
#11640=AXIS2_PLACEMENT_3D ( 'NONE', #39874, #47284, #15748 ) ;
#11641=VERTEX_POINT ( 'NONE', #14652 ) ;
#11642=CARTESIAN_POINT ( 'NONE',  ( 73.09196206113300320, -177.1207230881787780, 29.07697310430963356 ) ) ;
#11643=LINE ( 'NONE', #4272, #35490 ) ;
#11646=VERTEX_POINT ( 'NONE', #13612 ) ;
#11647=DIRECTION ( 'NONE',  ( -0.000000000000000000, 1.000000000000000000, -0.000000000000000000 ) ) ;
#11648=ORIENTED_EDGE ( 'NONE', *, *, #41508, .F. ) ;
#11649=CARTESIAN_POINT ( 'NONE',  ( 52.16997862029128186, -175.3837268820161057, 72.42760398749086903 ) ) ;
#11650=PLANE ( 'NONE',  #17484 ) ;
#11653=FACE_OUTER_BOUND ( 'NONE', #9632, .T. ) ;
#11654=VERTEX_POINT ( 'NONE', #45428 ) ;
#11655=ORIENTED_EDGE ( 'NONE', *, *, #28834, .T. ) ;
#11659=DIRECTION ( 'NONE',  ( -0.000000000000000000, 1.000000000000000000, -0.000000000000000000 ) ) ;
#11661=CARTESIAN_POINT ( 'NONE',  ( -172.0602536473422504, -189.7472609257535510, -10.18383939837523222 ) ) ;
#11669=DIRECTION ( 'NONE',  ( -0.000000000000000000, 1.000000000000000000, -0.000000000000000000 ) ) ;
#11670=LINE ( 'NONE', #48200, #16606 ) ;
#11672=VERTEX_POINT ( 'NONE', #5992 ) ;
#11673=ADVANCED_FACE ( 'NONE', ( #2564 ), #25447, .T. ) ;
#11677=DIRECTION ( 'NONE',  ( 0.000000000000000000, 0.000000000000000000, 1.000000000000000000 ) ) ;
#11680=EDGE_LOOP ( 'NONE', ( #29426, #10637, #40109, #33762 ) ) ;
#11681=CARTESIAN_POINT ( 'NONE',  ( -48.98765787015805984, -183.6283474603465606, -0.8610436117673551104 ) ) ;
#11683=LINE ( 'NONE', #51387, #40444 ) ;
#11684=ORIENTED_EDGE ( 'NONE', *, *, #28090, .T. ) ;
#11685=DIRECTION ( 'NONE',  ( 0.5586467658036476935, 0.000000000000000000, 0.8294056854502049880 ) ) ;
#11687=PLANE ( 'NONE',  #44144 ) ;
#11688=FACE_OUTER_BOUND ( 'NONE', #32652, .T. ) ;
#11693=ORIENTED_EDGE ( 'NONE', *, *, #42798, .F. ) ;
#11694=LINE ( 'NONE', #43751, #34537 ) ;
#11696=EDGE_CURVE ( 'NONE', #47995, #20677, #33842, .T. ) ;
#11697=ORIENTED_EDGE ( 'NONE', *, *, #1794, .T. ) ;
#11698=FACE_OUTER_BOUND ( 'NONE', #18303, .T. ) ;
#11699=ADVANCED_FACE ( 'NONE', ( #9943 ), #22014, .T. ) ;
#11701=ORIENTED_EDGE ( 'NONE', *, *, #43053, .F. ) ;
#11702=AXIS2_PLACEMENT_3D ( 'NONE', #20624, #36658, #28751 ) ;
#11706=CARTESIAN_POINT ( 'NONE',  ( 72.71365293123227502, -193.5000000000000000, -30.61552143554913030 ) ) ;
#11707=CARTESIAN_POINT ( 'NONE',  ( -63.09433862318514485, -189.7472609257535510, -124.1426420773539547 ) ) ;
#11710=CARTESIAN_POINT ( 'NONE',  ( 48.69345348225014902, -193.5000000000000000, -78.62880929222872339 ) ) ;
#11711=DIRECTION ( 'NONE',  ( 0.7765238627180482966, 0.000000000000000000, -0.6300878435817038881 ) ) ;
#11714=EDGE_CURVE ( 'NONE', #41052, #28664, #38519, .T. ) ;
#11716=DIRECTION ( 'NONE',  ( 0.000000000000000000, -1.000000000000000000, 0.000000000000000000 ) ) ;
#11717=CARTESIAN_POINT ( 'NONE',  ( 14.37129481273059106, -189.7472609257535510, -108.0501018472328241 ) ) ;
#11719=CARTESIAN_POINT ( 'NONE',  ( 73.09196206113300320, -193.5000000000000000, 29.07697310430963356 ) ) ;
#11720=CYLINDRICAL_SURFACE ( 'NONE', #2660, 125.0000000000000000 ) ;
#11723=AXIS2_PLACEMENT_3D ( 'NONE', #21482, #13068, #29095 ) ;
#11724=CARTESIAN_POINT ( 'NONE',  ( 10.22625775207003507, -183.6283474603465606, -109.2239789693433352 ) ) ;
#11725=ORIENTED_EDGE ( 'NONE', *, *, #5972, .F. ) ;
#11728=ORIENTED_EDGE ( 'NONE', *, *, #19726, .T. ) ;
#11730=EDGE_CURVE ( 'NONE', #51354, #10952, #38036, .T. ) ;
#11732=CARTESIAN_POINT ( 'NONE',  ( -140.8230258362169707, -189.7472609257535510, 84.24728067916045404 ) ) ;
#11733=DIRECTION ( 'NONE',  ( -0.000000000000000000, 1.000000000000000000, -0.000000000000000000 ) ) ;
#11735=DIRECTION ( 'NONE',  ( 0.000000000000000000, -1.000000000000000000, -0.000000000000000000 ) ) ;
#11739=AXIS2_PLACEMENT_3D ( 'NONE', #18442, #34457, #50505 ) ;
#11744=EDGE_LOOP ( 'NONE', ( #12567, #9037, #979, #2371 ) ) ;
#11745=CARTESIAN_POINT ( 'NONE',  ( -87.88805327685028601, -177.1207230881787780, 117.5715283571807106 ) ) ;
#11746=DIRECTION ( 'NONE',  ( 0.000000000000000000, 1.000000000000000000, 0.000000000000000000 ) ) ;
#11747=FACE_BOUND ( 'NONE', #46562, .T. ) ;
#11749=CARTESIAN_POINT ( 'NONE',  ( -95.72791768350677444, -183.6283474603465606, -115.7261930397105516 ) ) ;
#11751=EDGE_CURVE ( 'NONE', #14590, #33364, #39338, .T. ) ;
#11754=DIRECTION ( 'NONE',  ( -0.9890401873221623674, 0.000000000000000000, -0.1476465640024917925 ) ) ;
#11757=CIRCLE ( 'NONE', #18492, 125.0000000000000000 ) ;
#11758=FACE_OUTER_BOUND ( 'NONE', #20580, .T. ) ;
#11759=FACE_BOUND ( 'NONE', #21814, .T. ) ;
#11761=ORIENTED_EDGE ( 'NONE', *, *, #40119, .T. ) ;
#11762=EDGE_CURVE ( 'NONE', #28114, #17942, #26465, .T. ) ;
#11764=VERTEX_POINT ( 'NONE', #10186 ) ;
#11765=EDGE_CURVE ( 'NONE', #10187, #20971, #17576, .T. ) ;
#11767=DIRECTION ( 'NONE',  ( 0.000000000000000000, 0.000000000000000000, -1.000000000000000000 ) ) ;
#11773=EDGE_CURVE ( 'NONE', #6751, #3432, #38564, .T. ) ;
#11775=VERTEX_POINT ( 'NONE', #35645 ) ;
#11776=CARTESIAN_POINT ( 'NONE',  ( 60.02977459919873837, -175.3837268820161057, 60.01515274641010222 ) ) ;
#11777=CARTESIAN_POINT ( 'NONE',  ( -11.80936624585915418, -175.3837268820161057, -119.5003291395395735 ) ) ;
#11778=VERTEX_POINT ( 'NONE', #23822 ) ;
#11779=ORIENTED_EDGE ( 'NONE', *, *, #25017, .T. ) ;
#11780=LINE ( 'NONE', #15226, #42417 ) ;
#11781=ORIENTED_EDGE ( 'NONE', *, *, #10383, .T. ) ;
#11784=CARTESIAN_POINT ( 'NONE',  ( 64.29733702426837283, -175.3837268820161057, 53.91167979418564471 ) ) ;
#11785=ORIENTED_EDGE ( 'NONE', *, *, #28260, .T. ) ;
#11786=CARTESIAN_POINT ( 'NONE',  ( -48.47912675150885065, -189.7472609257535510, 6.938893903907228378E-15 ) ) ;
#11787=LINE ( 'NONE', #477, #27502 ) ;
#11789=AXIS2_PLACEMENT_3D ( 'NONE', #38921, #51047, #3697 ) ;
#11791=DIRECTION ( 'NONE',  ( 0.000000000000000000, -1.000000000000000000, -0.000000000000000000 ) ) ;
#11793=PLANE ( 'NONE',  #48878 ) ;
#11794=CARTESIAN_POINT ( 'NONE',  ( -47.70260288879081401, -189.7472609257535510, 0.6300878435817218737 ) ) ;
#11795=DIRECTION ( 'NONE',  ( 0.000000000000000000, 0.000000000000000000, 1.000000000000000000 ) ) ;
#11797=DIRECTION ( 'NONE',  ( 0.000000000000000000, 0.000000000000000000, -1.000000000000000000 ) ) ;
#11798=FACE_OUTER_BOUND ( 'NONE', #6545, .T. ) ;
#11800=DIRECTION ( 'NONE',  ( 0.000000000000000000, -0.000000000000000000, 1.000000000000000000 ) ) ;
#11803=DIRECTION ( 'NONE',  ( 0.000000000000000000, -1.000000000000000000, 0.000000000000000000 ) ) ;
#11804=EDGE_LOOP ( 'NONE', ( #8049, #1182, #16860, #29598 ) ) ;
#11807=ADVANCED_FACE ( 'NONE', ( #51967 ), #6773, .T. ) ;
#11810=EDGE_CURVE ( 'NONE', #32088, #26105, #34862, .T. ) ;
#11811=ORIENTED_EDGE ( 'NONE', *, *, #31586, .T. ) ;
#11812=EDGE_CURVE ( 'NONE', #18768, #29891, #31714, .T. ) ;
#11813=VERTEX_POINT ( 'NONE', #3337 ) ;
#11814=VERTEX_POINT ( 'NONE', #15700 ) ;
#11815=ADVANCED_FACE ( 'NONE', ( #46981 ), #14926, .F. ) ;
#11816=DIRECTION ( 'NONE',  ( -0.000000000000000000, 1.000000000000000000, -0.000000000000000000 ) ) ;
#11817=ADVANCED_FACE ( 'NONE', ( #22794 ), #47758, .F. ) ;
#11819=CARTESIAN_POINT ( 'NONE',  ( -104.8182102393454045, -189.7472609257535510, 111.5836353223472912 ) ) ;
#11820=CARTESIAN_POINT ( 'NONE',  ( 24.15597040328004752, -177.1207230881787780, -101.7307360698543874 ) ) ;
#11821=AXIS2_PLACEMENT_3D ( 'NONE', #26812, #40368, #8339 ) ;
#11823=EDGE_CURVE ( 'NONE', #28285, #28167, #26984, .T. ) ;
#11825=EDGE_CURVE ( 'NONE', #32738, #49319, #43017, .T. ) ;
#11826=CIRCLE ( 'NONE', #21905, 125.0000000000000000 ) ;
#11827=ORIENTED_EDGE ( 'NONE', *, *, #19070, .T. ) ;
#11828=VERTEX_POINT ( 'NONE', #3860 ) ;
#11831=DIRECTION ( 'NONE',  ( -0.6965510290630033685, 0.000000000000000000, 0.7175072570443249420 ) ) ;
#11832=EDGE_CURVE ( 'NONE', #37933, #23116, #39833, .T. ) ;
#11833=ORIENTED_EDGE ( 'NONE', *, *, #30567, .F. ) ;
#11834=EDGE_CURVE ( 'NONE', #4203, #37758, #19370, .T. ) ;
#11835=ADVANCED_FACE ( 'NONE', ( #10707 ), #51695, .T. ) ;
#11836=DIRECTION ( 'NONE',  ( -0.000000000000000000, 1.000000000000000000, -0.000000000000000000 ) ) ;
#11837=FACE_OUTER_BOUND ( 'NONE', #4971, .T. ) ;
#11838=CARTESIAN_POINT ( 'NONE',  ( 141.7825277784304205, -213.5000000000000000, -9.999999999999987566 ) ) ;
#11839=DIRECTION ( 'NONE',  ( -0.000000000000000000, 1.000000000000000000, -0.000000000000000000 ) ) ;
#11840=EDGE_LOOP ( 'NONE', ( #8776, #9321, #7825, #22044 ) ) ;
#11841=AXIS2_PLACEMENT_3D ( 'NONE', #16648, #32655, #8733 ) ;
#11843=EDGE_LOOP ( 'NONE', ( #1006, #7772, #36955, #33585 ) ) ;
#11846=DIRECTION ( 'NONE',  ( -0.000000000000000000, 1.000000000000000000, -0.000000000000000000 ) ) ;
#11849=CARTESIAN_POINT ( 'NONE',  ( -15.24927435600542047, -183.6283474603465606, 120.5021863277719092 ) ) ;
#11850=EDGE_CURVE ( 'NONE', #21083, #17362, #39577, .T. ) ;
#11851=ORIENTED_EDGE ( 'NONE', *, *, #50939, .F. ) ;
#11852=CARTESIAN_POINT ( 'NONE',  ( -81.47409310123204307, -183.6283474603465606, -119.5301634136912554 ) ) ;
#11853=DIRECTION ( 'NONE',  ( 0.000000000000000000, 0.000000000000000000, 1.000000000000000000 ) ) ;
#11854=ORIENTED_EDGE ( 'NONE', *, *, #42382, .T. ) ;
#11855=CARTESIAN_POINT ( 'NONE',  ( -172.5669052183642123, -193.5000000000000000, 15.07392567185553567 ) ) ;
#11857=AXIS2_PLACEMENT_3D ( 'NONE', #42453, #6479, #22507 ) ;
#11858=DIRECTION ( 'NONE',  ( -0.000000000000000000, 1.000000000000000000, 0.000000000000000000 ) ) ;
#11860=DIRECTION ( 'NONE',  ( 0.000000000000000000, 1.000000000000000000, -0.000000000000000000 ) ) ;
#11861=AXIS2_PLACEMENT_3D ( 'NONE', #26410, #29841, #45892 ) ;
#11866=VERTEX_POINT ( 'NONE', #30661 ) ;
#11867=PLANE ( 'NONE',  #33210 ) ;
#11868=DIRECTION ( 'NONE',  ( 0.000000000000000000, 1.000000000000000000, -0.000000000000000000 ) ) ;
#11870=CARTESIAN_POINT ( 'NONE',  ( -48.82732838694323618, -193.5000000000000000, -0.9374196611341184537 ) ) ;
#11874=AXIS2_PLACEMENT_3D ( 'NONE', #4460, #48624, #28618 ) ;
#11876=FACE_OUTER_BOUND ( 'NONE', #30073, .T. ) ;
#11878=VECTOR ( 'NONE', #26188, 999.9999999999998863 ) ;
#11879=LINE ( 'NONE', #35801, #12726 ) ;
#11881=CARTESIAN_POINT ( 'NONE',  ( -107.6930423737362190, -177.1207230881787780, 110.0850225811110761 ) ) ;
#11882=ORIENTED_EDGE ( 'NONE', *, *, #18590, .F. ) ;
#11883=VERTEX_POINT ( 'NONE', #8056 ) ;
#11884=DIRECTION ( 'NONE',  ( -0.000000000000000000, 1.000000000000000000, -0.000000000000000000 ) ) ;
#11885=CARTESIAN_POINT ( 'NONE',  ( -127.4665351220365892, -193.5000000000000000, -96.88131563365291754 ) ) ;
#11886=ORIENTED_EDGE ( 'NONE', *, *, #30191, .T. ) ;
#11887=ORIENTED_EDGE ( 'NONE', *, *, #8949, .T. ) ;
#11888=EDGE_CURVE ( 'NONE', #48776, #2708, #32220, .T. ) ;
#11889=ORIENTED_EDGE ( 'NONE', *, *, #19193, .T. ) ;
#11892=VECTOR ( 'NONE', #28657, 1000.000000000000000 ) ;
#11893=CARTESIAN_POINT ( 'NONE',  ( -171.9838957966129840, -189.7472609257535510, 19.27620354518724355 ) ) ;
#11894=PLANE ( 'NONE',  #49299 ) ;
#11895=AXIS2_PLACEMENT_3D ( 'NONE', #15074, #50806, #51323 ) ;
#11896=ORIENTED_EDGE ( 'NONE', *, *, #32929, .T. ) ;
#11898=EDGE_CURVE ( 'NONE', #8967, #35821, #49042, .T. ) ;
#11902=CARTESIAN_POINT ( 'NONE',  ( 15.23368049493606335, -175.3837268820161057, -107.5438431188757562 ) ) ;
#11904=DIRECTION ( 'NONE',  ( -0.000000000000000000, 1.000000000000000000, -0.000000000000000000 ) ) ;
#11905=CARTESIAN_POINT ( 'NONE',  ( 29.40217425202905233, -177.1207230881787780, -96.49160960477045990 ) ) ;
#11907=PLANE ( 'NONE',  #13786 ) ;
#11908=LINE ( 'NONE', #28708, #8956 ) ;
#11909=CARTESIAN_POINT ( 'NONE',  ( -22.44626007086657182, -177.1207230881787780, 122.2591094863196730 ) ) ;
#11910=LINE ( 'NONE', #20066, #10613 ) ;
#11914=VECTOR ( 'NONE', #30264, 1000.000000000000000 ) ;
#11921=LINE ( 'NONE', #14867, #6940 ) ;
#11922=DIRECTION ( 'NONE',  ( -0.8294056854502090959, 0.000000000000000000, 0.5586467658036415873 ) ) ;
#11926=DIRECTION ( 'NONE',  ( 0.000000000000000000, 1.000000000000000000, -0.000000000000000000 ) ) ;
#11927=ORIENTED_EDGE ( 'NONE', *, *, #3146, .T. ) ;
#11929=CARTESIAN_POINT ( 'NONE',  ( 7.859956736328458149, -193.5000000000000000, -111.5836353223468649 ) ) ;
#11935=EDGE_CURVE ( 'NONE', #12462, #47079, #37201, .T. ) ;
#11936=DIRECTION ( 'NONE',  ( 0.000000000000000000, -0.000000000000000000, 1.000000000000000000 ) ) ;
#11937=VECTOR ( 'NONE', #19705, 1000.000000000000000 ) ;
#11940=ORIENTED_EDGE ( 'NONE', *, *, #20326, .F. ) ;
#11941=ORIENTED_EDGE ( 'NONE', *, *, #472, .T. ) ;
#11944=EDGE_LOOP ( 'NONE', ( #596, #9595, #10897, #26076 ) ) ;
#11947=CIRCLE ( 'NONE', #13652, 125.0000000000000000 ) ;
#11950=DIRECTION ( 'NONE',  ( 0.000000000000000000, 1.000000000000000000, -0.000000000000000000 ) ) ;
#11952=VECTOR ( 'NONE', #41094, 1000.000000000000000 ) ;
#11953=ORIENTED_EDGE ( 'NONE', *, *, #31220, .F. ) ;
#11954=DIRECTION ( 'NONE',  ( 0.000000000000000000, -1.000000000000000000, 0.000000000000000000 ) ) ;
#11956=EDGE_CURVE ( 'NONE', #9002, #30647, #7468, .T. ) ;
#11959=DIRECTION ( 'NONE',  ( -0.000000000000000000, 1.000000000000000000, -0.000000000000000000 ) ) ;
#11961=LINE ( 'NONE', #23541, #11458 ) ;
#11962=ORIENTED_EDGE ( 'NONE', *, *, #44287, .T. ) ;
#11965=ORIENTED_EDGE ( 'NONE', *, *, #35748, .T. ) ;
#11966=DIRECTION ( 'NONE',  ( -0.6965510290630033685, 0.000000000000000000, 0.7175072570443249420 ) ) ;
#11968=CARTESIAN_POINT ( 'NONE',  ( -56.71246971489870958, -189.7472609257535510, -124.7285535218267682 ) ) ;
#11971=VECTOR ( 'NONE', #23827, 1000.000000000000000 ) ;
#11972=ORIENTED_EDGE ( 'NONE', *, *, #27480, .F. ) ;
#11974=PLANE ( 'NONE',  #3957 ) ;
#11975=VERTEX_POINT ( 'NONE', #21180 ) ;
#11977=VERTEX_POINT ( 'NONE', #159 ) ;
#11978=ORIENTED_EDGE ( 'NONE', *, *, #36487, .F. ) ;
#11979=DIRECTION ( 'NONE',  ( 0.000000000000000000, 1.000000000000000000, -0.000000000000000000 ) ) ;
#11981=CARTESIAN_POINT ( 'NONE',  ( -2.700932609314990351, -183.6283474603465606, -116.3157639405751667 ) ) ;
#11984=LINE ( 'NONE', #28282, #2383 ) ;
#11985=VECTOR ( 'NONE', #47835, 1000.000000000000227 ) ;
#11987=VECTOR ( 'NONE', #50688, 1000.000000000000000 ) ;
#11989=EDGE_LOOP ( 'NONE', ( #35512, #45663, #3391, #31984 ) ) ;
#11990=FACE_OUTER_BOUND ( 'NONE', #18184, .T. ) ;
#11992=CARTESIAN_POINT ( 'NONE',  ( -31.30262293407084329, -177.1207230881787780, -123.8142468240611436 ) ) ;
#11994=FACE_OUTER_BOUND ( 'NONE', #1083, .T. ) ;
#11995=FACE_OUTER_BOUND ( 'NONE', #37248, .T. ) ;
#11996=DIRECTION ( 'NONE',  ( 0.000000000000000000, 0.000000000000000000, 1.000000000000000000 ) ) ;
#11998=VECTOR ( 'NONE', #28305, 1000.000000000000000 ) ;
#12002=FACE_BOUND ( 'NONE', #26074, .T. ) ;
#12006=AXIS2_PLACEMENT_3D ( 'NONE', #7226, #43216, #19063 ) ;
#12008=ORIENTED_EDGE ( 'NONE', *, *, #46389, .T. ) ;
#12010=ORIENTED_EDGE ( 'NONE', *, *, #34594, .T. ) ;
#12012=DIRECTION ( 'NONE',  ( 0.000000000000000000, -0.000000000000000000, 1.000000000000000000 ) ) ;
#12013=FACE_BOUND ( 'NONE', #33867, .T. ) ;
#12014=CARTESIAN_POINT ( 'NONE',  ( -172.3973245609188041, -175.3837268820161057, 4.503971736581616092 ) ) ;
#12015=ORIENTED_EDGE ( 'NONE', *, *, #37586, .T. ) ;
#12016=EDGE_CURVE ( 'NONE', #44148, #43156, #42727, .T. ) ;
#12018=CIRCLE ( 'NONE', #41406, 125.0000000000000000 ) ;
#12019=ORIENTED_EDGE ( 'NONE', *, *, #49762, .T. ) ;
#12020=ORIENTED_EDGE ( 'NONE', *, *, #7699, .T. ) ;
#12021=LINE ( 'NONE', #36198, #4083 ) ;
#12022=VECTOR ( 'NONE', #1258, 1000.000000000000000 ) ;
#12023=ORIENTED_EDGE ( 'NONE', *, *, #28860, .T. ) ;
#12024=CARTESIAN_POINT ( 'NONE',  ( -49.45768324380835423, -177.1207230881787780, -0.2059786187411025149 ) ) ;
#12025=DIRECTION ( 'NONE',  ( -0.1768902751225733261, 0.000000000000000000, 0.9842305779475966077 ) ) ;
#12026=CARTESIAN_POINT ( 'NONE',  ( -47.55243714407701816, -193.5000000000000000, -0.3758275821142288420 ) ) ;
#12031=VERTEX_POINT ( 'NONE', #413 ) ;
#12032=DIRECTION ( 'NONE',  ( 0.000000000000000000, -1.000000000000000000, 0.000000000000000000 ) ) ;
#12033=VERTEX_POINT ( 'NONE', #8823 ) ;
#12034=DIRECTION ( 'NONE',  ( 0.000000000000000000, -0.000000000000000000, 1.000000000000000000 ) ) ;
#12035=VECTOR ( 'NONE', #2834, 1000.000000000000000 ) ;
#12037=ADVANCED_FACE ( 'NONE', ( #48786 ), #28781, .F. ) ;
#12038=EDGE_CURVE ( 'NONE', #12735, #20792, #49464, .T. ) ;
#12039=DIRECTION ( 'NONE',  ( 0.000000000000000000, 1.000000000000000000, 0.000000000000000000 ) ) ;
#12043=EDGE_LOOP ( 'NONE', ( #8945, #48752 ) ) ;
#12044=VECTOR ( 'NONE', #35145, 1000.000000000000000 ) ;
#12047=FACE_OUTER_BOUND ( 'NONE', #25787, .T. ) ;
#12049=DIRECTION ( 'NONE',  ( -0.000000000000000000, 1.000000000000000000, -0.000000000000000000 ) ) ;
#12050=CARTESIAN_POINT ( 'NONE',  ( 53.56330073376472711, -175.3837268820161057, 72.19655804062050208 ) ) ;
#12051=DIRECTION ( 'NONE',  ( 0.000000000000000000, -0.000000000000000000, 1.000000000000000000 ) ) ;
#12052=ORIENTED_EDGE ( 'NONE', *, *, #40206, .T. ) ;
#12054=EDGE_CURVE ( 'NONE', #19748, #6892, #4907, .T. ) ;
#12055=CIRCLE ( 'NONE', #44825, 125.0000000000000000 ) ;
#12056=DIRECTION ( 'NONE',  ( 0.9890401873221654760, 0.000000000000000000, -0.1476465640024710868 ) ) ;
#12057=CARTESIAN_POINT ( 'NONE',  ( -173.4724443937511751, -183.6283474603465606, 1.292495564989516454 ) ) ;
#12059=FACE_OUTER_BOUND ( 'NONE', #46392, .T. ) ;
#12060=ORIENTED_EDGE ( 'NONE', *, *, #16947, .F. ) ;
#12062=CARTESIAN_POINT ( 'NONE',  ( -7.515176836080581957, -183.6283474603465606, 117.0391155081705250 ) ) ;
#12065=ORIENTED_EDGE ( 'NONE', *, *, #7953, .F. ) ;
#12066=EDGE_LOOP ( 'NONE', ( #3846, #8341, #37130, #25197 ) ) ;
#12069=LINE ( 'NONE', #11045, #41313 ) ;
#12072=VECTOR ( 'NONE', #16757, 1000.000000000000000 ) ;
#12073=EDGE_LOOP ( 'NONE', ( #36097, #32914, #17637, #22500 ) ) ;
#12075=DIRECTION ( 'NONE',  ( 0.000000000000000000, 0.000000000000000000, -1.000000000000000000 ) ) ;
#12076=EDGE_LOOP ( 'NONE', ( #23781, #15142, #49073, #44626 ) ) ;
#12077=AXIS2_PLACEMENT_3D ( 'NONE', #48552, #28292, #36706 ) ;
#12078=ORIENTED_EDGE ( 'NONE', *, *, #42271, .T. ) ;
#12083=ORIENTED_EDGE ( 'NONE', *, *, #44217, .T. ) ;
#12086=DIRECTION ( 'NONE',  ( -0.2920567706369694982, 0.000000000000000000, -0.9564009842765243130 ) ) ;
#12088=ORIENTED_EDGE ( 'NONE', *, *, #44871, .F. ) ;
#12089=CARTESIAN_POINT ( 'NONE',  ( 18.49541618049843095, -193.5000000000000000, 105.5434062319798159 ) ) ;
#12092=ORIENTED_EDGE ( 'NONE', *, *, #31985, .F. ) ;
#12094=ADVANCED_FACE ( 'NONE', ( #21709 ), #29318, .T. ) ;
#12096=CARTESIAN_POINT ( 'NONE',  ( 20.93410174202488250, -189.7472609257535510, -102.7511748916624441 ) ) ;
#12099=LINE ( 'NONE', #40742, #36592 ) ;
#12100=EDGE_LOOP ( 'NONE', ( #23294, #37526, #27968, #49 ) ) ;
#12102=CARTESIAN_POINT ( 'NONE',  ( -159.8192355313504720, -193.5000000000000000, -56.81883646197830018 ) ) ;
#12103=CARTESIAN_POINT ( 'NONE',  ( 70.68712318874649725, -177.1207230881787780, -37.74128873232327663 ) ) ;
#12105=ADVANCED_FACE ( 'NONE', ( #21954 ), #25630, .F. ) ;
#12107=DIRECTION ( 'NONE',  ( 0.9890401873221633666, 0.000000000000000000, 0.1476465640024850756 ) ) ;
#12108=EDGE_CURVE ( 'NONE', #44462, #3230, #14334, .T. ) ;
#12109=AXIS2_PLACEMENT_3D ( 'NONE', #31563, #16069, #48121 ) ;
#12110=DIRECTION ( 'NONE',  ( 0.000000000000000000, 0.000000000000000000, 1.000000000000000000 ) ) ;
#12111=VECTOR ( 'NONE', #48162, 1000.000000000000000 ) ;
#12113=PLANE ( 'NONE',  #17545 ) ;
#12114=EDGE_CURVE ( 'NONE', #39091, #46272, #25386, .T. ) ;
#12116=AXIS2_PLACEMENT_3D ( 'NONE', #15079, #21914, #34503 ) ;
#12117=ADVANCED_FACE ( 'NONE', ( #5420 ), #50089, .T. ) ;
#12118=ORIENTED_EDGE ( 'NONE', *, *, #28607, .F. ) ;
#12120=ORIENTED_EDGE ( 'NONE', *, *, #29167, .F. ) ;
#12121=EDGE_CURVE ( 'NONE', #30190, #41581, #22211, .T. ) ;
#12122=DIRECTION ( 'NONE',  ( 0.000000000000000000, 0.000000000000000000, 1.000000000000000000 ) ) ;
#12123=LINE ( 'NONE', #44202, #5136 ) ;
#12124=EDGE_CURVE ( 'NONE', #1492, #12178, #50344, .T. ) ;
#12126=CARTESIAN_POINT ( 'NONE',  ( -48.47912675150885065, -183.6283474603465606, 6.938893903907228378E-15 ) ) ;
#12129=DIRECTION ( 'NONE',  ( -0.000000000000000000, 1.000000000000000000, -0.000000000000000000 ) ) ;
#12130=CARTESIAN_POINT ( 'NONE',  ( 44.30815888362531041, -193.5000000000000000, 83.75869879877569701 ) ) ;
#12132=CARTESIAN_POINT ( 'NONE',  ( -167.9436818089035057, -193.5000000000000000, 36.78613984830044359 ) ) ;
#12133=VERTEX_POINT ( 'NONE', #21437 ) ;
#12134=VERTEX_POINT ( 'NONE', #26404 ) ;
#12137=DIRECTION ( 'NONE',  ( 0.000000000000000000, 1.000000000000000000, 0.000000000000000000 ) ) ;
#12139=ORIENTED_EDGE ( 'NONE', *, *, #6428, .F. ) ;
#12140=AXIS2_PLACEMENT_3D ( 'NONE', #24668, #49633, #5495 ) ;
#12141=VERTEX_POINT ( 'NONE', #1724 ) ;
#12144=VECTOR ( 'NONE', #19129, 1000.000000000000114 ) ;
#12145=PLANE ( 'NONE',  #17760 ) ;
#12146=LINE ( 'NONE', #12671, #1458 ) ;
#12147=ORIENTED_EDGE ( 'NONE', *, *, #6223, .T. ) ;
#12148=EDGE_LOOP ( 'NONE', ( #35936, #41715, #1060, #38091 ) ) ;
#12152=LINE ( 'NONE', #16381, #40027 ) ;
#12153=CYLINDRICAL_SURFACE ( 'NONE', #47041, 125.0000000000000000 ) ;
#12154=CARTESIAN_POINT ( 'NONE',  ( 2.669657140899374337, -175.3837268820161057, 114.0561348912355868 ) ) ;
#12157=AXIS2_PLACEMENT_3D ( 'NONE', #8289, #11954, #1164 ) ;
#12159=ORIENTED_EDGE ( 'NONE', *, *, #6704, .F. ) ;
#12160=CARTESIAN_POINT ( 'NONE',  ( -99.62791064391781504, -175.3837268820161057, -114.0561348912352315 ) ) ;
#12166=DIRECTION ( 'NONE',  ( -0.7378332790417333475, 0.000000000000000000, 0.6749830015182038956 ) ) ;
#12167=DIRECTION ( 'NONE',  ( -0.000000000000000000, 1.000000000000000000, -0.000000000000000000 ) ) ;
#12168=EDGE_CURVE ( 'NONE', #50038, #1430, #48628, .T. ) ;
#12169=CIRCLE ( 'NONE', #433, 125.0000000000000000 ) ;
#12170=ORIENTED_EDGE ( 'NONE', *, *, #26239, .T. ) ;
#12172=EDGE_LOOP ( 'NONE', ( #7504, #6318, #8631, #12015 ) ) ;
#12173=CARTESIAN_POINT ( 'NONE',  ( -48.47912675150885065, -183.6283474603465606, 6.938893903907228378E-15 ) ) ;
#12174=LINE ( 'NONE', #51896, #20795 ) ;
#12176=CARTESIAN_POINT ( 'NONE',  ( 32.99469856375238663, -193.5000000000000000, 94.79987230212020677 ) ) ;
#12178=VERTEX_POINT ( 'NONE', #3013 ) ;
#12182=CARTESIAN_POINT ( 'NONE',  ( 67.29303306501927295, -193.5000000000000000, 47.13604789772129777 ) ) ;
#12185=CARTESIAN_POINT ( 'NONE',  ( 67.64905612629584652, -193.5000000000000000, -43.47841891815122750 ) ) ;
#12190=VECTOR ( 'NONE', #26343, 1000.000000000000000 ) ;
#12193=CARTESIAN_POINT ( 'NONE',  ( -118.9967449635792320, -175.3837268820161057, -103.2098131075562009 ) ) ;
#12195=CARTESIAN_POINT ( 'NONE',  ( -49.38192458147459263, -175.3837268820161057, -0.4300652022765235616 ) ) ;
#12197=VECTOR ( 'NONE', #37227, 1000.000000000000114 ) ;
#12198=EDGE_CURVE ( 'NONE', #40491, #42583, #30971, .T. ) ;
#12199=ORIENTED_EDGE ( 'NONE', *, *, #40056, .T. ) ;
#12201=VERTEX_POINT ( 'NONE', #19561 ) ;
#12203=AXIS2_PLACEMENT_3D ( 'NONE', #9157, #38025, #29625 ) ;
#12204=CARTESIAN_POINT ( 'NONE',  ( 30.05499637021956261, -183.6283474603465606, -97.24912084693207248 ) ) ;
#12206=VERTEX_POINT ( 'NONE', #2752 ) ;
#12209=PLANE ( 'NONE',  #21283 ) ;
#12210=VECTOR ( 'NONE', #18526, 1000.000000000000114 ) ;
#12212=AXIS2_PLACEMENT_3D ( 'NONE', #48843, #49095, #44379 ) ;
#12213=DIRECTION ( 'NONE',  ( 0.000000000000000000, -1.000000000000000000, 0.000000000000000000 ) ) ;
#12214=ORIENTED_EDGE ( 'NONE', *, *, #29740, .F. ) ;
#12215=CARTESIAN_POINT ( 'NONE',  ( -171.9740864388383557, -175.3837268820161057, -11.18012358327901623 ) ) ;
#12216=DIRECTION ( 'NONE',  ( -0.9890401873221623674, 0.000000000000000000, -0.1476465640024917925 ) ) ;
#12217=ORIENTED_EDGE ( 'NONE', *, *, #29494, .F. ) ;
#12219=CARTESIAN_POINT ( 'NONE',  ( -92.43312097795268301, -193.5000000000000000, -115.9484881370935483 ) ) ;
#12220=CARTESIAN_POINT ( 'NONE',  ( -71.40672220061269115, -189.7472609257535510, -122.8793122007208751 ) ) ;
#12221=PLANE ( 'NONE',  #2254 ) ;
#12223=EDGE_LOOP ( 'NONE', ( #40513, #33703, #39484, #29358 ) ) ;
#12224=ORIENTED_EDGE ( 'NONE', *, *, #17626, .F. ) ;
#12225=DIRECTION ( 'NONE',  ( 0.6965510290629932655, 0.000000000000000000, 0.7175072570443347120 ) ) ;
#12227=AXIS2_PLACEMENT_3D ( 'NONE', #43867, #7867, #32290 ) ;
#12232=ORIENTED_EDGE ( 'NONE', *, *, #24380, .T. ) ;
#12233=VECTOR ( 'NONE', #51836, 1000.000000000000114 ) ;
#12234=EDGE_CURVE ( 'NONE', #6625, #49882, #51381, .T. ) ;
#12235=EDGE_CURVE ( 'NONE', #33039, #9410, #11405, .T. ) ;
#12236=ORIENTED_EDGE ( 'NONE', *, *, #2219, .T. ) ;
#12237=PLANE ( 'NONE',  #25637 ) ;
#12240=DIRECTION ( 'NONE',  ( -0.000000000000000000, 1.000000000000000000, -0.000000000000000000 ) ) ;
#12241=AXIS2_PLACEMENT_3D ( 'NONE', #5551, #34423, #49688 ) ;
#12242=FACE_OUTER_BOUND ( 'NONE', #25160, .T. ) ;
#12245=DIRECTION ( 'NONE',  ( -0.000000000000000000, 1.000000000000000000, -0.000000000000000000 ) ) ;
#12246=VERTEX_POINT ( 'NONE', #6963 ) ;
#12248=VECTOR ( 'NONE', #50473, 1000.000000000000000 ) ;
#12249=VERTEX_POINT ( 'NONE', #43486 ) ;
#12252=DIRECTION ( 'NONE',  ( 0.2920567706369764371, 0.000000000000000000, -0.9564009842765223146 ) ) ;
#12253=ADVANCED_FACE ( 'NONE', ( #23263 ), #26679, .F. ) ;
#12254=DIRECTION ( 'NONE',  ( -0.6965510290629932655, 0.000000000000000000, -0.7175072570443347120 ) ) ;
#12255=DIRECTION ( 'NONE',  ( -0.000000000000000000, 1.000000000000000000, -0.000000000000000000 ) ) ;
#12257=PLANE ( 'NONE',  #12077 ) ;
#12258=PLANE ( 'NONE',  #211 ) ;
#12259=ORIENTED_EDGE ( 'NONE', *, *, #30585, .F. ) ;
#12260=CARTESIAN_POINT ( 'NONE',  ( -48.47912675150885065, -175.3837268820161057, 6.938893903907228378E-15 ) ) ;
#12261=CARTESIAN_POINT ( 'NONE',  ( 74.00867759460086859, -189.7472609257535510, 24.93467037017223120 ) ) ;
#12262=EDGE_CURVE ( 'NONE', #17784, #8540, #8323, .T. ) ;
#12263=FACE_BOUND ( 'NONE', #12937, .T. ) ;
#12264=VERTEX_POINT ( 'NONE', #7490 ) ;
#12266=VECTOR ( 'NONE', #6535, 1000.000000000000227 ) ;
#12267=CARTESIAN_POINT ( 'NONE',  ( -169.7849785064911998, -189.7472609257535510, -25.70779184431772890 ) ) ;
#12269=AXIS2_PLACEMENT_3D ( 'NONE', #30149, #10173, #13866 ) ;
#12274=DIRECTION ( 'NONE',  ( 0.000000000000000000, -1.000000000000000000, 0.000000000000000000 ) ) ;
#12278=PLANE ( 'NONE',  #23735 ) ;
#12280=VECTOR ( 'NONE', #9629, 1000.000000000000114 ) ;
#12282=VECTOR ( 'NONE', #27816, 1000.000000000000000 ) ;
#12285=ORIENTED_EDGE ( 'NONE', *, *, #42983, .T. ) ;
#12290=PLANE ( 'NONE',  #44403 ) ;
#12295=ORIENTED_EDGE ( 'NONE', *, *, #31823, .F. ) ;
#12296=LINE ( 'NONE', #19934, #6569 ) ;
#12298=EDGE_LOOP ( 'NONE', ( #8953, #9081, #20333, #24532 ) ) ;
#12299=VECTOR ( 'NONE', #51149, 1000.000000000000000 ) ;
#12300=EDGE_LOOP ( 'NONE', ( #38066, #35533, #35110, #26174 ) ) ;
#12301=AXIS2_PLACEMENT_3D ( 'NONE', #48738, #44791, #4322 ) ;
#12303=ORIENTED_EDGE ( 'NONE', *, *, #4493, .T. ) ;
#12304=CARTESIAN_POINT ( 'NONE',  ( -134.9506378406916554, -193.5000000000000000, 90.26448786734091811 ) ) ;
#12305=ORIENTED_EDGE ( 'NONE', *, *, #48652, .F. ) ;
#12306=CIRCLE ( 'NONE', #42546, 125.0000000000000000 ) ;
#12309=DIRECTION ( 'NONE',  ( -0.8455960035018234011, 0.000000000000000000, -0.5338233779647948429 ) ) ;
#12310=CARTESIAN_POINT ( 'NONE',  ( -59.81005805956450416, -193.5000000000000000, -123.4817304940906268 ) ) ;
#12311=ORIENTED_EDGE ( 'NONE', *, *, #44940, .F. ) ;
#12312=EDGE_LOOP ( 'NONE', ( #40167, #41245, #14869, #17478 ) ) ;
#12313=DIRECTION ( 'NONE',  ( -0.000000000000000000, 1.000000000000000000, -0.000000000000000000 ) ) ;
#12314=VECTOR ( 'NONE', #43772, 1000.000000000000114 ) ;
#12317=EDGE_CURVE ( 'NONE', #9325, #3589, #35170, .T. ) ;
#12318=DIRECTION ( 'NONE',  ( 0.8610436117673585521, 0.000000000000000000, -0.5085311186492154079 ) ) ;
#12319=FACE_OUTER_BOUND ( 'NONE', #15380, .T. ) ;
#12323=PLANE ( 'NONE',  #41495 ) ;
#12325=CIRCLE ( 'NONE', #32439, 125.0000000000000000 ) ;
#12330=ORIENTED_EDGE ( 'NONE', *, *, #10288, .F. ) ;
#12332=DIRECTION ( 'NONE',  ( 0.000000000000000000, 1.000000000000000000, -0.000000000000000000 ) ) ;
#12336=EDGE_LOOP ( 'NONE', ( #43344, #6042, #38213, #6065 ) ) ;
#12337=AXIS2_PLACEMENT_3D ( 'NONE', #16201, #12240, #28277 ) ;
#12338=DIRECTION ( 'NONE',  ( -0.08879589532294572540, 0.000000000000000000, 0.9960498426152160079 ) ) ;
#12340=DIRECTION ( 'NONE',  ( 0.000000000000000000, 0.000000000000000000, -1.000000000000000000 ) ) ;
#12341=CARTESIAN_POINT ( 'NONE',  ( -149.5539421794694022, -193.5000000000000000, 73.54509967498655953 ) ) ;
#12342=CARTESIAN_POINT ( 'NONE',  ( 76.51419089073347379, -183.6283474603465606, -1.292495564988661139 ) ) ;
#12343=CIRCLE ( 'NONE', #27426, 125.0000000000000000 ) ;
#12344=ORIENTED_EDGE ( 'NONE', *, *, #4131, .F. ) ;
#12345=ADVANCED_FACE ( 'NONE', ( #38506 ), #2501, .T. ) ;
#12347=ORIENTED_EDGE ( 'NONE', *, *, #51838, .T. ) ;
#12350=VECTOR ( 'NONE', #50841, 1000.000000000000000 ) ;
#12353=CARTESIAN_POINT ( 'NONE',  ( -165.2002711502080672, -193.5000000000000000, 44.73448837594998651 ) ) ;
#12355=EDGE_CURVE ( 'NONE', #47028, #46485, #50861, .T. ) ;
#12356=VECTOR ( 'NONE', #38977, 1000.000000000000000 ) ;
#12358=AXIS2_PLACEMENT_3D ( 'NONE', #27092, #30525, #16062 ) ;
#12359=PLANE ( 'NONE',  #14241 ) ;
#12360=CARTESIAN_POINT ( 'NONE',  ( -48.47912675150885065, -183.6283474603465606, 6.938893903907228378E-15 ) ) ;
#12362=PLANE ( 'NONE',  #10677 ) ;
#12364=EDGE_CURVE ( 'NONE', #19780, #19801, #32660, .T. ) ;
#12365=CARTESIAN_POINT ( 'NONE',  ( -48.88225018079680950, -193.5000000000000000, -0.9151456172430169067 ) ) ;
#12369=ORIENTED_EDGE ( 'NONE', *, *, #50286, .F. ) ;
#12370=DIRECTION ( 'NONE',  ( 0.9564009842765202052, 0.000000000000000000, 0.2920567706369833760 ) ) ;
#12371=FACE_OUTER_BOUND ( 'NONE', #21186, .T. ) ;
#12372=CARTESIAN_POINT ( 'NONE',  ( -48.47912675150885065, -175.3837268820161057, 6.938893903907228378E-15 ) ) ;
#12373=CARTESIAN_POINT ( 'NONE',  ( -48.47912675150885065, -183.6283474603465606, 6.938893903907228378E-15 ) ) ;
#12374=ORIENTED_EDGE ( 'NONE', *, *, #27187, .T. ) ;
#12375=CARTESIAN_POINT ( 'NONE',  ( -98.10897907742933910, -193.5000000000000000, 114.7252272087849434 ) ) ;
#12378=AXIS2_PLACEMENT_3D ( 'NONE', #17317, #17578, #41204 ) ;
#12379=DIRECTION ( 'NONE',  ( 0.9929810960135161402, 0.000000000000000000, 0.1182731709213730997 ) ) ;
#12380=ORIENTED_EDGE ( 'NONE', *, *, #24644, .T. ) ;
#12383=AXIS2_PLACEMENT_3D ( 'NONE', #21931, #13528, #21410 ) ;
#12386=DIRECTION ( 'NONE',  ( 0.000000000000000000, 0.000000000000000000, 1.000000000000000000 ) ) ;
#12390=VERTEX_POINT ( 'NONE', #8974 ) ;
#12391=CIRCLE ( 'NONE', #41783, 15.00000000000000000 ) ;
#12392=DIRECTION ( 'NONE',  ( -0.000000000000000000, 1.000000000000000000, 0.000000000000000000 ) ) ;
#12393=PLANE ( 'NONE',  #47108 ) ;
#12394=AXIS2_PLACEMENT_3D ( 'NONE', #26677, #2246, #2499 ) ;
#12395=PLANE ( 'NONE',  #34459 ) ;
#12396=CYLINDRICAL_SURFACE ( 'NONE', #35649, 125.0000000000000000 ) ;
#12397=DIRECTION ( 'NONE',  ( 0.000000000000000000, 0.000000000000000000, 1.000000000000000000 ) ) ;
#12398=DIRECTION ( 'NONE',  ( 0.000000000000000000, 0.000000000000000000, -1.000000000000000000 ) ) ;
#12400=CARTESIAN_POINT ( 'NONE',  ( -160.4991136281923900, -189.7472609257535510, 53.17445600718621534 ) ) ;
#12402=DIRECTION ( 'NONE',  ( 0.000000000000000000, -0.000000000000000000, -1.000000000000000000 ) ) ;
#12403=ORIENTED_EDGE ( 'NONE', *, *, #46073, .F. ) ;
#12404=VERTEX_POINT ( 'NONE', #5301 ) ;
#12405=EDGE_CURVE ( 'NONE', #16314, #29108, #44419, .T. ) ;
#12406=EDGE_CURVE ( 'NONE', #2342, #117, #17399, .T. ) ;
#12407=CARTESIAN_POINT ( 'NONE',  ( -141.5426765053792622, -193.5000000000000000, 81.94739446021135620 ) ) ;
#12408=CARTESIAN_POINT ( 'NONE',  ( 68.79964045138288498, -177.1207230881787780, 43.25148278810710423 ) ) ;
#12410=VECTOR ( 'NONE', #2686, 1000.000000000000114 ) ;
#12411=AXIS2_PLACEMENT_3D ( 'NONE', #1782, #22273, #41463 ) ;
#12412=ORIENTED_EDGE ( 'NONE', *, *, #32403, .T. ) ;
#12413=ORIENTED_EDGE ( 'NONE', *, *, #9568, .T. ) ;
#12414=FACE_OUTER_BOUND ( 'NONE', #17285, .T. ) ;
#12415=ADVANCED_FACE ( 'NONE', ( #1340 ), #9240, .T. ) ;
#12417=EDGE_CURVE ( 'NONE', #34708, #2282, #17652, .T. ) ;
#12418=CARTESIAN_POINT ( 'NONE',  ( -48.82732838694323618, -189.7472609257535510, -0.9374196611341184537 ) ) ;
#12419=DIRECTION ( 'NONE',  ( -0.000000000000000000, 1.000000000000000000, -0.000000000000000000 ) ) ;
#12421=ORIENTED_EDGE ( 'NONE', *, *, #45281, .F. ) ;
#12423=EDGE_LOOP ( 'NONE', ( #33888, #23106, #659, #45042 ) ) ;
#12424=LINE ( 'NONE', #16123, #43434 ) ;
#12425=DIRECTION ( 'NONE',  ( -0.000000000000000000, 1.000000000000000000, -0.000000000000000000 ) ) ;
#12426=CIRCLE ( 'NONE', #22543, 125.0000000000000000 ) ;
#12427=DIRECTION ( 'NONE',  ( 0.000000000000000000, -1.000000000000000000, 0.000000000000000000 ) ) ;
#12428=ORIENTED_EDGE ( 'NONE', *, *, #18830, .T. ) ;
#12430=CARTESIAN_POINT ( 'NONE',  ( -91.49662025983754177, -193.5000000000000000, -116.2991637277475405 ) ) ;
#12431=DIRECTION ( 'NONE',  ( -0.000000000000000000, 1.000000000000000000, 0.000000000000000000 ) ) ;
#12432=EDGE_LOOP ( 'NONE', ( #28015, #41305, #47065, #23922 ) ) ;
#12436=CARTESIAN_POINT ( 'NONE',  ( -48.47912675150885065, -175.3837268820161057, 1.000000000000006883 ) ) ;
#12438=ORIENTED_EDGE ( 'NONE', *, *, #30997, .F. ) ;
#12440=EDGE_LOOP ( 'NONE', ( #38611, #34712, #35125, #1955 ) ) ;
#12444=DIRECTION ( 'NONE',  ( 0.000000000000000000, 0.000000000000000000, 1.000000000000000000 ) ) ;
#12445=DIRECTION ( 'NONE',  ( 0.9842305779475954974, 0.000000000000000000, 0.1768902751225803205 ) ) ;
#12446=VERTEX_POINT ( 'NONE', #99 ) ;
#12447=DIRECTION ( 'NONE',  ( -0.6965510290629982615, 0.000000000000000000, 0.7175072570443298270 ) ) ;
#12449=ORIENTED_EDGE ( 'NONE', *, *, #26435, .T. ) ;
#12450=PLANE ( 'NONE',  #13990 ) ;
#12451=ORIENTED_EDGE ( 'NONE', *, *, #42216, .F. ) ;
#12453=AXIS2_PLACEMENT_3D ( 'NONE', #36363, #27960, #15633 ) ;
#12454=VECTOR ( 'NONE', #18128, 1000.000000000000000 ) ;
#12455=CARTESIAN_POINT ( 'NONE',  ( 70.91428087927182844, -193.5000000000000000, -33.48461921608518566 ) ) ;
#12457=VECTOR ( 'NONE', #31821, 1000.000000000000000 ) ;
#12458=CARTESIAN_POINT ( 'NONE',  ( -118.9967449635792462, -189.7472609257535510, -103.2098131075562009 ) ) ;
#12459=DIRECTION ( 'NONE',  ( -0.000000000000000000, 1.000000000000000000, -0.000000000000000000 ) ) ;
#12460=DIRECTION ( 'NONE',  ( -0.000000000000000000, 1.000000000000000000, -0.000000000000000000 ) ) ;
#12462=VERTEX_POINT ( 'NONE', #5042 ) ;
#12464=EDGE_LOOP ( 'NONE', ( #43768, #2535, #17177, #43949 ) ) ;
#12465=EDGE_CURVE ( 'NONE', #22595, #13288, #34354, .T. ) ;
#12466=ORIENTED_EDGE ( 'NONE', *, *, #17663, .F. ) ;
#12467=VECTOR ( 'NONE', #11196, 1000.000000000000000 ) ;
#12470=VERTEX_POINT ( 'NONE', #1074 ) ;
#12471=EDGE_CURVE ( 'NONE', #47778, #50157, #18424, .T. ) ;
#12472=ADVANCED_FACE ( 'NONE', ( #4060 ), #33135, .F. ) ;
#12474=ADVANCED_FACE ( 'NONE', ( #36104 ), #16146, .T. ) ;
#12475=DIRECTION ( 'NONE',  ( 0.6528221181905119463, 0.000000000000000000, 0.7575112421616284619 ) ) ;
#12476=ADVANCED_FACE ( 'NONE', ( #37337 ), #41531, .T. ) ;
#12478=AXIS2_PLACEMENT_3D ( 'NONE', #39065, #3075, #43275 ) ;
#12479=DIRECTION ( 'NONE',  ( 0.000000000000000000, 0.000000000000000000, -1.000000000000000000 ) ) ;
#12480=CARTESIAN_POINT ( 'NONE',  ( 61.22907552172956969, -177.1207230881787780, -57.79541595648220920 ) ) ;
#12481=VERTEX_POINT ( 'NONE', #34182 ) ;
#12482=DIRECTION ( 'NONE',  ( 0.000000000000000000, 0.000000000000000000, -1.000000000000000000 ) ) ;
#12483=ADVANCED_FACE ( 'NONE', ( #38631 ), #42307, .T. ) ;
#12484=ORIENTED_EDGE ( 'NONE', *, *, #32333, .F. ) ;
#12485=CARTESIAN_POINT ( 'NONE',  ( -47.50057025920934706, -175.3837268820161057, -0.2059786187410884151 ) ) ;
#12486=CARTESIAN_POINT ( 'NONE',  ( -33.86391487983341619, -193.5000000000000000, 124.1426420773540542 ) ) ;
#12487=EDGE_CURVE ( 'NONE', #51223, #10121, #2474, .T. ) ;
#12489=DIRECTION ( 'NONE',  ( 0.000000000000000000, 1.000000000000000000, -0.000000000000000000 ) ) ;
#12491=ORIENTED_EDGE ( 'NONE', *, *, #31655, .T. ) ;
#12493=VERTEX_POINT ( 'NONE', #1853 ) ;
#12494=DIRECTION ( 'NONE',  ( 0.9646355819083614058, 0.000000000000000000, -0.2635871660690581320 ) ) ;
#12496=AXIS2_PLACEMENT_3D ( 'NONE', #48405, #11860, #12386 ) ;
#12498=VECTOR ( 'NONE', #6025, 1000.000000000000000 ) ;
#12499=CARTESIAN_POINT ( 'NONE',  ( -48.77118352214581876, -177.1207230881787780, -0.9564009842765195391 ) ) ;
#12501=FACE_OUTER_BOUND ( 'NONE', #8435, .T. ) ;
#12502=EDGE_LOOP ( 'NONE', ( #12746, #41271, #37915, #38586 ) ) ;
#12505=EDGE_CURVE ( 'NONE', #7989, #18995, #29979, .T. ) ;
#12506=VERTEX_POINT ( 'NONE', #26543 ) ;
#12507=CARTESIAN_POINT ( 'NONE',  ( 44.58442300236217903, -177.1207230881787780, -81.94739446021065987 ) ) ;
#12508=ORIENTED_EDGE ( 'NONE', *, *, #37557, .F. ) ;
#12509=CIRCLE ( 'NONE', #37690, 125.0000000000000000 ) ;
#12510=CARTESIAN_POINT ( 'NONE',  ( 11.66870402553033692, -193.5000000000000000, 108.4360005853211248 ) ) ;
#12512=CARTESIAN_POINT ( 'NONE',  ( -41.30311180514221547, -189.7472609257535510, 123.7921848946937899 ) ) ;
#12514=CARTESIAN_POINT ( 'NONE',  ( -148.6149069237406195, -183.6283474603465606, -74.81861753132355375 ) ) ;
#12517=DIRECTION ( 'NONE',  ( 0.000000000000000000, 0.000000000000000000, 1.000000000000000000 ) ) ;
#12518=ORIENTED_EDGE ( 'NONE', *, *, #37514, .T. ) ;
#12519=ADVANCED_FACE ( 'NONE', ( #42581 ), #46032, .T. ) ;
#12521=EDGE_CURVE ( 'NONE', #33429, #36752, #6597, .T. ) ;
#12522=EDGE_LOOP ( 'NONE', ( #7538, #21794, #21935, #31912 ) ) ;
#12523=CARTESIAN_POINT ( 'NONE',  ( -47.66663987350317200, -177.1207230881787780, -0.5829794791144634614 ) ) ;
#12525=DIRECTION ( 'NONE',  ( 0.000000000000000000, 0.000000000000000000, 1.000000000000000000 ) ) ;
#12526=DIRECTION ( 'NONE',  ( 0.000000000000000000, -1.000000000000000000, 0.000000000000000000 ) ) ;
#12527=DIRECTION ( 'NONE',  ( 0.000000000000000000, 0.000000000000000000, 1.000000000000000000 ) ) ;
#12528=DIRECTION ( 'NONE',  ( -0.05924062789370006937, 0.000000000000000000, -0.9982437317643222396 ) ) ;
#12532=DIRECTION ( 'NONE',  ( 0.000000000000000000, 0.000000000000000000, 1.000000000000000000 ) ) ;
#12533=FACE_BOUND ( 'NONE', #51906, .T. ) ;
#12535=VECTOR ( 'NONE', #48235, 1000.000000000000000 ) ;
#12536=CYLINDRICAL_SURFACE ( 'NONE', #8828, 125.0000000000000000 ) ;
#12538=AXIS2_PLACEMENT_3D ( 'NONE', #16453, #48525, #677 ) ;
#12541=EDGE_CURVE ( 'NONE', #48639, #50010, #33537, .T. ) ;
#12543=ORIENTED_EDGE ( 'NONE', *, *, #2754, .F. ) ;
#12547=DIRECTION ( 'NONE',  ( 0.000000000000000000, -0.000000000000000000, -1.000000000000000000 ) ) ;
#12551=ORIENTED_EDGE ( 'NONE', *, *, #2656, .T. ) ;
#12553=ORIENTED_EDGE ( 'NONE', *, *, #13436, .F. ) ;
#12555=DIRECTION ( 'NONE',  ( -0.8455960035018311727, 0.000000000000000000, 0.5338233779647826305 ) ) ;
#12558=LINE ( 'NONE', #21228, #2422 ) ;
#12560=FACE_OUTER_BOUND ( 'NONE', #22254, .T. ) ;
#12563=PLANE ( 'NONE',  #32315 ) ;
#12567=ORIENTED_EDGE ( 'NONE', *, *, #25001, .F. ) ;
#12568=VERTEX_POINT ( 'NONE', #37250 ) ;
#12570=EDGE_LOOP ( 'NONE', ( #11178, #18865, #23848, #39702 ) ) ;
#12572=ORIENTED_EDGE ( 'NONE', *, *, #42962, .T. ) ;
#12573=DIRECTION ( 'NONE',  ( -0.9720229140804107493, 0.000000000000000000, -0.2348860457809842095 ) ) ;
#12574=CARTESIAN_POINT ( 'NONE',  ( -171.9838957966129556, -193.5000000000000000, 19.27620354518722579 ) ) ;
#12575=EDGE_LOOP ( 'NONE', ( #22398, #13459, #40204, #44509 ) ) ;
#12577=CARTESIAN_POINT ( 'NONE',  ( -170.2790847791494855, -183.6283474603465606, -28.10285082451570915 ) ) ;
#12578=EDGE_LOOP ( 'NONE', ( #406, #7316, #21211, #10934 ) ) ;
#12579=EDGE_LOOP ( 'NONE', ( #13155, #3317, #31925, #13503 ) ) ;
#12580=DIRECTION ( 'NONE',  ( 0.000000000000000000, 0.000000000000000000, 1.000000000000000000 ) ) ;
#12583=DIRECTION ( 'NONE',  ( -0.9785564922995017012, 0.000000000000000000, -0.2059786187411094538 ) ) ;
#12584=DIRECTION ( 'NONE',  ( 0.000000000000000000, 0.000000000000000000, 1.000000000000000000 ) ) ;
#12585=CARTESIAN_POINT ( 'NONE',  ( -167.9436818089035057, -177.1207230881787780, 36.78613984830044359 ) ) ;
#12586=CARTESIAN_POINT ( 'NONE',  ( -163.3872488209693756, -183.6283474603465606, -49.20491319441543254 ) ) ;
#12588=DIRECTION ( 'NONE',  ( -0.9785564922995017012, 0.000000000000000000, -0.2059786187411094538 ) ) ;
#12589=AXIS2_PLACEMENT_3D ( 'NONE', #24841, #40862, #37441 ) ;
#12590=VECTOR ( 'NONE', #14558, 1000.000000000000114 ) ;
#12592=EDGE_LOOP ( 'NONE', ( #50550, #27693, #8744, #39271 ) ) ;
#12594=DIRECTION ( 'NONE',  ( -0.000000000000000000, 1.000000000000000000, 0.000000000000000000 ) ) ;
#12595=CARTESIAN_POINT ( 'NONE',  ( -77.67449977936063021, -175.3837268820161057, -121.5427093402339267 ) ) ;
#12597=ORIENTED_EDGE ( 'NONE', *, *, #49778, .F. ) ;
#12598=EDGE_CURVE ( 'NONE', #17248, #24620, #33570, .T. ) ;
#12599=ORIENTED_EDGE ( 'NONE', *, *, #24643, .T. ) ;
#12601=DIRECTION ( 'NONE',  ( 0.000000000000000000, -0.000000000000000000, -1.000000000000000000 ) ) ;
#12602=CIRCLE ( 'NONE', #42841, 125.0000000000000000 ) ;
#12603=DIRECTION ( 'NONE',  ( -0.000000000000000000, 1.000000000000000000, 0.000000000000000000 ) ) ;
#12604=CARTESIAN_POINT ( 'NONE',  ( -99.02518858244150124, -193.5000000000000000, 114.3245189510261497 ) ) ;
#12606=ORIENTED_EDGE ( 'NONE', *, *, #22182, .F. ) ;
#12610=CARTESIAN_POINT ( 'NONE',  ( -152.3176060415594861, -177.1207230881787780, -69.58857822034967455 ) ) ;
#12611=ORIENTED_EDGE ( 'NONE', *, *, #44601, .T. ) ;
#12613=EDGE_CURVE ( 'NONE', #48065, #17157, #36989, .T. ) ;
#12614=FACE_OUTER_BOUND ( 'NONE', #51166, .T. ) ;
#12615=VECTOR ( 'NONE', #16876, 1000.000000000000000 ) ;
#12616=DIRECTION ( 'NONE',  ( 0.9960498426152177842, 0.000000000000000000, -0.08879589532292482545 ) ) ;
#12617=CARTESIAN_POINT ( 'NONE',  ( 75.04604393171729271, -175.3837268820161057, -10.84123789944573701 ) ) ;
#12620=ORIENTED_EDGE ( 'NONE', *, *, #13599, .T. ) ;
#12623=PLANE ( 'NONE',  #29750 ) ;
#12625=VERTEX_POINT ( 'NONE', #17288 ) ;
#12626=CARTESIAN_POINT ( 'NONE',  ( -140.1460956102404509, -193.5000000000000000, 84.98333260264821831 ) ) ;
#12628=CARTESIAN_POINT ( 'NONE',  ( 54.46899307705341187, -183.6283474603465606, -70.89911581792812001 ) ) ;
#12630=CARTESIAN_POINT ( 'NONE',  ( 30.50828161901818092, -183.6283474603465606, 96.88131563365348597 ) ) ;
#12633=CARTESIAN_POINT ( 'NONE',  ( 62.13187335169531167, -193.5000000000000000, -58.22548115875872554 ) ) ;
#12634=DIRECTION ( 'NONE',  ( 0.000000000000000000, 0.000000000000000000, -1.000000000000000000 ) ) ;
#12637=LINE ( 'NONE', #8973, #15731 ) ;
#12638=CARTESIAN_POINT ( 'NONE',  ( -47.78257572244585560, -189.7472609257535510, -0.7175072570443230546 ) ) ;
#12639=PLANE ( 'NONE',  #24019 ) ;
#12643=VERTEX_POINT ( 'NONE', #4949 ) ;
#12644=CARTESIAN_POINT ( 'NONE',  ( 18.00181100848376303, -177.1207230881787780, -105.8550183720733742 ) ) ;
#12647=CARTESIAN_POINT ( 'NONE',  ( -59.86929868745817629, -183.6283474603465606, -124.4799742258549458 ) ) ;
#12648=CIRCLE ( 'NONE', #86, 125.0000000000000000 ) ;
#12651=DIRECTION ( 'NONE',  ( 0.9720229140804123036, 0.000000000000000000, -0.2348860457809775759 ) ) ;
#12653=EDGE_CURVE ( 'NONE', #7505, #6993, #37507, .T. ) ;
#12656=EDGE_CURVE ( 'NONE', #25190, #38286, #16781, .T. ) ;
#12659=DIRECTION ( 'NONE',  ( 0.000000000000000000, -1.000000000000000000, 0.000000000000000000 ) ) ;
#12662=DIRECTION ( 'NONE',  ( -0.000000000000000000, 1.000000000000000000, -0.000000000000000000 ) ) ;
#12663=CARTESIAN_POINT ( 'NONE',  ( -26.20043062753591201, -189.7472609257535510, -122.9986166548862911 ) ) ;
#12664=ORIENTED_EDGE ( 'NONE', *, *, #12235, .T. ) ;
#12666=VECTOR ( 'NONE', #31938, 1000.000000000000000 ) ;
#12668=EDGE_CURVE ( 'NONE', #32981, #23734, #5206, .T. ) ;
#12669=DIRECTION ( 'NONE',  ( -0.5586467658036415873, 0.000000000000000000, -0.8294056854502090959 ) ) ;
#12670=DIRECTION ( 'NONE',  ( 0.000000000000000000, 1.000000000000000000, 0.000000000000000000 ) ) ;
#12671=CARTESIAN_POINT ( 'NONE',  ( 49.10711742958949344, -193.5000000000000000, 78.11481899503480975 ) ) ;
#12672=ORIENTED_EDGE ( 'NONE', *, *, #43872, .F. ) ;
#12673=EDGE_CURVE ( 'NONE', #26290, #16305, #43616, .T. ) ;
#12674=ORIENTED_EDGE ( 'NONE', *, *, #27243, .T. ) ;
#12675=LINE ( 'NONE', #8737, #2322 ) ;
#12676=DIRECTION ( 'NONE',  ( 0.9960498426152177842, 0.000000000000000000, -0.08879589532292482545 ) ) ;
#12677=CARTESIAN_POINT ( 'NONE',  ( -47.60339180931321579, -193.5000000000000000, 0.4827922027307559594 ) ) ;
#12680=CARTESIAN_POINT ( 'NONE',  ( -31.30262293407085039, -183.6283474603465606, -123.8142468240611294 ) ) ;
#12681=VERTEX_POINT ( 'NONE', #29357 ) ;
#12682=PLANE ( 'NONE',  #38939 ) ;
#12683=AXIS2_PLACEMENT_3D ( 'NONE', #27459, #39293, #43747 ) ;
#12684=VERTEX_POINT ( 'NONE', #25172 ) ;
#12685=CARTESIAN_POINT ( 'NONE',  ( -48.13092511607445090, -177.1207230881787780, -0.9374196611341135688 ) ) ;
#12687=DIRECTION ( 'NONE',  ( -0.5085311186492273983, 0.000000000000000000, 0.8610436117673514467 ) ) ;
#12688=ORIENTED_EDGE ( 'NONE', *, *, #4473, .T. ) ;
#12692=EDGE_LOOP ( 'NONE', ( #35246, #28567, #24664, #11000 ) ) ;
#12693=CARTESIAN_POINT ( 'NONE',  ( -26.20043062753592977, -175.3837268820161057, -122.9986166548863196 ) ) ;
#12694=CARTESIAN_POINT ( 'NONE',  ( -156.7610986364826999, -193.5000000000000000, -62.45009659481510766 ) ) ;
#12695=EDGE_CURVE ( 'NONE', #28854, #37405, #48834, .T. ) ;
#12697=ORIENTED_EDGE ( 'NONE', *, *, #48895, .T. ) ;
#12699=VECTOR ( 'NONE', #8782, 1000.000000000000000 ) ;
#12700=LINE ( 'NONE', #37670, #6320 ) ;
#12702=DIRECTION ( 'NONE',  ( -0.2348860457809911206, 0.000000000000000000, 0.9720229140804089729 ) ) ;
#12703=ORIENTED_EDGE ( 'NONE', *, *, #23468, .F. ) ;
#12704=VECTOR ( 'NONE', #46634, 1000.000000000000114 ) ;
#12707=CARTESIAN_POINT ( 'NONE',  ( -48.47912675150885065, -177.1207230881787780, 6.938893903907228378E-15 ) ) ;
#12708=PLANE ( 'NONE',  #43189 ) ;
#12709=DIRECTION ( 'NONE',  ( 0.000000000000000000, 0.000000000000000000, 1.000000000000000000 ) ) ;
#12710=ADVANCED_FACE ( 'NONE', ( #33042 ), #41711, .T. ) ;
#12711=CARTESIAN_POINT ( 'NONE',  ( -167.9436818089035057, -177.1207230881787780, 36.78613984830044359 ) ) ;
#12712=EDGE_CURVE ( 'NONE', #11444, #28167, #1762, .T. ) ;
#12713=VERTEX_POINT ( 'NONE', #41442 ) ;
#12714=CARTESIAN_POINT ( 'NONE',  ( -47.47956591500005885, -177.1207230881787780, 0.02963332782257025594 ) ) ;
#12715=ORIENTED_EDGE ( 'NONE', *, *, #12234, .F. ) ;
#12717=EDGE_CURVE ( 'NONE', #12625, #34416, #20967, .T. ) ;
#12718=DIRECTION ( 'NONE',  ( -0.000000000000000000, 1.000000000000000000, 0.000000000000000000 ) ) ;
#12719=DIRECTION ( 'NONE',  ( 0.000000000000000000, 0.000000000000000000, 1.000000000000000000 ) ) ;
#12722=EDGE_CURVE ( 'NONE', #13819, #48760, #29613, .T. ) ;
#12723=EDGE_LOOP ( 'NONE', ( #33996, #4481, #14501, #43674 ) ) ;
#12725=AXIS2_PLACEMENT_3D ( 'NONE', #39285, #11155, #4070 ) ;
#12726=VECTOR ( 'NONE', #39722, 1000.000000000000000 ) ;
#12727=DIRECTION ( 'NONE',  ( 0.6528221181905280446, 0.000000000000000000, -0.7575112421616145841 ) ) ;
#12728=ORIENTED_EDGE ( 'NONE', *, *, #44591, .F. ) ;
#12730=ORIENTED_EDGE ( 'NONE', *, *, #39465, .T. ) ;
#12732=FACE_OUTER_BOUND ( 'NONE', #14530, .T. ) ;
#12735=VERTEX_POINT ( 'NONE', #45666 ) ;
#12736=CIRCLE ( 'NONE', #3517, 125.0000000000000000 ) ;
#12737=ORIENTED_EDGE ( 'NONE', *, *, #33827, .T. ) ;
#12738=VERTEX_POINT ( 'NONE', #40926 ) ;
#12740=LINE ( 'NONE', #8805, #46152 ) ;
#12742=CARTESIAN_POINT ( 'NONE',  ( -121.5885020763900997, -193.5000000000000000, -101.3904297239420913 ) ) ;
#12745=EDGE_LOOP ( 'NONE', ( #49237, #13668, #30713, #40875 ) ) ;
#12746=ORIENTED_EDGE ( 'NONE', *, *, #34547, .T. ) ;
#12747=LINE ( 'NONE', #36409, #13032 ) ;
#12748=EDGE_LOOP ( 'NONE', ( #33201, #50401, #45219, #25902 ) ) ;
#12750=DIRECTION ( 'NONE',  ( 0.000000000000000000, 0.000000000000000000, -1.000000000000000000 ) ) ;
#12751=ADVANCED_FACE ( 'NONE', ( #9650 ), #25678, .F. ) ;
#12753=CIRCLE ( 'NONE', #9403, 124.9999999999999858 ) ;
#12754=EDGE_CURVE ( 'NONE', #2898, #50750, #42753, .T. ) ;
#12756=EDGE_CURVE ( 'NONE', #33118, #42260, #38787, .T. ) ;
#12758=DIRECTION ( 'NONE',  ( 0.000000000000000000, 0.000000000000000000, -1.000000000000000000 ) ) ;
#12759=ORIENTED_EDGE ( 'NONE', *, *, #1594, .T. ) ;
#12760=LINE ( 'NONE', #19884, #33415 ) ;
#12761=EDGE_LOOP ( 'NONE', ( #45379, #18813, #44950, #2695 ) ) ;
#12763=ORIENTED_EDGE ( 'NONE', *, *, #17676, .F. ) ;
#12764=DIRECTION ( 'NONE',  ( 0.000000000000000000, 0.000000000000000000, 1.000000000000000000 ) ) ;
#12765=EDGE_CURVE ( 'NONE', #20806, #2378, #42479, .T. ) ;
#12766=CARTESIAN_POINT ( 'NONE',  ( 22.03849146056077757, -189.7472609257535510, 103.2098131075567409 ) ) ;
#12767=DIRECTION ( 'NONE',  ( 0.000000000000000000, -1.000000000000000000, 0.000000000000000000 ) ) ;
#12768=PLANE ( 'NONE',  #47433 ) ;
#12770=FACE_OUTER_BOUND ( 'NONE', #39583, .T. ) ;
#12771=DIRECTION ( 'NONE',  ( 0.9960498426152171181, 0.000000000000000000, -0.08879589532293157006 ) ) ;
#12772=ADVANCED_FACE ( 'NONE', ( #43001 ), #46186, .T. ) ;
#12773=ORIENTED_EDGE ( 'NONE', *, *, #33684, .F. ) ;
#12774=DIRECTION ( 'NONE',  ( 0.8124868780056825335, 0.000000000000000000, -0.5829794791144703447 ) ) ;
#12775=DIRECTION ( 'NONE',  ( 0.000000000000000000, 0.000000000000000000, -1.000000000000000000 ) ) ;
#12776=AXIS2_PLACEMENT_3D ( 'NONE', #35227, #7121, #11303 ) ;
#12777=VECTOR ( 'NONE', #6960, 1000.000000000000000 ) ;
#12778=EDGE_CURVE ( 'NONE', #5079, #32692, #22531, .T. ) ;
#12780=FACE_BOUND ( 'NONE', #36818, .T. ) ;
#12781=ORIENTED_EDGE ( 'NONE', *, *, #27566, .T. ) ;
#12784=EDGE_CURVE ( 'NONE', #49515, #14469, #34585, .T. ) ;
#12785=LINE ( 'NONE', #28553, #18035 ) ;
#12786=ORIENTED_EDGE ( 'NONE', *, *, #5598, .T. ) ;
#12788=EDGE_CURVE ( 'NONE', #45115, #27547, #34348, .T. ) ;
#12789=ORIENTED_EDGE ( 'NONE', *, *, #26891, .F. ) ;
#12790=DIRECTION ( 'NONE',  ( 0.000000000000000000, 0.000000000000000000, 1.000000000000000000 ) ) ;
#12795=LINE ( 'NONE', #974, #47243 ) ;
#12796=ORIENTED_EDGE ( 'NONE', *, *, #1569, .F. ) ;
#12797=AXIS2_PLACEMENT_3D ( 'NONE', #20730, #1539, #17321 ) ;
#12799=EDGE_CURVE ( 'NONE', #37529, #30910, #1685, .T. ) ;
#12800=ORIENTED_EDGE ( 'NONE', *, *, #41967, .F. ) ;
#12804=CARTESIAN_POINT ( 'NONE',  ( 21.21056010634072564, -175.3837268820161057, 103.7706487676302061 ) ) ;
#12805=ORIENTED_EDGE ( 'NONE', *, *, #29740, .T. ) ;
#12806=CARTESIAN_POINT ( 'NONE',  ( 52.59568867645218404, -193.5000000000000000, -73.54509967498589162 ) ) ;
#12807=FACE_OUTER_BOUND ( 'NONE', #21427, .T. ) ;
#12808=PLANE ( 'NONE',  #9563 ) ;
#12809=VECTOR ( 'NONE', #51468, 1000.000000000000227 ) ;
#12811=EDGE_CURVE ( 'NONE', #33588, #7429, #50349, .T. ) ;
#12812=LINE ( 'NONE', #35964, #34021 ) ;
#12813=ORIENTED_EDGE ( 'NONE', *, *, #28568, .T. ) ;
#12814=CARTESIAN_POINT ( 'NONE',  ( 74.80070215680143519, -183.6283474603465606, 13.35228579481199596 ) ) ;
#12815=FACE_OUTER_BOUND ( 'NONE', #43784, .T. ) ;
#12816=ORIENTED_EDGE ( 'NONE', *, *, #49475, .T. ) ;
#12818=CIRCLE ( 'NONE', #8621, 125.0000000000000000 ) ;
#12821=ORIENTED_EDGE ( 'NONE', *, *, #41733, .F. ) ;
#12822=CARTESIAN_POINT ( 'NONE',  ( 76.48781641346532467, -175.3837268820161057, 2.874563619424060246 ) ) ;
#12823=EDGE_LOOP ( 'NONE', ( #41728, #1387, #4723, #24322 ) ) ;
#12825=CARTESIAN_POINT ( 'NONE',  ( -135.6699833737243353, -193.5000000000000000, 89.56983042009326823 ) ) ;
#12826=EDGE_CURVE ( 'NONE', #40339, #48757, #14372, .T. ) ;
#12827=EDGE_CURVE ( 'NONE', #34100, #9007, #7007, .T. ) ;
#12828=VECTOR ( 'NONE', #13908, 1000.000000000000000 ) ;
#12829=DIRECTION ( 'NONE',  ( 0.9785564922995032555, 0.000000000000000000, 0.2059786187411021818 ) ) ;
#12830=VERTEX_POINT ( 'NONE', #3055 ) ;
#12834=ADVANCED_FACE ( 'NONE', ( #31171 ), #47221, .T. ) ;
#12835=ORIENTED_EDGE ( 'NONE', *, *, #964, .F. ) ;
#12836=CYLINDRICAL_SURFACE ( 'NONE', #37111, 125.0000000000000000 ) ;
#12841=AXIS2_PLACEMENT_3D ( 'NONE', #24028, #6968, #43490 ) ;
#12846=CARTESIAN_POINT ( 'NONE',  ( -173.0563034899574859, -189.7472609257535510, -10.27263529369816908 ) ) ;
#12851=CARTESIAN_POINT ( 'NONE',  ( -48.53836737940255119, -175.3837268820161057, -0.9982437317643153563 ) ) ;
#12852=EDGE_CURVE ( 'NONE', #47304, #23327, #6233, .T. ) ;
#12853=LINE ( 'NONE', #24957, #27771 ) ;
#12855=CARTESIAN_POINT ( 'NONE',  ( -114.9600645115007467, -183.6283474603465606, 105.8550183720738147 ) ) ;
#12858=VECTOR ( 'NONE', #23397, 1000.000000000000000 ) ;
#12863=VECTOR ( 'NONE', #36060, 1000.000000000000000 ) ;
#12864=DIRECTION ( 'NONE',  ( -0.000000000000000000, 1.000000000000000000, -0.000000000000000000 ) ) ;
#12865=FACE_OUTER_BOUND ( 'NONE', #37225, .T. ) ;
#12866=DIRECTION ( 'NONE',  ( 0.000000000000000000, -0.000000000000000000, -1.000000000000000000 ) ) ;
#12867=ORIENTED_EDGE ( 'NONE', *, *, #20608, .T. ) ;
#12870=PLANE ( 'NONE',  #51197 ) ;
#12871=VERTEX_POINT ( 'NONE', #397 ) ;
#12872=CARTESIAN_POINT ( 'NONE',  ( -53.47502265695602119, -183.6283474603465606, -124.9001241957025883 ) ) ;
#12873=ORIENTED_EDGE ( 'NONE', *, *, #19845, .F. ) ;
#12874=LINE ( 'NONE', #43458, #28368 ) ;
#12875=ORIENTED_EDGE ( 'NONE', *, *, #33827, .F. ) ;
#12877=VECTOR ( 'NONE', #48616, 1000.000000000000227 ) ;
#12878=CIRCLE ( 'NONE', #6188, 125.0000000000000000 ) ;
#12879=DIRECTION ( 'NONE',  ( -0.000000000000000000, 1.000000000000000000, 0.000000000000000000 ) ) ;
#12881=CARTESIAN_POINT ( 'NONE',  ( -75.31296732259116311, -183.6283474603465606, -121.0625654437172614 ) ) ;
#12882=DIRECTION ( 'NONE',  ( -0.000000000000000000, -1.000000000000000000, 0.000000000000000000 ) ) ;
#12884=DIRECTION ( 'NONE',  ( 0.000000000000000000, 0.000000000000000000, 1.000000000000000000 ) ) ;
#12887=DIRECTION ( 'NONE',  ( 0.000000000000000000, 0.000000000000000000, -1.000000000000000000 ) ) ;
#12888=ORIENTED_EDGE ( 'NONE', *, *, #19651, .T. ) ;
#12889=ADVANCED_FACE ( 'NONE', ( #143 ), #15421, .T. ) ;
#12891=FACE_OUTER_BOUND ( 'NONE', #5557, .T. ) ;
#12892=DIRECTION ( 'NONE',  ( 0.000000000000000000, 0.000000000000000000, 1.000000000000000000 ) ) ;
#12893=DIRECTION ( 'NONE',  ( 0.000000000000000000, 1.000000000000000000, 0.000000000000000000 ) ) ;
#12894=AXIS2_PLACEMENT_3D ( 'NONE', #24521, #36614, #5349 ) ;
#12896=CARTESIAN_POINT ( 'NONE',  ( -173.4291566779743050, -189.7472609257535510, 3.534122433558314125 ) ) ;
#12898=DIRECTION ( 'NONE',  ( -0.9473263538541876194, 0.000000000000000000, -0.3202698538628486746 ) ) ;
#12899=CARTESIAN_POINT ( 'NONE',  ( -47.63353074800702558, -189.7472609257535510, -0.5338233779647817423 ) ) ;
#12900=VERTEX_POINT ( 'NONE', #47467 ) ;
#12903=DIRECTION ( 'NONE',  ( 0.000000000000000000, 0.000000000000000000, 1.000000000000000000 ) ) ;
#12904=FACE_OUTER_BOUND ( 'NONE', #34674, .T. ) ;
#12906=DIRECTION ( 'NONE',  ( 0.000000000000000000, 1.000000000000000000, 0.000000000000000000 ) ) ;
#12908=VERTEX_POINT ( 'NONE', #39816 ) ;
#12909=CARTESIAN_POINT ( 'NONE',  ( -168.8371699641976704, -175.3837268820161057, 33.74820638215506108 ) ) ;
#12910=DIRECTION ( 'NONE',  ( -0.000000000000000000, 1.000000000000000000, -0.000000000000000000 ) ) ;
#12911=EDGE_CURVE ( 'NONE', #27896, #39147, #44034, .T. ) ;
#12912=VECTOR ( 'NONE', #48015, 1000.000000000000000 ) ;
#12913=CARTESIAN_POINT ( 'NONE',  ( -71.40672220061269115, -175.3837268820161057, -122.8793122007208751 ) ) ;
#12915=CARTESIAN_POINT ( 'NONE',  ( -81.70897914701313880, -193.5000000000000000, -120.5021863277716534 ) ) ;
#12916=AXIS2_PLACEMENT_3D ( 'NONE', #40893, #28799, #8836 ) ;
#12918=FACE_OUTER_BOUND ( 'NONE', #32187, .T. ) ;
#12919=FACE_OUTER_BOUND ( 'NONE', #2640, .T. ) ;
#12920=CARTESIAN_POINT ( 'NONE',  ( -47.50057025920934706, -193.5000000000000000, 0.2059786187411091207 ) ) ;
#12922=ORIENTED_EDGE ( 'NONE', *, *, #18472, .T. ) ;
#12923=ORIENTED_EDGE ( 'NONE', *, *, #47907, .F. ) ;
#12924=CARTESIAN_POINT ( 'NONE',  ( -51.89154260666836649, -177.1207230881787780, 124.9534129907280828 ) ) ;
#12925=DIRECTION ( 'NONE',  ( -0.2920567706369764371, 0.000000000000000000, 0.9564009842765223146 ) ) ;
#12931=DIRECTION ( 'NONE',  ( 0.000000000000000000, 0.000000000000000000, -1.000000000000000000 ) ) ;
#12934=EDGE_CURVE ( 'NONE', #28114, #39634, #48524, .T. ) ;
#12935=FACE_OUTER_BOUND ( 'NONE', #14646, .T. ) ;
#12936=LINE ( 'NONE', #36871, #24120 ) ;
#12937=EDGE_LOOP ( 'NONE', ( #47426, #9261, #24819, #45784 ) ) ;
#12938=DIRECTION ( 'NONE',  ( 0.000000000000000000, 1.000000000000000000, 0.000000000000000000 ) ) ;
#12940=ORIENTED_EDGE ( 'NONE', *, *, #23126, .F. ) ;
#12942=ORIENTED_EDGE ( 'NONE', *, *, #47675, .F. ) ;
#12943=VECTOR ( 'NONE', #19431, 1000.000000000000000 ) ;
#12944=ADVANCED_FACE ( 'NONE', ( #48248 ), #24075, .T. ) ;
#12946=CARTESIAN_POINT ( 'NONE',  ( -112.1919339979530150, -175.3837268820161057, 107.5438431188761683 ) ) ;
#12947=CARTESIAN_POINT ( 'NONE',  ( 74.77174840718836890, -193.5000000000000000, 20.83798868929603643 ) ) ;
#12948=AXIS2_PLACEMENT_3D ( 'NONE', #25089, #25854, #1144 ) ;
#12949=VERTEX_POINT ( 'NONE', #35626 ) ;
#12950=ADVANCED_FACE ( 'NONE', ( #40091 ), #7776, .F. ) ;
#12951=ORIENTED_EDGE ( 'NONE', *, *, #43319, .T. ) ;
#12953=LINE ( 'NONE', #25068, #28359 ) ;
#12955=CARTESIAN_POINT ( 'NONE',  ( -48.47912675150885065, -175.3837268820161057, 6.938893903907228378E-15 ) ) ;
#12956=DIRECTION ( 'NONE',  ( -0.000000000000000000, 1.000000000000000000, -0.000000000000000000 ) ) ;
#12958=DIRECTION ( 'NONE',  ( -0.000000000000000000, 1.000000000000000000, -0.000000000000000000 ) ) ;
#12962=VERTEX_POINT ( 'NONE', #31427 ) ;
#12963=LINE ( 'NONE', #16684, #24034 ) ;
#12964=VERTEX_POINT ( 'NONE', #11446 ) ;
#12966=DIRECTION ( 'NONE',  ( 0.6528221181905227155, 0.000000000000000000, -0.7575112421616191360 ) ) ;
#12968=ORIENTED_EDGE ( 'NONE', *, *, #29528, .T. ) ;
#12970=DIRECTION ( 'NONE',  ( -0.7575112421616191360, 0.000000000000000000, -0.6528221181905227155 ) ) ;
#12973=CARTESIAN_POINT ( 'NONE',  ( -11.17913199888832843, -189.7472609257535510, 119.3051146910914326 ) ) ;
#12974=ORIENTED_EDGE ( 'NONE', *, *, #18207, .F. ) ;
#12975=PLANE ( 'NONE',  #27836 ) ;
#12977=ORIENTED_EDGE ( 'NONE', *, *, #47534, .T. ) ;
#12979=CARTESIAN_POINT ( 'NONE',  ( -8.721998590732187751, -177.1207230881787780, -118.5089480183145270 ) ) ;
#12980=VERTEX_POINT ( 'NONE', #8302 ) ;
#12981=AXIS2_PLACEMENT_3D ( 'NONE', #42290, #2372, #18402 ) ;
#12982=CIRCLE ( 'NONE', #2903, 125.0000000000000000 ) ;
#12985=CIRCLE ( 'NONE', #49965, 125.0000000000000000 ) ;
#12987=CARTESIAN_POINT ( 'NONE',  ( -173.4460699164830260, -175.3837268820161057, -2.874563619423202265 ) ) ;
#12991=ORIENTED_EDGE ( 'NONE', *, *, #36154, .F. ) ;
#12997=AXIS2_PLACEMENT_3D ( 'NONE', #11389, #7474, #47926 ) ;
#12998=CARTESIAN_POINT ( 'NONE',  ( -47.57632892154310866, -183.6283474603465606, -0.4300652022765113491 ) ) ;
#12999=ORIENTED_EDGE ( 'NONE', *, *, #896, .F. ) ;
#13000=ORIENTED_EDGE ( 'NONE', *, *, #5805, .T. ) ;
#13001=ORIENTED_EDGE ( 'NONE', *, *, #34535, .T. ) ;
#13003=CARTESIAN_POINT ( 'NONE',  ( -48.47912675150885065, -183.6283474603465606, 6.938893903907228378E-15 ) ) ;
#13004=DIRECTION ( 'NONE',  ( 0.000000000000000000, 1.000000000000000000, -0.000000000000000000 ) ) ;
#13005=FACE_OUTER_BOUND ( 'NONE', #8430, .T. ) ;
#13007=FACE_OUTER_BOUND ( 'NONE', #32466, .T. ) ;
#13008=VERTEX_POINT ( 'NONE', #39561 ) ;
#13009=ADVANCED_FACE ( 'NONE', ( #19606 ), #51678, .T. ) ;
#13010=EDGE_CURVE ( 'NONE', #24862, #10381, #37712, .T. ) ;
#13011=EDGE_CURVE ( 'NONE', #12713, #24991, #4200, .T. ) ;
#13012=ORIENTED_EDGE ( 'NONE', *, *, #3112, .T. ) ;
#13014=ORIENTED_EDGE ( 'NONE', *, *, #10991, .F. ) ;
#13015=VERTEX_POINT ( 'NONE', #4611 ) ;
#13016=EDGE_CURVE ( 'NONE', #36281, #31485, #12740, .T. ) ;
#13017=VECTOR ( 'NONE', #21852, 1000.000000000000114 ) ;
#13018=FACE_OUTER_BOUND ( 'NONE', #6214, .T. ) ;
#13019=EDGE_CURVE ( 'NONE', #48355, #6199, #44558, .T. ) ;
#13020=DIRECTION ( 'NONE',  ( 0.000000000000000000, 1.000000000000000000, -0.000000000000000000 ) ) ;
#13021=CIRCLE ( 'NONE', #51634, 125.0000000000000000 ) ;
#13023=PLANE ( 'NONE',  #17866 ) ;
#13027=CARTESIAN_POINT ( 'NONE',  ( -48.47912675150885065, -175.3837268820161057, 125.0000000000000000 ) ) ;
#13028=ORIENTED_EDGE ( 'NONE', *, *, #50354, .F. ) ;
#13030=ORIENTED_EDGE ( 'NONE', *, *, #971, .F. ) ;
#13032=VECTOR ( 'NONE', #44043, 1000.000000000000000 ) ;
#13034=AXIS2_PLACEMENT_3D ( 'NONE', #28502, #5132, #27987 ) ;
#13035=PLANE ( 'NONE',  #45800 ) ;
#13040=CARTESIAN_POINT ( 'NONE',  ( -117.0614752283615019, -193.5000000000000000, 103.3076327631967928 ) ) ;
#13041=CARTESIAN_POINT ( 'NONE',  ( -129.4514457347087273, -193.5000000000000000, 95.22858582633115532 ) ) ;
#13042=DIRECTION ( 'NONE',  ( 0.000000000000000000, 0.000000000000000000, 1.000000000000000000 ) ) ;
#13043=AXIS2_PLACEMENT_3D ( 'NONE', #17809, #22981, #21236 ) ;
#13044=FACE_BOUND ( 'NONE', #46602, .T. ) ;
#13048=CARTESIAN_POINT ( 'NONE',  ( -130.2106798473772642, -175.3837268820161057, 94.57776286494217288 ) ) ;
#13051=ORIENTED_EDGE ( 'NONE', *, *, #33725, .F. ) ;
#13052=CARTESIAN_POINT ( 'NONE',  ( 55.92943606843918047, -189.7472609257535510, -66.89437584437831674 ) ) ;
#13055=DIRECTION ( 'NONE',  ( -0.9473263538541876194, 0.000000000000000000, -0.3202698538628486746 ) ) ;
#13056=ORIENTED_EDGE ( 'NONE', *, *, #18533, .F. ) ;
#13057=AXIS2_PLACEMENT_3D ( 'NONE', #26082, #21643, #37663 ) ;
#13059=ADVANCED_FACE ( 'NONE', ( #37187 ), #9342, .F. ) ;
#13060=ADVANCED_FACE ( 'NONE', ( #49558 ), #925, .T. ) ;
#13061=EDGE_CURVE ( 'NONE', #3589, #44850, #20638, .T. ) ;
#13063=VERTEX_POINT ( 'NONE', #676 ) ;
#13067=DIRECTION ( 'NONE',  ( 0.000000000000000000, -1.000000000000000000, 0.000000000000000000 ) ) ;
#13068=DIRECTION ( 'NONE',  ( 0.7175072570443249420, 0.000000000000000000, 0.6965510290630033685 ) ) ;
#13069=ORIENTED_EDGE ( 'NONE', *, *, #5103, .F. ) ;
#13070=VECTOR ( 'NONE', #7908, 1000.000000000000000 ) ;
#13071=FACE_OUTER_BOUND ( 'NONE', #43452, .T. ) ;
#13073=AXIS2_PLACEMENT_3D ( 'NONE', #18506, #19023, #47139 ) ;
#13078=VECTOR ( 'NONE', #29112, 1000.000000000000227 ) ;
#13079=ADVANCED_FACE ( 'NONE', ( #29556 ), #8543, .F. ) ;
#13080=CIRCLE ( 'NONE', #32391, 125.0000000000000000 ) ;
#13081=DIRECTION ( 'NONE',  ( -0.000000000000000000, 1.000000000000000000, -0.000000000000000000 ) ) ;
#13082=CARTESIAN_POINT ( 'NONE',  ( 32.34187644556188701, -189.7472609257535510, 94.04236105995856576 ) ) ;
#13083=EDGE_LOOP ( 'NONE', ( #23623, #16842, #3079, #48576 ) ) ;
#13088=ADVANCED_FACE ( 'NONE', ( #5405 ), #24578, .F. ) ;
#13089=CARTESIAN_POINT ( 'NONE',  ( -116.2964108826154330, -183.6283474603465606, -105.0038855142073260 ) ) ;
#13090=ORIENTED_EDGE ( 'NONE', *, *, #46564, .F. ) ;
#13091=CARTESIAN_POINT ( 'NONE',  ( 8.294189685504184339, -189.7472609257535510, -110.2396968984190977 ) ) ;
#13093=EDGE_CURVE ( 'NONE', #48020, #51413, #4889, .T. ) ;
#13094=DIRECTION ( 'NONE',  ( -0.000000000000000000, 1.000000000000000000, -0.000000000000000000 ) ) ;
#13095=PLANE ( 'NONE',  #25879 ) ;
#13097=FACE_OUTER_BOUND ( 'NONE', #26136, .T. ) ;
#13099=ORIENTED_EDGE ( 'NONE', *, *, #49093, .F. ) ;
#13101=AXIS2_PLACEMENT_3D ( 'NONE', #6332, #2638, #34692 ) ;
#13103=AXIS2_PLACEMENT_3D ( 'NONE', #9432, #25972, #25457 ) ;
#13104=CARTESIAN_POINT ( 'NONE',  ( 39.18328161278951427, -189.7472609257535510, 89.10837311819236106 ) ) ;
#13105=ORIENTED_EDGE ( 'NONE', *, *, #33964, .F. ) ;
#13106=CIRCLE ( 'NONE', #485, 125.0000000000000000 ) ;
#13107=PLANE ( 'NONE',  #43184 ) ;
#13108=VECTOR ( 'NONE', #38685, 1000.000000000000000 ) ;
#13114=CARTESIAN_POINT ( 'NONE',  ( 75.95066919219054569, -175.3837268820161057, -11.92584929509535385 ) ) ;
#13116=ORIENTED_EDGE ( 'NONE', *, *, #37869, .T. ) ;
#13117=ORIENTED_EDGE ( 'NONE', *, *, #48386, .T. ) ;
#13119=VECTOR ( 'NONE', #51146, 1000.000000000000000 ) ;
#13121=CARTESIAN_POINT ( 'NONE',  ( 60.02977459919872416, -193.5000000000000000, 60.01515274641010222 ) ) ;
#13123=ORIENTED_EDGE ( 'NONE', *, *, #7918, .T. ) ;
#13125=VECTOR ( 'NONE', #13946, 1000.000000000000000 ) ;
#13127=AXIS2_PLACEMENT_3D ( 'NONE', #12372, #43662, #16321 ) ;
#13128=ADVANCED_FACE ( 'NONE', ( #33517 ), #41638, .T. ) ;
#13129=DIRECTION ( 'NONE',  ( 0.000000000000000000, 1.000000000000000000, 0.000000000000000000 ) ) ;
#13132=CARTESIAN_POINT ( 'NONE',  ( -48.47912675150885065, -183.6283474603465606, 6.938893903907228378E-15 ) ) ;
#13134=EDGE_CURVE ( 'NONE', #11371, #10636, #36107, .T. ) ;
#13135=EDGE_CURVE ( 'NONE', #49319, #16002, #23512, .T. ) ;
#13136=EDGE_CURVE ( 'NONE', #38627, #28107, #6698, .T. ) ;
#13138=DIRECTION ( 'NONE',  ( 0.6528221181905119463, 0.000000000000000000, 0.7575112421616284619 ) ) ;
#13142=CYLINDRICAL_SURFACE ( 'NONE', #43503, 125.0000000000000000 ) ;
#13143=VECTOR ( 'NONE', #16483, 1000.000000000000000 ) ;
#13144=AXIS2_PLACEMENT_3D ( 'NONE', #45066, #112, #20342 ) ;
#13146=EDGE_CURVE ( 'NONE', #45652, #38573, #9857, .T. ) ;
#13149=EDGE_CURVE ( 'NONE', #33039, #49664, #1967, .T. ) ;
#13150=EDGE_CURVE ( 'NONE', #46777, #17068, #33606, .T. ) ;
#13154=FACE_OUTER_BOUND ( 'NONE', #51109, .T. ) ;
#13155=ORIENTED_EDGE ( 'NONE', *, *, #6398, .T. ) ;
#13159=VECTOR ( 'NONE', #25981, 999.9999999999998863 ) ;
#13160=CARTESIAN_POINT ( 'NONE',  ( -47.82630463331833681, -183.6283474603465606, 0.7575112421616305713 ) ) ;
#13161=AXIS2_PLACEMENT_3D ( 'NONE', #48482, #24540, #36634 ) ;
#13162=ORIENTED_EDGE ( 'NONE', *, *, #40725, .T. ) ;
#13163=LINE ( 'NONE', #9478, #24738 ) ;
#13165=ORIENTED_EDGE ( 'NONE', *, *, #29852, .T. ) ;
#13166=EDGE_CURVE ( 'NONE', #3937, #40253, #14580, .T. ) ;
#13169=DIRECTION ( 'NONE',  ( -0.2920567706369833760, 0.000000000000000000, 0.9564009842765202052 ) ) ;
#13171=VERTEX_POINT ( 'NONE', #26658 ) ;
#13172=EDGE_CURVE ( 'NONE', #32165, #26290, #2227, .T. ) ;
#13175=FACE_BOUND ( 'NONE', #10071, .T. ) ;
#13176=LINE ( 'NONE', #29444, #47515 ) ;
#13177=EDGE_LOOP ( 'NONE', ( #20687, #42146, #9291, #23836 ) ) ;
#13179=CYLINDRICAL_SURFACE ( 'NONE', #50948, 125.0000000000000000 ) ;
#13184=CARTESIAN_POINT ( 'NONE',  ( -19.28375372365792728, -175.3837268820161057, 121.5427093402341541 ) ) ;
#13185=EDGE_CURVE ( 'NONE', #21275, #44850, #16817, .T. ) ;
#13186=CARTESIAN_POINT ( 'NONE',  ( 50.70030191143631271, -177.1207230881787780, -76.08180419845318454 ) ) ;
#13189=CARTESIAN_POINT ( 'NONE',  ( 25.43954814678888710, -183.6283474603465606, 100.8019320314832754 ) ) ;
#13190=PLANE ( 'NONE',  #37868 ) ;
#13194=LINE ( 'NONE', #40769, #46450 ) ;
#13195=AXIS2_PLACEMENT_3D ( 'NONE', #51359, #19300, #28187 ) ;
#13196=CIRCLE ( 'NONE', #14069, 125.0000000000000000 ) ;
#13198=LINE ( 'NONE', #24757, #2718 ) ;
#13200=ORIENTED_EDGE ( 'NONE', *, *, #7952, .T. ) ;
#13201=CIRCLE ( 'NONE', #9000, 125.0000000000000000 ) ;
#13202=EDGE_LOOP ( 'NONE', ( #33084, #30088, #23181, #18275 ) ) ;
#13203=EDGE_CURVE ( 'NONE', #12033, #41128, #39434, .T. ) ;
#13204=EDGE_CURVE ( 'NONE', #31327, #3759, #38216, .T. ) ;
#13205=FACE_OUTER_BOUND ( 'NONE', #6293, .T. ) ;
#13206=VECTOR ( 'NONE', #19787, 1000.000000000000000 ) ;
#13207=CARTESIAN_POINT ( 'NONE',  ( -48.47912675150885065, -189.7472609257535510, 6.938893903907228378E-15 ) ) ;
#13208=CARTESIAN_POINT ( 'NONE',  ( -15.81236726369125023, -193.5000000000000000, -120.6560517527615417 ) ) ;
#13209=ORIENTED_EDGE ( 'NONE', *, *, #19202, .T. ) ;
#13211=VERTEX_POINT ( 'NONE', #6943 ) ;
#13212=CARTESIAN_POINT ( 'NONE',  ( 64.44365795514079309, -175.3837268820161057, -53.60452120946195009 ) ) ;
#13213=DIRECTION ( 'NONE',  ( -0.3482016354343866471, 0.000000000000000000, -0.9374196611341253371 ) ) ;
#13214=DIRECTION ( 'NONE',  ( -0.000000000000000000, 1.000000000000000000, 0.000000000000000000 ) ) ;
#13215=VERTEX_POINT ( 'NONE', #18268 ) ;
#13217=VECTOR ( 'NONE', #7283, 1000.000000000000000 ) ;
#13219=ORIENTED_EDGE ( 'NONE', *, *, #19208, .T. ) ;
#13221=EDGE_CURVE ( 'NONE', #49515, #17649, #34288, .T. ) ;
#13222=DIRECTION ( 'NONE',  ( -0.000000000000000000, 1.000000000000000000, -0.000000000000000000 ) ) ;
#13225=AXIS2_PLACEMENT_3D ( 'NONE', #21549, #45462, #1572 ) ;
#13226=ORIENTED_EDGE ( 'NONE', *, *, #19984, .F. ) ;
#13227=PLANE ( 'NONE',  #17380 ) ;
#13229=PLANE ( 'NONE',  #16509 ) ;
#13230=ADVANCED_FACE ( 'NONE', ( #38984 ), #18771, .T. ) ;
#13232=VECTOR ( 'NONE', #8794, 1000.000000000000000 ) ;
#13233=ORIENTED_EDGE ( 'NONE', *, *, #40053, .F. ) ;
#13234=DIRECTION ( 'NONE',  ( -0.000000000000000000, 1.000000000000000000, -0.000000000000000000 ) ) ;
#13236=AXIS2_PLACEMENT_3D ( 'NONE', #44693, #36274, #275 ) ;
#13237=VERTEX_POINT ( 'NONE', #44236 ) ;
#13240=PLANE ( 'NONE',  #204 ) ;
#13243=CIRCLE ( 'NONE', #24859, 125.0000000000000000 ) ;
#13247=DIRECTION ( 'NONE',  ( -0.000000000000000000, -1.000000000000000000, 0.000000000000000000 ) ) ;
#13248=ORIENTED_EDGE ( 'NONE', *, *, #24720, .F. ) ;
#13249=CARTESIAN_POINT ( 'NONE',  ( 63.31225588004632243, -177.1207230881787780, 55.92572546981597981 ) ) ;
#13253=LINE ( 'NONE', #34255, #34963 ) ;
#13256=DIRECTION ( 'NONE',  ( -0.000000000000000000, -1.000000000000000000, 0.000000000000000000 ) ) ;
#13257=EDGE_LOOP ( 'NONE', ( #25420, #15587, #2524, #6863 ) ) ;
#13258=ORIENTED_EDGE ( 'NONE', *, *, #33779, .T. ) ;
#13259=AXIS2_PLACEMENT_3D ( 'NONE', #7983, #48719, #20324 ) ;
#13262=CARTESIAN_POINT ( 'NONE',  ( -48.47912675150885065, -175.3837268820161057, 124.0000000000000142 ) ) ;
#13264=AXIS2_PLACEMENT_3D ( 'NONE', #5336, #28952, #41844 ) ;
#13267=EDGE_CURVE ( 'NONE', #9868, #7246, #8232, .T. ) ;
#13269=DIRECTION ( 'NONE',  ( -0.000000000000000000, 1.000000000000000000, -0.000000000000000000 ) ) ;
#13271=VERTEX_POINT ( 'NONE', #27683 ) ;
#13272=LINE ( 'NONE', #29799, #34009 ) ;
#13274=CARTESIAN_POINT ( 'NONE',  ( 50.27798938500057346, -183.6283474603465606, 74.98773087994527486 ) ) ;
#13279=ORIENTED_EDGE ( 'NONE', *, *, #14110, .T. ) ;
#13281=VECTOR ( 'NONE', #34913, 1000.000000000000000 ) ;
#13282=FACE_OUTER_BOUND ( 'NONE', #38421, .T. ) ;
#13284=ADVANCED_FACE ( 'NONE', ( #7962 ), #20057, .T. ) ;
#13285=PLANE ( 'NONE',  #32923 ) ;
#13286=PLANE ( 'NONE',  #31420 ) ;
#13288=VERTEX_POINT ( 'NONE', #39258 ) ;
#13291=ORIENTED_EDGE ( 'NONE', *, *, #10221, .F. ) ;
#13292=AXIS2_PLACEMENT_3D ( 'NONE', #51140, #15124, #46401 ) ;
#13293=PLANE ( 'NONE',  #24964 ) ;
#13295=CARTESIAN_POINT ( 'NONE',  ( -48.47912675150883643, -173.5000000000000284, -125.0000000000000000 ) ) ;
#13297=CARTESIAN_POINT ( 'NONE',  ( 49.27559354810669845, -177.1207230881787780, -76.29032973288636299 ) ) ;
#13298=DIRECTION ( 'NONE',  ( -0.9646355819083594074, 0.000000000000000000, 0.2635871660690647933 ) ) ;
#13302=EDGE_CURVE ( 'NONE', #48835, #43321, #47157, .T. ) ;
#13304=VERTEX_POINT ( 'NONE', #19535 ) ;
#13307=LINE ( 'NONE', #48793, #7710 ) ;
#13308=ORIENTED_EDGE ( 'NONE', *, *, #20230, .T. ) ;
#13309=ADVANCED_FACE ( 'NONE', ( #27936 ), #48184, .T. ) ;
#13310=DIRECTION ( 'NONE',  ( -0.5085311186492216251, 0.000000000000000000, 0.8610436117673548884 ) ) ;
#13311=FACE_OUTER_BOUND ( 'NONE', #32698, .T. ) ;
#13314=PLANE ( 'NONE',  #3039 ) ;
#13315=VECTOR ( 'NONE', #33064, 1000.000000000000000 ) ;
#13316=ADVANCED_FACE ( 'NONE', ( #15876 ), #12153, .T. ) ;
#13317=DIRECTION ( 'NONE',  ( -0.000000000000000000, -1.000000000000000000, 0.000000000000000000 ) ) ;
#13318=CARTESIAN_POINT ( 'NONE',  ( -152.3176060415594861, -177.1207230881787780, -69.58857822034967455 ) ) ;
#13319=VERTEX_POINT ( 'NONE', #11902 ) ;
#13321=ORIENTED_EDGE ( 'NONE', *, *, #17550, .F. ) ;
#13322=CARTESIAN_POINT ( 'NONE',  ( -147.8383830610225971, -183.6283474603465606, -74.18852968774183410 ) ) ;
#13323=ORIENTED_EDGE ( 'NONE', *, *, #32392, .T. ) ;
#13325=EDGE_CURVE ( 'NONE', #50173, #40815, #24266, .T. ) ;
#13326=EDGE_LOOP ( 'NONE', ( #11725, #26110, #1042, #8765 ) ) ;
#13327=EDGE_CURVE ( 'NONE', #26701, #41833, #31622, .T. ) ;
#13329=CARTESIAN_POINT ( 'NONE',  ( -144.0067397530739584, -193.5000000000000000, -80.61932246194587037 ) ) ;
#13331=EDGE_CURVE ( 'NONE', #6422, #43736, #23240, .T. ) ;
#13333=FACE_BOUND ( 'NONE', #33876, .T. ) ;
#13335=ORIENTED_EDGE ( 'NONE', *, *, #9880, .F. ) ;
#13336=AXIS2_PLACEMENT_3D ( 'NONE', #23602, #3122, #15214 ) ;
#13338=ORIENTED_EDGE ( 'NONE', *, *, #9616, .F. ) ;
#13340=VERTEX_POINT ( 'NONE', #36083 ) ;
#13341=DIRECTION ( 'NONE',  ( -0.2920567706369694982, 0.000000000000000000, -0.9564009842765243130 ) ) ;
#13342=AXIS2_PLACEMENT_3D ( 'NONE', #188, #16237, #40915 ) ;
#13343=DIRECTION ( 'NONE',  ( 0.000000000000000000, -1.000000000000000000, 0.000000000000000000 ) ) ;
#13344=ORIENTED_EDGE ( 'NONE', *, *, #41657, .F. ) ;
#13346=DIRECTION ( 'NONE',  ( 0.000000000000000000, 1.000000000000000000, 0.000000000000000000 ) ) ;
#13347=CARTESIAN_POINT ( 'NONE',  ( 76.48781641346532467, -189.7472609257535510, 2.874563619424056249 ) ) ;
#13349=EDGE_LOOP ( 'NONE', ( #10341, #23795, #36305, #33524 ) ) ;
#13350=AXIS2_PLACEMENT_3D ( 'NONE', #31188, #35383, #2814 ) ;
#13353=VERTEX_POINT ( 'NONE', #51360 ) ;
#13354=DIRECTION ( 'NONE',  ( -0.05924062789372142729, 0.000000000000000000, 0.9982437317643209074 ) ) ;
#13357=ORIENTED_EDGE ( 'NONE', *, *, #28179, .T. ) ;
#13359=CARTESIAN_POINT ( 'NONE',  ( -48.47912675150885065, -177.1207230881787780, 6.938893903907228378E-15 ) ) ;
#13362=CARTESIAN_POINT ( 'NONE',  ( -10.02015192278479816, -177.1207230881787780, -117.8859915627474493 ) ) ;
#13363=VERTEX_POINT ( 'NONE', #31884 ) ;
#13364=FACE_OUTER_BOUND ( 'NONE', #5796, .T. ) ;
#13367=DIRECTION ( 'NONE',  ( 0.000000000000000000, -1.000000000000000000, 0.000000000000000000 ) ) ;
#13368=LINE ( 'NONE', #5237, #46577 ) ;
#13371=DIRECTION ( 'NONE',  ( -0.000000000000000000, 1.000000000000000000, -0.000000000000000000 ) ) ;
#13372=ORIENTED_EDGE ( 'NONE', *, *, #4725, .T. ) ;
#13374=VECTOR ( 'NONE', #21998, 1000.000000000000000 ) ;
#13375=CARTESIAN_POINT ( 'NONE',  ( 15.80042947435468470, -193.5000000000000000, 107.2060569716377927 ) ) ;
#13377=EDGE_CURVE ( 'NONE', #26105, #1712, #845, .T. ) ;
#13379=CARTESIAN_POINT ( 'NONE',  ( 72.14504940832446778, -175.3837268820161057, -32.78426643622660208 ) ) ;
#13380=LINE ( 'NONE', #48872, #28847 ) ;
#13381=FACE_OUTER_BOUND ( 'NONE', #8308, .T. ) ;
#13384=EDGE_LOOP ( 'NONE', ( #32411, #36902, #21700, #43416 ) ) ;
#13385=CARTESIAN_POINT ( 'NONE',  ( -88.49718702276007321, -183.6283474603465606, -117.3655938605927673 ) ) ;
#13386=LINE ( 'NONE', #45207, #26249 ) ;
#13388=DIRECTION ( 'NONE',  ( -0.5586467658036415873, 0.000000000000000000, -0.8294056854502090959 ) ) ;
#13389=ADVANCED_FACE ( 'NONE', ( #35825 ), #47922, .T. ) ;
#13390=ORIENTED_EDGE ( 'NONE', *, *, #20390, .T. ) ;
#13392=AXIS2_PLACEMENT_3D ( 'NONE', #2110, #5833, #10022 ) ;
#13393=DIRECTION ( 'NONE',  ( 0.000000000000000000, -0.000000000000000000, 1.000000000000000000 ) ) ;
#13394=EDGE_CURVE ( 'NONE', #7329, #5830, #32394, .T. ) ;
#13395=DIRECTION ( 'NONE',  ( -0.6965510290629882695, 0.000000000000000000, -0.7175072570443395970 ) ) ;
#13396=LINE ( 'NONE', #29409, #31263 ) ;
#13397=LINE ( 'NONE', #33097, #20356 ) ;
#13401=VERTEX_POINT ( 'NONE', #29240 ) ;
#13402=CARTESIAN_POINT ( 'NONE',  ( -166.1003692892502102, -183.6283474603465606, -42.31126686685033889 ) ) ;
#13404=CARTESIAN_POINT ( 'NONE',  ( -49.29161362951452929, -193.5000000000000000, -0.5829794791144748967 ) ) ;
#13405=AXIS2_PLACEMENT_3D ( 'NONE', #50622, #34331, #14360 ) ;
#13406=ORIENTED_EDGE ( 'NONE', *, *, #31081, .F. ) ;
#13408=EDGE_LOOP ( 'NONE', ( #28139, #27807, #19325, #18987 ) ) ;
#13409=CARTESIAN_POINT ( 'NONE',  ( 9.518239912201957864, -213.5000000000000000, 110.7307791902283043 ) ) ;
#13410=DIRECTION ( 'NONE',  ( -0.000000000000000000, 1.000000000000000000, -0.000000000000000000 ) ) ;
#13411=ORIENTED_EDGE ( 'NONE', *, *, #25650, .F. ) ;
#13412=CARTESIAN_POINT ( 'NONE',  ( -29.85296035031868911, -193.5000000000000000, 122.5936119678275702 ) ) ;
#13414=ORIENTED_EDGE ( 'NONE', *, *, #16236, .T. ) ;
#13415=FACE_OUTER_BOUND ( 'NONE', #50016, .T. ) ;
#13416=VERTEX_POINT ( 'NONE', #24511 ) ;
#13417=DIRECTION ( 'NONE',  ( 0.1182731709213592358, 0.000000000000000000, 0.9929810960135178055 ) ) ;
#13418=ORIENTED_EDGE ( 'NONE', *, *, #31823, .T. ) ;
#13420=CARTESIAN_POINT ( 'NONE',  ( 24.88090138098523241, -177.1207230881787780, 99.97252634603304955 ) ) ;
#13421=DIRECTION ( 'NONE',  ( 1.000000000000000000, 0.000000000000000000, -0.000000000000000000 ) ) ;
#13422=ORIENTED_EDGE ( 'NONE', *, *, #50690, .T. ) ;
#13423=VERTEX_POINT ( 'NONE', #8478 ) ;
#13425=VECTOR ( 'NONE', #20616, 1000.000000000000000 ) ;
#13427=DIRECTION ( 'NONE',  ( 0.000000000000000000, -1.000000000000000000, 0.000000000000000000 ) ) ;
#13428=CARTESIAN_POINT ( 'NONE',  ( -130.7087404384255080, -189.7472609257535510, -94.14505102712755047 ) ) ;
#13429=DIRECTION ( 'NONE',  ( 0.000000000000000000, -1.000000000000000000, 0.000000000000000000 ) ) ;
#13430=ORIENTED_EDGE ( 'NONE', *, *, #30055, .F. ) ;
#13431=CARTESIAN_POINT ( 'NONE',  ( 26.10278175629141018, -189.7472609257535510, -99.06333546307678262 ) ) ;
#13432=CYLINDRICAL_SURFACE ( 'NONE', #46697, 125.0000000000000000 ) ;
#13436=EDGE_CURVE ( 'NONE', #7246, #45277, #40530, .T. ) ;
#13437=ORIENTED_EDGE ( 'NONE', *, *, #51660, .T. ) ;
#13439=LINE ( 'NONE', #33140, #45615 ) ;
#13440=CARTESIAN_POINT ( 'NONE',  ( 9.518239912201957864, -213.5000000000000000, -110.7307791902283043 ) ) ;
#13441=EDGE_CURVE ( 'NONE', #20535, #8894, #16382, .T. ) ;
#13444=VECTOR ( 'NONE', #2654, 1000.000000000000000 ) ;
#13446=EDGE_CURVE ( 'NONE', #14916, #27618, #45539, .T. ) ;
#13451=ADVANCED_FACE ( 'NONE', ( #32908 ), #25297, .T. ) ;
#13453=EDGE_CURVE ( 'NONE', #30392, #44484, #17436, .T. ) ;
#13454=DIRECTION ( 'NONE',  ( 0.9960498426152165630, 0.000000000000000000, 0.08879589532293852283 ) ) ;
#13456=DIRECTION ( 'NONE',  ( 0.000000000000000000, -0.000000000000000000, 1.000000000000000000 ) ) ;
#13457=ORIENTED_EDGE ( 'NONE', *, *, #3377, .T. ) ;
#13458=ADVANCED_FACE ( 'NONE', ( #28699 ), #44755, .F. ) ;
#13459=ORIENTED_EDGE ( 'NONE', *, *, #25265, .F. ) ;
#13460=LINE ( 'NONE', #45013, #3088 ) ;
#13461=ADVANCED_FACE ( 'NONE', ( #49499 ), #4820, .T. ) ;
#13463=AXIS2_PLACEMENT_3D ( 'NONE', #14813, #30828, #46875 ) ;
#13465=FACE_OUTER_BOUND ( 'NONE', #8291, .T. ) ;
#13466=ORIENTED_EDGE ( 'NONE', *, *, #28496, .F. ) ;
#13467=ORIENTED_EDGE ( 'NONE', *, *, #40053, .T. ) ;
#13468=ORIENTED_EDGE ( 'NONE', *, *, #35982, .T. ) ;
#13469=FACE_OUTER_BOUND ( 'NONE', #46887, .T. ) ;
#13470=DIRECTION ( 'NONE',  ( -0.9890401873221654760, 0.000000000000000000, 0.1476465640024710868 ) ) ;
#13471=FACE_OUTER_BOUND ( 'NONE', #49867, .T. ) ;
#13472=ORIENTED_EDGE ( 'NONE', *, *, #3146, .F. ) ;
#13473=ADVANCED_FACE ( 'NONE', ( #12935 ), #45028, .T. ) ;
#13474=CARTESIAN_POINT ( 'NONE',  ( -18.31235070009513421, -189.7472609257535510, 121.3052580173829966 ) ) ;
#13475=DIRECTION ( 'NONE',  ( 0.000000000000000000, 0.000000000000000000, -1.000000000000000000 ) ) ;
#13478=FACE_OUTER_BOUND ( 'NONE', #26133, .T. ) ;
#13479=EDGE_LOOP ( 'NONE', ( #4727, #26591, #46433, #31282 ) ) ;
#13481=ORIENTED_EDGE ( 'NONE', *, *, #42109, .T. ) ;
#13482=FACE_OUTER_BOUND ( 'NONE', #47911, .T. ) ;
#13483=FACE_OUTER_BOUND ( 'NONE', #47599, .T. ) ;
#13485=ORIENTED_EDGE ( 'NONE', *, *, #12934, .F. ) ;
#13486=ORIENTED_EDGE ( 'NONE', *, *, #9529, .T. ) ;
#13491=VECTOR ( 'NONE', #43493, 1000.000000000000000 ) ;
#13492=ADVANCED_FACE ( 'NONE', ( #17158 ), #33175, .T. ) ;
#13494=ORIENTED_EDGE ( 'NONE', *, *, #44666, .F. ) ;
#13497=VECTOR ( 'NONE', #17937, 1000.000000000000000 ) ;
#13500=EDGE_CURVE ( 'NONE', #44345, #18213, #38417, .T. ) ;
#13501=ORIENTED_EDGE ( 'NONE', *, *, #12114, .F. ) ;
#13502=FACE_OUTER_BOUND ( 'NONE', #3188, .T. ) ;
#13503=ORIENTED_EDGE ( 'NONE', *, *, #18878, .T. ) ;
#13505=DIRECTION ( 'NONE',  ( 0.1476465640024710868, 0.000000000000000000, 0.9890401873221654760 ) ) ;
#13506=EDGE_LOOP ( 'NONE', ( #48352, #10564, #45191, #12664 ) ) ;
#13507=DIRECTION ( 'NONE',  ( -0.000000000000000000, 1.000000000000000000, -0.000000000000000000 ) ) ;
#13508=CARTESIAN_POINT ( 'NONE',  ( -27.18512803868276251, -193.5000000000000000, -123.1729094355498404 ) ) ;
#13509=LINE ( 'NONE', #29274, #28244 ) ;
#13510=LINE ( 'NONE', #39158, #25749 ) ;
#13511=VERTEX_POINT ( 'NONE', #2151 ) ;
#13512=DIRECTION ( 'NONE',  ( 0.5085311186492154079, 0.000000000000000000, 0.8610436117673585521 ) ) ;
#13513=VERTEX_POINT ( 'NONE', #1652 ) ;
#13518=CARTESIAN_POINT ( 'NONE',  ( -69.59623518921151231, -175.3837268820161057, 122.1886788576023974 ) ) ;
#13519=VERTEX_POINT ( 'NONE', #42352 ) ;
#13521=DIRECTION ( 'NONE',  ( -0.000000000000000000, 1.000000000000000000, -0.000000000000000000 ) ) ;
#13523=CARTESIAN_POINT ( 'NONE',  ( 68.72094416275764672, -193.5000000000000000, -40.49875167738977666 ) ) ;
#13525=CARTESIAN_POINT ( 'NONE',  ( -104.3615810019516772, -193.5000000000000000, 110.6939782313525455 ) ) ;
#13527=CARTESIAN_POINT ( 'NONE',  ( -47.53180039765466347, -193.5000000000000000, 0.3202698538628485636 ) ) ;
#13528=DIRECTION ( 'NONE',  ( 0.000000000000000000, 1.000000000000000000, -0.000000000000000000 ) ) ;
#13529=AXIS2_PLACEMENT_3D ( 'NONE', #53, #12910, #24235 ) ;
#13530=DIRECTION ( 'NONE',  ( 0.000000000000000000, 0.000000000000000000, -1.000000000000000000 ) ) ;
#13531=CARTESIAN_POINT ( 'NONE',  ( -48.47912675150885065, -183.6283474603465606, 6.938893903907228378E-15 ) ) ;
#13534=AXIS2_PLACEMENT_3D ( 'NONE', #20160, #48024, #8080 ) ;
#13535=ORIENTED_EDGE ( 'NONE', *, *, #38410, .T. ) ;
#13536=DIRECTION ( 'NONE',  ( 0.000000000000000000, 0.000000000000000000, 1.000000000000000000 ) ) ;
#13538=DIRECTION ( 'NONE',  ( 0.2059786187411021818, 0.000000000000000000, -0.9785564922995032555 ) ) ;
#13540=VERTEX_POINT ( 'NONE', #10055 ) ;
#13541=EDGE_CURVE ( 'NONE', #21790, #21281, #14256, .T. ) ;
#13542=ORIENTED_EDGE ( 'NONE', *, *, #26102, .F. ) ;
#13545=VERTEX_POINT ( 'NONE', #18454 ) ;
#13547=FACE_OUTER_BOUND ( 'NONE', #35434, .T. ) ;
#13549=CARTESIAN_POINT ( 'NONE',  ( -168.0489871616337325, -175.3837268820161057, -32.84887689123905119 ) ) ;
#13550=EDGE_CURVE ( 'NONE', #13353, #22103, #27737, .T. ) ;
#13552=EDGE_CURVE ( 'NONE', #22586, #17429, #30019, .T. ) ;
#13554=LINE ( 'NONE', #49829, #49355 ) ;
#13555=ORIENTED_EDGE ( 'NONE', *, *, #9284, .T. ) ;
#13557=ORIENTED_EDGE ( 'NONE', *, *, #30832, .T. ) ;
#13559=CARTESIAN_POINT ( 'NONE',  ( -88.23625491228467865, -177.1207230881787780, 118.5089480183148254 ) ) ;
#13560=ORIENTED_EDGE ( 'NONE', *, *, #3448, .T. ) ;
#13567=AXIS2_PLACEMENT_3D ( 'NONE', #21071, #1092, #21337 ) ;
#13569=FACE_BOUND ( 'NONE', #19373, .T. ) ;
#13570=ORIENTED_EDGE ( 'NONE', *, *, #6016, .T. ) ;
#13571=EDGE_CURVE ( 'NONE', #32376, #5586, #27631, .T. ) ;
#13572=CARTESIAN_POINT ( 'NONE',  ( -47.51449116960048968, -193.5000000000000000, -0.2635871660690578544 ) ) ;
#13574=ORIENTED_EDGE ( 'NONE', *, *, #6041, .F. ) ;
#13575=DIRECTION ( 'NONE',  ( -0.000000000000000000, 1.000000000000000000, -0.000000000000000000 ) ) ;
#13576=ORIENTED_EDGE ( 'NONE', *, *, #30111, .F. ) ;
#13577=VECTOR ( 'NONE', #32891, 1000.000000000000000 ) ;
#13579=DIRECTION ( 'NONE',  ( 0.000000000000000000, 0.000000000000000000, 1.000000000000000000 ) ) ;
#13581=DIRECTION ( 'NONE',  ( 0.000000000000000000, -1.000000000000000000, -0.000000000000000000 ) ) ;
#13585=CARTESIAN_POINT ( 'NONE',  ( -9.671950287350391307, -183.6283474603465606, -118.8234112238815499 ) ) ;
#13586=ORIENTED_EDGE ( 'NONE', *, *, #13978, .T. ) ;
#13587=EDGE_LOOP ( 'NONE', ( #40309, #11978, #34632, #36777 ) ) ;
#13588=ORIENTED_EDGE ( 'NONE', *, *, #47967, .F. ) ;
#13589=CARTESIAN_POINT ( 'NONE',  ( -48.18706998087187543, -189.7472609257535510, -0.9564009842765152092 ) ) ;
#13590=CARTESIAN_POINT ( 'NONE',  ( -47.92047998570519951, -177.1207230881787780, -0.8294056854501942189 ) ) ;
#13591=ORIENTED_EDGE ( 'NONE', *, *, #28788, .F. ) ;
#13592=DIRECTION ( 'NONE',  ( 0.7765238627180393038, 0.000000000000000000, 0.6300878435817147682 ) ) ;
#13594=LINE ( 'NONE', #4954, #13769 ) ;
#13596=ORIENTED_EDGE ( 'NONE', *, *, #34108, .T. ) ;
#13598=VECTOR ( 'NONE', #28370, 1000.000000000000000 ) ;
#13599=EDGE_CURVE ( 'NONE', #8154, #29294, #5603, .T. ) ;
#13602=ORIENTED_EDGE ( 'NONE', *, *, #20807, .T. ) ;
#13605=ORIENTED_EDGE ( 'NONE', *, *, #32772, .T. ) ;
#13609=ORIENTED_EDGE ( 'NONE', *, *, #4906, .T. ) ;
#13610=CYLINDRICAL_SURFACE ( 'NONE', #6167, 125.0000000000000000 ) ;
#13611=ADVANCED_FACE ( 'NONE', ( #33946 ), #14516, .T. ) ;
#13612=CARTESIAN_POINT ( 'NONE',  ( -173.0003472773501301, -189.7472609257535510, 10.93003379476953896 ) ) ;
#13614=EDGE_CURVE ( 'NONE', #46248, #9912, #26069, .T. ) ;
#13616=ORIENTED_EDGE ( 'NONE', *, *, #34591, .T. ) ;
#13617=VECTOR ( 'NONE', #41233, 1000.000000000000114 ) ;
#13621=EDGE_CURVE ( 'NONE', #47039, #32136, #6368, .T. ) ;
#13622=CARTESIAN_POINT ( 'NONE',  ( 14.72514937628683640, -189.7472609257535510, -106.6827995071083706 ) ) ;
#13624=CARTESIAN_POINT ( 'NONE',  ( -49.29161362951452929, -183.6283474603465606, -0.5829794791144748967 ) ) ;
#13628=LINE ( 'NONE', #41750, #25592 ) ;
#13631=DIRECTION ( 'NONE',  ( -0.8455960035018311727, 0.000000000000000000, 0.5338233779647826305 ) ) ;
#13632=ORIENTED_EDGE ( 'NONE', *, *, #28284, .T. ) ;
#13634=DIRECTION ( 'NONE',  ( -0.000000000000000000, 1.000000000000000000, -0.000000000000000000 ) ) ;
#13635=DIRECTION ( 'NONE',  ( -0.9720229140804139689, 0.000000000000000000, 0.2348860457809708036 ) ) ;
#13637=VERTEX_POINT ( 'NONE', #46573 ) ;
#13638=EDGE_CURVE ( 'NONE', #5249, #35097, #26328, .T. ) ;
#13639=AXIS2_PLACEMENT_3D ( 'NONE', #7364, #12313, #24413 ) ;
#13640=CARTESIAN_POINT ( 'NONE',  ( -169.6719064342497632, -183.6283474603465606, 30.61552143554992256 ) ) ;
#13643=CARTESIAN_POINT ( 'NONE',  ( -98.71382891444399377, -193.5000000000000000, -114.4616734920523555 ) ) ;
#13645=VECTOR ( 'NONE', #24436, 1000.000000000000000 ) ;
#13648=DIRECTION ( 'NONE',  ( 0.000000000000000000, 0.000000000000000000, -1.000000000000000000 ) ) ;
#13649=DIRECTION ( 'NONE',  ( 0.000000000000000000, 0.000000000000000000, 1.000000000000000000 ) ) ;
#13650=LINE ( 'NONE', #17358, #29157 ) ;
#13651=DIRECTION ( 'NONE',  ( -0.8757349421956310831, 0.000000000000000000, -0.4827922027307550712 ) ) ;
#13652=AXIS2_PLACEMENT_3D ( 'NONE', #9983, #2067, #13649 ) ;
#13653=ORIENTED_EDGE ( 'NONE', *, *, #43262, .T. ) ;
#13654=AXIS2_PLACEMENT_3D ( 'NONE', #5100, #24284, #33197 ) ;
#13655=LINE ( 'NONE', #12872, #19746 ) ;
#13658=VECTOR ( 'NONE', #47768, 1000.000000000000114 ) ;
#13659=VECTOR ( 'NONE', #4551, 1000.000000000000114 ) ;
#13663=VERTEX_POINT ( 'NONE', #35754 ) ;
#13668=ORIENTED_EDGE ( 'NONE', *, *, #37586, .F. ) ;
#13670=CARTESIAN_POINT ( 'NONE',  ( 52.75081385575904136, -193.5000000000000000, 71.61357856150600298 ) ) ;
#13671=ORIENTED_EDGE ( 'NONE', *, *, #7691, .T. ) ;
#13674=CARTESIAN_POINT ( 'NONE',  ( -137.2624501260119985, -193.5000000000000000, 87.99159897727967916 ) ) ;
#13676=ORIENTED_EDGE ( 'NONE', *, *, #41659, .T. ) ;
#13677=EDGE_CURVE ( 'NONE', #15110, #36975, #26055, .T. ) ;
#13680=CARTESIAN_POINT ( 'NONE',  ( -58.29063029684667896, -177.1207230881787780, 124.6143426664034735 ) ) ;
#13681=ORIENTED_EDGE ( 'NONE', *, *, #10878, .T. ) ;
#13682=ORIENTED_EDGE ( 'NONE', *, *, #38410, .F. ) ;
#13683=EDGE_CURVE ( 'NONE', #22697, #18236, #58, .T. ) ;
#13685=DIRECTION ( 'NONE',  ( 0.000000000000000000, 0.000000000000000000, 1.000000000000000000 ) ) ;
#13687=EDGE_CURVE ( 'NONE', #16507, #1774, #23926, .T. ) ;
#13688=DIRECTION ( 'NONE',  ( 0.000000000000000000, 0.000000000000000000, -1.000000000000000000 ) ) ;
#13690=DIRECTION ( 'NONE',  ( 0.2059786187411021818, 0.000000000000000000, -0.9785564922995032555 ) ) ;
#13692=CARTESIAN_POINT ( 'NONE',  ( -92.78132261338707565, -193.5000000000000000, -116.8859077982276773 ) ) ;
#13693=DIRECTION ( 'NONE',  ( -0.000000000000000000, 1.000000000000000000, -0.000000000000000000 ) ) ;
#13694=ORIENTED_EDGE ( 'NONE', *, *, #22622, .T. ) ;
#13696=DIRECTION ( 'NONE',  ( -0.000000000000000000, 1.000000000000000000, -0.000000000000000000 ) ) ;
#13700=ORIENTED_EDGE ( 'NONE', *, *, #27233, .F. ) ;
#13701=AXIS2_PLACEMENT_3D ( 'NONE', #45516, #50500, #14495 ) ;
#13702=DIRECTION ( 'NONE',  ( 0.9027978299657446470, 0.000000000000000000, -0.4300652022765183435 ) ) ;
#13703=FACE_OUTER_BOUND ( 'NONE', #4577, .T. ) ;
#13704=DIRECTION ( 'NONE',  ( 0.000000000000000000, -0.000000000000000000, -1.000000000000000000 ) ) ;
#13708=DIRECTION ( 'NONE',  ( -0.000000000000000000, 1.000000000000000000, -0.000000000000000000 ) ) ;
#13709=DIRECTION ( 'NONE',  ( -0.8757349421956310831, 0.000000000000000000, -0.4827922027307550712 ) ) ;
#13710=FACE_OUTER_BOUND ( 'NONE', #25567, .T. ) ;
#13711=ORIENTED_EDGE ( 'NONE', *, *, #12114, .T. ) ;
#13713=ORIENTED_EDGE ( 'NONE', *, *, #3514, .F. ) ;
#13714=CARTESIAN_POINT ( 'NONE',  ( -172.1341525481709880, -193.5000000000000000, 18.28755301364337527 ) ) ;
#13717=CARTESIAN_POINT ( 'NONE',  ( -66.64622755927948106, -193.5000000000000000, 123.6727797384707515 ) ) ;
#13719=ORIENTED_EDGE ( 'NONE', *, *, #20608, .F. ) ;
#13720=ORIENTED_EDGE ( 'NONE', *, *, #48437, .F. ) ;
#13726=CARTESIAN_POINT ( 'NONE',  ( -159.0901268547125653, -183.6283474603465606, 58.22548115875957109 ) ) ;
#13727=CIRCLE ( 'NONE', #38890, 125.0000000000000000 ) ;
#13728=ORIENTED_EDGE ( 'NONE', *, *, #36196, .T. ) ;
#13729=ADVANCED_FACE ( 'NONE', ( #34991 ), #39682, .T. ) ;
#13730=CARTESIAN_POINT ( 'NONE',  ( -48.36085358058748085, -193.5000000000000000, -0.9929810960135100339 ) ) ;
#13731=PLANE ( 'NONE',  #25797 ) ;
#13734=EDGE_CURVE ( 'NONE', #25410, #48442, #22724, .T. ) ;
#13735=ADVANCED_FACE ( 'NONE', ( #11837 ), #47864, .F. ) ;
#13736=CARTESIAN_POINT ( 'NONE',  ( -69.77312546433408613, -175.3837268820161057, 123.1729094355499967 ) ) ;
#13739=ORIENTED_EDGE ( 'NONE', *, *, #5725, .T. ) ;
#13740=CARTESIAN_POINT ( 'NONE',  ( -48.47912675150885065, -183.6283474603465606, 6.938893903907228378E-15 ) ) ;
#13741=EDGE_CURVE ( 'NONE', #43244, #5084, #7646, .T. ) ;
#13742=CYLINDRICAL_SURFACE ( 'NONE', #12894, 125.0000000000000000 ) ;
#13743=CARTESIAN_POINT ( 'NONE',  ( -13.05859477122062273, -175.3837268820161057, -118.8334608768479796 ) ) ;
#13747=ORIENTED_EDGE ( 'NONE', *, *, #19651, .F. ) ;
#13750=DIRECTION ( 'NONE',  ( 0.000000000000000000, 0.000000000000000000, 1.000000000000000000 ) ) ;
#13752=DIRECTION ( 'NONE',  ( -0.000000000000000000, 1.000000000000000000, -0.000000000000000000 ) ) ;
#13753=AXIS2_PLACEMENT_3D ( 'NONE', #8071, #173, #20409 ) ;
#13755=ORIENTED_EDGE ( 'NONE', *, *, #13916, .F. ) ;
#13756=PLANE ( 'NONE',  #32603 ) ;
#13757=DIRECTION ( 'NONE',  ( 0.000000000000000000, 0.000000000000000000, 1.000000000000000000 ) ) ;
#13758=CIRCLE ( 'NONE', #40591, 125.0000000000000000 ) ;
#13759=ORIENTED_EDGE ( 'NONE', *, *, #35320, .T. ) ;
#13763=CARTESIAN_POINT ( 'NONE',  ( -105.7090724259148118, -175.3837268820161057, 111.1293539894142839 ) ) ;
#13765=ORIENTED_EDGE ( 'NONE', *, *, #42268, .F. ) ;
#13766=DIRECTION ( 'NONE',  ( 0.000000000000000000, -1.000000000000000000, 0.000000000000000000 ) ) ;
#13768=CARTESIAN_POINT ( 'NONE',  ( 58.48829670243886625, -193.5000000000000000, -64.67588669375805921 ) ) ;
#13769=VECTOR ( 'NONE', #9925, 1000.000000000000000 ) ;
#13770=CARTESIAN_POINT ( 'NONE',  ( 76.21810084846656252, -183.6283474603465606, -8.694908215727984668 ) ) ;
#13771=EDGE_CURVE ( 'NONE', #26852, #39115, #16310, .T. ) ;
#13773=PLANE ( 'NONE',  #3597 ) ;
#13775=PLANE ( 'NONE',  #49634 ) ;
#13777=EDGE_LOOP ( 'NONE', ( #34667, #8601, #8450, #3873 ) ) ;
#13782=DIRECTION ( 'NONE',  ( 0.000000000000000000, 1.000000000000000000, 0.000000000000000000 ) ) ;
#13784=DIRECTION ( 'NONE',  ( 0.000000000000000000, 0.000000000000000000, -1.000000000000000000 ) ) ;
#13786=AXIS2_PLACEMENT_3D ( 'NONE', #27942, #41580, #50008 ) ;
#13789=ADVANCED_FACE ( 'NONE', ( #36527 ), #40468, .T. ) ;
#13790=EDGE_CURVE ( 'NONE', #23116, #14590, #32598, .T. ) ;
#13793=EDGE_LOOP ( 'NONE', ( #1963, #40748, #14602, #29411 ) ) ;
#13798=LINE ( 'NONE', #10626, #12350 ) ;
#13799=CARTESIAN_POINT ( 'NONE',  ( -157.8637630444124795, -193.5000000000000000, -60.49794494914009135 ) ) ;
#13801=CARTESIAN_POINT ( 'NONE',  ( -112.1919339979530150, -189.7472609257535510, 107.5438431188761825 ) ) ;
#13802=DIRECTION ( 'NONE',  ( 0.7378332790417189146, 0.000000000000000000, 0.6749830015182196608 ) ) ;
#13806=VECTOR ( 'NONE', #28769, 1000.000000000000000 ) ;
#13807=ORIENTED_EDGE ( 'NONE', *, *, #21333, .T. ) ;
#13809=ORIENTED_EDGE ( 'NONE', *, *, #42407, .F. ) ;
#13810=VERTEX_POINT ( 'NONE', #41251 ) ;
#13812=FACE_OUTER_BOUND ( 'NONE', #2327, .T. ) ;
#13815=CARTESIAN_POINT ( 'NONE',  ( -93.85419746441394295, -193.5000000000000000, 115.4006183233324805 ) ) ;
#13819=VERTEX_POINT ( 'NONE', #36806 ) ;
#13821=ORIENTED_EDGE ( 'NONE', *, *, #38469, .T. ) ;
#13822=DIRECTION ( 'NONE',  ( 0.000000000000000000, 0.000000000000000000, 1.000000000000000000 ) ) ;
#13824=FACE_OUTER_BOUND ( 'NONE', #27949, .T. ) ;
#13827=VECTOR ( 'NONE', #31794, 999.9999999999998863 ) ;
#13828=CARTESIAN_POINT ( 'NONE',  ( -238.7407812814481076, -213.5000000000000000, -9.999999999999987566 ) ) ;
#13829=CARTESIAN_POINT ( 'NONE',  ( -0.3054481938615516423, -193.5000000000000000, 115.3442529744090450 ) ) ;
#13830=DIRECTION ( 'NONE',  ( 0.000000000000000000, 0.000000000000000000, -1.000000000000000000 ) ) ;
#13832=AXIS2_PLACEMENT_3D ( 'NONE', #10916, #26933, #3023 ) ;
#13836=ORIENTED_EDGE ( 'NONE', *, *, #35560, .F. ) ;
#13837=AXIS2_PLACEMENT_3D ( 'NONE', #33890, #13931, #49437 ) ;
#13839=VERTEX_POINT ( 'NONE', #12617 ) ;
#13840=ORIENTED_EDGE ( 'NONE', *, *, #44337, .T. ) ;
#13841=DIRECTION ( 'NONE',  ( -0.2348860457809911206, 0.000000000000000000, 0.9720229140804089729 ) ) ;
#13842=VECTOR ( 'NONE', #33702, 1000.000000000000000 ) ;
#13845=DIRECTION ( 'NONE',  ( 0.000000000000000000, -1.000000000000000000, 0.000000000000000000 ) ) ;
#13846=DIRECTION ( 'NONE',  ( -0.1182731709213523247, 0.000000000000000000, -0.9929810960135185827 ) ) ;
#13847=DIRECTION ( 'NONE',  ( -0.000000000000000000, 1.000000000000000000, -0.000000000000000000 ) ) ;
#13848=ORIENTED_EDGE ( 'NONE', *, *, #45895, .F. ) ;
#13849=EDGE_CURVE ( 'NONE', #36957, #44616, #273, .T. ) ;
#13850=EDGE_CURVE ( 'NONE', #39091, #49365, #22276, .T. ) ;
#13855=ORIENTED_EDGE ( 'NONE', *, *, #28113, .F. ) ;
#13856=LINE ( 'NONE', #21224, #2428 ) ;
#13857=CARTESIAN_POINT ( 'NONE',  ( 49.10711742958949344, -189.7472609257535510, 78.11481899503480975 ) ) ;
#13858=VECTOR ( 'NONE', #2046, 1000.000000000000000 ) ;
#13864=CIRCLE ( 'NONE', #49960, 124.9999999999999858 ) ;
#13865=VECTOR ( 'NONE', #5782, 999.9999999999998863 ) ;
#13866=DIRECTION ( 'NONE',  ( 0.7765238627180482966, 0.000000000000000000, -0.6300878435817038881 ) ) ;
#13867=ORIENTED_EDGE ( 'NONE', *, *, #4016, .F. ) ;
#13868=DIRECTION ( 'NONE',  ( 0.02963332782254913048, 0.000000000000000000, 0.9995608365087946812 ) ) ;
#13869=ORIENTED_EDGE ( 'NONE', *, *, #40425, .F. ) ;
#13870=VERTEX_POINT ( 'NONE', #8422 ) ;
#13871=AXIS2_PLACEMENT_3D ( 'NONE', #46263, #46011, #25241 ) ;
#13872=EDGE_CURVE ( 'NONE', #31730, #45161, #24449, .T. ) ;
#13873=ORIENTED_EDGE ( 'NONE', *, *, #7630, .F. ) ;
#13875=LINE ( 'NONE', #7216, #9655 ) ;
#13876=VECTOR ( 'NONE', #21147, 1000.000000000000000 ) ;
#13877=EDGE_LOOP ( 'NONE', ( #9569, #45667, #24764, #6638 ) ) ;
#13878=DIRECTION ( 'NONE',  ( 0.000000000000000000, 0.000000000000000000, 1.000000000000000000 ) ) ;
#13879=DIRECTION ( 'NONE',  ( 0.000000000000000000, -1.000000000000000000, 0.000000000000000000 ) ) ;
#13880=ORIENTED_EDGE ( 'NONE', *, *, #11541, .F. ) ;
#13882=AXIS2_PLACEMENT_3D ( 'NONE', #1596, #26262, #2089 ) ;
#13884=EDGE_CURVE ( 'NONE', #1575, #11111, #1267, .T. ) ;
#13886=VERTEX_POINT ( 'NONE', #40997 ) ;
#13887=DIRECTION ( 'NONE',  ( -0.9473263538541946138, 0.000000000000000000, 0.3202698538628279690 ) ) ;
#13888=LINE ( 'NONE', #42508, #1236 ) ;
#13889=DIRECTION ( 'NONE',  ( -0.000000000000000000, 1.000000000000000000, -0.000000000000000000 ) ) ;
#13890=FACE_OUTER_BOUND ( 'NONE', #39215, .T. ) ;
#13893=CARTESIAN_POINT ( 'NONE',  ( -48.02249751411513756, -193.5000000000000000, -0.8896570909947397743 ) ) ;
#13894=CARTESIAN_POINT ( 'NONE',  ( -49.38192458147459263, -177.1207230881787780, -0.4300652022765235616 ) ) ;
#13897=CYLINDRICAL_SURFACE ( 'NONE', #7845, 125.0000000000000000 ) ;
#13900=VERTEX_POINT ( 'NONE', #6047 ) ;
#13901=AXIS2_PLACEMENT_3D ( 'NONE', #11347, #26352, #22423 ) ;
#13902=DIRECTION ( 'NONE',  ( 0.000000000000000000, -1.000000000000000000, 0.000000000000000000 ) ) ;
#13906=CARTESIAN_POINT ( 'NONE',  ( -105.4063847101409692, -175.3837268820161057, -111.2847127925096231 ) ) ;
#13908=DIRECTION ( 'NONE',  ( -0.000000000000000000, 1.000000000000000000, -0.000000000000000000 ) ) ;
#13910=CARTESIAN_POINT ( 'NONE',  ( -48.47912675150885065, -183.6283474603465606, 6.938893903907228378E-15 ) ) ;
#13912=CIRCLE ( 'NONE', #43270, 125.0000000000000000 ) ;
#13915=CARTESIAN_POINT ( 'NONE',  ( 75.04604393171727850, -193.5000000000000000, -10.84123789944574234 ) ) ;
#13916=EDGE_CURVE ( 'NONE', #23163, #7887, #42550, .T. ) ;
#13917=VECTOR ( 'NONE', #24220, 1000.000000000000000 ) ;
#13919=ORIENTED_EDGE ( 'NONE', *, *, #48451, .F. ) ;
#13920=DIRECTION ( 'NONE',  ( 0.000000000000000000, -0.000000000000000000, 1.000000000000000000 ) ) ;
#13921=ORIENTED_EDGE ( 'NONE', *, *, #16048, .T. ) ;
#13924=ORIENTED_EDGE ( 'NONE', *, *, #25578, .T. ) ;
#13925=CARTESIAN_POINT ( 'NONE',  ( -64.08700758308647494, -193.5000000000000000, -124.0217483183786840 ) ) ;
#13926=ORIENTED_EDGE ( 'NONE', *, *, #35612, .T. ) ;
#13927=LINE ( 'NONE', #29950, #46883 ) ;
#13929=ORIENTED_EDGE ( 'NONE', *, *, #40966, .T. ) ;
#13930=DIRECTION ( 'NONE',  ( 0.000000000000000000, 1.000000000000000000, 0.000000000000000000 ) ) ;
#13931=DIRECTION ( 'NONE',  ( -0.9842305779475992722, 0.000000000000000000, 0.1768902751225592818 ) ) ;
#13932=ORIENTED_EDGE ( 'NONE', *, *, #3241, .F. ) ;
#13933=VECTOR ( 'NONE', #11284, 1000.000000000000227 ) ;
#13934=EDGE_CURVE ( 'NONE', #11778, #28008, #9995, .T. ) ;
#13935=DIRECTION ( 'NONE',  ( 0.5338233779647948429, 0.000000000000000000, -0.8455960035018234011 ) ) ;
#13936=AXIS2_PLACEMENT_3D ( 'NONE', #33653, #550, #13688 ) ;
#13937=VERTEX_POINT ( 'NONE', #29425 ) ;
#13938=FACE_OUTER_BOUND ( 'NONE', #26179, .T. ) ;
#13939=ORIENTED_EDGE ( 'NONE', *, *, #13302, .T. ) ;
#13940=CIRCLE ( 'NONE', #9736, 125.0000000000000000 ) ;
#13944=EDGE_LOOP ( 'NONE', ( #30602, #14018, #28509, #37379 ) ) ;
#13945=ORIENTED_EDGE ( 'NONE', *, *, #11825, .T. ) ;
#13946=DIRECTION ( 'NONE',  ( -0.000000000000000000, 1.000000000000000000, -0.000000000000000000 ) ) ;
#13947=VERTEX_POINT ( 'NONE', #18645 ) ;
#13954=DIRECTION ( 'NONE',  ( -0.000000000000000000, 1.000000000000000000, -0.000000000000000000 ) ) ;
#13955=DIRECTION ( 'NONE',  ( -0.7765238627180349740, 0.000000000000000000, -0.6300878435817203194 ) ) ;
#13958=DIRECTION ( 'NONE',  ( -0.000000000000000000, 1.000000000000000000, -0.000000000000000000 ) ) ;
#13960=AXIS2_PLACEMENT_3D ( 'NONE', #43225, #34811, #35089 ) ;
#13965=CARTESIAN_POINT ( 'NONE',  ( -48.47912675150885065, -183.6283474603465606, 6.938893903907228378E-15 ) ) ;
#13966=EDGE_CURVE ( 'NONE', #16290, #12249, #14702, .T. ) ;
#13968=CARTESIAN_POINT ( 'NONE',  ( 73.03012110230136500, -193.5000000000000000, 24.72869175143111420 ) ) ;
#13971=AXIS2_PLACEMENT_3D ( 'NONE', #7118, #43109, #23154 ) ;
#13972=DIRECTION ( 'NONE',  ( 0.9890401873221644768, 0.000000000000000000, -0.1476465640024779702 ) ) ;
#13973=DIRECTION ( 'NONE',  ( -0.000000000000000000, 1.000000000000000000, -0.000000000000000000 ) ) ;
#13974=DIRECTION ( 'NONE',  ( 0.000000000000000000, 0.000000000000000000, 1.000000000000000000 ) ) ;
#13977=ORIENTED_EDGE ( 'NONE', *, *, #12754, .F. ) ;
#13978=EDGE_CURVE ( 'NONE', #39444, #39193, #34826, .T. ) ;
#13981=LINE ( 'NONE', #30009, #11914 ) ;
#13982=ORIENTED_EDGE ( 'NONE', *, *, #49749, .T. ) ;
#13984=ORIENTED_EDGE ( 'NONE', *, *, #5737, .F. ) ;
#13988=DIRECTION ( 'NONE',  ( 0.000000000000000000, 0.000000000000000000, 1.000000000000000000 ) ) ;
#13990=AXIS2_PLACEMENT_3D ( 'NONE', #9047, #20332, #44520 ) ;
#13991=CARTESIAN_POINT ( 'NONE',  ( -154.6193097927903182, -189.7472609257535510, -66.02470404298122730 ) ) ;
#13992=AXIS2_PLACEMENT_3D ( 'NONE', #49019, #36668, #40587 ) ;
#13993=CARTESIAN_POINT ( 'NONE',  ( -170.5806857741408180, -177.1207230881787780, -21.61797988633146872 ) ) ;
#13995=AXIS2_PLACEMENT_3D ( 'NONE', #40224, #15826, #44448 ) ;
#13996=DIRECTION ( 'NONE',  ( 0.000000000000000000, -1.000000000000000000, 0.000000000000000000 ) ) ;
#13997=DIRECTION ( 'NONE',  ( -0.000000000000000000, 1.000000000000000000, -0.000000000000000000 ) ) ;
#13998=DIRECTION ( 'NONE',  ( 0.000000000000000000, -0.000000000000000000, 1.000000000000000000 ) ) ;
#14000=EDGE_CURVE ( 'NONE', #32000, #4695, #34951, .T. ) ;
#14014=DIRECTION ( 'NONE',  ( -0.6068001458186002006, 0.000000000000000000, 0.7948544414133481562 ) ) ;
#14017=AXIS2_PLACEMENT_3D ( 'NONE', #4022, #4536, #51337 ) ;
#14018=ORIENTED_EDGE ( 'NONE', *, *, #24005, .F. ) ;
#14019=CARTESIAN_POINT ( 'NONE',  ( -99.62791064391784346, -193.5000000000000000, -114.0561348912352173 ) ) ;
#14020=DIRECTION ( 'NONE',  ( -0.000000000000000000, 1.000000000000000000, -0.000000000000000000 ) ) ;
#14021=ORIENTED_EDGE ( 'NONE', *, *, #46435, .T. ) ;
#14022=CARTESIAN_POINT ( 'NONE',  ( 68.79964045138289919, -177.1207230881787780, 43.25148278810711133 ) ) ;
#14023=ORIENTED_EDGE ( 'NONE', *, *, #27253, .F. ) ;
#14024=VECTOR ( 'NONE', #39703, 1000.000000000000000 ) ;
#14025=DIRECTION ( 'NONE',  ( 0.000000000000000000, 0.000000000000000000, -1.000000000000000000 ) ) ;
#14026=CARTESIAN_POINT ( 'NONE',  ( -32.98951909085346301, -193.5000000000000000, 123.0287672223652891 ) ) ;
#14027=CIRCLE ( 'NONE', #43392, 125.0000000000000000 ) ;
#14028=LINE ( 'NONE', #42126, #45505 ) ;
#14031=VECTOR ( 'NONE', #41030, 1000.000000000000114 ) ;
#14032=DIRECTION ( 'NONE',  ( -0.000000000000000000, 1.000000000000000000, -0.000000000000000000 ) ) ;
#14034=CARTESIAN_POINT ( 'NONE',  ( 37.29583330861160562, -189.7472609257535510, -89.54698061029594669 ) ) ;
#14038=DIRECTION ( 'NONE',  ( 0.7378332790417239107, 0.000000000000000000, 0.6749830015182142207 ) ) ;
#14039=ORIENTED_EDGE ( 'NONE', *, *, #45031, .F. ) ;
#14040=DIRECTION ( 'NONE',  ( -0.000000000000000000, -0.000000000000000000, 1.000000000000000000 ) ) ;
#14041=VECTOR ( 'NONE', #8118, 1000.000000000000000 ) ;
#14043=LINE ( 'NONE', #17203, #50384 ) ;
#14044=DIRECTION ( 'NONE',  ( 0.7765238627180393038, 0.000000000000000000, 0.6300878435817147682 ) ) ;
#14046=ORIENTED_EDGE ( 'NONE', *, *, #26880, .F. ) ;
#14047=DIRECTION ( 'NONE',  ( 0.000000000000000000, 1.000000000000000000, -0.000000000000000000 ) ) ;
#14048=EDGE_CURVE ( 'NONE', #9666, #8625, #2128, .T. ) ;
#14052=AXIS2_PLACEMENT_3D ( 'NONE', #9506, #41547, #2125 ) ;
#14053=EDGE_LOOP ( 'NONE', ( #2528, #15558, #19753, #26899 ) ) ;
#14055=CARTESIAN_POINT ( 'NONE',  ( -172.3334410065085933, -177.1207230881787780, -6.025661128238047226 ) ) ;
#14057=DIRECTION ( 'NONE',  ( 0.000000000000000000, 0.000000000000000000, -1.000000000000000000 ) ) ;
#14058=CARTESIAN_POINT ( 'NONE',  ( -48.47912675150885065, -177.1207230881787780, 6.938893903907228378E-15 ) ) ;
#14060=EDGE_CURVE ( 'NONE', #30477, #6939, #14452, .T. ) ;
#14062=FACE_OUTER_BOUND ( 'NONE', #28, .T. ) ;
#14063=ORIENTED_EDGE ( 'NONE', *, *, #4059, .T. ) ;
#14065=ORIENTED_EDGE ( 'NONE', *, *, #31357, .F. ) ;
#14066=DIRECTION ( 'NONE',  ( 0.000000000000000000, 1.000000000000000000, 0.000000000000000000 ) ) ;
#14067=DIRECTION ( 'NONE',  ( -0.000000000000000000, 1.000000000000000000, -0.000000000000000000 ) ) ;
#14068=CIRCLE ( 'NONE', #27471, 125.0000000000000000 ) ;
#14069=AXIS2_PLACEMENT_3D ( 'NONE', #21092, #1111, #17159 ) ;
#14070=AXIS2_PLACEMENT_3D ( 'NONE', #35380, #7020, #43015 ) ;
#14071=LINE ( 'NONE', #1454, #29558 ) ;
#14072=CARTESIAN_POINT ( 'NONE',  ( -162.9896759831413249, -177.1207230881787780, -50.12318939043961308 ) ) ;
#14078=ORIENTED_EDGE ( 'NONE', *, *, #14000, .T. ) ;
#14085=ORIENTED_EDGE ( 'NONE', *, *, #22640, .F. ) ;
#14086=EDGE_CURVE ( 'NONE', #44743, #26606, #38214, .T. ) ;
#14088=DIRECTION ( 'NONE',  ( 0.9720229140804089729, 0.000000000000000000, 0.2348860457809911206 ) ) ;
#14091=FACE_OUTER_BOUND ( 'NONE', #36190, .T. ) ;
#14093=CIRCLE ( 'NONE', #25865, 125.0000000000000000 ) ;
#14094=EDGE_CURVE ( 'NONE', #34425, #34216, #2610, .T. ) ;
#14095=CARTESIAN_POINT ( 'NONE',  ( -156.2577088867455473, -177.1207230881787780, -63.31490529818420754 ) ) ;
#14097=PLANE ( 'NONE',  #2861 ) ;
#14098=DIRECTION ( 'NONE',  ( 0.000000000000000000, -1.000000000000000000, 0.000000000000000000 ) ) ;
#14099=ADVANCED_FACE ( 'NONE', ( #27800 ), #42808, .T. ) ;
#14101=EDGE_CURVE ( 'NONE', #22800, #29344, #39157, .T. ) ;
#14102=LINE ( 'NONE', #10395, #9368 ) ;
#14103=ORIENTED_EDGE ( 'NONE', *, *, #35216, .T. ) ;
#14105=EDGE_CURVE ( 'NONE', #17063, #1035, #14973, .T. ) ;
#14107=ORIENTED_EDGE ( 'NONE', *, *, #10571, .F. ) ;
#14108=EDGE_LOOP ( 'NONE', ( #29264, #38167, #50837, #36684 ) ) ;
#14109=DIRECTION ( 'NONE',  ( 0.000000000000000000, 0.000000000000000000, -1.000000000000000000 ) ) ;
#14110=EDGE_CURVE ( 'NONE', #17428, #1806, #7340, .T. ) ;
#14112=EDGE_CURVE ( 'NONE', #13304, #47014, #19163, .T. ) ;
#14113=VECTOR ( 'NONE', #48659, 1000.000000000000227 ) ;
#14114=DIRECTION ( 'NONE',  ( -0.000000000000000000, 1.000000000000000000, -0.000000000000000000 ) ) ;
#14115=EDGE_CURVE ( 'NONE', #28621, #37366, #35430, .T. ) ;
#14116=DIRECTION ( 'NONE',  ( 0.6068001458185945385, 0.000000000000000000, -0.7948544414133523750 ) ) ;
#14117=DIRECTION ( 'NONE',  ( 0.000000000000000000, 0.000000000000000000, -1.000000000000000000 ) ) ;
#14118=ORIENTED_EDGE ( 'NONE', *, *, #18313, .F. ) ;
#14119=FACE_OUTER_BOUND ( 'NONE', #8687, .T. ) ;
#14121=LINE ( 'NONE', #41704, #14307 ) ;
#14126=ORIENTED_EDGE ( 'NONE', *, *, #41272, .T. ) ;
#14127=CARTESIAN_POINT ( 'NONE',  ( 31.28129687248616619, -177.1207230881787780, 96.24590808611479531 ) ) ;
#14129=DIRECTION ( 'NONE',  ( 0.9995608365087942371, 0.000000000000000000, 0.02963332782256331357 ) ) ;
#14130=AXIS2_PLACEMENT_3D ( 'NONE', #30938, #43019, #23053 ) ;
#14131=VECTOR ( 'NONE', #51288, 1000.000000000000000 ) ;
#14133=DIRECTION ( 'NONE',  ( -0.2920567706369833760, 0.000000000000000000, 0.9564009842765202052 ) ) ;
#14134=DIRECTION ( 'NONE',  ( -0.000000000000000000, 1.000000000000000000, -0.000000000000000000 ) ) ;
#14136=AXIS2_PLACEMENT_3D ( 'NONE', #25545, #36860, #25290 ) ;
#14138=ADVANCED_FACE ( 'NONE', ( #31232 ), #51744, .F. ) ;
#14139=CARTESIAN_POINT ( 'NONE',  ( -47.63353074800703268, -183.6283474603465606, 0.5338233779648018373 ) ) ;
#14140=ORIENTED_EDGE ( 'NONE', *, *, #27084, .T. ) ;
#14141=DIRECTION ( 'NONE',  ( 0.000000000000000000, 1.000000000000000000, 0.000000000000000000 ) ) ;
#14142=ORIENTED_EDGE ( 'NONE', *, *, #48504, .F. ) ;
#14143=VECTOR ( 'NONE', #27281, 1000.000000000000000 ) ;
#14145=CARTESIAN_POINT ( 'NONE',  ( -169.2746641285359317, -189.7472609257535510, -32.14713283941908628 ) ) ;
#14147=CARTESIAN_POINT ( 'NONE',  ( -32.87124591993210743, -189.7472609257535510, 124.0217483183788261 ) ) ;
#14148=VERTEX_POINT ( 'NONE', #2864 ) ;
#14151=ORIENTED_EDGE ( 'NONE', *, *, #36153, .F. ) ;
#14152=PLANE ( 'NONE',  #29194 ) ;
#14153=VERTEX_POINT ( 'NONE', #3635 ) ;
#14154=VECTOR ( 'NONE', #4437, 1000.000000000000000 ) ;
#14156=CARTESIAN_POINT ( 'NONE',  ( -170.9669310976187830, -189.7472609257535510, -24.93467037017131105 ) ) ;
#14157=CARTESIAN_POINT ( 'NONE',  ( 27.23560471289044571, -193.5000000000000000, 99.45993886622845537 ) ) ;
#14159=LINE ( 'NONE', #1014, #17344 ) ;
#14160=ORIENTED_EDGE ( 'NONE', *, *, #3512, .F. ) ;
#14161=CARTESIAN_POINT ( 'NONE',  ( 74.31448861501726810, -193.5000000000000000, -23.38221600314288651 ) ) ;
#14162=LINE ( 'NONE', #34874, #27274 ) ;
#14163=EDGE_CURVE ( 'NONE', #28107, #2431, #39880, .T. ) ;
#14167=EDGE_LOOP ( 'NONE', ( #44213, #51520, #35331, #29645 ) ) ;
#14168=LINE ( 'NONE', #30186, #7039 ) ;
#14170=EDGE_CURVE ( 'NONE', #21107, #15488, #11524, .T. ) ;
#14171=EDGE_CURVE ( 'NONE', #26317, #26852, #5606, .T. ) ;
#14172=DIRECTION ( 'NONE',  ( 0.000000000000000000, 1.000000000000000000, -0.000000000000000000 ) ) ;
#14174=ORIENTED_EDGE ( 'NONE', *, *, #33184, .T. ) ;
#14179=DIRECTION ( 'NONE',  ( 0.9027978299657387629, 0.000000000000000000, 0.4300652022765304450 ) ) ;
#14181=CYLINDRICAL_SURFACE ( 'NONE', #31284, 125.0000000000000000 ) ;
#14183=AXIS2_PLACEMENT_3D ( 'NONE', #28573, #48833, #44615 ) ;
#14185=CARTESIAN_POINT ( 'NONE',  ( -171.9128728525929262, -189.7472609257535510, 11.83705339977325011 ) ) ;
#14186=CARTESIAN_POINT ( 'NONE',  ( 35.67816836544800907, -177.1207230881787780, -92.42591454022745268 ) ) ;
#14187=LINE ( 'NONE', #13915, #26651 ) ;
#14195=ORIENTED_EDGE ( 'NONE', *, *, #15475, .F. ) ;
#14197=DIRECTION ( 'NONE',  ( -0.000000000000000000, 0.000000000000000000, 1.000000000000000000 ) ) ;
#14199=ORIENTED_EDGE ( 'NONE', *, *, #195, .F. ) ;
#14200=CARTESIAN_POINT ( 'NONE',  ( -170.8336150310144887, -175.3837268820161057, 25.58083653558494319 ) ) ;
#14201=CARTESIAN_POINT ( 'NONE',  ( -7.223120065443619175, -177.1207230881787780, 117.9955164924470523 ) ) ;
#14202=ORIENTED_EDGE ( 'NONE', *, *, #22622, .F. ) ;
#14203=DIRECTION ( 'NONE',  ( 0.000000000000000000, -0.000000000000000000, -1.000000000000000000 ) ) ;
#14204=VERTEX_POINT ( 'NONE', #43068 ) ;
#14205=CARTESIAN_POINT ( 'NONE',  ( 70.91428087927182844, -189.7472609257535510, -33.48461921608517855 ) ) ;
#14209=CYLINDRICAL_SURFACE ( 'NONE', #588, 125.0000000000000000 ) ;
#14210=CYLINDRICAL_SURFACE ( 'NONE', #44136, 125.0000000000000000 ) ;
#14211=VERTEX_POINT ( 'NONE', #23105 ) ;
#14212=VERTEX_POINT ( 'NONE', #992 ) ;
#14214=LINE ( 'NONE', #46274, #12248 ) ;
#14215=VERTEX_POINT ( 'NONE', #8103 ) ;
#14217=DIRECTION ( 'NONE',  ( -0.9646355819083556327, 0.000000000000000000, -0.2635871660690782825 ) ) ;
#14218=ORIENTED_EDGE ( 'NONE', *, *, #1130, .F. ) ;
#14219=FACE_OUTER_BOUND ( 'NONE', #11680, .T. ) ;
#14221=DIRECTION ( 'NONE',  ( 0.000000000000000000, -0.000000000000000000, 1.000000000000000000 ) ) ;
#14223=LINE ( 'NONE', #18159, #5623 ) ;
#14225=ADVANCED_FACE ( 'NONE', ( #20442 ), #36461, .T. ) ;
#14226=CARTESIAN_POINT ( 'NONE',  ( -22.62315034598913144, -193.5000000000000000, 121.2748789083720737 ) ) ;
#14227=CARTESIAN_POINT ( 'NONE',  ( 60.58466639580034752, -175.3837268820161057, -61.07445476073404222 ) ) ;
#14228=AXIS2_PLACEMENT_3D ( 'NONE', #19812, #5561, #25514 ) ;
#14229=CARTESIAN_POINT ( 'NONE',  ( 64.44365795514079309, -175.3837268820161057, -53.60452120946194299 ) ) ;
#14230=ORIENTED_EDGE ( 'NONE', *, *, #20865, .T. ) ;
#14231=DIRECTION ( 'NONE',  ( -0.000000000000000000, 1.000000000000000000, -0.000000000000000000 ) ) ;
#14232=DIRECTION ( 'NONE',  ( -0.000000000000000000, 1.000000000000000000, -0.000000000000000000 ) ) ;
#14233=LINE ( 'NONE', #46045, #882 ) ;
#14234=DIRECTION ( 'NONE',  ( 0.000000000000000000, -1.000000000000000000, 0.000000000000000000 ) ) ;
#14237=CARTESIAN_POINT ( 'NONE',  ( -47.70260288879080690, -177.1207230881787780, -0.6300878435817026668 ) ) ;
#14238=EDGE_CURVE ( 'NONE', #32692, #17784, #12812, .T. ) ;
#14239=DIRECTION ( 'NONE',  ( -0.000000000000000000, 1.000000000000000000, -0.000000000000000000 ) ) ;
#14240=CARTESIAN_POINT ( 'NONE',  ( -101.0675409952199999, -193.5000000000000000, 113.3995532942341100 ) ) ;
#14241=AXIS2_PLACEMENT_3D ( 'NONE', #22, #16060, #8168 ) ;
#14242=VERTEX_POINT ( 'NONE', #8615 ) ;
#14244=DIRECTION ( 'NONE',  ( 0.000000000000000000, 0.000000000000000000, 1.000000000000000000 ) ) ;
#14246=VERTEX_POINT ( 'NONE', #20977 ) ;
#14247=ORIENTED_EDGE ( 'NONE', *, *, #34821, .T. ) ;
#14248=ORIENTED_EDGE ( 'NONE', *, *, #800, .F. ) ;
#14249=PLANE ( 'NONE',  #21707 ) ;
#14250=EDGE_CURVE ( 'NONE', #24816, #40259, #12169, .T. ) ;
#14251=CARTESIAN_POINT ( 'NONE',  ( -173.4190745413846457, -193.5000000000000000, -3.874202661594927211 ) ) ;
#14252=PLANE ( 'NONE',  #50683 ) ;
#14253=VERTEX_POINT ( 'NONE', #4171 ) ;
#14255=CARTESIAN_POINT ( 'NONE',  ( -16.77927958806651887, -183.6283474603465606, -120.9136869416130082 ) ) ;
#14256=LINE ( 'NONE', #49739, #47898 ) ;
#14258=FACE_OUTER_BOUND ( 'NONE', #17031, .T. ) ;
#14259=VERTEX_POINT ( 'NONE', #24147 ) ;
#14261=DIRECTION ( 'NONE',  ( 0.4566292373937200777, 0.000000000000000000, -0.8896570909947436601 ) ) ;
#14262=ORIENTED_EDGE ( 'NONE', *, *, #5437, .F. ) ;
#14263=CARTESIAN_POINT ( 'NONE',  ( -48.47912675150885065, -173.5000000000000284, 6.938893903907228378E-15 ) ) ;
#14264=ORIENTED_EDGE ( 'NONE', *, *, #26783, .F. ) ;
#14266=CARTESIAN_POINT ( 'NONE',  ( -72.96029774493612763, -177.1207230881787780, 122.5792489240759551 ) ) ;
#14267=DIRECTION ( 'NONE',  ( 0.000000000000000000, 0.000000000000000000, 1.000000000000000000 ) ) ;
#14268=EDGE_CURVE ( 'NONE', #47168, #27526, #48586, .T. ) ;
#14269=ORIENTED_EDGE ( 'NONE', *, *, #32403, .F. ) ;
#14270=LINE ( 'NONE', #10322, #46653 ) ;
#14271=DIRECTION ( 'NONE',  ( 0.000000000000000000, 1.000000000000000000, 0.000000000000000000 ) ) ;
#14272=VECTOR ( 'NONE', #14502, 1000.000000000000114 ) ;
#14273=ORIENTED_EDGE ( 'NONE', *, *, #49159, .F. ) ;
#14274=DIRECTION ( 'NONE',  ( -0.000000000000000000, 1.000000000000000000, 0.000000000000000000 ) ) ;
#14275=DIRECTION ( 'NONE',  ( -0.000000000000000000, 1.000000000000000000, -0.000000000000000000 ) ) ;
#14276=ORIENTED_EDGE ( 'NONE', *, *, #34047, .F. ) ;
#14277=ADVANCED_FACE ( 'NONE', ( #20186 ), #12563, .F. ) ;
#14278=DIRECTION ( 'NONE',  ( 0.000000000000000000, 0.000000000000000000, 1.000000000000000000 ) ) ;
#14282=ORIENTED_EDGE ( 'NONE', *, *, #13790, .T. ) ;
#14284=ORIENTED_EDGE ( 'NONE', *, *, #13541, .T. ) ;
#14289=DIRECTION ( 'NONE',  ( 0.000000000000000000, -1.000000000000000000, 0.000000000000000000 ) ) ;
#14290=DIRECTION ( 'NONE',  ( 0.000000000000000000, 0.000000000000000000, 1.000000000000000000 ) ) ;
#14291=FACE_OUTER_BOUND ( 'NONE', #11206, .T. ) ;
#14293=VERTEX_POINT ( 'NONE', #24646 ) ;
#14294=VECTOR ( 'NONE', #49269, 1000.000000000000000 ) ;
#14295=FACE_OUTER_BOUND ( 'NONE', #48062, .T. ) ;
#14296=VERTEX_POINT ( 'NONE', #13082 ) ;
#14298=EDGE_CURVE ( 'NONE', #33552, #6834, #48048, .T. ) ;
#14300=CARTESIAN_POINT ( 'NONE',  ( -48.13092511607445090, -193.5000000000000000, -0.9374196611341135688 ) ) ;
#14301=ORIENTED_EDGE ( 'NONE', *, *, #43060, .F. ) ;
#14303=CARTESIAN_POINT ( 'NONE',  ( -75.48985759771373694, -193.5000000000000000, -122.0467960216648606 ) ) ;
#14305=DIRECTION ( 'NONE',  ( 0.000000000000000000, 1.000000000000000000, 0.000000000000000000 ) ) ;
#14307=VECTOR ( 'NONE', #25419, 1000.000000000000000 ) ;
#14308=DIRECTION ( 'NONE',  ( 0.000000000000000000, 1.000000000000000000, 0.000000000000000000 ) ) ;
#14309=VERTEX_POINT ( 'NONE', #36745 ) ;
#14310=CARTESIAN_POINT ( 'NONE',  ( -12.10142301649613827, -175.3837268820161057, -118.5439281552630746 ) ) ;
#14311=DIRECTION ( 'NONE',  ( 0.9646355819083614058, 0.000000000000000000, -0.2635871660690581320 ) ) ;
#14313=CARTESIAN_POINT ( 'NONE',  ( -127.0132498732365889, -193.5000000000000000, 97.24912084693261249 ) ) ;
#14315=ORIENTED_EDGE ( 'NONE', *, *, #34957, .F. ) ;
#14316=EDGE_LOOP ( 'NONE', ( #30080, #8241, #22985, #36858 ) ) ;
#14317=PLANE ( 'NONE',  #33342 ) ;
#14318=CARTESIAN_POINT ( 'NONE',  ( -114.1105527140175155, -177.1207230881787780, 106.3838142112217611 ) ) ;
#14319=LINE ( 'NONE', #29306, #24529 ) ;
#14320=PLANE ( 'NONE',  #32245 ) ;
#14321=ORIENTED_EDGE ( 'NONE', *, *, #2522, .F. ) ;
#14322=EDGE_CURVE ( 'NONE', #23058, #17439, #743, .T. ) ;
#14324=EDGE_CURVE ( 'NONE', #26117, #15950, #25180, .T. ) ;
#14328=EDGE_LOOP ( 'NONE', ( #30565, #25282, #34102, #17928 ) ) ;
#14329=EDGE_LOOP ( 'NONE', ( #25019, #17401, #37000, #47201 ) ) ;
#14330=DIRECTION ( 'NONE',  ( -0.000000000000000000, 1.000000000000000000, -0.000000000000000000 ) ) ;
#14331=LINE ( 'NONE', #3525, #51866 ) ;
#14334=LINE ( 'NONE', #49827, #1577 ) ;
#14336=EDGE_CURVE ( 'NONE', #45141, #15701, #29850, .T. ) ;
#14337=CARTESIAN_POINT ( 'NONE',  ( 71.87891646118019651, -193.5000000000000000, -33.74820638215424395 ) ) ;
#14344=CARTESIAN_POINT ( 'NONE',  ( -48.47912675150885065, -177.1207230881787780, 6.938893903907228378E-15 ) ) ;
#14345=ORIENTED_EDGE ( 'NONE', *, *, #45609, .F. ) ;
#14347=LINE ( 'NONE', #34054, #26544 ) ;
#14349=LINE ( 'NONE', #10392, #17301 ) ;
#14351=CARTESIAN_POINT ( 'NONE',  ( -142.2007120195389405, -183.6283474603465606, 81.19354792697799894 ) ) ;
#14354=ORIENTED_EDGE ( 'NONE', *, *, #11242, .F. ) ;
#14355=CIRCLE ( 'NONE', #43721, 124.9999999999999858 ) ;
#14357=DIRECTION ( 'NONE',  ( 0.000000000000000000, -1.000000000000000000, 0.000000000000000000 ) ) ;
#14359=AXIS2_PLACEMENT_3D ( 'NONE', #37625, #42325, #26560 ) ;
#14360=DIRECTION ( 'NONE',  ( 0.000000000000000000, 0.000000000000000000, -1.000000000000000000 ) ) ;
#14361=ORIENTED_EDGE ( 'NONE', *, *, #11119, .T. ) ;
#14365=FACE_OUTER_BOUND ( 'NONE', #45629, .T. ) ;
#14366=CARTESIAN_POINT ( 'NONE',  ( -167.8725343822893308, -175.3837268820161057, 33.48461921608600278 ) ) ;
#14367=CARTESIAN_POINT ( 'NONE',  ( -150.5215542367829471, -189.7472609257535510, -72.19655804061974891 ) ) ;
#14368=ORIENTED_EDGE ( 'NONE', *, *, #14390, .T. ) ;
#14369=EDGE_LOOP ( 'NONE', ( #13869, #27468, #38682, #3519 ) ) ;
#14371=LINE ( 'NONE', #39042, #23399 ) ;
#14372=LINE ( 'NONE', #19101, #38591 ) ;
#14374=EDGE_CURVE ( 'NONE', #51005, #885, #37518, .T. ) ;
#14377=CARTESIAN_POINT ( 'NONE',  ( -48.47912675150885065, -175.3837268820161057, 6.938893903907228378E-15 ) ) ;
#14380=EDGE_CURVE ( 'NONE', #11828, #7505, #18122, .T. ) ;
#14382=EDGE_CURVE ( 'NONE', #48981, #43364, #5532, .T. ) ;
#14383=PLANE ( 'NONE',  #29073 ) ;
#14385=CARTESIAN_POINT ( 'NONE',  ( -142.9772358822569629, -177.1207230881787780, 81.82363577055969017 ) ) ;
#14386=ORIENTED_EDGE ( 'NONE', *, *, #28558, .F. ) ;
#14389=CARTESIAN_POINT ( 'NONE',  ( 11.61413489515541997, -183.6283474603465606, -109.6074810615842381 ) ) ;
#14390=EDGE_CURVE ( 'NONE', #38746, #45026, #23152, .T. ) ;
#14391=ORIENTED_EDGE ( 'NONE', *, *, #14413, .T. ) ;
#14393=VECTOR ( 'NONE', #10661, 1000.000000000000000 ) ;
#14395=FACE_OUTER_BOUND ( 'NONE', #50647, .T. ) ;
#14396=DIRECTION ( 'NONE',  ( 0.000000000000000000, 0.000000000000000000, 1.000000000000000000 ) ) ;
#14397=ORIENTED_EDGE ( 'NONE', *, *, #52036, .F. ) ;
#14399=DIRECTION ( 'NONE',  ( 0.2348860457809707758, 0.000000000000000000, 0.9720229140804138579 ) ) ;
#14402=EDGE_CURVE ( 'NONE', #18133, #40906, #8878, .T. ) ;
#14403=CIRCLE ( 'NONE', #22762, 125.0000000000000000 ) ;
#14405=CARTESIAN_POINT ( 'NONE',  ( -151.5051191635538146, -193.5000000000000000, -69.00559874123520387 ) ) ;
#14406=DIRECTION ( 'NONE',  ( 0.9960498426152171181, 0.000000000000000000, -0.08879589532293157006 ) ) ;
#14407=ADVANCED_FACE ( 'NONE', ( #30868 ), #37771, .F. ) ;
#14408=LINE ( 'NONE', #46218, #37079 ) ;
#14409=LINE ( 'NONE', #7993, #18190 ) ;
#14410=ORIENTED_EDGE ( 'NONE', *, *, #32061, .T. ) ;
#14411=CARTESIAN_POINT ( 'NONE',  ( -1.771278280434267272, -177.1207230881787780, -115.9455772817710226 ) ) ;
#14412=LINE ( 'NONE', #42513, #23938 ) ;
#14413=EDGE_CURVE ( 'NONE', #3228, #11975, #5476, .T. ) ;
#14415=DIRECTION ( 'NONE',  ( 0.8757349421956345248, 0.000000000000000000, 0.4827922027307490205 ) ) ;
#14417=VERTEX_POINT ( 'NONE', #18777 ) ;
#14418=DIRECTION ( 'NONE',  ( 0.000000000000000000, 1.000000000000000000, 0.000000000000000000 ) ) ;
#14419=CYLINDRICAL_SURFACE ( 'NONE', #518, 124.9999999999999858 ) ;
#14420=AXIS2_PLACEMENT_3D ( 'NONE', #21270, #25985, #17346 ) ;
#14422=CARTESIAN_POINT ( 'NONE',  ( -75.48985759771373694, -193.5000000000000000, -122.0467960216648606 ) ) ;
#14423=ORIENTED_EDGE ( 'NONE', *, *, #16107, .T. ) ;
#14425=LINE ( 'NONE', #10460, #11296 ) ;
#14426=DIRECTION ( 'NONE',  ( -0.4300652022765304450, 0.000000000000000000, 0.9027978299657387629 ) ) ;
#14427=ORIENTED_EDGE ( 'NONE', *, *, #47868, .T. ) ;
#14428=DIRECTION ( 'NONE',  ( 0.000000000000000000, 1.000000000000000000, 0.000000000000000000 ) ) ;
#14432=CARTESIAN_POINT ( 'NONE',  ( -3.104056038602969636, -177.1207230881787780, -115.4006183233321536 ) ) ;
#14434=AXIS2_PLACEMENT_3D ( 'NONE', #12633, #48395, #51829 ) ;
#14436=AXIS2_PLACEMENT_3D ( 'NONE', #44582, #49050, #48549 ) ;
#14439=VECTOR ( 'NONE', #23968, 1000.000000000000000 ) ;
#14445=DIRECTION ( 'NONE',  ( 0.000000000000000000, -0.000000000000000000, -1.000000000000000000 ) ) ;
#14447=EDGE_CURVE ( 'NONE', #21989, #31290, #9409, .T. ) ;
#14448=EDGE_CURVE ( 'NONE', #35821, #10145, #47496, .T. ) ;
#14449=AXIS2_PLACEMENT_3D ( 'NONE', #14300, #38192, #1691 ) ;
#14450=ADVANCED_FACE ( 'NONE', ( #6705 ), #22722, .F. ) ;
#14451=DIRECTION ( 'NONE',  ( -1.000000000000000000, 0.000000000000000000, -0.000000000000000000 ) ) ;
#14452=LINE ( 'NONE', #25756, #28108 ) ;
#14453=EDGE_LOOP ( 'NONE', ( #6161, #48211, #10993, #4800 ) ) ;
#14454=DIRECTION ( 'NONE',  ( 0.000000000000000000, 0.000000000000000000, 1.000000000000000000 ) ) ;
#14455=LINE ( 'NONE', #30982, #5481 ) ;
#14457=AXIS2_PLACEMENT_3D ( 'NONE', #41560, #17427, #49727 ) ;
#14460=ORIENTED_EDGE ( 'NONE', *, *, #34658, .F. ) ;
#14463=CARTESIAN_POINT ( 'NONE',  ( -48.02249751411513756, -175.3837268820161057, -0.8896570909947397743 ) ) ;
#14465=DIRECTION ( 'NONE',  ( 0.000000000000000000, -0.000000000000000000, 1.000000000000000000 ) ) ;
#14468=CARTESIAN_POINT ( 'NONE',  ( 47.91692961953209107, -175.3837268820161057, -77.99872144864700374 ) ) ;
#14469=VERTEX_POINT ( 'NONE', #23249 ) ;
#14470=FACE_OUTER_BOUND ( 'NONE', #49496, .T. ) ;
#14471=CARTESIAN_POINT ( 'NONE',  ( -116.2964108826154188, -183.6283474603465606, -105.0038855142073402 ) ) ;
#14472=EDGE_CURVE ( 'NONE', #32376, #30580, #15362, .T. ) ;
#14473=ORIENTED_EDGE ( 'NONE', *, *, #25390, .T. ) ;
#14475=CARTESIAN_POINT ( 'NONE',  ( -25.72842157752850056, -175.3837268820161057, 121.8950816227734606 ) ) ;
#14479=DIRECTION ( 'NONE',  ( -0.02963332782257007553, 0.000000000000000000, 0.9995608365087941261 ) ) ;
#14480=EDGE_CURVE ( 'NONE', #49617, #19338, #46641, .T. ) ;
#14481=VERTEX_POINT ( 'NONE', #36092 ) ;
#14484=EDGE_CURVE ( 'NONE', #35254, #31290, #2993, .T. ) ;
#14485=AXIS2_PLACEMENT_3D ( 'NONE', #8997, #45520, #25033 ) ;
#14486=PLANE ( 'NONE',  #7795 ) ;
#14487=ORIENTED_EDGE ( 'NONE', *, *, #45099, .T. ) ;
#14489=CARTESIAN_POINT ( 'NONE',  ( -151.9915035862630646, -177.1207230881787780, 70.07273251429431582 ) ) ;
#14490=DIRECTION ( 'NONE',  ( -0.5586467658036476935, 0.000000000000000000, -0.8294056854502049880 ) ) ;
#14491=CARTESIAN_POINT ( 'NONE',  ( -170.2790847791494855, -177.1207230881787780, -28.10285082451569494 ) ) ;
#14492=ORIENTED_EDGE ( 'NONE', *, *, #27666, .F. ) ;
#14493=AXIS2_PLACEMENT_3D ( 'NONE', #43887, #44147, #12866 ) ;
#14495=DIRECTION ( 'NONE',  ( 0.000000000000000000, -0.000000000000000000, -1.000000000000000000 ) ) ;
#14496=VECTOR ( 'NONE', #45701, 1000.000000000000000 ) ;
#14498=LINE ( 'NONE', #42599, #25348 ) ;
#14499=CARTESIAN_POINT ( 'NONE',  ( -8.169009709621407822, -177.1207230881787780, 118.3219948448695504 ) ) ;
#14501=ORIENTED_EDGE ( 'NONE', *, *, #45334, .T. ) ;
#14502=DIRECTION ( 'NONE',  ( -0.6528221181905280446, 0.000000000000000000, 0.7575112421616145841 ) ) ;
#14503=CARTESIAN_POINT ( 'NONE',  ( -49.42645310536303782, -177.1207230881787780, -0.3202698538628417357 ) ) ;
#14507=DIRECTION ( 'NONE',  ( 0.9720229140804123036, 0.000000000000000000, -0.2348860457809775759 ) ) ;
#14508=AXIS2_PLACEMENT_3D ( 'NONE', #32493, #40614, #41152 ) ;
#14510=EDGE_CURVE ( 'NONE', #19179, #20432, #40278, .T. ) ;
#14511=FACE_OUTER_BOUND ( 'NONE', #44415, .T. ) ;
#14512=FACE_OUTER_BOUND ( 'NONE', #32389, .T. ) ;
#14514=VECTOR ( 'NONE', #13973, 1000.000000000000000 ) ;
#14516=PLANE ( 'NONE',  #16018 ) ;
#14517=DIRECTION ( 'NONE',  ( -0.000000000000000000, 1.000000000000000000, -0.000000000000000000 ) ) ;
#14520=CARTESIAN_POINT ( 'NONE',  ( -48.65601702663143868, -193.5000000000000000, 0.9842305779476024918 ) ) ;
#14521=VERTEX_POINT ( 'NONE', #23499 ) ;
#14523=ORIENTED_EDGE ( 'NONE', *, *, #51071, .F. ) ;
#14524=DIRECTION ( 'NONE',  ( 0.000000000000000000, 1.000000000000000000, 0.000000000000000000 ) ) ;
#14525=CARTESIAN_POINT ( 'NONE',  ( 43.18784210722336780, -189.7472609257535510, -84.98333260264752198 ) ) ;
#14526=PLANE ( 'NONE',  #37470 ) ;
#14527=CIRCLE ( 'NONE', #43879, 125.0000000000000000 ) ;
#14528=AXIS2_PLACEMENT_3D ( 'NONE', #17855, #1298, #45993 ) ;
#14529=AXIS2_PLACEMENT_3D ( 'NONE', #31924, #47962, #7754 ) ;
#14530=EDGE_LOOP ( 'NONE', ( #4810, #50780, #36365, #35468 ) ) ;
#14532=FACE_OUTER_BOUND ( 'NONE', #31807, .T. ) ;
#14533=CARTESIAN_POINT ( 'NONE',  ( 57.61256176024322428, -193.5000000000000000, -64.19309449102732401 ) ) ;
#14535=EDGE_CURVE ( 'NONE', #49769, #6620, #50840, .T. ) ;
#14536=DIRECTION ( 'NONE',  ( 0.000000000000000000, 0.000000000000000000, -1.000000000000000000 ) ) ;
#14537=DIRECTION ( 'NONE',  ( 0.000000000000000000, 0.000000000000000000, 1.000000000000000000 ) ) ;
#14538=EDGE_LOOP ( 'NONE', ( #12305, #25554, #11118, #27180 ) ) ;
#14540=CLOSED_SHELL ( 'NONE', ( #26600, #22889, #17432, #9243, #24067, #20478, #44637, #7014, #18969, #1952, #31723, #1501, #2691, #22480, #4851, #43630, #49599, #28438, #31811, #25525, #8330, #44454, #24460, #3789, #4661, #9767, #33319, #16052, #49049, #36568, #30013, #25813, #38141, #12415, #13458, #11486, #33301, #42080, #16354, #26548, #9163, #46801, #21140, #24285, #29391, #43921, #6404, #39523, #30098, #9765, #37012, #46639, #418, #9594, #44955, #6962, #20082, #7116, #25296, #26635, #32646, #11807, #8491, #48180, #40069, #5326, #20813, #25543, #15460, #38172, #23811, #2845, #10694, #30536, #5128, #19559, #19961, #39052, #44880, #17456, #49337, #40292, #35929, #50078, #28482, #44309, #13611, #44944, #27268, #14138, #42524, #25031, #34660, #1753, #13059, #47582, #36927, #36861, #26642, #10515, #49493, #1793, #36207, #15699, #35862, #22473, #23521, #39620, #7566, #40466, #2852, #9285, #19044, #2177, #25861, #41430, #35687, #9577, #44019, #21941, #22316, #48403, #47500, #26527, #712, #5594, #10883, #562, #17927, #37899, #48519, #45580, #16958, #39127, #47222, #597, #11457, #13789, #35372, #28076, #11028, #9640, #31651, #46254, #13735, #46367, #1808, #34323, #12094, #12472, #24126, #42706, #35876, #34312, #36386, #39638, #36882, #18912, #3072, #4874, #15718, #15579, #20126, #1196, #9187, #20164, #3886, #19595, #49976, #18689, #8155, #7660, #29458, #23407, #16720, #21130, #32993, #1727, #2256, #40699, #36032, #42396, #29642, #8796, #192, #32251, #43326, #19893, #5283, #15994, #15722, #18276, #26967, #22686, #35566, #48150, #20661, #45442, #39896, #51285, #33235, #16953, #309, #5368, #48085, #27895, #5501, #35921, #33088, #14947, #17826, #3412, #11532, #26321, #49293, #35373, #21524, #25052, #28571, #611, #44304, #43579, #22342, #6103, #39462, #44376, #35604, #44472, #27197, #36728, #19841, #16066, #48790, #35167, #45902, #7282, #19274, #51394, #3111, #37516, #4976, #38007, #23248, #2459, #32720, #32770, #29731, #12710, #9283, #41921, #12476, #30254, #7092, #30061, #37746, #42499, #1220, #32591, #41426, #44870, #51845, #32994, #38347, #14791, #42328, #40832, #16673, #1212, #24299, #17906, #18886, #932, #33387, #25039, #19218, #23722, #6249, #13284, #46988, #24762, #21752, #28539, #42188, #17129, #36302, #40884, #8827, #13451, #42680, #4301, #40646, #9458, #1944, #20975, #43291, #15081, #20793, #4792, #42658, #6690, #43152, #12117, #13389, #2636, #29794, #30160, #38527, #24638, #18337, #26488, #16108, #45340, #33252, #22229, #33441, #39176, #50864, #2513, #24340, #33411, #8550, #47486, #34556, #43541, #253, #31034, #3238, #42765, #8267, #24972, #6334, #34839, #16356, #5976, #12037, #15341, #31478, #44240, #26141, #46164, #6617, #31169, #43518, #30802, #52021, #13309, #28979, #14099, #43637, #9898, #19082, #15741, #15395, #27841, #19901, #41154, #45531, #22148, #26670, #33207, #39948, #26008, #44824, #30194, #14407, #19837, #26006, #29395, #6616, #27772, #8205, #31472, #47756, #25907, #24698, #9083, #8926, #29436, #42197, #49868, #44446, #50757, #3841, #4466, #23568, #25308, #46291, #40595, #33698, #28495, #29435, #23738, #8917, #17, #17184, #24427, #2809, #37148, #26883, #45318, #3193, #7059, #19256, #16585, #2194, #26163, #29484, #29146, #9376, #34280, #41228, #38959, #16658, #37049, #40420, #22160, #43865, #51486, #15582, #11815, #4084, #38220, #9723, #16963, #20368, #33461, #22761, #48182, #9832, #38160, #42017, #13461, #3752, #29276, #20299, #5099, #30788, #36886, #32701, #29707, #34833, #4238, #42084, #8780, #51088, #45873, #43397, #16774, #27847, #47513, #31424, #50201, #39981, #30642, #41594, #20545, #45258, #5677, #45427, #11523, #46213, #40577, #24826, #35334, #48984, #50009, #17946, #49474, #27787, #12751, #35496, #22744, #13060, #13729, #33939, #47082, #34195, #29885, #14843, #17316, #17332, #26552, #47476, #32899, #20851, #5386, #38852, #46286, #17901, #12105, #25903, #21433, #17487, #17966, #34988, #25357, #32072, #37102, #11673, #5899, #46050, #33012, #34717, #29508, #24309, #43622, #7083, #25600, #37108, #26063, #12519, #47144, #17372, #43687, #5044, #31942, #16058, #13128, #14225, #50141, #40448, #15165, #21212, #29323, #3168, #13473, #13009, #45799, #3351, #40122, #21234, #35534, #18599, #27826, #43118, #9941, #8028, #51664, #15112, #15060, #48011, #21435, #40139, #50066, #28013, #20741, #37218, #48101, #43511, #3761, #30528, #25937, #30744, #23045, #8486, #27134, #7022, #35497, #32071, #16361, #35974, #6531, #44461, #44954, #39502, #36504, #37748, #17554, #45981, #44826, #25199, #50061, #30394, #11412, #22765, #50492, #46847, #26973, #18390, #18592, #49470, #33958, #43141, #3215, #4187, #34332, #23412, #48574, #50105, #51240, #1260, #34345, #34775, #16223, #50718, #22784, #36205, #32137, #23396, #12253, #34036, #37002, #39036, #22826, #28205, #16939, #1287, #1526, #6036, #24761, #33365, #36322, #29144, #14718, #41008, #33849, #51507, #48991, #6678, #4479, #11101, #27264, #16298, #31289, #19604, #7328, #1146, #25214, #45932, #41162, #3819, #21294, #7043, #37469, #46436, #31960, #1306, #34314, #31782, #682, #28253, #25291, #51955, #51470, #35277, #51299, #46684, #46552, #41363, #19016, #43349, #51026, #30441, #44918, #27216, #29394, #31916, #47798, #13492, #38185, #33883, #22101, #40965, #42010, #10387, #41026, #9875, #28835, #18180, #2529, #7760, #38763, #41247, #36743, #32665, #16501, #15733, #9055, #48764, #18489, #21658, #6116, #15217, #15054, #35213, #37542, #48545, #39400, #39415, #9253, #4088, #30509, #18580, #11170, #28726, #44740, #3691, #20923, #3389, #35549, #26091, #12345, #21851, #44771, #20627, #7373, #31845, #9491, #12889, #5453, #11699, #37886, #4223, #28178, #40070, #47855, #26185, #43617, #45537, #35421, #40395, #2472, #10600, #50704, #24872, #31795, #36559, #14691, #28898, #46667, #29030, #46064, #35105, #18663, #51521, #23430, #50689, #11104, #39459, #48818, #22459, #1390, #270, #37808, #4434, #4775, #37282, #47553, #6413, #18196, #47956, #51016, #25641, #1512, #8948, #26799, #10771, #50411, #21213, #9524, #29806, #4517, #15067, #12483, #546, #38467, #43528, #8324, #1131, #51995, #26299, #40276, #32066, #25417, #43327, #10836, #29658, #18179, #236, #763, #6267, #49766, #21184, #41317, #15166, #15328, #39838, #20124, #30613, #42044, #15480, #16126, #16652, #29683, #18755, #21804, #24486, #16937, #16289, #52032, #27956, #6471, #42639, #11352, #17910, #6689, #7187, #35342, #30935, #14277, #14632, #45617, #33650, #10612, #41448, #11067, #51416, #25989, #31413, #5768, #29515, #40649, #44874, #49909, #3358, #42772, #37192, #27667, #27261, #47753, #50695, #46916, #9239, #13316, #45532, #37222, #35924, #40337, #10171, #50406, #5137, #38547, #46557, #39460, #8445, #702, #7211, #7811, #5387, #23036, #29812, #43683, #50301, #6871, #28145, #11157, #7247, #36928, #47152, #16311, #1442, #22945, #38588, #45626, #19464, #30198, #51980, #26304, #15216, #11817, #7323, #37989, #4647, #30174, #22759, #36859, #44161, #5887, #2908, #49815, #27625, #31456, #15696, #23308, #32830, #18311, #27916, #561, #45487, #1570, #18013, #36114, #21055, #31983, #35281, #2482, #34739, #22095, #21390, #45543, #1638, #35847, #27587, #45560, #19229, #12944, #9885, #2862, #37401, #13079, #4795, #29239, #11545, #11409, #13088, #42066, #7738, #33938, #2144, #1764, #17298, #22449, #37163, #41103, #43034, #7736, #15422, #34688, #30444, #48629, #5198, #33259, #11835, #44726, #35209, #21818, #47200, #12834, #18603, #2830, #24961, #47589, #9312, #51348, #49115, #23923, #44596, #8978, #14743, #1655, #28190, #41393, #42613, #44121, #12950, #25848, #46999, #15942, #36907, #46845, #31647, #35783, #37449, #46779, #1640, #36692, #6131, #37288, #25644, #29684, #29501, #8501, #5829, #8876, #16584, #7320, #16932, #10178, #36782, #25358, #23056, #3755, #9428, #44932, #10255, #41953, #17668, #27630, #35623, #7753, #25293, #3701, #16695, #41221, #39984, #15047, #39360, #10407, #15355, #27066, #36216, #4728, #38605, #1721, #28606, #48679, #45623, #12474, #44957, #40706, #35147, #5614, #4675, #10291, #31418, #32505, #18245, #19773, #39744, #6021, #9056, #1070, #42956, #48972, #34909, #16715, #10903, #21455, #26271, #23869, #37373, #41067, #10625, #23471, #2711, #8279, #21436, #33093, #33122, #26672, #51379, #50740, #12772, #33393, #50652, #43811, #37213, #38990, #28998, #28665, #49710, #613, #27537, #3333, #20722, #49684, #40763, #28518, #42200, #35026, #25317, #47924, #42967, #51356, #27495, #22752, #37255, #17794, #15337, #16562, #13230, #23445, #3454, #27119, #26958, #39239, #6378, #42336, #51585, #26064, #26298, #3124, #48603, #51675, #10289, #26901, #16182, #36545, #14450, #7573 ) ) ;
#14542=EDGE_CURVE ( 'NONE', #3584, #6218, #39070, .T. ) ;
#14543=ORIENTED_EDGE ( 'NONE', *, *, #21289, .T. ) ;
#14545=ORIENTED_EDGE ( 'NONE', *, *, #25607, .F. ) ;
#14548=VERTEX_POINT ( 'NONE', #48193 ) ;
#14552=DIRECTION ( 'NONE',  ( 0.000000000000000000, -0.000000000000000000, -1.000000000000000000 ) ) ;
#14557=FACE_OUTER_BOUND ( 'NONE', #40527, .T. ) ;
#14558=DIRECTION ( 'NONE',  ( 0.9995608365087944591, 0.000000000000000000, -0.02963332782255633305 ) ) ;
#14559=DIRECTION ( 'NONE',  ( 0.9646355819083594074, 0.000000000000000000, -0.2635871660690647933 ) ) ;
#14560=VERTEX_POINT ( 'NONE', #43978 ) ;
#14561=ORIENTED_EDGE ( 'NONE', *, *, #18087, .T. ) ;
#14562=LINE ( 'NONE', #46890, #45089 ) ;
#14563=VECTOR ( 'NONE', #37910, 1000.000000000000114 ) ;
#14567=ORIENTED_EDGE ( 'NONE', *, *, #20200, .T. ) ;
#14568=CARTESIAN_POINT ( 'NONE',  ( 71.15591247552653442, -183.6283474603465606, 36.22785377504035154 ) ) ;
#14571=CARTESIAN_POINT ( 'NONE',  ( -140.5933766095837427, -189.7472609257535510, -84.49831343337066869 ) ) ;
#14573=AXIS2_PLACEMENT_3D ( 'NONE', #5714, #21729, #2001 ) ;
#14574=DIRECTION ( 'NONE',  ( -0.000000000000000000, 1.000000000000000000, -0.000000000000000000 ) ) ;
#14576=EDGE_LOOP ( 'NONE', ( #43871, #44823, #14315, #13945 ) ) ;
#14578=VERTEX_POINT ( 'NONE', #35567 ) ;
#14580=LINE ( 'NONE', #2489, #38621 ) ;
#14582=DIRECTION ( 'NONE',  ( 0.1476465640024851034, 0.000000000000000000, -0.9890401873221634776 ) ) ;
#14583=DIRECTION ( 'NONE',  ( 0.000000000000000000, 1.000000000000000000, 0.000000000000000000 ) ) ;
#14585=EDGE_CURVE ( 'NONE', #29842, #3318, #7974, .T. ) ;
#14588=VECTOR ( 'NONE', #15189, 1000.000000000000114 ) ;
#14590=VERTEX_POINT ( 'NONE', #43722 ) ;
#14594=DIRECTION ( 'NONE',  ( 0.1182731709213660498, 0.000000000000000000, -0.9929810960135169173 ) ) ;
#14597=DIRECTION ( 'NONE',  ( -0.000000000000000000, 1.000000000000000000, 0.000000000000000000 ) ) ;
#14598=AXIS2_PLACEMENT_3D ( 'NONE', #46066, #29742, #50514 ) ;
#14600=CARTESIAN_POINT ( 'NONE',  ( 30.05499637021956971, -183.6283474603465606, -97.24912084693207248 ) ) ;
#14602=ORIENTED_EDGE ( 'NONE', *, *, #30115, .F. ) ;
#14603=CARTESIAN_POINT ( 'NONE',  ( -94.78385179329475818, -183.6283474603465606, 115.0304316645283080 ) ) ;
#14607=LINE ( 'NONE', #38761, #5989 ) ;
#14608=ORIENTED_EDGE ( 'NONE', *, *, #20518, .F. ) ;
#14610=EDGE_LOOP ( 'NONE', ( #41634, #45156, #8301, #23020 ) ) ;
#14612=EDGE_CURVE ( 'NONE', #7467, #37183, #8019, .T. ) ;
#14613=AXIS2_PLACEMENT_3D ( 'NONE', #31511, #12318, #8386 ) ;
#14614=EDGE_CURVE ( 'NONE', #14148, #43465, #19799, .T. ) ;
#14615=EDGE_LOOP ( 'NONE', ( #24632, #12311, #42686, #44929 ) ) ;
#14616=DIRECTION ( 'NONE',  ( -0.9646355819083556327, 0.000000000000000000, -0.2635871660690782825 ) ) ;
#14618=CIRCLE ( 'NONE', #43980, 125.0000000000000000 ) ;
#14621=ORIENTED_EDGE ( 'NONE', *, *, #28865, .F. ) ;
#14622=FACE_OUTER_BOUND ( 'NONE', #16055, .T. ) ;
#14623=CARTESIAN_POINT ( 'NONE',  ( -150.1390659022305840, -193.5000000000000000, 72.73415134496005408 ) ) ;
#14624=ORIENTED_EDGE ( 'NONE', *, *, #19784, .T. ) ;
#14625=CARTESIAN_POINT ( 'NONE',  ( -171.2727421180348415, -183.6283474603465606, 23.38221600314377113 ) ) ;
#14626=EDGE_CURVE ( 'NONE', #24680, #40690, #31892, .T. ) ;
#14627=CARTESIAN_POINT ( 'NONE',  ( -59.16959496120701090, -193.5000000000000000, 123.5388265266452237 ) ) ;
#14629=CARTESIAN_POINT ( 'NONE',  ( -48.47912675150885065, -189.7472609257535510, -0.9999999999999931166 ) ) ;
#14630=VERTEX_POINT ( 'NONE', #24007 ) ;
#14631=VERTEX_POINT ( 'NONE', #45302 ) ;
#14632=ADVANCED_FACE ( 'NONE', ( #21364 ), #44503, .T. ) ;
#14633=EDGE_CURVE ( 'NONE', #39640, #49743, #28971, .T. ) ;
#14635=LINE ( 'NONE', #12185, #41016 ) ;
#14636=CARTESIAN_POINT ( 'NONE',  ( 75.17589904515342880, -193.5000000000000000, -18.28755301364250130 ) ) ;
#14641=ORIENTED_EDGE ( 'NONE', *, *, #31100, .F. ) ;
#14642=DIRECTION ( 'NONE',  ( -0.000000000000000000, 1.000000000000000000, 0.000000000000000000 ) ) ;
#14643=ORIENTED_EDGE ( 'NONE', *, *, #32441, .F. ) ;
#14644=CYLINDRICAL_SURFACE ( 'NONE', #47445, 10.00000000000000000 ) ;
#14646=EDGE_LOOP ( 'NONE', ( #7806, #7044, #46949, #21977 ) ) ;
#14648=EDGE_LOOP ( 'NONE', ( #47360, #41721, #35106, #34538 ) ) ;
#14649=CARTESIAN_POINT ( 'NONE',  ( -48.93575598890255662, -189.7472609257535510, -0.8896570909947461026 ) ) ;
#14650=VECTOR ( 'NONE', #42816, 1000.000000000000000 ) ;
#14651=DIRECTION ( 'NONE',  ( 0.000000000000000000, 1.000000000000000000, -0.000000000000000000 ) ) ;
#14652=CARTESIAN_POINT ( 'NONE',  ( -48.47912675150885065, -173.5000000000000284, 125.0000000000000000 ) ) ;
#14653=ORIENTED_EDGE ( 'NONE', *, *, #807, .T. ) ;
#14654=DIRECTION ( 'NONE',  ( 0.000000000000000000, -1.000000000000000000, 0.000000000000000000 ) ) ;
#14655=ORIENTED_EDGE ( 'NONE', *, *, #35582, .T. ) ;
#14656=AXIS2_PLACEMENT_3D ( 'NONE', #6667, #18234, #42129 ) ;
#14657=ORIENTED_EDGE ( 'NONE', *, *, #19979, .T. ) ;
#14658=CARTESIAN_POINT ( 'NONE',  ( -130.7087404384255080, -175.3837268820161057, -94.14505102712755047 ) ) ;
#14659=LINE ( 'NONE', #26738, #26409 ) ;
#14660=FACE_OUTER_BOUND ( 'NONE', #31373, .T. ) ;
#14661=LINE ( 'NONE', #20085, #49258 ) ;
#14662=VERTEX_POINT ( 'NONE', #49751 ) ;
#14664=CARTESIAN_POINT ( 'NONE',  ( -161.2555905272864152, -189.7472609257535510, -53.91167979418494838 ) ) ;
#14665=LINE ( 'NONE', #7041, #36398 ) ;
#14667=VERTEX_POINT ( 'NONE', #33187 ) ;
#14668=AXIS2_PLACEMENT_3D ( 'NONE', #51609, #7968, #7720 ) ;
#14669=DIRECTION ( 'NONE',  ( -0.000000000000000000, 1.000000000000000000, -0.000000000000000000 ) ) ;
#14671=DIRECTION ( 'NONE',  ( 0.000000000000000000, -1.000000000000000000, 0.000000000000000000 ) ) ;
#14672=ORIENTED_EDGE ( 'NONE', *, *, #46778, .F. ) ;
#14673=EDGE_CURVE ( 'NONE', #38136, #35121, #37388, .T. ) ;
#14675=EDGE_CURVE ( 'NONE', #28774, #17068, #1661, .T. ) ;
#14677=EDGE_CURVE ( 'NONE', #48253, #43006, #21102, .T. ) ;
#14679=ORIENTED_EDGE ( 'NONE', *, *, #6762, .F. ) ;
#14680=CARTESIAN_POINT ( 'NONE',  ( -47.53180039765465636, -193.5000000000000000, -0.3202698538628280800 ) ) ;
#14681=AXIS2_PLACEMENT_3D ( 'NONE', #15182, #35141, #10968 ) ;
#14683=CARTESIAN_POINT ( 'NONE',  ( 40.30419662299490113, -177.1207230881787780, -87.99159897727903967 ) ) ;
#14684=EDGE_CURVE ( 'NONE', #9853, #5202, #42422, .T. ) ;
#14685=CIRCLE ( 'NONE', #11326, 125.0000000000000000 ) ;
#14686=CARTESIAN_POINT ( 'NONE',  ( 75.60865171534661044, -183.6283474603465606, -15.07392567185467236 ) ) ;
#14687=EDGE_CURVE ( 'NONE', #10667, #21060, #17447, .T. ) ;
#14690=AXIS2_PLACEMENT_3D ( 'NONE', #15198, #35666, #19642 ) ;
#14691=ADVANCED_FACE ( 'NONE', ( #20583 ), #49233, .T. ) ;
#14693=ORIENTED_EDGE ( 'NONE', *, *, #32654, .T. ) ;
#14696=ORIENTED_EDGE ( 'NONE', *, *, #30751, .F. ) ;
#14699=AXIS2_PLACEMENT_3D ( 'NONE', #38202, #13782, #37700 ) ;
#14700=EDGE_CURVE ( 'NONE', #6669, #27166, #45550, .T. ) ;
#14701=CIRCLE ( 'NONE', #1264, 125.0000000000000000 ) ;
#14702=CIRCLE ( 'NONE', #41551, 125.0000000000000000 ) ;
#14703=DIRECTION ( 'NONE',  ( -0.6965510290630033685, 0.000000000000000000, 0.7175072570443249420 ) ) ;
#14705=CARTESIAN_POINT ( 'NONE',  ( -48.47912675150885065, -175.3837268820161057, 6.938893903907228378E-15 ) ) ;
#14707=DIRECTION ( 'NONE',  ( -0.3482016354343866471, 0.000000000000000000, -0.9374196611341253371 ) ) ;
#14710=DIRECTION ( 'NONE',  ( -0.000000000000000000, 1.000000000000000000, 0.000000000000000000 ) ) ;
#14712=CARTESIAN_POINT ( 'NONE',  ( -172.1341525481709880, -175.3837268820161057, 18.28755301364337527 ) ) ;
#14713=VERTEX_POINT ( 'NONE', #41072 ) ;
#14715=DIRECTION ( 'NONE',  ( 0.4300652022765245608, 0.000000000000000000, -0.9027978299657416494 ) ) ;
#14718=ADVANCED_FACE ( 'NONE', ( #13483 ), #13742, .T. ) ;
#14719=ORIENTED_EDGE ( 'NONE', *, *, #22775, .F. ) ;
#14722=DIRECTION ( 'NONE',  ( -0.9473263538541876194, 0.000000000000000000, -0.3202698538628486746 ) ) ;
#14723=AXIS2_PLACEMENT_3D ( 'NONE', #46039, #50487, #19196 ) ;
#14724=CARTESIAN_POINT ( 'NONE',  ( 46.01898237923984425, -183.6283474603465606, -81.82363577055903647 ) ) ;
#14725=VERTEX_POINT ( 'NONE', #33467 ) ;
#14726=CARTESIAN_POINT ( 'NONE',  ( -48.47912675150885065, -188.5000000000000284, -14.99999999999999289 ) ) ;
#14730=VECTOR ( 'NONE', #1124, 1000.000000000000000 ) ;
#14732=CIRCLE ( 'NONE', #39907, 125.0000000000000000 ) ;
#14734=DIRECTION ( 'NONE',  ( 0.8757349421956412971, 0.000000000000000000, -0.4827922027307366970 ) ) ;
#14735=LINE ( 'NONE', #26551, #34844 ) ;
#14736=AXIS2_PLACEMENT_3D ( 'NONE', #41421, #25408, #17537 ) ;
#14737=EDGE_CURVE ( 'NONE', #33172, #45478, #615, .T. ) ;
#14738=CARTESIAN_POINT ( 'NONE',  ( -14.28570516517293676, -183.6283474603465606, 120.2323164553486663 ) ) ;
#14739=ORIENTED_EDGE ( 'NONE', *, *, #32211, .T. ) ;
#14741=DIRECTION ( 'NONE',  ( -0.000000000000000000, 1.000000000000000000, -0.000000000000000000 ) ) ;
#14742=AXIS2_PLACEMENT_3D ( 'NONE', #21758, #25436, #29889 ) ;
#14743=ADVANCED_FACE ( 'NONE', ( #37124 ), #25558, .T. ) ;
#14744=CARTESIAN_POINT ( 'NONE',  ( 33.09766481721658238, -189.7472609257535510, 93.38753978496653474 ) ) ;
#14746=CARTESIAN_POINT ( 'NONE',  ( -120.2975302769383177, -183.6283474603465606, 102.3089288139533863 ) ) ;
#14747=EDGE_CURVE ( 'NONE', #29477, #12246, #869, .T. ) ;
#14748=EDGE_CURVE ( 'NONE', #41150, #6819, #6887, .T. ) ;
#14750=VECTOR ( 'NONE', #3642, 1000.000000000000000 ) ;
#14752=AXIS2_PLACEMENT_3D ( 'NONE', #7477, #32149, #36350 ) ;
#14754=EDGE_CURVE ( 'NONE', #20769, #36975, #6128, .T. ) ;
#14755=CARTESIAN_POINT ( 'NONE',  ( -48.47912675150885065, -175.3837268820161057, 6.938893903907228378E-15 ) ) ;
#14756=DIRECTION ( 'NONE',  ( 0.000000000000000000, -1.000000000000000000, -0.000000000000000000 ) ) ;
#14757=DIRECTION ( 'NONE',  ( 0.6068001458185945385, 0.000000000000000000, -0.7948544414133523750 ) ) ;
#14759=EDGE_CURVE ( 'NONE', #38746, #51182, #9801, .T. ) ;
#14760=CARTESIAN_POINT ( 'NONE',  ( -138.3705904895685705, -177.1207230881787780, -86.85922373029296750 ) ) ;
#14762=CARTESIAN_POINT ( 'NONE',  ( -91.84482189527190599, -189.7472609257535510, -117.2365833888816553 ) ) ;
#14765=VECTOR ( 'NONE', #12588, 1000.000000000000000 ) ;
#14766=EDGE_CURVE ( 'NONE', #45352, #22881, #25828, .T. ) ;
#14768=LINE ( 'NONE', #15275, #40975 ) ;
#14769=AXIS2_PLACEMENT_3D ( 'NONE', #30805, #47359, #30287 ) ;
#14771=EDGE_CURVE ( 'NONE', #23058, #32062, #40565, .T. ) ;
#14772=CARTESIAN_POINT ( 'NONE',  ( 69.14211578623219623, -193.5000000000000000, 42.31126686685117733 ) ) ;
#14773=LINE ( 'NONE', #28052, #27179 ) ;
#14774=VERTEX_POINT ( 'NONE', #21892 ) ;
#14775=EDGE_CURVE ( 'NONE', #11672, #9277, #1907, .T. ) ;
#14777=DIRECTION ( 'NONE',  ( 0.000000000000000000, 0.000000000000000000, -1.000000000000000000 ) ) ;
#14778=DIRECTION ( 'NONE',  ( 0.000000000000000000, 0.000000000000000000, 1.000000000000000000 ) ) ;
#14779=FACE_OUTER_BOUND ( 'NONE', #11744, .T. ) ;
#14780=VERTEX_POINT ( 'NONE', #17950 ) ;
#14781=AXIS2_PLACEMENT_3D ( 'NONE', #26932, #2512, #42448 ) ;
#14782=FACE_OUTER_BOUND ( 'NONE', #9944, .T. ) ;
#14783=ORIENTED_EDGE ( 'NONE', *, *, #50050, .F. ) ;
#14785=VERTEX_POINT ( 'NONE', #22917 ) ;
#14786=CARTESIAN_POINT ( 'NONE',  ( -32.87124591993210743, -175.3837268820161057, 124.0217483183788119 ) ) ;
#14787=VECTOR ( 'NONE', #7910, 1000.000000000000000 ) ;
#14789=EDGE_CURVE ( 'NONE', #3419, #45115, #18719, .T. ) ;
#14791=ADVANCED_FACE ( 'NONE', ( #29757 ), #51058, .T. ) ;
#14792=VECTOR ( 'NONE', #47436, 1000.000000000000000 ) ;
#14794=DIRECTION ( 'NONE',  ( -0.000000000000000000, 1.000000000000000000, -0.000000000000000000 ) ) ;
#14796=ORIENTED_EDGE ( 'NONE', *, *, #2542, .T. ) ;
#14797=DIRECTION ( 'NONE',  ( 0.000000000000000000, 0.000000000000000000, 1.000000000000000000 ) ) ;
#14798=DIRECTION ( 'NONE',  ( 0.9374196611341183427, 0.000000000000000000, 0.3482016354344059095 ) ) ;
#14800=DIRECTION ( 'NONE',  ( -0.000000000000000000, 1.000000000000000000, -0.000000000000000000 ) ) ;
#14802=ORIENTED_EDGE ( 'NONE', *, *, #31656, .T. ) ;
#14804=ORIENTED_EDGE ( 'NONE', *, *, #47522, .F. ) ;
#14805=CIRCLE ( 'NONE', #50888, 125.0000000000000000 ) ;
#14806=AXIS2_PLACEMENT_3D ( 'NONE', #8572, #4378, #40890 ) ;
#14807=LINE ( 'NONE', #11097, #46621 ) ;
#14809=ORIENTED_EDGE ( 'NONE', *, *, #30380, .F. ) ;
#14810=CIRCLE ( 'NONE', #15627, 125.0000000000000000 ) ;
#14811=AXIS2_PLACEMENT_3D ( 'NONE', #15512, #12594, #47837 ) ;
#14813=CARTESIAN_POINT ( 'NONE',  ( -47.64924157374594671, -189.7472609257535510, 124.9972451320097377 ) ) ;
#14818=DIRECTION ( 'NONE',  ( 0.9151456172430210145, 0.000000000000000000, -0.4031234292879665171 ) ) ;
#14823=DIRECTION ( 'NONE',  ( 0.000000000000000000, 0.000000000000000000, 1.000000000000000000 ) ) ;
#14825=ORIENTED_EDGE ( 'NONE', *, *, #48392, .T. ) ;
#14827=CIRCLE ( 'NONE', #24903, 125.0000000000000000 ) ;
#14829=DIRECTION ( 'NONE',  ( 0.000000000000000000, -1.000000000000000000, -0.000000000000000000 ) ) ;
#14830=CIRCLE ( 'NONE', #2207, 125.0000000000000000 ) ;
#14835=EDGE_CURVE ( 'NONE', #39207, #7752, #42106, .T. ) ;
#14837=FACE_OUTER_BOUND ( 'NONE', #28437, .T. ) ;
#14838=DIRECTION ( 'NONE',  ( 0.2635871660690581320, 0.000000000000000000, 0.9646355819083614058 ) ) ;
#14839=FACE_OUTER_BOUND ( 'NONE', #38059, .T. ) ;
#14842=ORIENTED_EDGE ( 'NONE', *, *, #36257, .F. ) ;
#14843=ADVANCED_FACE ( 'NONE', ( #2938 ), #50276, .T. ) ;
#14844=ORIENTED_EDGE ( 'NONE', *, *, #27114, .F. ) ;
#14845=DIRECTION ( 'NONE',  ( 0.000000000000000000, -1.000000000000000000, 0.000000000000000000 ) ) ;
#14849=CIRCLE ( 'NONE', #33286, 125.0000000000000000 ) ;
#14850=CARTESIAN_POINT ( 'NONE',  ( -48.47912675150885065, -183.6283474603465606, 6.938893903907228378E-15 ) ) ;
#14851=DIRECTION ( 'NONE',  ( 0.7175072570443348230, 0.000000000000000000, -0.6965510290629933765 ) ) ;
#14853=VECTOR ( 'NONE', #13693, 1000.000000000000000 ) ;
#14855=DIRECTION ( 'NONE',  ( 0.000000000000000000, 1.000000000000000000, -0.000000000000000000 ) ) ;
#14856=DIRECTION ( 'NONE',  ( -0.9785564922995060311, 0.000000000000000000, 0.2059786187410889424 ) ) ;
#14858=ORIENTED_EDGE ( 'NONE', *, *, #34657, .T. ) ;
#14859=AXIS2_PLACEMENT_3D ( 'NONE', #22417, #1670, #14536 ) ;
#14860=CARTESIAN_POINT ( 'NONE',  ( 9.518239912201979180, -193.5000000000000000, 110.7307791902283043 ) ) ;
#14861=CARTESIAN_POINT ( 'NONE',  ( -48.47912675150885065, -177.1207230881787780, 6.938893903907228378E-15 ) ) ;
#14862=CARTESIAN_POINT ( 'NONE',  ( -111.6834028793037987, -189.7472609257535510, 106.6827995071088395 ) ) ;
#14865=CIRCLE ( 'NONE', #24081, 125.0000000000000000 ) ;
#14867=CARTESIAN_POINT ( 'NONE',  ( -123.0610352593084116, -193.5000000000000000, 99.06333546307732263 ) ) ;
#14868=CARTESIAN_POINT ( 'NONE',  ( -81.70897914701313880, -193.5000000000000000, -120.5021863277716534 ) ) ;
#14869=ORIENTED_EDGE ( 'NONE', *, *, #19596, .F. ) ;
#14870=CARTESIAN_POINT ( 'NONE',  ( -101.9736325116273434, -177.1207230881787780, 112.9749434763330669 ) ) ;
#14871=AXIS2_PLACEMENT_3D ( 'NONE', #27211, #35620, #43247 ) ;
#14874=DIRECTION ( 'NONE',  ( 0.000000000000000000, 1.000000000000000000, 0.000000000000000000 ) ) ;
#14875=DIRECTION ( 'NONE',  ( -0.000000000000000000, 1.000000000000000000, -0.000000000000000000 ) ) ;
#14876=VERTEX_POINT ( 'NONE', #14266 ) ;
#14877=FACE_OUTER_BOUND ( 'NONE', #15426, .T. ) ;
#14878=DIRECTION ( 'NONE',  ( 0.000000000000000000, 0.000000000000000000, 1.000000000000000000 ) ) ;
#14879=DIRECTION ( 'NONE',  ( 0.000000000000000000, 0.000000000000000000, 1.000000000000000000 ) ) ;
#14880=EDGE_CURVE ( 'NONE', #4103, #7207, #10315, .T. ) ;
#14881=DIRECTION ( 'NONE',  ( 0.000000000000000000, 0.000000000000000000, 1.000000000000000000 ) ) ;
#14882=CYLINDRICAL_SURFACE ( 'NONE', #11857, 125.0000000000000000 ) ;
#14884=AXIS2_PLACEMENT_3D ( 'NONE', #8817, #15694, #16462 ) ;
#14885=VECTOR ( 'NONE', #35794, 1000.000000000000114 ) ;
#14886=CARTESIAN_POINT ( 'NONE',  ( -14.28570516517293676, -183.6283474603465606, 120.2323164553486663 ) ) ;
#14887=FACE_OUTER_BOUND ( 'NONE', #31505, .T. ) ;
#14888=ORIENTED_EDGE ( 'NONE', *, *, #50706, .T. ) ;
#14889=VECTOR ( 'NONE', #35124, 1000.000000000000000 ) ;
#14890=ORIENTED_EDGE ( 'NONE', *, *, #36455, .F. ) ;
#14891=DIRECTION ( 'NONE',  ( 0.000000000000000000, -0.000000000000000000, -1.000000000000000000 ) ) ;
#14892=ORIENTED_EDGE ( 'NONE', *, *, #36509, .T. ) ;
#14893=AXIS2_PLACEMENT_3D ( 'NONE', #50068, #38215, #42156 ) ;
#14895=LINE ( 'NONE', #51411, #39361 ) ;
#14896=VECTOR ( 'NONE', #38923, 1000.000000000000227 ) ;
#14899=ORIENTED_EDGE ( 'NONE', *, *, #33687, .F. ) ;
#14900=LINE ( 'NONE', #27731, #49292 ) ;
#14901=CIRCLE ( 'NONE', #20774, 125.0000000000000000 ) ;
#14902=LINE ( 'NONE', #11710, #9322 ) ;
#14903=DIRECTION ( 'NONE',  ( -0.4566292373937077542, 0.000000000000000000, -0.8896570909947499883 ) ) ;
#14906=EDGE_LOOP ( 'NONE', ( #38296, #21244, #47965, #29362 ) ) ;
#14907=CIRCLE ( 'NONE', #24130, 125.0000000000000000 ) ;
#14908=DIRECTION ( 'NONE',  ( -0.9785564922995060311, 0.000000000000000000, 0.2059786187410889424 ) ) ;
#14910=EDGE_CURVE ( 'NONE', #20906, #23116, #8697, .T. ) ;
#14911=FACE_OUTER_BOUND ( 'NONE', #41488, .T. ) ;
#14912=DIRECTION ( 'NONE',  ( 0.000000000000000000, 0.000000000000000000, -1.000000000000000000 ) ) ;
#14913=EDGE_LOOP ( 'NONE', ( #13233, #17200, #42750, #17758 ) ) ;
#14915=FACE_OUTER_BOUND ( 'NONE', #33317, .T. ) ;
#14916=VERTEX_POINT ( 'NONE', #32084 ) ;
#14917=DIRECTION ( 'NONE',  ( 0.000000000000000000, 0.000000000000000000, -1.000000000000000000 ) ) ;
#14918=ORIENTED_EDGE ( 'NONE', *, *, #3052, .F. ) ;
#14921=CIRCLE ( 'NONE', #44282, 125.0000000000000000 ) ;
#14922=DIRECTION ( 'NONE',  ( 0.000000000000000000, 0.000000000000000000, -1.000000000000000000 ) ) ;
#14923=CARTESIAN_POINT ( 'NONE',  ( -49.21696003055057389, -189.7472609257535510, -0.6749830015182127774 ) ) ;
#14924=AXIS2_PLACEMENT_3D ( 'NONE', #29548, #45347, #49550 ) ;
#14926=PLANE ( 'NONE',  #30940 ) ;
#14927=ORIENTED_EDGE ( 'NONE', *, *, #24844, .T. ) ;
#14929=ORIENTED_EDGE ( 'NONE', *, *, #32846, .F. ) ;
#14930=EDGE_CURVE ( 'NONE', #51182, #40259, #3210, .T. ) ;
#14931=VERTEX_POINT ( 'NONE', #27874 ) ;
#14932=DIRECTION ( 'NONE',  ( -0.000000000000000000, 1.000000000000000000, -0.000000000000000000 ) ) ;
#14934=LINE ( 'NONE', #3344, #48257 ) ;
#14935=LINE ( 'NONE', #46989, #42324 ) ;
#14936=DIRECTION ( 'NONE',  ( 0.05924062789370748011, 0.000000000000000000, 0.9982437317643217956 ) ) ;
#14937=ORIENTED_EDGE ( 'NONE', *, *, #37810, .F. ) ;
#14938=AXIS2_PLACEMENT_3D ( 'NONE', #37920, #26346, #41336 ) ;
#14940=DIRECTION ( 'NONE',  ( -0.000000000000000000, 1.000000000000000000, -0.000000000000000000 ) ) ;
#14941=LINE ( 'NONE', #30948, #27997 ) ;
#14942=CARTESIAN_POINT ( 'NONE',  ( 66.42899531795131907, -183.6283474603465606, 49.20491319441622124 ) ) ;
#14944=EDGE_LOOP ( 'NONE', ( #12065, #39313, #4981, #9305 ) ) ;
#14945=LINE ( 'NONE', #30951, #18774 ) ;
#14946=FACE_OUTER_BOUND ( 'NONE', #50626, .T. ) ;
#14947=ADVANCED_FACE ( 'NONE', ( #31307 ), #43413, .F. ) ;
#14951=EDGE_CURVE ( 'NONE', #51603, #35121, #32, .T. ) ;
#14953=FACE_OUTER_BOUND ( 'NONE', #33183, .T. ) ;
#14954=VERTEX_POINT ( 'NONE', #35251 ) ;
#14955=CARTESIAN_POINT ( 'NONE',  ( 12.99855592850622799, -177.1207230881787780, 108.8370090194295017 ) ) ;
#14956=VERTEX_POINT ( 'NONE', #16073 ) ;
#14957=CYLINDRICAL_SURFACE ( 'NONE', #17583, 125.0000000000000000 ) ;
#14959=FACE_BOUND ( 'NONE', #42946, .T. ) ;
#14960=CARTESIAN_POINT ( 'NONE',  ( -112.7586829773731267, -193.5000000000000000, -107.2060569716373379 ) ) ;
#14962=EDGE_CURVE ( 'NONE', #18957, #5084, #40223, .T. ) ;
#14963=CIRCLE ( 'NONE', #8225, 124.9999999999999858 ) ;
#14965=VERTEX_POINT ( 'NONE', #19734 ) ;
#14967=CARTESIAN_POINT ( 'NONE',  ( 18.49541618049843095, -193.5000000000000000, 105.5434062319798159 ) ) ;
#14968=AXIS2_PLACEMENT_3D ( 'NONE', #15866, #17101, #23984 ) ;
#14970=LINE ( 'NONE', #38079, #3282 ) ;
#14971=VECTOR ( 'NONE', #20989, 1000.000000000000114 ) ;
#14973=LINE ( 'NONE', #7836, #7977 ) ;
#14974=ORIENTED_EDGE ( 'NONE', *, *, #10007, .T. ) ;
#14978=DIRECTION ( 'NONE',  ( -0.000000000000000000, 1.000000000000000000, -0.000000000000000000 ) ) ;
#14980=DIRECTION ( 'NONE',  ( -0.2348860457809911206, 0.000000000000000000, 0.9720229140804089729 ) ) ;
#14981=ORIENTED_EDGE ( 'NONE', *, *, #50403, .T. ) ;
#14986=DIRECTION ( 'NONE',  ( -0.9027978299657416494, 0.000000000000000000, -0.4300652022765245608 ) ) ;
#14989=ORIENTED_EDGE ( 'NONE', *, *, #43929, .F. ) ;
#14990=DIRECTION ( 'NONE',  ( 0.000000000000000000, 0.000000000000000000, 1.000000000000000000 ) ) ;
#14991=EDGE_LOOP ( 'NONE', ( #565, #14460, #50902, #13323 ) ) ;
#14992=DIRECTION ( 'NONE',  ( 0.000000000000000000, 0.000000000000000000, -1.000000000000000000 ) ) ;
#14993=VECTOR ( 'NONE', #50288, 1000.000000000000227 ) ;
#14994=DIRECTION ( 'NONE',  ( 0.000000000000000000, 0.000000000000000000, 1.000000000000000000 ) ) ;
#14995=VERTEX_POINT ( 'NONE', #47875 ) ;
#14997=CARTESIAN_POINT ( 'NONE',  ( 4.558749771216698221, -193.5000000000000000, -112.0852863853379233 ) ) ;
#14999=CARTESIAN_POINT ( 'NONE',  ( -34.51936650669028239, -189.7472609257535510, -124.2180546213278092 ) ) ;
#15001=FACE_OUTER_BOUND ( 'NONE', #33878, .T. ) ;
#15002=ORIENTED_EDGE ( 'NONE', *, *, #21951, .F. ) ;
#15007=DIRECTION ( 'NONE',  ( 0.000000000000000000, 0.000000000000000000, -1.000000000000000000 ) ) ;
#15009=VECTOR ( 'NONE', #2547, 1000.000000000000000 ) ;
#15011=DIRECTION ( 'NONE',  ( 0.3482016354343995812, 0.000000000000000000, -0.9374196611341205632 ) ) ;
#15012=DIRECTION ( 'NONE',  ( 0.000000000000000000, -1.000000000000000000, 0.000000000000000000 ) ) ;
#15013=DIRECTION ( 'NONE',  ( 0.000000000000000000, -0.000000000000000000, 1.000000000000000000 ) ) ;
#15015=CARTESIAN_POINT ( 'NONE',  ( -95.37971604807249548, -193.5000000000000000, -114.7887733785763942 ) ) ;
#15016=CARTESIAN_POINT ( 'NONE',  ( -49.45768324380835423, -189.7472609257535510, -0.2059786187411025149 ) ) ;
#15017=ORIENTED_EDGE ( 'NONE', *, *, #4969, .F. ) ;
#15018=AXIS2_PLACEMENT_3D ( 'NONE', #49625, #13879, #41734 ) ;
#15021=CARTESIAN_POINT ( 'NONE',  ( -70.24606818074167336, -189.7472609257535510, -122.0745693923549169 ) ) ;
#15022=PLANE ( 'NONE',  #14493 ) ;
#15023=ORIENTED_EDGE ( 'NONE', *, *, #35582, .F. ) ;
#15024=CARTESIAN_POINT ( 'NONE',  ( -147.0463339291295881, -183.6283474603465606, 76.87330921200150158 ) ) ;
#15025=CARTESIAN_POINT ( 'NONE',  ( 75.27070168362158142, -189.7472609257535510, 17.63462396184792169 ) ) ;
#15027=CIRCLE ( 'NONE', #35154, 125.0000000000000000 ) ;
#15028=ORIENTED_EDGE ( 'NONE', *, *, #42462, .F. ) ;
#15029=CIRCLE ( 'NONE', #39352, 125.0000000000000000 ) ;
#15030=ORIENTED_EDGE ( 'NONE', *, *, #41015, .F. ) ;
#15032=VECTOR ( 'NONE', #51227, 1000.000000000000000 ) ;
#15033=CYLINDRICAL_SURFACE ( 'NONE', #938, 125.0000000000000000 ) ;
#15034=ORIENTED_EDGE ( 'NONE', *, *, #15874, .F. ) ;
#15036=CARTESIAN_POINT ( 'NONE',  ( 69.72248760683812918, -193.5000000000000000, -37.47770156625421833 ) ) ;
#15037=DIRECTION ( 'NONE',  ( 0.000000000000000000, 0.000000000000000000, 1.000000000000000000 ) ) ;
#15038=VECTOR ( 'NONE', #43514, 1000.000000000000000 ) ;
#15039=CARTESIAN_POINT ( 'NONE',  ( 22.03849146056077757, -193.5000000000000000, 103.2098131075567409 ) ) ;
#15042=DIRECTION ( 'NONE',  ( 0.3202698538628279690, 0.000000000000000000, 0.9473263538541946138 ) ) ;
#15043=EDGE_LOOP ( 'NONE', ( #44176, #1504, #46345, #41766 ) ) ;
#15044=LINE ( 'NONE', #47350, #32258 ) ;
#15047=ADVANCED_FACE ( 'NONE', ( #1465 ), #41649, .T. ) ;
#15048=EDGE_CURVE ( 'NONE', #8272, #3435, #48532, .T. ) ;
#15053=ORIENTED_EDGE ( 'NONE', *, *, #28852, .T. ) ;
#15054=ADVANCED_FACE ( 'NONE', ( #4620 ), #45364, .T. ) ;
#15056=ORIENTED_EDGE ( 'NONE', *, *, #51545, .F. ) ;
#15057=DIRECTION ( 'NONE',  ( -0.000000000000000000, 1.000000000000000000, 0.000000000000000000 ) ) ;
#15059=ORIENTED_EDGE ( 'NONE', *, *, #38092, .F. ) ;
#15060=ADVANCED_FACE ( 'NONE', ( #37454 ), #686, .F. ) ;
#15063=VERTEX_POINT ( 'NONE', #13993 ) ;
#15064=CARTESIAN_POINT ( 'NONE',  ( 29.27398957514435196, -177.1207230881787780, -97.87467957287998388 ) ) ;
#15065=EDGE_CURVE ( 'NONE', #38645, #19776, #12018, .T. ) ;
#15066=PLANE ( 'NONE',  #28989 ) ;
#15067=ADVANCED_FACE ( 'NONE', ( #13471 ), #17932, .T. ) ;
#15070=ORIENTED_EDGE ( 'NONE', *, *, #25178, .T. ) ;
#15071=EDGE_CURVE ( 'NONE', #23360, #20728, #49996, .T. ) ;
#15073=DIRECTION ( 'NONE',  ( -0.000000000000000000, 1.000000000000000000, 0.000000000000000000 ) ) ;
#15074=CARTESIAN_POINT ( 'NONE',  ( -48.47912675150885065, -189.7472609257535510, 6.938893903907228378E-15 ) ) ;
#15075=ORIENTED_EDGE ( 'NONE', *, *, #23636, .F. ) ;
#15076=VECTOR ( 'NONE', #34845, 1000.000000000000000 ) ;
#15077=EDGE_CURVE ( 'NONE', #29008, #34513, #30520, .T. ) ;
#15079=CARTESIAN_POINT ( 'NONE',  ( -48.47912675150885065, -177.1207230881787780, 6.938893903907228378E-15 ) ) ;
#15080=CARTESIAN_POINT ( 'NONE',  ( -106.2948367055610106, -175.3837268820161057, -110.8257356506552185 ) ) ;
#15081=ADVANCED_FACE ( 'NONE', ( #34467 ), #37897, .T. ) ;
#15084=CARTESIAN_POINT ( 'NONE',  ( -88.23625491228470707, -183.6283474603465606, 118.5089480183148254 ) ) ;
#15087=VERTEX_POINT ( 'NONE', #6630 ) ;
#15088=ORIENTED_EDGE ( 'NONE', *, *, #19258, .F. ) ;
#15089=DIRECTION ( 'NONE',  ( -0.000000000000000000, 1.000000000000000000, -0.000000000000000000 ) ) ;
#15090=EDGE_CURVE ( 'NONE', #47251, #18925, #13727, .T. ) ;
#15091=AXIS2_PLACEMENT_3D ( 'NONE', #48772, #5670, #25118 ) ;
#15098=CARTESIAN_POINT ( 'NONE',  ( -47.74129347246713451, -175.3837268820161057, 0.6749830015182212151 ) ) ;
#15100=PLANE ( 'NONE',  #2288 ) ;
#15101=ORIENTED_EDGE ( 'NONE', *, *, #50777, .T. ) ;
#15102=VERTEX_POINT ( 'NONE', #26581 ) ;
#15104=DIRECTION ( 'NONE',  ( 0.000000000000000000, -0.000000000000000000, -1.000000000000000000 ) ) ;
#15106=CARTESIAN_POINT ( 'NONE',  ( -139.8555433305420195, -189.7472609257535510, -83.82333043185244037 ) ) ;
#15108=FACE_OUTER_BOUND ( 'NONE', #13326, .T. ) ;
#15109=CARTESIAN_POINT ( 'NONE',  ( -48.64924157374594671, -175.3837268820161057, 124.9998842437354227 ) ) ;
#15110=VERTEX_POINT ( 'NONE', #6364 ) ;
#15111=EDGE_CURVE ( 'NONE', #50966, #48020, #25815, .T. ) ;
#15112=ADVANCED_FACE ( 'NONE', ( #29482 ), #10051, .T. ) ;
#15113=CARTESIAN_POINT ( 'NONE',  ( -172.0602536473422504, -175.3837268820161057, -10.18383939837523222 ) ) ;
#15114=EDGE_CURVE ( 'NONE', #1772, #9394, #17148, .T. ) ;
#15115=EDGE_CURVE ( 'NONE', #29336, #4180, #1895, .T. ) ;
#15116=ORIENTED_EDGE ( 'NONE', *, *, #35151, .F. ) ;
#15117=ORIENTED_EDGE ( 'NONE', *, *, #42906, .F. ) ;
#15118=PLANE ( 'NONE',  #29789 ) ;
#15122=DIRECTION ( 'NONE',  ( -0.5085311186492094127, 0.000000000000000000, -0.8610436117673619938 ) ) ;
#15124=DIRECTION ( 'NONE',  ( -0.5829794791144703447, 0.000000000000000000, -0.8124868780056825335 ) ) ;
#15126=VECTOR ( 'NONE', #28237, 1000.000000000000000 ) ;
#15131=EDGE_LOOP ( 'NONE', ( #2356, #50233, #23599, #1664 ) ) ;
#15132=FACE_OUTER_BOUND ( 'NONE', #439, .T. ) ;
#15133=DIRECTION ( 'NONE',  ( 0.000000000000000000, -1.000000000000000000, 0.000000000000000000 ) ) ;
#15134=DIRECTION ( 'NONE',  ( -0.000000000000000000, 1.000000000000000000, -0.000000000000000000 ) ) ;
#15135=DIRECTION ( 'NONE',  ( -0.000000000000000000, 1.000000000000000000, -0.000000000000000000 ) ) ;
#15136=EDGE_CURVE ( 'NONE', #51892, #40491, #38139, .T. ) ;
#15137=DIRECTION ( 'NONE',  ( 0.9266896074318370369, 0.000000000000000000, -0.3758275821142292306 ) ) ;
#15138=ORIENTED_EDGE ( 'NONE', *, *, #32885, .F. ) ;
#15139=CIRCLE ( 'NONE', #26002, 125.0000000000000000 ) ;
#15140=CARTESIAN_POINT ( 'NONE',  ( -173.3294908491238004, -193.5000000000000000, -6.114457023560960991 ) ) ;
#15141=CARTESIAN_POINT ( 'NONE',  ( -21.64528618042744412, -193.5000000000000000, 121.0625654437174745 ) ) ;
#15142=ORIENTED_EDGE ( 'NONE', *, *, #32240, .F. ) ;
#15146=DIRECTION ( 'NONE',  ( -0.000000000000000000, 1.000000000000000000, -0.000000000000000000 ) ) ;
#15148=LINE ( 'NONE', #23018, #15038 ) ;
#15152=CARTESIAN_POINT ( 'NONE',  ( -72.96029774493611342, -183.6283474603465606, 122.5792489240759409 ) ) ;
#15153=DIRECTION ( 'NONE',  ( -0.1182731709213592358, 0.000000000000000000, -0.9929810960135178055 ) ) ;
#15155=ORIENTED_EDGE ( 'NONE', *, *, #20543, .T. ) ;
#15157=VECTOR ( 'NONE', #833, 1000.000000000000227 ) ;
#15158=ORIENTED_EDGE ( 'NONE', *, *, #38795, .T. ) ;
#15161=CARTESIAN_POINT ( 'NONE',  ( -85.77912150413021664, -189.7472609257535510, -119.3051146910911768 ) ) ;
#15162=CARTESIAN_POINT ( 'NONE',  ( -49.25565061422688728, -193.5000000000000000, -0.6300878435817132139 ) ) ;
#15165=ADVANCED_FACE ( 'NONE', ( #9526 ), #2424, .T. ) ;
#15166=ADVANCED_FACE ( 'NONE', ( #14512 ), #14252, .F. ) ;
#15169=DIRECTION ( 'NONE',  ( 0.7765238627180437447, 0.000000000000000000, -0.6300878435817094392 ) ) ;
#15170=ORIENTED_EDGE ( 'NONE', *, *, #1863, .F. ) ;
#15171=ORIENTED_EDGE ( 'NONE', *, *, #17539, .T. ) ;
#15172=VECTOR ( 'NONE', #44086, 999.9999999999998863 ) ;
#15173=DIRECTION ( 'NONE',  ( 0.000000000000000000, -1.000000000000000000, -0.000000000000000000 ) ) ;
#15174=DIRECTION ( 'NONE',  ( -0.000000000000000000, 1.000000000000000000, 0.000000000000000000 ) ) ;
#15175=CARTESIAN_POINT ( 'NONE',  ( -165.6791976657750354, -189.7472609257535510, 40.49875167739065773 ) ) ;
#15177=ORIENTED_EDGE ( 'NONE', *, *, #38650, .T. ) ;
#15178=CARTESIAN_POINT ( 'NONE',  ( -48.47912675150885065, -175.3837268820161057, 6.938893903907228378E-15 ) ) ;
#15180=ORIENTED_EDGE ( 'NONE', *, *, #20816, .T. ) ;
#15181=LINE ( 'NONE', #8326, #43046 ) ;
#15182=CARTESIAN_POINT ( 'NONE',  ( -48.02249751411514467, -193.5000000000000000, 0.8896570909947569827 ) ) ;
#15183=EDGE_CURVE ( 'NONE', #503, #26317, #46569, .T. ) ;
#15184=PLANE ( 'NONE',  #47968 ) ;
#15185=ORIENTED_EDGE ( 'NONE', *, *, #28792, .T. ) ;
#15187=PLANE ( 'NONE',  #49133 ) ;
#15188=VECTOR ( 'NONE', #21383, 999.9999999999998863 ) ;
#15189=DIRECTION ( 'NONE',  ( 0.2920567706369694982, 0.000000000000000000, 0.9564009842765243130 ) ) ;
#15190=LINE ( 'NONE', #47255, #11132 ) ;
#15191=ORIENTED_EDGE ( 'NONE', *, *, #28931, .T. ) ;
#15192=PLANE ( 'NONE',  #45649 ) ;
#15193=LINE ( 'NONE', #8072, #42507 ) ;
#15194=EDGE_CURVE ( 'NONE', #25116, #10598, #22650, .T. ) ;
#15196=FACE_BOUND ( 'NONE', #50614, .T. ) ;
#15197=ORIENTED_EDGE ( 'NONE', *, *, #17558, .F. ) ;
#15198=CARTESIAN_POINT ( 'NONE',  ( 37.99238433767461487, -189.7472609257535510, -90.26448786734027863 ) ) ;
#15200=ORIENTED_EDGE ( 'NONE', *, *, #8334, .T. ) ;
#15202=EDGE_CURVE ( 'NONE', #22344, #2222, #32002, .T. ) ;
#15205=VECTOR ( 'NONE', #27209, 999.9999999999998863 ) ;
#15206=FACE_BOUND ( 'NONE', #9414, .T. ) ;
#15207=DIRECTION ( 'NONE',  ( -0.000000000000000000, 1.000000000000000000, -0.000000000000000000 ) ) ;
#15208=FACE_OUTER_BOUND ( 'NONE', #17508, .T. ) ;
#15210=EDGE_CURVE ( 'NONE', #44900, #45352, #51538, .T. ) ;
#15211=VERTEX_POINT ( 'NONE', #19659 ) ;
#15212=LINE ( 'NONE', #11250, #14143 ) ;
#15213=ORIENTED_EDGE ( 'NONE', *, *, #39305, .T. ) ;
#15214=DIRECTION ( 'NONE',  ( 0.000000000000000000, 0.000000000000000000, -1.000000000000000000 ) ) ;
#15215=AXIS2_PLACEMENT_3D ( 'NONE', #20280, #1086, #16625 ) ;
#15216=ADVANCED_FACE ( 'NONE', ( #6874 ), #7831, .T. ) ;
#15217=ADVANCED_FACE ( 'NONE', ( #23859 ), #8101, .T. ) ;
#15219=LINE ( 'NONE', #26513, #39320 ) ;
#15220=DIRECTION ( 'NONE',  ( 0.2059786187410889424, 0.000000000000000000, 0.9785564922995060311 ) ) ;
#15221=VERTEX_POINT ( 'NONE', #24144 ) ;
#15222=PLANE ( 'NONE',  #29218 ) ;
#15226=CARTESIAN_POINT ( 'NONE',  ( 74.60098876342243557, -183.6283474603465606, 21.82395850507348811 ) ) ;
#15227=EDGE_LOOP ( 'NONE', ( #12008, #19742, #38613, #24372 ) ) ;
#15229=ORIENTED_EDGE ( 'NONE', *, *, #3817, .T. ) ;
#15230=CARTESIAN_POINT ( 'NONE',  ( -101.5170032742336446, -183.6283474603465606, 112.0852863853383070 ) ) ;
#15233=LINE ( 'NONE', #51244, #4866 ) ;
#15235=CARTESIAN_POINT ( 'NONE',  ( -11.80936624585915418, -175.3837268820161057, -119.5003291395395735 ) ) ;
#15236=VERTEX_POINT ( 'NONE', #28322 ) ;
#15237=DIRECTION ( 'NONE',  ( -0.000000000000000000, 1.000000000000000000, -0.000000000000000000 ) ) ;
#15238=PLANE ( 'NONE',  #3881 ) ;
#15241=EDGE_CURVE ( 'NONE', #46197, #33402, #14773, .T. ) ;
#15242=CARTESIAN_POINT ( 'NONE',  ( 41.00573479224732409, -177.1207230881787780, -87.27805883780175122 ) ) ;
#15244=DIRECTION ( 'NONE',  ( -0.000000000000000000, 1.000000000000000000, 0.000000000000000000 ) ) ;
#15245=DIRECTION ( 'NONE',  ( 0.000000000000000000, -1.000000000000000000, 0.000000000000000000 ) ) ;
#15246=EDGE_LOOP ( 'NONE', ( #13926, #32973, #12224, #16949 ) ) ;
#15248=CARTESIAN_POINT ( 'NONE',  ( 63.10841233855954613, -175.3837268820161057, -54.07611884703302962 ) ) ;
#15249=DIRECTION ( 'NONE',  ( -0.000000000000000000, -1.000000000000000000, 0.000000000000000000 ) ) ;
#15252=CARTESIAN_POINT ( 'NONE',  ( -49.47868758801764955, -177.1207230881787780, 0.02963332782255607284 ) ) ;
#15254=AXIS2_PLACEMENT_3D ( 'NONE', #46942, #26159, #2769 ) ;
#15256=DIRECTION ( 'NONE',  ( -0.4566292373937077542, 0.000000000000000000, -0.8896570909947499883 ) ) ;
#15257=EDGE_LOOP ( 'NONE', ( #18820, #43888, #35865, #28450 ) ) ;
#15258=ORIENTED_EDGE ( 'NONE', *, *, #31344, .T. ) ;
#15262=CARTESIAN_POINT ( 'NONE',  ( 23.54917025746143722, -177.1207230881787780, -100.9358816284410523 ) ) ;
#15264=CARTESIAN_POINT ( 'NONE',  ( 14.94072793302542124, -193.5000000000000000, 107.7168604805791574 ) ) ;
#15265=DIRECTION ( 'NONE',  ( 0.000000000000000000, 0.000000000000000000, 1.000000000000000000 ) ) ;
#15269=VECTOR ( 'NONE', #21398, 1000.000000000000227 ) ;
#15271=AXIS2_PLACEMENT_3D ( 'NONE', #44299, #8290, #11436 ) ;
#15274=ORIENTED_EDGE ( 'NONE', *, *, #21872, .F. ) ;
#15275=CARTESIAN_POINT ( 'NONE',  ( -169.7849785064912567, -193.5000000000000000, -25.70779184431766851 ) ) ;
#15276=EDGE_CURVE ( 'NONE', #30411, #32877, #31758, .T. ) ;
#15278=ORIENTED_EDGE ( 'NONE', *, *, #17856, .T. ) ;
#15279=EDGE_CURVE ( 'NONE', #10734, #3069, #12055, .T. ) ;
#15283=DIRECTION ( 'NONE',  ( -0.000000000000000000, 1.000000000000000000, -0.000000000000000000 ) ) ;
#15286=DIRECTION ( 'NONE',  ( 0.2635871660690715101, 0.000000000000000000, -0.9646355819083576311 ) ) ;
#15287=EDGE_LOOP ( 'NONE', ( #17659, #38002, #12991, #8698 ) ) ;
#15288=DIRECTION ( 'NONE',  ( 0.000000000000000000, 0.000000000000000000, 1.000000000000000000 ) ) ;
#15289=AXIS2_PLACEMENT_3D ( 'NONE', #40568, #49535, #28485 ) ;
#15291=CARTESIAN_POINT ( 'NONE',  ( -48.30901192927175458, -189.7472609257535510, -124.9998842437354227 ) ) ;
#15292=CARTESIAN_POINT ( 'NONE',  ( -111.6834028793037987, -193.5000000000000000, 106.6827995071088253 ) ) ;
#15295=DIRECTION ( 'NONE',  ( 0.000000000000000000, 0.000000000000000000, -1.000000000000000000 ) ) ;
#15296=ORIENTED_EDGE ( 'NONE', *, *, #35032, .F. ) ;
#15297=AXIS2_PLACEMENT_3D ( 'NONE', #45458, #784, #9200 ) ;
#15298=LINE ( 'NONE', #35509, #13917 ) ;
#15300=PLANE ( 'NONE',  #24810 ) ;
#15303=CARTESIAN_POINT ( 'NONE',  ( -48.47912675150885065, -175.3837268820161057, 6.938893903907228378E-15 ) ) ;
#15304=VERTEX_POINT ( 'NONE', #20179 ) ;
#15305=CARTESIAN_POINT ( 'NONE',  ( 75.48400724637754422, -183.6283474603465606, -16.06677968424457248 ) ) ;
#15306=CIRCLE ( 'NONE', #17824, 125.0000000000000000 ) ;
#15307=FACE_OUTER_BOUND ( 'NONE', #16389, .T. ) ;
#15308=AXIS2_PLACEMENT_3D ( 'NONE', #26922, #10904, #39520 ) ;
#15309=ORIENTED_EDGE ( 'NONE', *, *, #45941, .T. ) ;
#15312=VECTOR ( 'NONE', #22810, 1000.000000000000000 ) ;
#15313=VECTOR ( 'NONE', #6947, 1000.000000000000114 ) ;
#15316=FACE_OUTER_BOUND ( 'NONE', #41863, .T. ) ;
#15318=DIRECTION ( 'NONE',  ( -0.000000000000000000, 1.000000000000000000, -0.000000000000000000 ) ) ;
#15319=CARTESIAN_POINT ( 'NONE',  ( 141.7825277784304205, -213.5000000000000000, -9.999999999999987566 ) ) ;
#15320=LINE ( 'NONE', #36061, #48006 ) ;
#15322=LINE ( 'NONE', #3484, #29513 ) ;
#15323=ORIENTED_EDGE ( 'NONE', *, *, #45602, .F. ) ;
#15325=CIRCLE ( 'NONE', #9441, 125.0000000000000000 ) ;
#15327=ORIENTED_EDGE ( 'NONE', *, *, #49497, .F. ) ;
#15328=ADVANCED_FACE ( 'NONE', ( #8364 ), #24388, .T. ) ;
#15329=EDGE_CURVE ( 'NONE', #22157, #14204, #19646, .T. ) ;
#15331=EDGE_CURVE ( 'NONE', #50010, #16064, #459, .T. ) ;
#15335=EDGE_LOOP ( 'NONE', ( #4178, #943, #31882, #32275 ) ) ;
#15337=ADVANCED_FACE ( 'NONE', ( #12560 ), #28578, .T. ) ;
#15339=LINE ( 'NONE', #16114, #25868 ) ;
#15340=DIRECTION ( 'NONE',  ( 0.000000000000000000, 0.000000000000000000, 1.000000000000000000 ) ) ;
#15341=ADVANCED_FACE ( 'NONE', ( #37253 ), #28831, .T. ) ;
#15342=EDGE_CURVE ( 'NONE', #30647, #23694, #24915, .T. ) ;
#15344=DIRECTION ( 'NONE',  ( 0.9266896074318317078, 0.000000000000000000, 0.3758275821142421647 ) ) ;
#15345=VERTEX_POINT ( 'NONE', #49086 ) ;
#15346=CIRCLE ( 'NONE', #44717, 125.0000000000000000 ) ;
#15347=EDGE_LOOP ( 'NONE', ( #12867, #48424, #43407, #1150 ) ) ;
#15349=ORIENTED_EDGE ( 'NONE', *, *, #37644, .T. ) ;
#15350=LINE ( 'NONE', #35557, #34199 ) ;
#15352=CIRCLE ( 'NONE', #27070, 125.0000000000000000 ) ;
#15353=CARTESIAN_POINT ( 'NONE',  ( -48.47912675150885065, -183.6283474603465606, 6.938893903907228378E-15 ) ) ;
#15355=ADVANCED_FACE ( 'NONE', ( #41714 ), #986, .T. ) ;
#15356=FACE_OUTER_BOUND ( 'NONE', #27692, .T. ) ;
#15361=CIRCLE ( 'NONE', #42198, 125.0000000000000000 ) ;
#15362=LINE ( 'NONE', #88, #3822 ) ;
#15364=ORIENTED_EDGE ( 'NONE', *, *, #22554, .T. ) ;
#15365=ORIENTED_EDGE ( 'NONE', *, *, #32107, .T. ) ;
#15366=LINE ( 'NONE', #38738, #39864 ) ;
#15367=DIRECTION ( 'NONE',  ( -0.000000000000000000, -1.000000000000000000, 0.000000000000000000 ) ) ;
#15368=EDGE_LOOP ( 'NONE', ( #736, #10011, #34622, #9362 ) ) ;
#15372=CARTESIAN_POINT ( 'NONE',  ( -48.47912675150885065, -177.1207230881787780, 6.938893903907228378E-15 ) ) ;
#15374=LINE ( 'NONE', #14337, #4068 ) ;
#15375=EDGE_CURVE ( 'NONE', #11314, #43961, #45165, .T. ) ;
#15377=ORIENTED_EDGE ( 'NONE', *, *, #39363, .F. ) ;
#15378=DIRECTION ( 'NONE',  ( -0.000000000000000000, 1.000000000000000000, 0.000000000000000000 ) ) ;
#15379=CARTESIAN_POINT ( 'NONE',  ( -0.3054481938615516423, -183.6283474603465606, 115.3442529744090450 ) ) ;
#15380=EDGE_LOOP ( 'NONE', ( #6356, #17714, #27396, #13694 ) ) ;
#15381=CARTESIAN_POINT ( 'NONE',  ( 116.9235303384055840, -213.5000000000000000, 2.819679052520814125E-14 ) ) ;
#15382=FACE_OUTER_BOUND ( 'NONE', #34463, .T. ) ;
#15383=CARTESIAN_POINT ( 'NONE',  ( -158.0280232639029236, -189.7472609257535510, 60.19999396110247858 ) ) ;
#15384=AXIS2_PLACEMENT_3D ( 'NONE', #4202, #773, #36492 ) ;
#15386=AXIS2_PLACEMENT_3D ( 'NONE', #1755, #5965, #17792 ) ;
#15390=ORIENTED_EDGE ( 'NONE', *, *, #47135, .F. ) ;
#15391=AXIS2_PLACEMENT_3D ( 'NONE', #28159, #32637, #12398 ) ;
#15392=PLANE ( 'NONE',  #10520 ) ;
#15393=CARTESIAN_POINT ( 'NONE',  ( 69.14211578623219623, -183.6283474603465606, 42.31126686685117733 ) ) ;
#15394=ORIENTED_EDGE ( 'NONE', *, *, #11574, .T. ) ;
#15395=ADVANCED_FACE ( 'NONE', ( #21750 ), #12808, .T. ) ;
#15396=EDGE_CURVE ( 'NONE', #51222, #31290, #5210, .T. ) ;
#15397=ORIENTED_EDGE ( 'NONE', *, *, #32193, .T. ) ;
#15399=LINE ( 'NONE', #18807, #35517 ) ;
#15400=EDGE_CURVE ( 'NONE', #8154, #41535, #49610, .T. ) ;
#15401=CIRCLE ( 'NONE', #44765, 10.00000000000000178 ) ;
#15404=VERTEX_POINT ( 'NONE', #29361 ) ;
#15405=LINE ( 'NONE', #31414, #34820 ) ;
#15406=EDGE_CURVE ( 'NONE', #650, #4203, #13594, .T. ) ;
#15407=FACE_OUTER_BOUND ( 'NONE', #26786, .T. ) ;
#15410=CYLINDRICAL_SURFACE ( 'NONE', #19124, 10.00000000000000178 ) ;
#15414=DIRECTION ( 'NONE',  ( 0.000000000000000000, 0.000000000000000000, 1.000000000000000000 ) ) ;
#15415=EDGE_LOOP ( 'NONE', ( #14492, #23661, #6455, #21771 ) ) ;
#15416=EDGE_LOOP ( 'NONE', ( #24276, #11015, #50471, #48265 ) ) ;
#15417=CIRCLE ( 'NONE', #310, 125.0000000000000000 ) ;
#15418=EDGE_CURVE ( 'NONE', #48304, #48442, #37511, .T. ) ;
#15419=ORIENTED_EDGE ( 'NONE', *, *, #14322, .T. ) ;
#15421=CYLINDRICAL_SURFACE ( 'NONE', #36068, 125.0000000000000000 ) ;
#15422=ADVANCED_FACE ( 'NONE', ( #29617 ), #45669, .T. ) ;
#15425=CARTESIAN_POINT ( 'NONE',  ( 60.51025563957495734, -175.3837268820161057, 59.13814366165117065 ) ) ;
#15426=EDGE_LOOP ( 'NONE', ( #12597, #1823, #11580, #25695 ) ) ;
#15430=CARTESIAN_POINT ( 'NONE',  ( -112.7586829773731267, -189.7472609257535510, -107.2060569716373521 ) ) ;
#15431=ORIENTED_EDGE ( 'NONE', *, *, #6987, .F. ) ;
#15432=CARTESIAN_POINT ( 'NONE',  ( -48.53836737940257251, -189.7472609257535510, 0.9982437317643279018 ) ) ;
#15434=AXIS2_PLACEMENT_3D ( 'NONE', #1002, #12573, #44636 ) ;
#15436=LINE ( 'NONE', #30655, #42589 ) ;
#15437=CARTESIAN_POINT ( 'NONE',  ( -159.0901268547125653, -193.5000000000000000, 58.22548115875957109 ) ) ;
#15438=LINE ( 'NONE', #39575, #11207 ) ;
#15439=DIRECTION ( 'NONE',  ( -0.9982437317643222396, 0.000000000000000000, 0.05924062789370006937 ) ) ;
#15440=ORIENTED_EDGE ( 'NONE', *, *, #33400, .T. ) ;
#15441=FACE_OUTER_BOUND ( 'NONE', #8746, .T. ) ;
#15444=ORIENTED_EDGE ( 'NONE', *, *, #11473, .F. ) ;
#15447=CARTESIAN_POINT ( 'NONE',  ( 76.52053249983504202, -177.1207230881787780, -0.2918682030015403162 ) ) ;
#15448=AXIS2_PLACEMENT_3D ( 'NONE', #16028, #4713, #20743 ) ;
#15449=CARTESIAN_POINT ( 'NONE',  ( 53.18081239921338721, -175.3837268820161057, -72.73415134495935774 ) ) ;
#15450=FACE_OUTER_BOUND ( 'NONE', #7793, .T. ) ;
#15451=DIRECTION ( 'NONE',  ( 0.000000000000000000, 0.000000000000000000, 1.000000000000000000 ) ) ;
#15452=ORIENTED_EDGE ( 'NONE', *, *, #21501, .T. ) ;
#15453=LINE ( 'NONE', #43558, #33882 ) ;
#15455=CIRCLE ( 'NONE', #3685, 125.0000000000000000 ) ;
#15456=CARTESIAN_POINT ( 'NONE',  ( -173.2419626162308646, -177.1207230881787780, 7.696413904698416353 ) ) ;
#15457=ORIENTED_EDGE ( 'NONE', *, *, #16467, .F. ) ;
#15458=CARTESIAN_POINT ( 'NONE',  ( -48.47912675150885065, -177.1207230881787780, 6.938893903907228378E-15 ) ) ;
#15460=ADVANCED_FACE ( 'NONE', ( #51178 ), #3062, .T. ) ;
#15461=ORIENTED_EDGE ( 'NONE', *, *, #20343, .F. ) ;
#15462=EDGE_CURVE ( 'NONE', #12462, #48052, #11239, .T. ) ;
#15464=VECTOR ( 'NONE', #20707, 1000.000000000000000 ) ;
#15467=FACE_BOUND ( 'NONE', #33514, .T. ) ;
#15468=FACE_OUTER_BOUND ( 'NONE', #27083, .T. ) ;
#15469=ORIENTED_EDGE ( 'NONE', *, *, #38051, .F. ) ;
#15471=ORIENTED_EDGE ( 'NONE', *, *, #17883, .T. ) ;
#15473=DIRECTION ( 'NONE',  ( 0.000000000000000000, 1.000000000000000000, 0.000000000000000000 ) ) ;
#15475=EDGE_CURVE ( 'NONE', #29517, #38097, #43125, .T. ) ;
#15476=DIRECTION ( 'NONE',  ( 0.000000000000000000, -1.000000000000000000, 0.000000000000000000 ) ) ;
#15478=AXIS2_PLACEMENT_3D ( 'NONE', #2630, #10262, #18154 ) ;
#15480=ADVANCED_FACE ( 'NONE', ( #42485 ), #38790, .T. ) ;
#15483=EDGE_LOOP ( 'NONE', ( #5493, #37185, #32939, #45616 ) ) ;
#15484=DIRECTION ( 'NONE',  ( -0.000000000000000000, 1.000000000000000000, -0.000000000000000000 ) ) ;
#15485=DIRECTION ( 'NONE',  ( 0.000000000000000000, 1.000000000000000000, 0.000000000000000000 ) ) ;
#15486=ORIENTED_EDGE ( 'NONE', *, *, #44353, .T. ) ;
#15487=CARTESIAN_POINT ( 'NONE',  ( -161.6832731452239784, -189.7472609257535510, -53.00774697410100345 ) ) ;
#15488=VERTEX_POINT ( 'NONE', #10423 ) ;
#15489=DIRECTION ( 'NONE',  ( 0.000000000000000000, 0.000000000000000000, -1.000000000000000000 ) ) ;
#15490=ORIENTED_EDGE ( 'NONE', *, *, #26294, .T. ) ;
#15491=DIRECTION ( 'NONE',  ( 0.000000000000000000, -0.000000000000000000, 1.000000000000000000 ) ) ;
#15492=VERTEX_POINT ( 'NONE', #2796 ) ;
#15493=DIRECTION ( 'NONE',  ( 0.000000000000000000, 0.000000000000000000, 1.000000000000000000 ) ) ;
#15494=CARTESIAN_POINT ( 'NONE',  ( 12.99855592850622443, -177.1207230881787780, 108.8370090194294875 ) ) ;
#15496=ORIENTED_EDGE ( 'NONE', *, *, #42547, .T. ) ;
#15497=DIRECTION ( 'NONE',  ( 0.8757349421956379665, 0.000000000000000000, -0.4827922027307427477 ) ) ;
#15498=ORIENTED_EDGE ( 'NONE', *, *, #16334, .T. ) ;
#15502=DIRECTION ( 'NONE',  ( 0.000000000000000000, 0.000000000000000000, -1.000000000000000000 ) ) ;
#15508=LINE ( 'NONE', #20218, #12877 ) ;
#15511=ORIENTED_EDGE ( 'NONE', *, *, #11520, .F. ) ;
#15512=CARTESIAN_POINT ( 'NONE',  ( -48.53836737940255119, -189.7472609257535510, -0.9982437317643153563 ) ) ;
#15513=CARTESIAN_POINT ( 'NONE',  ( 40.30419662299490824, -183.6283474603465606, -87.99159897727903967 ) ) ;
#15515=CIRCLE ( 'NONE', #50747, 125.0000000000000000 ) ;
#15516=DIRECTION ( 'NONE',  ( -0.000000000000000000, 1.000000000000000000, -0.000000000000000000 ) ) ;
#15517=LINE ( 'NONE', #46298, #40888 ) ;
#15519=EDGE_CURVE ( 'NONE', #2868, #5990, #10169, .T. ) ;
#15522=CIRCLE ( 'NONE', #44886, 125.0000000000000000 ) ;
#15523=CARTESIAN_POINT ( 'NONE',  ( -29.73468717939733708, -193.5000000000000000, 123.5865930638410930 ) ) ;
#15525=VECTOR ( 'NONE', #6821, 1000.000000000000000 ) ;
#15526=DIRECTION ( 'NONE',  ( 0.4566292373937140270, 0.000000000000000000, -0.8896570909947467687 ) ) ;
#15527=CARTESIAN_POINT ( 'NONE',  ( -124.4642912599203584, -189.7472609257535510, 99.25348746834863789 ) ) ;
#15532=ORIENTED_EDGE ( 'NONE', *, *, #5424, .F. ) ;
#15535=LINE ( 'NONE', #12353, #46033 ) ;
#15538=FACE_OUTER_BOUND ( 'NONE', #3990, .T. ) ;
#15541=DIRECTION ( 'NONE',  ( 0.000000000000000000, -1.000000000000000000, 0.000000000000000000 ) ) ;
#15542=ORIENTED_EDGE ( 'NONE', *, *, #1048, .F. ) ;
#15548=EDGE_LOOP ( 'NONE', ( #18398, #23567, #17046, #34800 ) ) ;
#15553=CARTESIAN_POINT ( 'NONE',  ( -48.47912675150885065, -183.6283474603465606, 6.938893903907228378E-15 ) ) ;
#15554=VECTOR ( 'NONE', #29596, 1000.000000000000000 ) ;
#15558=ORIENTED_EDGE ( 'NONE', *, *, #2546, .F. ) ;
#15559=VECTOR ( 'NONE', #47749, 1000.000000000000227 ) ;
#15560=CARTESIAN_POINT ( 'NONE',  ( -109.0835867659424565, -193.5000000000000000, -109.3256576763154726 ) ) ;
#15562=FACE_OUTER_BOUND ( 'NONE', #3172, .T. ) ;
#15566=AXIS2_PLACEMENT_3D ( 'NONE', #26521, #42040, #14203 ) ;
#15568=EDGE_CURVE ( 'NONE', #11646, #15597, #42756, .T. ) ;
#15569=DIRECTION ( 'NONE',  ( 0.000000000000000000, 0.000000000000000000, 1.000000000000000000 ) ) ;
#15570=AXIS2_PLACEMENT_3D ( 'NONE', #51481, #27557, #43588 ) ;
#15572=DIRECTION ( 'NONE',  ( 0.000000000000000000, -0.000000000000000000, -1.000000000000000000 ) ) ;
#15573=EDGE_LOOP ( 'NONE', ( #2587, #20912, #48744, #5339 ) ) ;
#15574=CARTESIAN_POINT ( 'NONE',  ( -102.5006284722404502, -177.1207230881787780, -112.7238987608084386 ) ) ;
#15575=DIRECTION ( 'NONE',  ( 0.000000000000000000, -1.000000000000000000, 0.000000000000000000 ) ) ;
#15576=CYLINDRICAL_SURFACE ( 'NONE', #31907, 125.0000000000000000 ) ;
#15578=CARTESIAN_POINT ( 'NONE',  ( 11.61413489515543418, -177.1207230881787780, -109.6074810615842381 ) ) ;
#15579=ADVANCED_FACE ( 'NONE', ( #26718 ), #18577, .T. ) ;
#15581=FACE_OUTER_BOUND ( 'NONE', #34065, .T. ) ;
#15582=ADVANCED_FACE ( 'NONE', ( #46968 ), #10949, .T. ) ;
#15584=DIRECTION ( 'NONE',  ( -0.000000000000000000, 1.000000000000000000, -0.000000000000000000 ) ) ;
#15585=LINE ( 'NONE', #16358, #33138 ) ;
#15586=CARTESIAN_POINT ( 'NONE',  ( -67.10529315269982931, -183.6283474603465606, -122.5936119678274565 ) ) ;
#15587=ORIENTED_EDGE ( 'NONE', *, *, #11812, .F. ) ;
#15590=ORIENTED_EDGE ( 'NONE', *, *, #20484, .F. ) ;
#15591=DIRECTION ( 'NONE',  ( -0.000000000000000000, 1.000000000000000000, -0.000000000000000000 ) ) ;
#15592=CARTESIAN_POINT ( 'NONE',  ( -11.47118876952528765, -189.7472609257535510, 118.3487137068149053 ) ) ;
#15593=ORIENTED_EDGE ( 'NONE', *, *, #32069, .F. ) ;
#15596=VECTOR ( 'NONE', #26137, 1000.000000000000000 ) ;
#15597=VERTEX_POINT ( 'NONE', #47742 ) ;
#15600=FACE_OUTER_BOUND ( 'NONE', #2893, .T. ) ;
#15601=AXIS2_PLACEMENT_3D ( 'NONE', #14095, #22743, #39012 ) ;
#15602=DIRECTION ( 'NONE',  ( 0.000000000000000000, 0.000000000000000000, 1.000000000000000000 ) ) ;
#15603=VECTOR ( 'NONE', #27035, 1000.000000000000000 ) ;
#15604=DIRECTION ( 'NONE',  ( -0.000000000000000000, 1.000000000000000000, -0.000000000000000000 ) ) ;
#15606=EDGE_LOOP ( 'NONE', ( #46827, #27308, #12813, #36436 ) ) ;
#15607=ORIENTED_EDGE ( 'NONE', *, *, #19190, .T. ) ;
#15608=VECTOR ( 'NONE', #4831, 1000.000000000000000 ) ;
#15610=CARTESIAN_POINT ( 'NONE',  ( -109.9568094315246327, -183.6283474603465606, -108.8370090194290611 ) ) ;
#15612=DIRECTION ( 'NONE',  ( -0.7765238627180349740, 0.000000000000000000, -0.6300878435817203194 ) ) ;
#15613=PLANE ( 'NONE',  #22234 ) ;
#15614=VERTEX_POINT ( 'NONE', #15425 ) ;
#15616=DIRECTION ( 'NONE',  ( -0.000000000000000000, 1.000000000000000000, -0.000000000000000000 ) ) ;
#15618=EDGE_LOOP ( 'NONE', ( #12451, #5064, #4583, #21271 ) ) ;
#15619=ORIENTED_EDGE ( 'NONE', *, *, #26176, .F. ) ;
#15620=VECTOR ( 'NONE', #19437, 1000.000000000000114 ) ;
#15622=DIRECTION ( 'NONE',  ( -0.05924062789370748011, 0.000000000000000000, -0.9982437317643217956 ) ) ;
#15623=CIRCLE ( 'NONE', #9769, 125.0000000000000000 ) ;
#15625=ORIENTED_EDGE ( 'NONE', *, *, #41967, .T. ) ;
#15627=AXIS2_PLACEMENT_3D ( 'NONE', #36548, #5298, #12634 ) ;
#15632=ORIENTED_EDGE ( 'NONE', *, *, #27401, .F. ) ;
#15633=DIRECTION ( 'NONE',  ( 0.000000000000000000, 0.000000000000000000, 1.000000000000000000 ) ) ;
#15636=CIRCLE ( 'NONE', #22346, 124.9999999999999858 ) ;
#15637=DIRECTION ( 'NONE',  ( -0.7378332790417239107, 0.000000000000000000, -0.6749830015182142207 ) ) ;
#15640=VECTOR ( 'NONE', #30890, 999.9999999999998863 ) ;
#15641=CIRCLE ( 'NONE', #34207, 125.0000000000000000 ) ;
#15642=DIRECTION ( 'NONE',  ( -0.000000000000000000, 1.000000000000000000, -0.000000000000000000 ) ) ;
#15644=DIRECTION ( 'NONE',  ( -0.000000000000000000, 1.000000000000000000, -0.000000000000000000 ) ) ;
#15645=EDGE_CURVE ( 'NONE', #25767, #31054, #27745, .T. ) ;
#15646=VECTOR ( 'NONE', #11270, 1000.000000000000000 ) ;
#15647=LINE ( 'NONE', #19069, #44199 ) ;
#15648=EDGE_CURVE ( 'NONE', #25351, #4219, #8042, .T. ) ;
#15650=CARTESIAN_POINT ( 'NONE',  ( -131.8938452225253855, -177.1207230881787780, 93.09664195018557109 ) ) ;
#15651=VECTOR ( 'NONE', #22481, 1000.000000000000114 ) ;
#15652=VERTEX_POINT ( 'NONE', #23311 ) ;
#15655=LINE ( 'NONE', #39790, #13425 ) ;
#15658=EDGE_CURVE ( 'NONE', #43736, #47366, #36442, .T. ) ;
#15661=CARTESIAN_POINT ( 'NONE',  ( 67.29469129333651267, -177.1207230881787780, -44.41421852208627996 ) ) ;
#15662=CIRCLE ( 'NONE', #18172, 125.0000000000000000 ) ;
#15664=ORIENTED_EDGE ( 'NONE', *, *, #7396, .T. ) ;
#15665=LINE ( 'NONE', #3825, #24254 ) ;
#15667=VERTEX_POINT ( 'NONE', #48527 ) ;
#15669=CARTESIAN_POINT ( 'NONE',  ( 26.89923761108473954, -189.7472609257535510, -98.45863302693476271 ) ) ;
#15670=VECTOR ( 'NONE', #556, 1000.000000000000000 ) ;
#15672=CARTESIAN_POINT ( 'NONE',  ( -28.74596282265200387, -193.5000000000000000, 123.4325817657431230 ) ) ;
#15673=ORIENTED_EDGE ( 'NONE', *, *, #35536, .T. ) ;
#15675=ORIENTED_EDGE ( 'NONE', *, *, #11248, .T. ) ;
#15678=AXIS2_PLACEMENT_3D ( 'NONE', #48523, #23547, #11445 ) ;
#15679=CIRCLE ( 'NONE', #51767, 125.0000000000000000 ) ;
#15680=PLANE ( 'NONE',  #49482 ) ;
#15686=VECTOR ( 'NONE', #35891, 1000.000000000000000 ) ;
#15687=VECTOR ( 'NONE', #31052, 1000.000000000000114 ) ;
#15688=CARTESIAN_POINT ( 'NONE',  ( -171.9128728525929262, -193.5000000000000000, 11.83705339977326965 ) ) ;
#15693=ORIENTED_EDGE ( 'NONE', *, *, #40425, .T. ) ;
#15694=DIRECTION ( 'NONE',  ( -0.000000000000000000, 1.000000000000000000, 0.000000000000000000 ) ) ;
#15696=ADVANCED_FACE ( 'NONE', ( #47472 ), #43532, .T. ) ;
#15699=ADVANCED_FACE ( 'NONE', ( #3574 ), #31696, .T. ) ;
#15700=CARTESIAN_POINT ( 'NONE',  ( 45.66222513722991749, -183.6283474603465606, 80.70646587903453906 ) ) ;
#15701=VERTEX_POINT ( 'NONE', #51951 ) ;
#15702=DIRECTION ( 'NONE',  ( 0.000000000000000000, -0.000000000000000000, 1.000000000000000000 ) ) ;
#15704=ORIENTED_EDGE ( 'NONE', *, *, #19424, .F. ) ;
#15705=DIRECTION ( 'NONE',  ( -0.05924062789370006937, 0.000000000000000000, -0.9982437317643222396 ) ) ;
#15706=VECTOR ( 'NONE', #3166, 1000.000000000000114 ) ;
#15707=EDGE_CURVE ( 'NONE', #2833, #4101, #3733, .T. ) ;
#15708=CARTESIAN_POINT ( 'NONE',  ( -152.8713435144644563, -177.1207230881787780, -68.75510947788596638 ) ) ;
#15710=LINE ( 'NONE', #15449, #411 ) ;
#15711=CIRCLE ( 'NONE', #6485, 125.0000000000000000 ) ;
#15716=LINE ( 'NONE', #19637, #43114 ) ;
#15718=ADVANCED_FACE ( 'NONE', ( #12501 ), #20643, .T. ) ;
#15719=FACE_BOUND ( 'NONE', #47162, .T. ) ;
#15720=ORIENTED_EDGE ( 'NONE', *, *, #17963, .T. ) ;
#15722=ADVANCED_FACE ( 'NONE', ( #36680 ), #21422, .T. ) ;
#15723=VECTOR ( 'NONE', #28962, 1000.000000000000114 ) ;
#15726=AXIS2_PLACEMENT_3D ( 'NONE', #16092, #9247, #25269 ) ;
#15727=FACE_OUTER_BOUND ( 'NONE', #29457, .T. ) ;
#15728=EDGE_CURVE ( 'NONE', #13540, #30593, #25618, .T. ) ;
#15729=ORIENTED_EDGE ( 'NONE', *, *, #43423, .F. ) ;
#15731=VECTOR ( 'NONE', #40231, 1000.000000000000114 ) ;
#15733=ADVANCED_FACE ( 'NONE', ( #29560 ), #13286, .T. ) ;
#15734=VECTOR ( 'NONE', #17387, 1000.000000000000000 ) ;
#15735=EDGE_CURVE ( 'NONE', #16447, #34175, #37189, .T. ) ;
#15736=LINE ( 'NONE', #19394, #15891 ) ;
#15737=FACE_BOUND ( 'NONE', #47342, .T. ) ;
#15738=PLANE ( 'NONE',  #2768 ) ;
#15739=ORIENTED_EDGE ( 'NONE', *, *, #9829, .F. ) ;
#15741=ADVANCED_FACE ( 'NONE', ( #13007 ), #5151, .T. ) ;
#15742=ORIENTED_EDGE ( 'NONE', *, *, #641, .T. ) ;
#15743=VERTEX_POINT ( 'NONE', #5674 ) ;
#15744=CARTESIAN_POINT ( 'NONE',  ( -156.2577088867455473, -183.6283474603465606, -63.31490529818422885 ) ) ;
#15748=DIRECTION ( 'NONE',  ( 0.000000000000000000, 0.000000000000000000, 1.000000000000000000 ) ) ;
#15752=DIRECTION ( 'NONE',  ( 0.000000000000000000, 0.000000000000000000, -1.000000000000000000 ) ) ;
#15754=CARTESIAN_POINT ( 'NONE',  ( -60.80616967713028487, -193.5000000000000000, -123.3865623328508292 ) ) ;
#15755=CARTESIAN_POINT ( 'NONE',  ( -144.0067397530739584, -193.5000000000000000, -80.61932246194587037 ) ) ;
#15756=ORIENTED_EDGE ( 'NONE', *, *, #6800, .F. ) ;
#15757=AXIS2_PLACEMENT_3D ( 'NONE', #26437, #42470, #6495 ) ;
#15759=AXIS2_PLACEMENT_3D ( 'NONE', #21298, #26013, #41793 ) ;
#15760=AXIS2_PLACEMENT_3D ( 'NONE', #32744, #16464, #36413 ) ;
#15761=DIRECTION ( 'NONE',  ( -0.9785564922995046988, 0.000000000000000000, 0.2059786187410953262 ) ) ;
#15762=ORIENTED_EDGE ( 'NONE', *, *, #51776, .T. ) ;
#15763=CARTESIAN_POINT ( 'NONE',  ( 71.87891646118019651, -189.7472609257535510, -33.74820638215424395 ) ) ;
#15764=ORIENTED_EDGE ( 'NONE', *, *, #17007, .T. ) ;
#15768=CARTESIAN_POINT ( 'NONE',  ( -151.9915035862630646, -177.1207230881787780, 70.07273251429430161 ) ) ;
#15769=VERTEX_POINT ( 'NONE', #1455 ) ;
#15770=CARTESIAN_POINT ( 'NONE',  ( 71.15591247552652021, -177.1207230881787780, 36.22785377504034443 ) ) ;
#15771=LINE ( 'NONE', #31780, #47663 ) ;
#15772=ORIENTED_EDGE ( 'NONE', *, *, #27825, .F. ) ;
#15773=EDGE_CURVE ( 'NONE', #4130, #27476, #29036, .T. ) ;
#15775=EDGE_CURVE ( 'NONE', #47743, #6051, #7089, .T. ) ;
#15777=ORIENTED_EDGE ( 'NONE', *, *, #50380, .T. ) ;
#15779=PLANE ( 'NONE',  #29034 ) ;
#15780=CARTESIAN_POINT ( 'NONE',  ( -160.7804753152582293, -193.5000000000000000, -52.57768177182447999 ) ) ;
#15781=CARTESIAN_POINT ( 'NONE',  ( 31.28129687248616619, -193.5000000000000000, 96.24590808611479531 ) ) ;
#15782=CARTESIAN_POINT ( 'NONE',  ( -55.99477380783406488, -175.3837268820161057, 123.7720294769269742 ) ) ;
#15783=LINE ( 'NONE', #36235, #13827 ) ;
#15784=ORIENTED_EDGE ( 'NONE', *, *, #51886, .F. ) ;
#15786=CARTESIAN_POINT ( 'NONE',  ( -107.1845112550870027, -177.1207230881787780, 109.2239789693437331 ) ) ;
#15787=CARTESIAN_POINT ( 'NONE',  ( 50.70030191143631981, -183.6283474603465606, -76.08180419845318454 ) ) ;
#15788=ORIENTED_EDGE ( 'NONE', *, *, #572, .F. ) ;
#15789=CIRCLE ( 'NONE', #25003, 125.0000000000000000 ) ;
#15790=AXIS2_PLACEMENT_3D ( 'NONE', #28596, #44393, #44641 ) ;
#15791=CARTESIAN_POINT ( 'NONE',  ( -50.83192613281184435, -183.6283474603465606, 123.9784823535113816 ) ) ;
#15792=EDGE_CURVE ( 'NONE', #45794, #18389, #17506, .T. ) ;
#15793=AXIS2_PLACEMENT_3D ( 'NONE', #35299, #31356, #50322 ) ;
#15794=DIRECTION ( 'NONE',  ( -0.9890401873221654760, 0.000000000000000000, 0.1476465640024710868 ) ) ;
#15796=VERTEX_POINT ( 'NONE', #4615 ) ;
#15798=ORIENTED_EDGE ( 'NONE', *, *, #45278, .T. ) ;
#15800=FACE_OUTER_BOUND ( 'NONE', #48587, .T. ) ;
#15801=DIRECTION ( 'NONE',  ( -0.000000000000000000, 1.000000000000000000, -0.000000000000000000 ) ) ;
#15804=CARTESIAN_POINT ( 'NONE',  ( -48.47912675150885065, -175.3837268820161057, 6.938893903907228378E-15 ) ) ;
#15805=CIRCLE ( 'NONE', #33394, 125.0000000000000000 ) ;
#15806=ORIENTED_EDGE ( 'NONE', *, *, #26390, .T. ) ;
#15807=EDGE_LOOP ( 'NONE', ( #35191, #40838, #11017, #28298 ) ) ;
#15808=ORIENTED_EDGE ( 'NONE', *, *, #25015, .F. ) ;
#15809=DIRECTION ( 'NONE',  ( -0.8294056854502011022, 0.000000000000000000, -0.5586467658036535777 ) ) ;
#15812=DIRECTION ( 'NONE',  ( 0.000000000000000000, 0.000000000000000000, 1.000000000000000000 ) ) ;
#15815=VERTEX_POINT ( 'NONE', #33248 ) ;
#15816=AXIS2_PLACEMENT_3D ( 'NONE', #43792, #11735, #23824 ) ;
#15817=AXIS2_PLACEMENT_3D ( 'NONE', #44959, #24987, #1587 ) ;
#15819=ORIENTED_EDGE ( 'NONE', *, *, #20503, .F. ) ;
#15821=CIRCLE ( 'NONE', #11602, 125.0000000000000000 ) ;
#15823=EDGE_CURVE ( 'NONE', #45342, #41076, #41643, .T. ) ;
#15824=DIRECTION ( 'NONE',  ( -0.6749830015182091136, 0.000000000000000000, -0.7378332790417285736 ) ) ;
#15826=DIRECTION ( 'NONE',  ( 0.000000000000000000, 1.000000000000000000, 0.000000000000000000 ) ) ;
#15827=PLANE ( 'NONE',  #49181 ) ;
#15828=ORIENTED_EDGE ( 'NONE', *, *, #15279, .F. ) ;
#15829=AXIS2_PLACEMENT_3D ( 'NONE', #3258, #35298, #35547 ) ;
#15830=PLANE ( 'NONE',  #42451 ) ;
#15833=ORIENTED_EDGE ( 'NONE', *, *, #2683, .F. ) ;
#15834=DIRECTION ( 'NONE',  ( -0.8858462335218260097, 0.000000000000000000, -0.4639789333096864810 ) ) ;
#15835=CARTESIAN_POINT ( 'NONE',  ( -144.6608085595393618, -189.7472609257535510, -78.26291788638665992 ) ) ;
#15837=EDGE_LOOP ( 'NONE', ( #36953, #10545, #6490, #50522 ) ) ;
#15841=EDGE_LOOP ( 'NONE', ( #15756, #6659, #49520, #3561 ) ) ;
#15842=PLANE ( 'NONE',  #34983 ) ;
#15846=EDGE_CURVE ( 'NONE', #25260, #4153, #25371, .T. ) ;
#15847=DIRECTION ( 'NONE',  ( 0.9785564922995017012, 0.000000000000000000, 0.2059786187411094538 ) ) ;
#15848=CARTESIAN_POINT ( 'NONE',  ( -63.09433862318514485, -189.7472609257535510, -124.1426420773539547 ) ) ;
#15849=FACE_OUTER_BOUND ( 'NONE', #5362, .T. ) ;
#15850=CARTESIAN_POINT ( 'NONE',  ( -161.2555905272863868, -189.7472609257535510, -53.91167979418499812 ) ) ;
#15852=CIRCLE ( 'NONE', #7445, 125.0000000000000000 ) ;
#15853=CARTESIAN_POINT ( 'NONE',  ( -170.0502155641509319, -193.5000000000000000, -29.07697310430878090 ) ) ;
#15854=CARTESIAN_POINT ( 'NONE',  ( -48.98765787015805984, -175.3837268820161057, -0.8610436117673551104 ) ) ;
#15855=LINE ( 'NONE', #42912, #25362 ) ;
#15856=EDGE_LOOP ( 'NONE', ( #38289, #26196, #40511, #10296 ) ) ;
#15857=AXIS2_PLACEMENT_3D ( 'NONE', #13925, #2079, #50971 ) ;
#15858=ORIENTED_EDGE ( 'NONE', *, *, #18488, .T. ) ;
#15861=DIRECTION ( 'NONE',  ( 0.000000000000000000, 1.000000000000000000, 0.000000000000000000 ) ) ;
#15863=AXIS2_PLACEMENT_3D ( 'NONE', #1234, #33310, #13341 ) ;
#15865=EDGE_LOOP ( 'NONE', ( #3453, #39294, #4544, #109 ) ) ;
#15866=CARTESIAN_POINT ( 'NONE',  ( -48.47912675150885065, -173.5000000000000284, 6.938893903907228378E-15 ) ) ;
#15868=CARTESIAN_POINT ( 'NONE',  ( -48.59739992243020623, -183.6283474603465606, -0.9929810960135115883 ) ) ;
#15869=LINE ( 'NONE', #26898, #17424 ) ;
#15871=ORIENTED_EDGE ( 'NONE', *, *, #7398, .T. ) ;
#15874=EDGE_CURVE ( 'NONE', #18957, #11444, #24712, .T. ) ;
#15875=CARTESIAN_POINT ( 'NONE',  ( -158.3442440847886985, -189.7472609257535510, -59.62093586438118109 ) ) ;
#15876=FACE_OUTER_BOUND ( 'NONE', #5125, .T. ) ;
#15877=DIRECTION ( 'NONE',  ( -0.000000000000000000, 1.000000000000000000, -0.000000000000000000 ) ) ;
#15881=DIRECTION ( 'NONE',  ( -0.6528221181905280446, 0.000000000000000000, 0.7575112421616145841 ) ) ;
#15882=EDGE_CURVE ( 'NONE', #17543, #37732, #28900, .T. ) ;
#15883=DIRECTION ( 'NONE',  ( -0.000000000000000000, 1.000000000000000000, -0.000000000000000000 ) ) ;
#15884=CARTESIAN_POINT ( 'NONE',  ( 47.70255505652112049, -193.5000000000000000, 78.26291788638732783 ) ) ;
#15885=ORIENTED_EDGE ( 'NONE', *, *, #28871, .T. ) ;
#15886=ORIENTED_EDGE ( 'NONE', *, *, #46606, .T. ) ;
#15887=EDGE_CURVE ( 'NONE', #51600, #46293, #22718, .T. ) ;
#15888=ORIENTED_EDGE ( 'NONE', *, *, #16504, .F. ) ;
#15890=DIRECTION ( 'NONE',  ( 0.000000000000000000, 0.000000000000000000, 1.000000000000000000 ) ) ;
#15891=VECTOR ( 'NONE', #2593, 1000.000000000000000 ) ;
#15897=EDGE_LOOP ( 'NONE', ( #21217, #38064, #44738, #463 ) ) ;
#15900=CARTESIAN_POINT ( 'NONE',  ( -48.47912675150885065, -183.6283474603465606, 6.938893903907228378E-15 ) ) ;
#15902=FACE_BOUND ( 'NONE', #6274, .T. ) ;
#15903=LINE ( 'NONE', #47950, #42854 ) ;
#15905=EDGE_LOOP ( 'NONE', ( #4974, #43713, #28809, #52005 ) ) ;
#15906=DIRECTION ( 'NONE',  ( 0.000000000000000000, 1.000000000000000000, -0.000000000000000000 ) ) ;
#15907=CYLINDRICAL_SURFACE ( 'NONE', #24703, 125.0000000000000000 ) ;
#15908=FACE_OUTER_BOUND ( 'NONE', #43207, .T. ) ;
#15909=DIRECTION ( 'NONE',  ( 0.4566292373937140270, 0.000000000000000000, -0.8896570909947467687 ) ) ;
#15910=AXIS2_PLACEMENT_3D ( 'NONE', #10784, #6326, #10510 ) ;
#15912=DIRECTION ( 'NONE',  ( 0.3758275821142292861, 0.000000000000000000, 0.9266896074318371479 ) ) ;
#15914=ORIENTED_EDGE ( 'NONE', *, *, #33546, .T. ) ;
#15916=DIRECTION ( 'NONE',  ( 0.000000000000000000, -0.000000000000000000, -1.000000000000000000 ) ) ;
#15917=ORIENTED_EDGE ( 'NONE', *, *, #7691, .F. ) ;
#15918=VERTEX_POINT ( 'NONE', #50846 ) ;
#15920=CARTESIAN_POINT ( 'NONE',  ( -170.6250538923603131, -189.7472609257535510, 26.55884942729649723 ) ) ;
#15922=AXIS2_PLACEMENT_3D ( 'NONE', #723, #31988, #24132 ) ;
#15927=DIRECTION ( 'NONE',  ( -0.9929810960135185827, 0.000000000000000000, 0.1182731709213523247 ) ) ;
#15928=CIRCLE ( 'NONE', #27656, 124.9999999999999858 ) ;
#15929=EDGE_CURVE ( 'NONE', #12643, #38136, #49898, .T. ) ;
#15930=EDGE_CURVE ( 'NONE', #8565, #18537, #22200, .T. ) ;
#15932=FACE_OUTER_BOUND ( 'NONE', #2195, .T. ) ;
#15933=ORIENTED_EDGE ( 'NONE', *, *, #39410, .T. ) ;
#15934=ORIENTED_EDGE ( 'NONE', *, *, #27608, .F. ) ;
#15935=EDGE_LOOP ( 'NONE', ( #35080, #30105, #47072, #38597 ) ) ;
#15936=CARTESIAN_POINT ( 'NONE',  ( -169.2746641285359317, -189.7472609257535510, -32.14713283941905786 ) ) ;
#15937=DIRECTION ( 'NONE',  ( -0.5085311186492273983, 0.000000000000000000, 0.8610436117673514467 ) ) ;
#15938=PLANE ( 'NONE',  #25124 ) ;
#15939=DIRECTION ( 'NONE',  ( -0.000000000000000000, -1.000000000000000000, 0.000000000000000000 ) ) ;
#15942=ADVANCED_FACE ( 'NONE', ( #19040 ), #50074, .T. ) ;
#15943=EDGE_CURVE ( 'NONE', #32738, #42284, #22202, .T. ) ;
#15944=AXIS2_PLACEMENT_3D ( 'NONE', #13590, #13343, #33311 ) ;
#15945=DIRECTION ( 'NONE',  ( 0.000000000000000000, 0.000000000000000000, 1.000000000000000000 ) ) ;
#15948=FACE_OUTER_BOUND ( 'NONE', #37680, .T. ) ;
#15949=VERTEX_POINT ( 'NONE', #34290 ) ;
#15950=VERTEX_POINT ( 'NONE', #2998 ) ;
#15952=LINE ( 'NONE', #44568, #32494 ) ;
#15953=DIRECTION ( 'NONE',  ( 0.000000000000000000, 0.000000000000000000, 1.000000000000000000 ) ) ;
#15954=EDGE_CURVE ( 'NONE', #9440, #14212, #42162, .T. ) ;
#15955=CARTESIAN_POINT ( 'NONE',  ( -47.50057025920934706, -177.1207230881787780, 0.2059786187411091207 ) ) ;
#15961=DIRECTION ( 'NONE',  ( -0.000000000000000000, 1.000000000000000000, -0.000000000000000000 ) ) ;
#15963=PLANE ( 'NONE',  #33709 ) ;
#15964=CARTESIAN_POINT ( 'NONE',  ( 75.01583293582058332, -193.5000000000000000, 11.18012358327990086 ) ) ;
#15965=DIRECTION ( 'NONE',  ( 0.3482016354343928088, 0.000000000000000000, 0.9374196611341231167 ) ) ;
#15966=CARTESIAN_POINT ( 'NONE',  ( -48.71401279728982558, -193.5000000000000000, -0.9720229140804069745 ) ) ;
#15967=LINE ( 'NONE', #44066, #15312 ) ;
#15968=ORIENTED_EDGE ( 'NONE', *, *, #31518, .F. ) ;
#15970=CARTESIAN_POINT ( 'NONE',  ( 10.73478887071927623, -193.5000000000000000, -110.0850225811106924 ) ) ;
#15971=FACE_BOUND ( 'NONE', #37143, .T. ) ;
#15972=EDGE_LOOP ( 'NONE', ( #30147, #17389, #41203, #33955 ) ) ;
#15976=FACE_OUTER_BOUND ( 'NONE', #25481, .T. ) ;
#15977=ORIENTED_EDGE ( 'NONE', *, *, #22114, .T. ) ;
#15978=AXIS2_PLACEMENT_3D ( 'NONE', #13474, #9530, #48959 ) ;
#15979=AXIS2_PLACEMENT_3D ( 'NONE', #45768, #41825, #6343 ) ;
#15980=LINE ( 'NONE', #20423, #1668 ) ;
#15981=FACE_BOUND ( 'NONE', #29639, .T. ) ;
#15982=CARTESIAN_POINT ( 'NONE',  ( -73.94077438226447896, -177.1207230881787780, 122.3793467049372481 ) ) ;
#15984=EDGE_CURVE ( 'NONE', #17851, #16442, #30866, .T. ) ;
#15990=VERTEX_POINT ( 'NONE', #30587 ) ;
#15991=LINE ( 'NONE', #15744, #47751 ) ;
#15993=ORIENTED_EDGE ( 'NONE', *, *, #24893, .F. ) ;
#15994=ADVANCED_FACE ( 'NONE', ( #46909 ), #14320, .F. ) ;
#15995=DIRECTION ( 'NONE',  ( -0.6965510290629982615, 0.000000000000000000, 0.7175072570443298270 ) ) ;
#15996=EDGE_CURVE ( 'NONE', #8921, #18649, #9603, .T. ) ;
#15998=EDGE_CURVE ( 'NONE', #42041, #33417, #45867, .T. ) ;
#16001=DIRECTION ( 'NONE',  ( -0.1768902751225666370, 0.000000000000000000, -0.9842305779475979399 ) ) ;
#16002=VERTEX_POINT ( 'NONE', #48187 ) ;
#16003=CARTESIAN_POINT ( 'NONE',  ( 1.663811650136608034, -175.3837268820161057, -113.4093733337827530 ) ) ;
#16004=DIRECTION ( 'NONE',  ( -0.4031234292879600778, 0.000000000000000000, -0.9151456172430237901 ) ) ;
#16008=FACE_OUTER_BOUND ( 'NONE', #42048, .T. ) ;
#16009=ORIENTED_EDGE ( 'NONE', *, *, #28184, .F. ) ;
#16010=DIRECTION ( 'NONE',  ( -0.000000000000000000, 1.000000000000000000, -0.000000000000000000 ) ) ;
#16012=EDGE_CURVE ( 'NONE', #779, #19842, #7123, .T. ) ;
#16013=DIRECTION ( 'NONE',  ( 0.000000000000000000, 0.000000000000000000, 1.000000000000000000 ) ) ;
#16015=DIRECTION ( 'NONE',  ( 0.000000000000000000, 1.000000000000000000, 0.000000000000000000 ) ) ;
#16017=EDGE_LOOP ( 'NONE', ( #6138, #43422, #12330, #12347 ) ) ;
#16018=AXIS2_PLACEMENT_3D ( 'NONE', #46834, #46320, #10821 ) ;
#16019=CIRCLE ( 'NONE', #29423, 125.0000000000000000 ) ;
#16020=ORIENTED_EDGE ( 'NONE', *, *, #36138, .T. ) ;
#16021=CARTESIAN_POINT ( 'NONE',  ( -36.09284319799462537, -193.5000000000000000, 124.3848060646152618 ) ) ;
#16022=DIRECTION ( 'NONE',  ( -0.7765238627180393038, 0.000000000000000000, -0.6300878435817147682 ) ) ;
#16025=DIRECTION ( 'NONE',  ( 6.978251959525016136E-17, 0.000000000000000000, 1.000000000000000000 ) ) ;
#16027=ORIENTED_EDGE ( 'NONE', *, *, #38177, .F. ) ;
#16028=CARTESIAN_POINT ( 'NONE',  ( -48.47912675150885065, -183.6283474603465606, 6.938893903907228378E-15 ) ) ;
#16030=LINE ( 'NONE', #12057, #15620 ) ;
#16032=ORIENTED_EDGE ( 'NONE', *, *, #5257, .F. ) ;
#16033=VECTOR ( 'NONE', #41379, 1000.000000000000000 ) ;
#16034=CARTESIAN_POINT ( 'NONE',  ( -171.5592422664403216, -183.6283474603465606, -21.82395850507258928 ) ) ;
#16036=DIRECTION ( 'NONE',  ( 0.9646355819083576311, 0.000000000000000000, 0.2635871660690715101 ) ) ;
#16039=VERTEX_POINT ( 'NONE', #15109 ) ;
#16040=EDGE_CURVE ( 'NONE', #19079, #7467, #36087, .T. ) ;
#16041=CARTESIAN_POINT ( 'NONE',  ( -48.47912675150885065, -189.7472609257535510, 6.938893903907228378E-15 ) ) ;
#16042=FACE_OUTER_BOUND ( 'NONE', #21506, .T. ) ;
#16043=PLANE ( 'NONE',  #36289 ) ;
#16044=CARTESIAN_POINT ( 'NONE',  ( -154.2693405752510500, -175.3837268820161057, 66.58401203837830451 ) ) ;
#16046=VERTEX_POINT ( 'NONE', #27424 ) ;
#16048=EDGE_CURVE ( 'NONE', #3432, #150, #26428, .T. ) ;
#16049=EDGE_CURVE ( 'NONE', #16791, #25116, #44242, .T. ) ;
#16051=VERTEX_POINT ( 'NONE', #8235 ) ;
#16052=ADVANCED_FACE ( 'NONE', ( #83 ), #15613, .T. ) ;
#16055=EDGE_LOOP ( 'NONE', ( #25884, #30517, #1840, #21311 ) ) ;
#16056=ORIENTED_EDGE ( 'NONE', *, *, #32905, .F. ) ;
#16058=ADVANCED_FACE ( 'NONE', ( #43718 ), #3271, .T. ) ;
#16060=DIRECTION ( 'NONE',  ( 0.000000000000000000, -1.000000000000000000, 0.000000000000000000 ) ) ;
#16062=DIRECTION ( 'NONE',  ( 0.000000000000000000, 0.000000000000000000, -1.000000000000000000 ) ) ;
#16063=CARTESIAN_POINT ( 'NONE',  ( -106.4764934152196645, -213.5000000000000000, 110.7307791902283043 ) ) ;
#16064=VERTEX_POINT ( 'NONE', #11661 ) ;
#16065=CIRCLE ( 'NONE', #10166, 124.9999999999999858 ) ;
#16066=ADVANCED_FACE ( 'NONE', ( #23745 ), #47408, .T. ) ;
#16067=DIRECTION ( 'NONE',  ( 0.000000000000000000, 1.000000000000000000, 0.000000000000000000 ) ) ;
#16068=ORIENTED_EDGE ( 'NONE', *, *, #51189, .F. ) ;
#16069=DIRECTION ( 'NONE',  ( 0.000000000000000000, -1.000000000000000000, 0.000000000000000000 ) ) ;
#16071=EDGE_CURVE ( 'NONE', #5652, #45186, #23497, .T. ) ;
#16072=CARTESIAN_POINT ( 'NONE',  ( -109.5001801941309196, -177.1207230881787780, -107.9473519284343297 ) ) ;
#16073=CARTESIAN_POINT ( 'NONE',  ( -16.77927958806650821, -177.1207230881787780, -120.9136869416130082 ) ) ;
#16075=LINE ( 'NONE', #20261, #27357 ) ;
#16076=VERTEX_POINT ( 'NONE', #11905 ) ;
#16082=DIRECTION ( 'NONE',  ( 0.000000000000000000, 1.000000000000000000, -0.000000000000000000 ) ) ;
#16083=VECTOR ( 'NONE', #4862, 1000.000000000000000 ) ;
#16084=DIRECTION ( 'NONE',  ( -0.000000000000000000, 1.000000000000000000, 0.000000000000000000 ) ) ;
#16085=ORIENTED_EDGE ( 'NONE', *, *, #8288, .F. ) ;
#16086=CARTESIAN_POINT ( 'NONE',  ( 141.7825277784304205, -193.5000000000000000, -9.999999999999987566 ) ) ;
#16089=AXIS2_PLACEMENT_3D ( 'NONE', #43633, #40200, #47068 ) ;
#16091=ORIENTED_EDGE ( 'NONE', *, *, #37513, .T. ) ;
#16092=CARTESIAN_POINT ( 'NONE',  ( -48.47912675150885065, -189.7472609257535510, 6.938893903907228378E-15 ) ) ;
#16093=ORIENTED_EDGE ( 'NONE', *, *, #20694, .F. ) ;
#16094=CARTESIAN_POINT ( 'NONE',  ( 58.12687231399078058, -177.1207230881787780, -63.33473559879913495 ) ) ;
#16095=FACE_OUTER_BOUND ( 'NONE', #25982, .T. ) ;
#16097=DIRECTION ( 'NONE',  ( 0.000000000000000000, 1.000000000000000000, -0.000000000000000000 ) ) ;
#16098=DIRECTION ( 'NONE',  ( -0.9646355819083594074, 0.000000000000000000, 0.2635871660690647933 ) ) ;
#16101=AXIS2_PLACEMENT_3D ( 'NONE', #10422, #45412, #29881 ) ;
#16102=PLANE ( 'NONE',  #1821 ) ;
#16103=LINE ( 'NONE', #32117, #12111 ) ;
#16104=DIRECTION ( 'NONE',  ( 0.9995608365087942371, 0.000000000000000000, 0.02963332782256331357 ) ) ;
#16107=EDGE_CURVE ( 'NONE', #31330, #26846, #20544, .T. ) ;
#16108=ADVANCED_FACE ( 'NONE', ( #36609 ), #45297, .T. ) ;
#16110=CARTESIAN_POINT ( 'NONE',  ( -48.47912675150885065, -175.3837268820161057, 6.938893903907228378E-15 ) ) ;
#16111=ORIENTED_EDGE ( 'NONE', *, *, #51330, .F. ) ;
#16114=CARTESIAN_POINT ( 'NONE',  ( 76.04209377433249983, -189.7472609257535510, -10.93003379476865611 ) ) ;
#16116=DIRECTION ( 'NONE',  ( 0.000000000000000000, 0.000000000000000000, 1.000000000000000000 ) ) ;
#16117=DIRECTION ( 'NONE',  ( 0.000000000000000000, -1.000000000000000000, 0.000000000000000000 ) ) ;
#16118=VECTOR ( 'NONE', #27967, 1000.000000000000000 ) ;
#16119=ORIENTED_EDGE ( 'NONE', *, *, #4162, .T. ) ;
#16122=ORIENTED_EDGE ( 'NONE', *, *, #34270, .T. ) ;
#16123=CARTESIAN_POINT ( 'NONE',  ( -116.2964108826154330, -177.1207230881787780, -105.0038855142073260 ) ) ;
#16125=CARTESIAN_POINT ( 'NONE',  ( -23.01747912075234836, -177.1207230881787780, -122.3793467049370634 ) ) ;
#16126=ADVANCED_FACE ( 'NONE', ( #32911 ), #9535, .T. ) ;
#16127=FACE_OUTER_BOUND ( 'NONE', #41458, .T. ) ;
#16129=VERTEX_POINT ( 'NONE', #29244 ) ;
#16130=CARTESIAN_POINT ( 'NONE',  ( 9.518239912201957864, -193.5000000000000000, -110.7307791902283043 ) ) ;
#16132=CARTESIAN_POINT ( 'NONE',  ( -48.47912675150885065, -175.3837268820161057, -0.9999999999999931166 ) ) ;
#16133=CARTESIAN_POINT ( 'NONE',  ( -155.4465502054561057, -193.5000000000000000, 64.67588669375881238 ) ) ;
#16134=AXIS2_PLACEMENT_3D ( 'NONE', #46618, #41359, #21922 ) ;
#16136=EDGE_LOOP ( 'NONE', ( #34409, #2072, #46061, #31449 ) ) ;
#16137=ORIENTED_EDGE ( 'NONE', *, *, #45313, .T. ) ;
#16139=ORIENTED_EDGE ( 'NONE', *, *, #44534, .T. ) ;
#16140=VECTOR ( 'NONE', #40017, 1000.000000000000227 ) ;
#16142=CARTESIAN_POINT ( 'NONE',  ( -98.71382891444395113, -189.7472609257535510, -114.4616734920523555 ) ) ;
#16144=CARTESIAN_POINT ( 'NONE',  ( -78.64590280292341617, -175.3837268820161057, -121.3052580173827408 ) ) ;
#16145=PLANE ( 'NONE',  #29589 ) ;
#16146=PLANE ( 'NONE',  #20936 ) ;
#16148=PLANE ( 'NONE',  #22571 ) ;
#16149=VERTEX_POINT ( 'NONE', #17441 ) ;
#16152=CARTESIAN_POINT ( 'NONE',  ( -48.47912675150885065, -183.6283474603465606, 6.938893903907228378E-15 ) ) ;
#16155=EDGE_LOOP ( 'NONE', ( #27323, #27827, #30679, #24615 ) ) ;
#16156=AXIS2_PLACEMENT_3D ( 'NONE', #16021, #480, #23883 ) ;
#16157=CARTESIAN_POINT ( 'NONE',  ( 34.23904069044534992, -177.1207230881787780, -92.37913469314065651 ) ) ;
#16160=DIRECTION ( 'NONE',  ( -0.5586467658036476935, 0.000000000000000000, -0.8294056854502049880 ) ) ;
#16162=ORIENTED_EDGE ( 'NONE', *, *, #42993, .T. ) ;
#16164=EDGE_LOOP ( 'NONE', ( #32733, #25933, #16343, #35072 ) ) ;
#16165=ORIENTED_EDGE ( 'NONE', *, *, #42216, .T. ) ;
#16167=VERTEX_POINT ( 'NONE', #29488 ) ;
#16168=ORIENTED_EDGE ( 'NONE', *, *, #29045, .T. ) ;
#16169=FACE_OUTER_BOUND ( 'NONE', #37959, .T. ) ;
#16170=EDGE_CURVE ( 'NONE', #29802, #25337, #32398, .T. ) ;
#16171=CIRCLE ( 'NONE', #45552, 125.0000000000000000 ) ;
#16172=VECTOR ( 'NONE', #19811, 1000.000000000000000 ) ;
#16176=VERTEX_POINT ( 'NONE', #605 ) ;
#16178=DIRECTION ( 'NONE',  ( 0.000000000000000000, -1.000000000000000000, 0.000000000000000000 ) ) ;
#16179=ORIENTED_EDGE ( 'NONE', *, *, #43345, .T. ) ;
#16180=LINE ( 'NONE', #28504, #10713 ) ;
#16181=CYLINDRICAL_SURFACE ( 'NONE', #46810, 125.0000000000000000 ) ;
#16182=ADVANCED_FACE ( 'NONE', ( #16388 ), #45032, .F. ) ;
#16186=VERTEX_POINT ( 'NONE', #25552 ) ;
#16188=CARTESIAN_POINT ( 'NONE',  ( -29.73468717939733708, -177.1207230881787780, 123.5865930638410930 ) ) ;
#16189=CARTESIAN_POINT ( 'NONE',  ( 8.750818922897904528, -175.3837268820161057, -111.1293539894138434 ) ) ;
#16190=EDGE_CURVE ( 'NONE', #30709, #30058, #28703, .T. ) ;
#16194=AXIS2_PLACEMENT_3D ( 'NONE', #42179, #41931, #26149 ) ;
#16197=ORIENTED_EDGE ( 'NONE', *, *, #48142, .F. ) ;
#16199=ORIENTED_EDGE ( 'NONE', *, *, #48156, .F. ) ;
#16200=ORIENTED_EDGE ( 'NONE', *, *, #25634, .F. ) ;
#16201=CARTESIAN_POINT ( 'NONE',  ( -47.82630463331833681, -193.5000000000000000, 0.7575112421616305713 ) ) ;
#16203=DIRECTION ( 'NONE',  ( 0.9266896074318343723, 0.000000000000000000, -0.3758275821142357809 ) ) ;
#16207=CIRCLE ( 'NONE', #4463, 125.0000000000000000 ) ;
#16208=ORIENTED_EDGE ( 'NONE', *, *, #37307, .F. ) ;
#16209=VECTOR ( 'NONE', #189, 1000.000000000000000 ) ;
#16210=VERTEX_POINT ( 'NONE', #48709 ) ;
#16212=AXIS2_PLACEMENT_3D ( 'NONE', #51329, #3240, #4014 ) ;
#16213=LINE ( 'NONE', #7801, #50497 ) ;
#16216=EDGE_CURVE ( 'NONE', #50565, #36650, #19712, .T. ) ;
#16217=FACE_OUTER_BOUND ( 'NONE', #118, .T. ) ;
#16218=DIRECTION ( 'NONE',  ( 0.6068001458185945385, 0.000000000000000000, -0.7948544414133523750 ) ) ;
#16219=VECTOR ( 'NONE', #45142, 1000.000000000000000 ) ;
#16220=ORIENTED_EDGE ( 'NONE', *, *, #30492, .T. ) ;
#16221=CARTESIAN_POINT ( 'NONE',  ( 34.23904069044534992, -193.5000000000000000, -92.37913469314065651 ) ) ;
#16223=ADVANCED_FACE ( 'NONE', ( #13478 ), #44760, .T. ) ;
#16224=FACE_BOUND ( 'NONE', #15043, .T. ) ;
#16226=CARTESIAN_POINT ( 'NONE',  ( -40.90423906728908321, -193.5000000000000000, -124.7702732086912221 ) ) ;
#16227=AXIS2_PLACEMENT_3D ( 'NONE', #51008, #22623, #18676 ) ;
#16229=ORIENTED_EDGE ( 'NONE', *, *, #34748, .T. ) ;
#16230=DIRECTION ( 'NONE',  ( 0.000000000000000000, 1.000000000000000000, 0.000000000000000000 ) ) ;
#16231=EDGE_CURVE ( 'NONE', #48776, #44261, #17221, .T. ) ;
#16232=ORIENTED_EDGE ( 'NONE', *, *, #39261, .T. ) ;
#16233=EDGE_CURVE ( 'NONE', #36797, #5120, #14701, .T. ) ;
#16235=LINE ( 'NONE', #32247, #10888 ) ;
#16236=EDGE_CURVE ( 'NONE', #23376, #5997, #33180, .T. ) ;
#16237=DIRECTION ( 'NONE',  ( -0.000000000000000000, 1.000000000000000000, -0.000000000000000000 ) ) ;
#16239=VERTEX_POINT ( 'NONE', #36345 ) ;
#16241=AXIS2_PLACEMENT_3D ( 'NONE', #36034, #3708, #51822 ) ;
#16245=CARTESIAN_POINT ( 'NONE',  ( -172.4465090799742484, -193.5000000000000000, -2.844930291600638927 ) ) ;
#16246=AXIS2_PLACEMENT_3D ( 'NONE', #37007, #36755, #32805 ) ;
#16247=VERTEX_POINT ( 'NONE', #337 ) ;
#16249=CARTESIAN_POINT ( 'NONE',  ( 6.443011874827243801, -177.1207230881787780, 112.2878385610370771 ) ) ;
#16250=DIRECTION ( 'NONE',  ( 0.000000000000000000, -1.000000000000000000, 0.000000000000000000 ) ) ;
#16252=VERTEX_POINT ( 'NONE', #5083 ) ;
#16258=DIRECTION ( 'NONE',  ( 0.000000000000000000, 1.000000000000000000, 0.000000000000000000 ) ) ;
#16261=DIRECTION ( 'NONE',  ( -0.3202698538628350744, 0.000000000000000000, -0.9473263538541923934 ) ) ;
#16262=EDGE_LOOP ( 'NONE', ( #33238, #14160, #32442, #37099 ) ) ;
#16263=CYLINDRICAL_SURFACE ( 'NONE', #24089, 125.0000000000000000 ) ;
#16264=DIRECTION ( 'NONE',  ( -0.000000000000000000, 1.000000000000000000, -0.000000000000000000 ) ) ;
#16265=ORIENTED_EDGE ( 'NONE', *, *, #39151, .T. ) ;
#16266=AXIS2_PLACEMENT_3D ( 'NONE', #42341, #30263, #6866 ) ;
#16268=DIRECTION ( 'NONE',  ( 0.5829794791144650157, 0.000000000000000000, 0.8124868780056864193 ) ) ;
#16269=LINE ( 'NONE', #40176, #41606 ) ;
#16270=PLANE ( 'NONE',  #14613 ) ;
#16271=CARTESIAN_POINT ( 'NONE',  ( -142.6204786402482512, -177.1207230881787780, -80.70646587903382851 ) ) ;
#16272=DIRECTION ( 'NONE',  ( -0.8124868780056742068, 0.000000000000000000, -0.5829794791144820021 ) ) ;
#16273=CARTESIAN_POINT ( 'NONE',  ( -4.176930889631405464, -189.7472609257535510, 116.8859077982279615 ) ) ;
#16275=VERTEX_POINT ( 'NONE', #41318 ) ;
#16278=AXIS2_PLACEMENT_3D ( 'NONE', #29100, #8875, #17803 ) ;
#16279=CARTESIAN_POINT ( 'NONE',  ( -120.2975302769383177, -177.1207230881787780, 102.3089288139534005 ) ) ;
#16280=CARTESIAN_POINT ( 'NONE',  ( -12.13476221271688615, -193.5000000000000000, 119.5996955107804638 ) ) ;
#16281=CARTESIAN_POINT ( 'NONE',  ( -49.38192458147459263, -183.6283474603465606, -0.4300652022765235616 ) ) ;
#16283=CYLINDRICAL_SURFACE ( 'NONE', #38267, 125.0000000000000000 ) ;
#16285=DIRECTION ( 'NONE',  ( -0.000000000000000000, 1.000000000000000000, -0.000000000000000000 ) ) ;
#16286=CARTESIAN_POINT ( 'NONE',  ( 1.352451982137491404, -189.7472609257535510, 113.5465278748096978 ) ) ;
#16289=ADVANCED_FACE ( 'NONE', ( #30795 ), #21631, .T. ) ;
#16290=VERTEX_POINT ( 'NONE', #13736 ) ;
#16292=DIRECTION ( 'NONE',  ( 0.000000000000000000, -0.000000000000000000, 1.000000000000000000 ) ) ;
#16293=EDGE_CURVE ( 'NONE', #19975, #35261, #2081, .T. ) ;
#16295=DIRECTION ( 'NONE',  ( 0.000000000000000000, 0.000000000000000000, 1.000000000000000000 ) ) ;
#16296=CARTESIAN_POINT ( 'NONE',  ( -14.28570516517293854, -183.6283474603465606, 120.2323164553486521 ) ) ;
#16297=CIRCLE ( 'NONE', #9586, 125.0000000000000000 ) ;
#16298=ADVANCED_FACE ( 'NONE', ( #50271 ), #30278, .T. ) ;
#16300=VECTOR ( 'NONE', #51255, 1000.000000000000000 ) ;
#16303=VECTOR ( 'NONE', #9624, 1000.000000000000000 ) ;
#16305=VERTEX_POINT ( 'NONE', #41853 ) ;
#16306=CARTESIAN_POINT ( 'NONE',  ( -117.6201219941651601, -175.3837268820161057, 104.1370384486469760 ) ) ;
#16307=VECTOR ( 'NONE', #49297, 1000.000000000000000 ) ;
#16308=EDGE_LOOP ( 'NONE', ( #30950, #25816, #30903, #15397 ) ) ;
#16309=CARTESIAN_POINT ( 'NONE',  ( 141.7825277784304205, -213.5000000000000000, 41.45482488023466772 ) ) ;
#16310=LINE ( 'NONE', #5019, #16844 ) ;
#16311=ADVANCED_FACE ( 'NONE', ( #6374 ), #38671, .F. ) ;
#16313=CARTESIAN_POINT ( 'NONE',  ( -48.47912675150885065, -177.1207230881787780, 6.938893903907228378E-15 ) ) ;
#16314=VERTEX_POINT ( 'NONE', #1902 ) ;
#16315=DIRECTION ( 'NONE',  ( -0.5085311186492154079, 0.000000000000000000, -0.8610436117673585521 ) ) ;
#16319=LINE ( 'NONE', #17572, #49295 ) ;
#16321=DIRECTION ( 'NONE',  ( 0.000000000000000000, 0.000000000000000000, -1.000000000000000000 ) ) ;
#16322=FACE_OUTER_BOUND ( 'NONE', #7486, .T. ) ;
#16324=EDGE_CURVE ( 'NONE', #9367, #14713, #38424, .T. ) ;
#16326=DIRECTION ( 'NONE',  ( 0.2635871660690715101, 0.000000000000000000, -0.9646355819083576311 ) ) ;
#16327=DIRECTION ( 'NONE',  ( -0.7378332790417189146, 0.000000000000000000, -0.6749830015182196608 ) ) ;
#16328=ORIENTED_EDGE ( 'NONE', *, *, #3625, .T. ) ;
#16329=DIRECTION ( 'NONE',  ( 0.9890401873221644768, 0.000000000000000000, -0.1476465640024779702 ) ) ;
#16331=AXIS2_PLACEMENT_3D ( 'NONE', #49443, #4758, #33119 ) ;
#16333=VECTOR ( 'NONE', #44475, 1000.000000000000114 ) ;
#16334=EDGE_CURVE ( 'NONE', #5462, #6625, #25569, .T. ) ;
#16335=EDGE_CURVE ( 'NONE', #32062, #24955, #29749, .T. ) ;
#16336=EDGE_CURVE ( 'NONE', #35575, #51281, #10827, .T. ) ;
#16337=EDGE_LOOP ( 'NONE', ( #24412, #51647, #36115, #24336 ) ) ;
#16338=EDGE_CURVE ( 'NONE', #18266, #24476, #45801, .T. ) ;
#16339=DIRECTION ( 'NONE',  ( -0.000000000000000000, 1.000000000000000000, -0.000000000000000000 ) ) ;
#16341=AXIS2_PLACEMENT_3D ( 'NONE', #8513, #40304, #31914 ) ;
#16342=EDGE_CURVE ( 'NONE', #5990, #6703, #45730, .T. ) ;
#16343=ORIENTED_EDGE ( 'NONE', *, *, #4453, .T. ) ;
#16344=CARTESIAN_POINT ( 'NONE',  ( -48.47912675150885065, -188.5000000000000284, -14.99999999999999289 ) ) ;
#16345=EDGE_LOOP ( 'NONE', ( #28620, #8242, #43659, #21417 ) ) ;
#16346=DIRECTION ( 'NONE',  ( 0.000000000000000000, 0.000000000000000000, -1.000000000000000000 ) ) ;
#16348=FACE_OUTER_BOUND ( 'NONE', #962, .T. ) ;
#16349=PLANE ( 'NONE',  #8420 ) ;
#16350=DIRECTION ( 'NONE',  ( 0.000000000000000000, 0.000000000000000000, 1.000000000000000000 ) ) ;
#16353=AXIS2_PLACEMENT_3D ( 'NONE', #37904, #30024, #9796 ) ;
#16354=ADVANCED_FACE ( 'NONE', ( #26333 ), #18458, .T. ) ;
#16356=ADVANCED_FACE ( 'NONE', ( #14782 ), #42626, .T. ) ;
#16357=LINE ( 'NONE', #32370, #40399 ) ;
#16358=CARTESIAN_POINT ( 'NONE',  ( -63.43218022845230308, -189.7472609257535510, 124.1024020384604540 ) ) ;
#16359=CARTESIAN_POINT ( 'NONE',  ( -147.8383830610225971, -193.5000000000000000, -74.18852968774183410 ) ) ;
#16361=ADVANCED_FACE ( 'NONE', ( #43132 ), #31045, .F. ) ;
#16362=ORIENTED_EDGE ( 'NONE', *, *, #10157, .T. ) ;
#16363=PLANE ( 'NONE',  #5663 ) ;
#16369=VERTEX_POINT ( 'NONE', #51817 ) ;
#16373=DIRECTION ( 'NONE',  ( -0.4031234292879792847, 0.000000000000000000, 0.9151456172430153524 ) ) ;
#16374=DIRECTION ( 'NONE',  ( -0.1768902751225733261, 0.000000000000000000, 0.9842305779475966077 ) ) ;
#16376=ORIENTED_EDGE ( 'NONE', *, *, #50725, .T. ) ;
#16378=VECTOR ( 'NONE', #437, 1000.000000000000000 ) ;
#16379=ORIENTED_EDGE ( 'NONE', *, *, #39268, .T. ) ;
#16380=EDGE_CURVE ( 'NONE', #32293, #50764, #17262, .T. ) ;
#16381=CARTESIAN_POINT ( 'NONE',  ( -162.4844509910036550, -193.5000000000000000, -48.77484799213890909 ) ) ;
#16382=LINE ( 'NONE', #858, #20165 ) ;
#16383=FACE_OUTER_BOUND ( 'NONE', #27636, .T. ) ;
#16384=VERTEX_POINT ( 'NONE', #7900 ) ;
#16385=CIRCLE ( 'NONE', #43194, 125.0000000000000000 ) ;
#16386=CARTESIAN_POINT ( 'NONE',  ( -171.4559849729830603, -177.1207230881787780, 22.39848972532369942 ) ) ;
#16388=FACE_OUTER_BOUND ( 'NONE', #15483, .T. ) ;
#16389=EDGE_LOOP ( 'NONE', ( #47542, #21581, #33637, #15213 ) ) ;
#16390=DIRECTION ( 'NONE',  ( -0.8294056854502011022, 0.000000000000000000, -0.5586467658036535777 ) ) ;
#16391=CARTESIAN_POINT ( 'NONE',  ( -160.0666658415768211, -193.5000000000000000, 54.07611884703389649 ) ) ;
#16392=AXIS2_PLACEMENT_3D ( 'NONE', #25763, #10245, #30467 ) ;
#16393=DIRECTION ( 'NONE',  ( 0.000000000000000000, 1.000000000000000000, 0.000000000000000000 ) ) ;
#16395=AXIS2_PLACEMENT_3D ( 'NONE', #4489, #524, #24988 ) ;
#16397=VERTEX_POINT ( 'NONE', #22912 ) ;
#16398=VERTEX_POINT ( 'NONE', #38925 ) ;
#16399=PLANE ( 'NONE',  #20602 ) ;
#16400=CYLINDRICAL_SURFACE ( 'NONE', #13259, 124.9999999999999858 ) ;
#16401=ORIENTED_EDGE ( 'NONE', *, *, #5473, .F. ) ;
#16402=CARTESIAN_POINT ( 'NONE',  ( -48.47912675150885065, -183.6283474603465606, 6.938893903907228378E-15 ) ) ;
#16403=LINE ( 'NONE', #28981, #7759 ) ;
#16404=EDGE_CURVE ( 'NONE', #40001, #12462, #7651, .T. ) ;
#16410=EDGE_CURVE ( 'NONE', #1773, #16914, #2931, .T. ) ;
#16412=DIRECTION ( 'NONE',  ( -0.000000000000000000, 1.000000000000000000, -0.000000000000000000 ) ) ;
#16413=EDGE_LOOP ( 'NONE', ( #44632, #19647, #70, #18512 ) ) ;
#16414=FACE_BOUND ( 'NONE', #32898, .T. ) ;
#16415=VECTOR ( 'NONE', #42894, 1000.000000000000000 ) ;
#16416=DIRECTION ( 'NONE',  ( 0.000000000000000000, 0.000000000000000000, -1.000000000000000000 ) ) ;
#16417=ORIENTED_EDGE ( 'NONE', *, *, #24024, .F. ) ;
#16419=VECTOR ( 'NONE', #18168, 1000.000000000000000 ) ;
#16420=FACE_OUTER_BOUND ( 'NONE', #12300, .T. ) ;
#16426=VERTEX_POINT ( 'NONE', #39195 ) ;
#16427=ORIENTED_EDGE ( 'NONE', *, *, #16894, .F. ) ;
#16429=AXIS2_PLACEMENT_3D ( 'NONE', #4361, #20131, #40340 ) ;
#16431=CARTESIAN_POINT ( 'NONE',  ( -170.2790847791494855, -183.6283474603465606, -28.10285082451569494 ) ) ;
#16434=EDGE_LOOP ( 'NONE', ( #17548, #39537, #435, #29319 ) ) ;
#16435=CARTESIAN_POINT ( 'NONE',  ( 53.56330073376472001, -189.7472609257535510, 72.19655804062048787 ) ) ;
#16436=VECTOR ( 'NONE', #24465, 1000.000000000000114 ) ;
#16442=VERTEX_POINT ( 'NONE', #36028 ) ;
#16444=FACE_OUTER_BOUND ( 'NONE', #44595, .T. ) ;
#16447=VERTEX_POINT ( 'NONE', #32078 ) ;
#16448=VERTEX_POINT ( 'NONE', #48119 ) ;
#16450=DIRECTION ( 'NONE',  ( 0.000000000000000000, 0.000000000000000000, 1.000000000000000000 ) ) ;
#16453=CARTESIAN_POINT ( 'NONE',  ( -48.47912675150885065, -177.1207230881787780, 6.938893903907228378E-15 ) ) ;
#16454=CIRCLE ( 'NONE', #46687, 125.0000000000000000 ) ;
#16458=ORIENTED_EDGE ( 'NONE', *, *, #14880, .F. ) ;
#16460=ORIENTED_EDGE ( 'NONE', *, *, #34275, .F. ) ;
#16461=ORIENTED_EDGE ( 'NONE', *, *, #40850, .T. ) ;
#16462=DIRECTION ( 'NONE',  ( 0.000000000000000000, 0.000000000000000000, 1.000000000000000000 ) ) ;
#16464=DIRECTION ( 'NONE',  ( -0.000000000000000000, 1.000000000000000000, -0.000000000000000000 ) ) ;
#16465=CIRCLE ( 'NONE', #45843, 125.0000000000000000 ) ;
#16466=DIRECTION ( 'NONE',  ( 0.000000000000000000, 0.000000000000000000, -1.000000000000000000 ) ) ;
#16467=EDGE_CURVE ( 'NONE', #36797, #794, #47616, .T. ) ;
#16468=CARTESIAN_POINT ( 'NONE',  ( 65.79610465833508215, -193.5000000000000000, -50.65739320401928580 ) ) ;
#16469=EDGE_LOOP ( 'NONE', ( #3224, #4951, #34420, #12019 ) ) ;
#16471=VECTOR ( 'NONE', #17890, 1000.000000000000000 ) ;
#16472=EDGE_LOOP ( 'NONE', ( #11854, #32957, #15729, #20161 ) ) ;
#16473=AXIS2_PLACEMENT_3D ( 'NONE', #3801, #10659, #42966 ) ;
#16474=VERTEX_POINT ( 'NONE', #11321 ) ;
#16477=CARTESIAN_POINT ( 'NONE',  ( -67.22356632362124174, -177.1207230881787780, -123.5865930638409509 ) ) ;
#16479=PLANE ( 'NONE',  #44816 ) ;
#16480=DIRECTION ( 'NONE',  ( -0.000000000000000000, 1.000000000000000000, -0.000000000000000000 ) ) ;
#16481=EDGE_LOOP ( 'NONE', ( #41595, #12796, #38748, #14679 ) ) ;
#16483=DIRECTION ( 'NONE',  ( -0.000000000000000000, 1.000000000000000000, -0.000000000000000000 ) ) ;
#16484=FACE_OUTER_BOUND ( 'NONE', #7017, .T. ) ;
#16485=FACE_BOUND ( 'NONE', #1365, .T. ) ;
#16486=ORIENTED_EDGE ( 'NONE', *, *, #35594, .F. ) ;
#16488=AXIS2_PLACEMENT_3D ( 'NONE', #32497, #24109, #44583 ) ;
#16489=EDGE_CURVE ( 'NONE', #13663, #51264, #2126, .T. ) ;
#16491=AXIS2_PLACEMENT_3D ( 'NONE', #21848, #44988, #37859 ) ;
#16493=ORIENTED_EDGE ( 'NONE', *, *, #5095, .F. ) ;
#16495=VERTEX_POINT ( 'NONE', #34995 ) ;
#16496=DIRECTION ( 'NONE',  ( -0.000000000000000000, 1.000000000000000000, -0.000000000000000000 ) ) ;
#16497=CIRCLE ( 'NONE', #25838, 124.9999999999999858 ) ;
#16498=CARTESIAN_POINT ( 'NONE',  ( 15.23368049493606335, -189.7472609257535510, -107.5438431188757136 ) ) ;
#16499=CARTESIAN_POINT ( 'NONE',  ( 69.04371411670898340, -193.5000000000000000, -39.55227055146230697 ) ) ;
#16501=ADVANCED_FACE ( 'NONE', ( #27095 ), #7137, .T. ) ;
#16502=CIRCLE ( 'NONE', #45879, 125.0000000000000000 ) ;
#16503=AXIS2_PLACEMENT_3D ( 'NONE', #6260, #50933, #22281 ) ;
#16504=EDGE_CURVE ( 'NONE', #28628, #49289, #36518, .T. ) ;
#16507=VERTEX_POINT ( 'NONE', #11599 ) ;
#16508=ORIENTED_EDGE ( 'NONE', *, *, #38177, .T. ) ;
#16509=AXIS2_PLACEMENT_3D ( 'NONE', #25829, #9542, #6129 ) ;
#16510=CARTESIAN_POINT ( 'NONE',  ( 116.9235303384055840, -213.5000000000000000, 10.00000000000000000 ) ) ;
#16513=VECTOR ( 'NONE', #35177, 999.9999999999998863 ) ;
#16514=DIRECTION ( 'NONE',  ( 0.7765238627180349740, 0.000000000000000000, 0.6300878435817203194 ) ) ;
#16516=CARTESIAN_POINT ( 'NONE',  ( -173.0563034899574859, -189.7472609257535510, -10.27263529369817618 ) ) ;
#16517=EDGE_CURVE ( 'NONE', #28894, #50885, #7159, .T. ) ;
#16519=DIRECTION ( 'NONE',  ( 0.000000000000000000, -1.000000000000000000, -0.000000000000000000 ) ) ;
#16520=ORIENTED_EDGE ( 'NONE', *, *, #7386, .F. ) ;
#16521=DIRECTION ( 'NONE',  ( -0.000000000000000000, 1.000000000000000000, -0.000000000000000000 ) ) ;
#16522=DIRECTION ( 'NONE',  ( 0.000000000000000000, -0.000000000000000000, 1.000000000000000000 ) ) ;
#16524=VECTOR ( 'NONE', #23522, 1000.000000000000000 ) ;
#16525=ORIENTED_EDGE ( 'NONE', *, *, #20067, .F. ) ;
#16526=AXIS2_PLACEMENT_3D ( 'NONE', #10086, #38184, #17723 ) ;
#16527=FACE_OUTER_BOUND ( 'NONE', #10154, .T. ) ;
#16528=EDGE_LOOP ( 'NONE', ( #16825, #20237, #46310, #46107 ) ) ;
#16531=VECTOR ( 'NONE', #15089, 1000.000000000000000 ) ;
#16532=CARTESIAN_POINT ( 'NONE',  ( 35.67816836544798065, -183.6283474603465606, -92.42591454022746689 ) ) ;
#16533=EDGE_CURVE ( 'NONE', #6563, #44074, #29808, .T. ) ;
#16534=CARTESIAN_POINT ( 'NONE',  ( -2.700932609314997457, -193.5000000000000000, -116.3157639405751809 ) ) ;
#16535=EDGE_LOOP ( 'NONE', ( #46347, #19364, #1343, #7920 ) ) ;
#16536=DIRECTION ( 'NONE',  ( -0.000000000000000000, 1.000000000000000000, -0.000000000000000000 ) ) ;
#16538=ORIENTED_EDGE ( 'NONE', *, *, #43964, .F. ) ;
#16540=VERTEX_POINT ( 'NONE', #21041 ) ;
#16541=LINE ( 'NONE', #31785, #40475 ) ;
#16542=CIRCLE ( 'NONE', #45057, 125.0000000000000000 ) ;
#16543=EDGE_CURVE ( 'NONE', #14578, #3536, #20509, .T. ) ;
#16545=AXIS2_PLACEMENT_3D ( 'NONE', #51361, #23999, #35559 ) ;
#16546=DIRECTION ( 'NONE',  ( 0.000000000000000000, -0.000000000000000000, 1.000000000000000000 ) ) ;
#16547=DIRECTION ( 'NONE',  ( -0.6965510290629882695, 0.000000000000000000, -0.7175072570443395970 ) ) ;
#16548=LINE ( 'NONE', #35452, #6459 ) ;
#16549=AXIS2_PLACEMENT_3D ( 'NONE', #36349, #1119, #28455 ) ;
#16550=AXIS2_PLACEMENT_3D ( 'NONE', #36838, #28414, #44463 ) ;
#16553=PLANE ( 'NONE',  #19458 ) ;
#16556=DIRECTION ( 'NONE',  ( -0.000000000000000000, 1.000000000000000000, -0.000000000000000000 ) ) ;
#16558=FACE_OUTER_BOUND ( 'NONE', #19046, .T. ) ;
#16562=ADVANCED_FACE ( 'NONE', ( #13415 ), #36277, .F. ) ;
#16564=DIRECTION ( 'NONE',  ( 0.000000000000000000, 0.000000000000000000, 1.000000000000000000 ) ) ;
#16566=ORIENTED_EDGE ( 'NONE', *, *, #40704, .T. ) ;
#16567=EDGE_LOOP ( 'NONE', ( #23480, #19673, #37430, #17681 ) ) ;
#16571=CARTESIAN_POINT ( 'NONE',  ( -145.2888470698896981, -193.5000000000000000, -77.48473115145239376 ) ) ;
#16575=CARTESIAN_POINT ( 'NONE',  ( 72.68824389704326450, -175.3837268820161057, -26.35287080855459863 ) ) ;
#16578=ORIENTED_EDGE ( 'NONE', *, *, #7832, .F. ) ;
#16579=AXIS2_PLACEMENT_3D ( 'NONE', #27208, #23021, #46686 ) ;
#16582=LINE ( 'NONE', #24983, #27540 ) ;
#16583=VECTOR ( 'NONE', #18074, 1000.000000000000000 ) ;
#16584=ADVANCED_FACE ( 'NONE', ( #24453 ), #20781, .F. ) ;
#16585=ADVANCED_FACE ( 'NONE', ( #48380 ), #1320, .T. ) ;
#16592=ORIENTED_EDGE ( 'NONE', *, *, #49030, .T. ) ;
#16593=CARTESIAN_POINT ( 'NONE',  ( -48.47912675150885065, -189.7472609257535510, 6.938893903907228378E-15 ) ) ;
#16594=ORIENTED_EDGE ( 'NONE', *, *, #11245, .F. ) ;
#16599=EDGE_CURVE ( 'NONE', #13870, #34792, #44440, .T. ) ;
#16601=DIRECTION ( 'NONE',  ( 0.000000000000000000, 1.000000000000000000, 0.000000000000000000 ) ) ;
#16602=CARTESIAN_POINT ( 'NONE',  ( 73.66680038934278230, -193.5000000000000000, -26.55884942729568365 ) ) ;
#16605=DIRECTION ( 'NONE',  ( -0.3758275821142357809, 0.000000000000000000, -0.9266896074318343723 ) ) ;
#16606=VECTOR ( 'NONE', #94, 1000.000000000000227 ) ;
#16607=CARTESIAN_POINT ( 'NONE',  ( -48.65601702663143868, -189.7472609257535510, 0.9842305779476024918 ) ) ;
#16608=AXIS2_PLACEMENT_3D ( 'NONE', #23380, #43602, #7597 ) ;
#16609=EDGE_CURVE ( 'NONE', #512, #48767, #41002, .T. ) ;
#16610=CARTESIAN_POINT ( 'NONE',  ( 28.02885774092381865, -189.7472609257535510, 98.85104101073331151 ) ) ;
#16611=ORIENTED_EDGE ( 'NONE', *, *, #38996, .F. ) ;
#16613=DIRECTION ( 'NONE',  ( 0.000000000000000000, 0.000000000000000000, 1.000000000000000000 ) ) ;
#16614=AXIS2_PLACEMENT_3D ( 'NONE', #5068, #5859, #9270 ) ;
#16615=CARTESIAN_POINT ( 'NONE',  ( -21.46839590530488451, -177.1207230881787780, 122.0467960216650738 ) ) ;
#16616=EDGE_CURVE ( 'NONE', #20140, #32545, #41549, .T. ) ;
#16618=DIRECTION ( 'NONE',  ( 0.9473263538541923934, 0.000000000000000000, -0.3202698538628350744 ) ) ;
#16622=ORIENTED_EDGE ( 'NONE', *, *, #29301, .T. ) ;
#16623=VECTOR ( 'NONE', #4880, 1000.000000000000000 ) ;
#16624=CARTESIAN_POINT ( 'NONE',  ( -9.671950287350391307, -193.5000000000000000, -118.8234112238815499 ) ) ;
#16625=DIRECTION ( 'NONE',  ( 0.000000000000000000, 0.000000000000000000, 1.000000000000000000 ) ) ;
#16626=CARTESIAN_POINT ( 'NONE',  ( -49.32472275501067571, -177.1207230881787780, -0.5338233779647935107 ) ) ;
#16629=PLANE ( 'NONE',  #11169 ) ;
#16630=AXIS2_PLACEMENT_3D ( 'NONE', #22320, #34414, #14454 ) ;
#16631=FACE_OUTER_BOUND ( 'NONE', #41409, .T. ) ;
#16632=CYLINDRICAL_SURFACE ( 'NONE', #50563, 125.0000000000000000 ) ;
#16633=FACE_OUTER_BOUND ( 'NONE', #29874, .T. ) ;
#16634=VERTEX_POINT ( 'NONE', #49441 ) ;
#16635=ORIENTED_EDGE ( 'NONE', *, *, #36402, .F. ) ;
#16636=LINE ( 'NONE', #8725, #47631 ) ;
#16637=DIRECTION ( 'NONE',  ( -0.6068001458185890984, 0.000000000000000000, -0.7948544414133565938 ) ) ;
#16638=ORIENTED_EDGE ( 'NONE', *, *, #32991, .F. ) ;
#16639=VECTOR ( 'NONE', #10709, 1000.000000000000114 ) ;
#16643=FACE_OUTER_BOUND ( 'NONE', #41020, .T. ) ;
#16644=VECTOR ( 'NONE', #19225, 1000.000000000000000 ) ;
#16645=EDGE_CURVE ( 'NONE', #2312, #45117, #27286, .T. ) ;
#16648=CARTESIAN_POINT ( 'NONE',  ( -48.13092511607445800, -183.6283474603465606, 0.9374196611341301111 ) ) ;
#16649=DIRECTION ( 'NONE',  ( -0.000000000000000000, 1.000000000000000000, 0.000000000000000000 ) ) ;
#16650=VERTEX_POINT ( 'NONE', #42558 ) ;
#16652=ADVANCED_FACE ( 'NONE', ( #22070 ), #33641, .T. ) ;
#16656=FACE_OUTER_BOUND ( 'NONE', #49626, .T. ) ;
#16657=ORIENTED_EDGE ( 'NONE', *, *, #44149, .T. ) ;
#16658=ADVANCED_FACE ( 'NONE', ( #6054 ), #49939, .T. ) ;
#16659=CARTESIAN_POINT ( 'NONE',  ( -142.9772358822569629, -177.1207230881787780, 81.82363577055969017 ) ) ;
#16664=LINE ( 'NONE', #45036, #49257 ) ;
#16666=DIRECTION ( 'NONE',  ( -0.000000000000000000, 1.000000000000000000, -0.000000000000000000 ) ) ;
#16667=CARTESIAN_POINT ( 'NONE',  ( 74.77174840718836890, -183.6283474603465606, 20.83798868929603998 ) ) ;
#16669=VECTOR ( 'NONE', #18405, 1000.000000000000000 ) ;
#16670=ORIENTED_EDGE ( 'NONE', *, *, #9633, .F. ) ;
#16673=ADVANCED_FACE ( 'NONE', ( #45738 ), #9731, .T. ) ;
#16674=LINE ( 'NONE', #36621, #39244 ) ;
#16675=EDGE_LOOP ( 'NONE', ( #26873, #43280, #8538, #35973 ) ) ;
#16676=CARTESIAN_POINT ( 'NONE',  ( 75.47134233844786877, -189.7472609257535510, -3.504489105734906129 ) ) ;
#16678=DIRECTION ( 'NONE',  ( 0.000000000000000000, -1.000000000000000000, 0.000000000000000000 ) ) ;
#16684=CARTESIAN_POINT ( 'NONE',  ( -70.42295845586430403, -189.7472609257535510, -123.0587999703025019 ) ) ;
#16685=EDGE_LOOP ( 'NONE', ( #41648, #19731, #4991, #13422 ) ) ;
#16687=AXIS2_PLACEMENT_3D ( 'NONE', #42282, #10998, #46765 ) ;
#16688=DIRECTION ( 'NONE',  ( 0.000000000000000000, -0.000000000000000000, -1.000000000000000000 ) ) ;
#16689=EDGE_LOOP ( 'NONE', ( #1617, #19498, #9809, #26927 ) ) ;
#16690=VECTOR ( 'NONE', #3376, 1000.000000000000000 ) ;
#16691=DIRECTION ( 'NONE',  ( 0.000000000000000000, 1.000000000000000000, 0.000000000000000000 ) ) ;
#16692=PLANE ( 'NONE',  #3724 ) ;
#16695=ADVANCED_FACE ( 'NONE', ( #46512 ), #10001, .T. ) ;
#16697=FACE_OUTER_BOUND ( 'NONE', #7243, .T. ) ;
#16698=VERTEX_POINT ( 'NONE', #5816 ) ;
#16702=DIRECTION ( 'NONE',  ( 0.000000000000000000, -1.000000000000000000, -0.000000000000000000 ) ) ;
#16703=ORIENTED_EDGE ( 'NONE', *, *, #12108, .F. ) ;
#16705=DIRECTION ( 'NONE',  ( 0.9960498426152171181, 0.000000000000000000, -0.08879589532293157006 ) ) ;
#16708=DIRECTION ( 'NONE',  ( 0.000000000000000000, 0.000000000000000000, 1.000000000000000000 ) ) ;
#16710=PLANE ( 'NONE',  #44063 ) ;
#16711=VERTEX_POINT ( 'NONE', #6577 ) ;
#16712=CARTESIAN_POINT ( 'NONE',  ( 57.66105628977221897, -193.5000000000000000, 66.02470404298190942 ) ) ;
#16713=PLANE ( 'NONE',  #22458 ) ;
#16714=EDGE_CURVE ( 'NONE', #18469, #23765, #50462, .T. ) ;
#16715=ADVANCED_FACE ( 'NONE', ( #34666 ), #26015, .T. ) ;
#16717=DIRECTION ( 'NONE',  ( -0.6528221181905119463, 0.000000000000000000, -0.7575112421616284619 ) ) ;
#16718=ORIENTED_EDGE ( 'NONE', *, *, #4731, .T. ) ;
#16720=ADVANCED_FACE ( 'NONE', ( #6306 ), #38612, .F. ) ;
#16721=ORIENTED_EDGE ( 'NONE', *, *, #46479, .F. ) ;
#16725=AXIS2_PLACEMENT_3D ( 'NONE', #48357, #12338, #44420 ) ;
#16726=DIRECTION ( 'NONE',  ( 0.000000000000000000, -1.000000000000000000, 0.000000000000000000 ) ) ;
#16728=CARTESIAN_POINT ( 'NONE',  ( -33.52607327456454556, -175.3837268820161057, -124.1024020384603119 ) ) ;
#16730=AXIS2_PLACEMENT_3D ( 'NONE', #12499, #16726, #8546 ) ;
#16733=ORIENTED_EDGE ( 'NONE', *, *, #48, .T. ) ;
#16735=CARTESIAN_POINT ( 'NONE',  ( -172.6359455740846442, -193.5000000000000000, -14.49428645563791562 ) ) ;
#16740=EDGE_CURVE ( 'NONE', #33166, #33429, #8018, .T. ) ;
#16742=DIRECTION ( 'NONE',  ( 0.000000000000000000, 0.000000000000000000, -1.000000000000000000 ) ) ;
#16743=ORIENTED_EDGE ( 'NONE', *, *, #30841, .F. ) ;
#16744=CARTESIAN_POINT ( 'NONE',  ( -41.24387117724851493, -175.3837268820161057, 124.7904286264581231 ) ) ;
#16746=EDGE_CURVE ( 'NONE', #20693, #6892, #21413, .T. ) ;
#16748=EDGE_LOOP ( 'NONE', ( #49264, #46400, #34836, #19933 ) ) ;
#16750=CARTESIAN_POINT ( 'NONE',  ( 51.05451324771860300, -177.1207230881787780, 75.61781872352698031 ) ) ;
#16751=FACE_OUTER_BOUND ( 'NONE', #49678, .T. ) ;
#16752=DIRECTION ( 'NONE',  ( -0.000000000000000000, 1.000000000000000000, -0.000000000000000000 ) ) ;
#16753=DIRECTION ( 'NONE',  ( 0.000000000000000000, 1.000000000000000000, 0.000000000000000000 ) ) ;
#16754=PLANE ( 'NONE',  #9593 ) ;
#16755=CARTESIAN_POINT ( 'NONE',  ( -47.57632892154311577, -193.5000000000000000, 0.4300652022765314997 ) ) ;
#16757=DIRECTION ( 'NONE',  ( -0.000000000000000000, 1.000000000000000000, -0.000000000000000000 ) ) ;
#16758=DIRECTION ( 'NONE',  ( -0.000000000000000000, 1.000000000000000000, -0.000000000000000000 ) ) ;
#16759=DIRECTION ( 'NONE',  ( 0.000000000000000000, 0.000000000000000000, -1.000000000000000000 ) ) ;
#16760=FACE_BOUND ( 'NONE', #22892, .T. ) ;
#16764=VERTEX_POINT ( 'NONE', #46774 ) ;
#16766=PLANE ( 'NONE',  #34527 ) ;
#16767=ORIENTED_EDGE ( 'NONE', *, *, #28902, .F. ) ;
#16771=CARTESIAN_POINT ( 'NONE',  ( -9.671950287350391307, -183.6283474603465606, -118.8234112238815641 ) ) ;
#16773=ORIENTED_EDGE ( 'NONE', *, *, #20144, .T. ) ;
#16774=ADVANCED_FACE ( 'NONE', ( #22848 ), #7349, .T. ) ;
#16775=EDGE_CURVE ( 'NONE', #975, #17445, #35970, .T. ) ;
#16777=EDGE_LOOP ( 'NONE', ( #8016, #24071, #8778, #49831 ) ) ;
#16781=LINE ( 'NONE', #9146, #3327 ) ;
#16783=LINE ( 'NONE', #8605, #1599 ) ;
#16784=DIRECTION ( 'NONE',  ( 0.000000000000000000, -1.000000000000000000, 0.000000000000000000 ) ) ;
#16787=CARTESIAN_POINT ( 'NONE',  ( -152.8876895714563773, -193.5000000000000000, 66.89437584437911255 ) ) ;
#16788=ORIENTED_EDGE ( 'NONE', *, *, #24913, .T. ) ;
#16790=CARTESIAN_POINT ( 'NONE',  ( -51.83230197877465883, -193.5000000000000000, 123.9551692589637639 ) ) ;
#16791=VERTEX_POINT ( 'NONE', #2869 ) ;
#16792=ORIENTED_EDGE ( 'NONE', *, *, #49922, .F. ) ;
#16793=VECTOR ( 'NONE', #33625, 1000.000000000000000 ) ;
#16794=EDGE_CURVE ( 'NONE', #46169, #17312, #26785, .T. ) ;
#16796=VERTEX_POINT ( 'NONE', #27806 ) ;
#16798=ORIENTED_EDGE ( 'NONE', *, *, #268, .F. ) ;
#16799=CARTESIAN_POINT ( 'NONE',  ( -171.5592422664403216, -177.1207230881787780, -21.82395850507255730 ) ) ;
#16800=CARTESIAN_POINT ( 'NONE',  ( -70.58093260035833794, -193.5000000000000000, 122.0143860769388908 ) ) ;
#16803=CARTESIAN_POINT ( 'NONE',  ( 70.02079272397770637, -183.6283474603465606, -36.52255268223056817 ) ) ;
#16804=ORIENTED_EDGE ( 'NONE', *, *, #8391, .T. ) ;
#16805=EDGE_CURVE ( 'NONE', #9746, #24906, #31772, .T. ) ;
#16810=DIRECTION ( 'NONE',  ( -0.000000000000000000, 1.000000000000000000, -0.000000000000000000 ) ) ;
#16811=EDGE_LOOP ( 'NONE', ( #17310, #49928, #25866, #7322 ) ) ;
#16812=DIRECTION ( 'NONE',  ( 0.000000000000000000, 1.000000000000000000, 0.000000000000000000 ) ) ;
#16814=FACE_OUTER_BOUND ( 'NONE', #20295, .T. ) ;
#16816=DIRECTION ( 'NONE',  ( -0.9890401873221654760, 0.000000000000000000, 0.1476465640024710868 ) ) ;
#16817=CIRCLE ( 'NONE', #43649, 125.0000000000000000 ) ;
#16818=AXIS2_PLACEMENT_3D ( 'NONE', #30365, #46673, #26697 ) ;
#16819=CARTESIAN_POINT ( 'NONE',  ( -48.47912675150885065, -175.3837268820161057, 6.938893903907228378E-15 ) ) ;
#16820=EDGE_LOOP ( 'NONE', ( #41093, #33690, #5131, #4311 ) ) ;
#16822=CARTESIAN_POINT ( 'NONE',  ( -153.7332855749581881, -189.7472609257535510, 67.42819922234390617 ) ) ;
#16824=DIRECTION ( 'NONE',  ( 0.4566292373937077542, 0.000000000000000000, 0.8896570909947499883 ) ) ;
#16825=ORIENTED_EDGE ( 'NONE', *, *, #14880, .T. ) ;
#16826=ORIENTED_EDGE ( 'NONE', *, *, #51590, .T. ) ;
#16828=EDGE_CURVE ( 'NONE', #37393, #46831, #11780, .T. ) ;
#16829=CARTESIAN_POINT ( 'NONE',  ( -47.78257572244586271, -193.5000000000000000, 0.7175072570443418174 ) ) ;
#16831=CARTESIAN_POINT ( 'NONE',  ( 63.39453919430264506, -175.3837268820161057, 53.48161459190911415 ) ) ;
#16832=CARTESIAN_POINT ( 'NONE',  ( -74.51199343215203896, -177.1207230881787780, -122.2591094863194741 ) ) ;
#16833=DIRECTION ( 'NONE',  ( 0.000000000000000000, 1.000000000000000000, 0.000000000000000000 ) ) ;
#16834=ORIENTED_EDGE ( 'NONE', *, *, #27600, .T. ) ;
#16836=EDGE_CURVE ( 'NONE', #32761, #47736, #3384, .T. ) ;
#16838=ORIENTED_EDGE ( 'NONE', *, *, #46492, .F. ) ;
#16840=ORIENTED_EDGE ( 'NONE', *, *, #26234, .F. ) ;
#16841=EDGE_CURVE ( 'NONE', #16447, #26457, #35437, .T. ) ;
#16842=ORIENTED_EDGE ( 'NONE', *, *, #2583, .F. ) ;
#16843=CARTESIAN_POINT ( 'NONE',  ( -145.6517069852672535, -193.5000000000000000, 78.62880929222943394 ) ) ;
#16844=VECTOR ( 'NONE', #37317, 1000.000000000000000 ) ;
#16848=DIRECTION ( 'NONE',  ( -0.000000000000000000, 1.000000000000000000, 0.000000000000000000 ) ) ;
#16850=ORIENTED_EDGE ( 'NONE', *, *, #9598, .T. ) ;
#16852=DIRECTION ( 'NONE',  ( -0.000000000000000000, 1.000000000000000000, -0.000000000000000000 ) ) ;
#16853=ORIENTED_EDGE ( 'NONE', *, *, #46754, .F. ) ;
#16854=CARTESIAN_POINT ( 'NONE',  ( -122.3978016498073345, -177.1207230881787780, -100.8019320314827070 ) ) ;
#16857=DIRECTION ( 'NONE',  ( -0.8294056854502011022, 0.000000000000000000, -0.5586467658036535777 ) ) ;
#16858=CARTESIAN_POINT ( 'NONE',  ( 10.73478887071926202, -183.6283474603465606, -110.0850225811106924 ) ) ;
#16859=LINE ( 'NONE', #24729, #23982 ) ;
#16860=ORIENTED_EDGE ( 'NONE', *, *, #989, .T. ) ;
#16861=CARTESIAN_POINT ( 'NONE',  ( -48.47912675150885065, -183.6283474603465606, 6.938893903907228378E-15 ) ) ;
#16864=AXIS2_PLACEMENT_3D ( 'NONE', #15152, #35890, #20631 ) ;
#16865=ORIENTED_EDGE ( 'NONE', *, *, #8217, .F. ) ;
#16866=LINE ( 'NONE', #5040, #32516 ) ;
#16870=CARTESIAN_POINT ( 'NONE',  ( 15.80042947435468470, -175.3837268820161057, 107.2060569716377927 ) ) ;
#16873=CARTESIAN_POINT ( 'NONE',  ( 46.40005841627164074, -177.1207230881787780, 81.38144888055276738 ) ) ;
#16874=FACE_OUTER_BOUND ( 'NONE', #6178, .T. ) ;
#16876=DIRECTION ( 'NONE',  ( -0.000000000000000000, 1.000000000000000000, -0.000000000000000000 ) ) ;
#16877=EDGE_CURVE ( 'NONE', #30392, #5462, #23111, .T. ) ;
#16880=EDGE_CURVE ( 'NONE', #12738, #13511, #18901, .T. ) ;
#16881=AXIS2_PLACEMENT_3D ( 'NONE', #5514, #18105, #2061 ) ;
#16882=LINE ( 'NONE', #17414, #48962 ) ;
#16883=DIRECTION ( 'NONE',  ( -0.000000000000000000, 1.000000000000000000, -0.000000000000000000 ) ) ;
#16884=DIRECTION ( 'NONE',  ( 0.6965510290629982615, 0.000000000000000000, -0.7175072570443298270 ) ) ;
#16886=ORIENTED_EDGE ( 'NONE', *, *, #24744, .F. ) ;
#16887=ORIENTED_EDGE ( 'NONE', *, *, #13934, .F. ) ;
#16888=CARTESIAN_POINT ( 'NONE',  ( 56.77503207194101265, -193.5000000000000000, -67.42819922234311036 ) ) ;
#16889=EDGE_CURVE ( 'NONE', #3837, #4082, #19413, .T. ) ;
#16890=EDGE_CURVE ( 'NONE', #31952, #17151, #35183, .T. ) ;
#16891=CARTESIAN_POINT ( 'NONE',  ( 73.03012110230136500, -189.7472609257535510, 24.72869175143112130 ) ) ;
#16893=ORIENTED_EDGE ( 'NONE', *, *, #15418, .F. ) ;
#16894=EDGE_CURVE ( 'NONE', #49449, #36064, #7079, .T. ) ;
#16895=VECTOR ( 'NONE', #16373, 1000.000000000000114 ) ;
#16897=DIRECTION ( 'NONE',  ( 0.8757349421956345248, 0.000000000000000000, 0.4827922027307490205 ) ) ;
#16898=DIRECTION ( 'NONE',  ( 0.000000000000000000, 0.000000000000000000, 1.000000000000000000 ) ) ;
#16899=LINE ( 'NONE', #49222, #10681 ) ;
#16902=CARTESIAN_POINT ( 'NONE',  ( 76.51419089073348800, -183.6283474603465606, -1.292495564988658030 ) ) ;
#16903=DIRECTION ( 'NONE',  ( -0.000000000000000000, 1.000000000000000000, -0.000000000000000000 ) ) ;
#16905=DIRECTION ( 'NONE',  ( 0.4031234292879730674, 0.000000000000000000, -0.9151456172430181280 ) ) ;
#16906=ORIENTED_EDGE ( 'NONE', *, *, #30478, .T. ) ;
#16907=DIRECTION ( 'NONE',  ( 0.000000000000000000, 0.000000000000000000, 1.000000000000000000 ) ) ;
#16909=ORIENTED_EDGE ( 'NONE', *, *, #41659, .F. ) ;
#16910=CARTESIAN_POINT ( 'NONE',  ( -169.1033029113419559, -175.3837268820161057, 32.78426643622745473 ) ) ;
#16911=CARTESIAN_POINT ( 'NONE',  ( 21.49274850782854074, -175.3837268820161057, -103.5805805771126700 ) ) ;
#16912=LINE ( 'NONE', #15884, #50095 ) ;
#16914=VERTEX_POINT ( 'NONE', #51487 ) ;
#16919=CARTESIAN_POINT ( 'NONE',  ( 74.61260187273137490, -193.5000000000000000, -14.98512977653175682 ) ) ;
#16920=LINE ( 'NONE', #28722, #41327 ) ;
#16921=EDGE_LOOP ( 'NONE', ( #10297, #28074, #32477, #47603 ) ) ;
#16923=CIRCLE ( 'NONE', #32848, 125.0000000000000000 ) ;
#16924=CARTESIAN_POINT ( 'NONE',  ( -48.47912675150885065, -189.7472609257535510, 6.938893903907228378E-15 ) ) ;
#16925=EDGE_LOOP ( 'NONE', ( #8767, #41803, #40760, #48710 ) ) ;
#16926=DIRECTION ( 'NONE',  ( -0.000000000000000000, 1.000000000000000000, -0.000000000000000000 ) ) ;
#16928=FACE_BOUND ( 'NONE', #1380, .T. ) ;
#16929=VECTOR ( 'NONE', #38661, 1000.000000000000000 ) ;
#16930=CARTESIAN_POINT ( 'NONE',  ( 76.01188277843579044, -175.3837268820161057, 11.26891947860284482 ) ) ;
#16932=ADVANCED_FACE ( 'NONE', ( #27294 ), #39379, .T. ) ;
#16933=FACE_OUTER_BOUND ( 'NONE', #30247, .T. ) ;
#16934=EDGE_CURVE ( 'NONE', #34425, #7329, #460, .T. ) ;
#16936=FACE_OUTER_BOUND ( 'NONE', #18759, .T. ) ;
#16937=ADVANCED_FACE ( 'NONE', ( #36468 ), #749, .T. ) ;
#16938=CARTESIAN_POINT ( 'NONE',  ( -172.9701362814535912, -193.5000000000000000, -11.26891947860193177 ) ) ;
#16939=ADVANCED_FACE ( 'NONE', ( #21243 ), #20717, .T. ) ;
#16941=LINE ( 'NONE', #9059, #16083 ) ;
#16943=VERTEX_POINT ( 'NONE', #45176 ) ;
#16944=DIRECTION ( 'NONE',  ( 0.000000000000000000, 0.000000000000000000, 1.000000000000000000 ) ) ;
#16945=DIRECTION ( 'NONE',  ( 0.000000000000000000, 0.000000000000000000, -1.000000000000000000 ) ) ;
#16946=ORIENTED_EDGE ( 'NONE', *, *, #42376, .T. ) ;
#16947=EDGE_CURVE ( 'NONE', #48520, #16369, #8373, .T. ) ;
#16948=AXIS2_PLACEMENT_3D ( 'NONE', #8701, #16326, #24466 ) ;
#16949=ORIENTED_EDGE ( 'NONE', *, *, #8664, .T. ) ;
#16951=EDGE_CURVE ( 'NONE', #43961, #31341, #21489, .T. ) ;
#16952=AXIS2_PLACEMENT_3D ( 'NONE', #27451, #35084, #24031 ) ;
#16953=ADVANCED_FACE ( 'NONE', ( #16527 ), #24156, .T. ) ;
#16956=DIRECTION ( 'NONE',  ( 0.6068001458185890984, 0.000000000000000000, 0.7948544414133565938 ) ) ;
#16957=ORIENTED_EDGE ( 'NONE', *, *, #906, .T. ) ;
#16958=ADVANCED_FACE ( 'NONE', ( #4177 ), #20984, .T. ) ;
#16959=CARTESIAN_POINT ( 'NONE',  ( 5.542374969221969039, -183.6283474603465606, 112.7238987608088223 ) ) ;
#16960=EDGE_LOOP ( 'NONE', ( #23064, #13494, #2183, #2258 ) ) ;
#16961=CARTESIAN_POINT ( 'NONE',  ( 59.80284513346456521, -183.6283474603465606, 62.45009659481583952 ) ) ;
#16962=FACE_OUTER_BOUND ( 'NONE', #335, .T. ) ;
#16963=ADVANCED_FACE ( 'NONE', ( #16008 ), #33054, .T. ) ;
#16965=DIRECTION ( 'NONE',  ( 0.000000000000000000, -1.000000000000000000, 0.000000000000000000 ) ) ;
#16968=ORIENTED_EDGE ( 'NONE', *, *, #24024, .T. ) ;
#16969=ORIENTED_EDGE ( 'NONE', *, *, #11551, .T. ) ;
#16973=CIRCLE ( 'NONE', #27858, 125.0000000000000000 ) ;
#16974=PLANE ( 'NONE',  #767 ) ;
#16976=CARTESIAN_POINT ( 'NONE',  ( -48.93575598890257794, -189.7472609257535510, 0.8896570909947506545 ) ) ;
#16977=VERTEX_POINT ( 'NONE', #28844 ) ;
#16979=ORIENTED_EDGE ( 'NONE', *, *, #33907, .T. ) ;
#16980=LINE ( 'NONE', #49034, #5558 ) ;
#16982=ORIENTED_EDGE ( 'NONE', *, *, #22212, .F. ) ;
#16983=FACE_OUTER_BOUND ( 'NONE', #25589, .T. ) ;
#16984=CARTESIAN_POINT ( 'NONE',  ( -172.7479958471414250, -183.6283474603465606, -13.49993235881364129 ) ) ;
#16985=AXIS2_PLACEMENT_3D ( 'NONE', #7603, #16268, #44118 ) ;
#16986=DIRECTION ( 'NONE',  ( -0.000000000000000000, 1.000000000000000000, -0.000000000000000000 ) ) ;
#16988=ORIENTED_EDGE ( 'NONE', *, *, #6736, .T. ) ;
#16989=CARTESIAN_POINT ( 'NONE',  ( -172.0839188101925004, -193.5000000000000000, -18.62405380494756812 ) ) ;
#16990=ORIENTED_EDGE ( 'NONE', *, *, #49795, .F. ) ;
#16991=AXIS2_PLACEMENT_3D ( 'NONE', #7879, #20233, #39168 ) ;
#16992=EDGE_CURVE ( 'NONE', #9008, #1918, #44897, .T. ) ;
#16993=EDGE_LOOP ( 'NONE', ( #29890, #13700, #1705, #41413 ) ) ;
#16994=DIRECTION ( 'NONE',  ( -0.6300878435817203194, 0.000000000000000000, 0.7765238627180349740 ) ) ;
#16997=EDGE_CURVE ( 'NONE', #21200, #43863, #24827, .T. ) ;
#17000=DIRECTION ( 'NONE',  ( 0.000000000000000000, -1.000000000000000000, -0.000000000000000000 ) ) ;
#17001=CARTESIAN_POINT ( 'NONE',  ( 9.336583202542589888, -193.5000000000000000, 110.8257356506556306 ) ) ;
#17005=FACE_OUTER_BOUND ( 'NONE', #45565, .T. ) ;
#17006=AXIS2_PLACEMENT_3D ( 'NONE', #11579, #31025, #27604 ) ;
#17007=EDGE_CURVE ( 'NONE', #11775, #19173, #24396, .T. ) ;
#17008=DIRECTION ( 'NONE',  ( 0.000000000000000000, 1.000000000000000000, 0.000000000000000000 ) ) ;
#17009=FACE_BOUND ( 'NONE', #4870, .T. ) ;
#17011=VECTOR ( 'NONE', #45127, 1000.000000000000000 ) ;
#17012=VECTOR ( 'NONE', #14040, 1000.000000000000000 ) ;
#17014=LINE ( 'NONE', #33021, #15554 ) ;
#17015=ORIENTED_EDGE ( 'NONE', *, *, #18589, .T. ) ;
#17016=DIRECTION ( 'NONE',  ( 0.000000000000000000, -1.000000000000000000, 0.000000000000000000 ) ) ;
#17021=EDGE_CURVE ( 'NONE', #5202, #32592, #51130, .T. ) ;
#17023=EDGE_CURVE ( 'NONE', #23880, #1605, #6457, .T. ) ;
#17024=FACE_OUTER_BOUND ( 'NONE', #26952, .T. ) ;
#17025=DIRECTION ( 'NONE',  ( 0.8858462335218260097, -0.000000000000000000, -0.4639789333096864810 ) ) ;
#17027=AXIS2_PLACEMENT_3D ( 'NONE', #50097, #30106, #42443 ) ;
#17028=EDGE_CURVE ( 'NONE', #10986, #8881, #34295, .T. ) ;
#17029=CARTESIAN_POINT ( 'NONE',  ( -171.7589556598192644, -193.5000000000000000, -13.35228579481115574 ) ) ;
#17030=ORIENTED_EDGE ( 'NONE', *, *, #5067, .F. ) ;
#17031=EDGE_LOOP ( 'NONE', ( #1273, #23457, #36275, #8007 ) ) ;
#17034=ORIENTED_EDGE ( 'NONE', *, *, #29928, .F. ) ;
#17041=AXIS2_PLACEMENT_3D ( 'NONE', #34694, #11803, #11285 ) ;
#17042=VECTOR ( 'NONE', #38846, 1000.000000000000000 ) ;
#17044=LINE ( 'NONE', #24916, #25894 ) ;
#17045=DIRECTION ( 'NONE',  ( -0.000000000000000000, 1.000000000000000000, -0.000000000000000000 ) ) ;
#17046=ORIENTED_EDGE ( 'NONE', *, *, #41754, .T. ) ;
#17047=CARTESIAN_POINT ( 'NONE',  ( -74.33510315702947935, -193.5000000000000000, -121.2748789083718606 ) ) ;
#17050=AXIS2_PLACEMENT_3D ( 'NONE', #27980, #51927, #24047 ) ;
#17056=ORIENTED_EDGE ( 'NONE', *, *, #29075, .F. ) ;
#17057=LINE ( 'NONE', #49108, #49834 ) ;
#17062=ORIENTED_EDGE ( 'NONE', *, *, #44831, .F. ) ;
#17063=VERTEX_POINT ( 'NONE', #30873 ) ;
#17065=DIRECTION ( 'NONE',  ( 0.000000000000000000, 0.000000000000000000, 1.000000000000000000 ) ) ;
#17066=DIRECTION ( 'NONE',  ( -0.000000000000000000, 1.000000000000000000, 0.000000000000000000 ) ) ;
#17067=FACE_OUTER_BOUND ( 'NONE', #954, .T. ) ;
#17068=VERTEX_POINT ( 'NONE', #14860 ) ;
#17070=DIRECTION ( 'NONE',  ( 0.000000000000000000, 0.000000000000000000, -1.000000000000000000 ) ) ;
#17075=CARTESIAN_POINT ( 'NONE',  ( -166.8403286750647680, -193.5000000000000000, -40.19484891389966918 ) ) ;
#17078=AXIS2_PLACEMENT_3D ( 'NONE', #23979, #39489, #43953 ) ;
#17080=EDGE_LOOP ( 'NONE', ( #33834, #36318, #42024, #48546 ) ) ;
#17081=LINE ( 'NONE', #13121, #37835 ) ;
#17083=EDGE_LOOP ( 'NONE', ( #51061, #43074, #34220, #37708 ) ) ;
#17088=AXIS2_PLACEMENT_3D ( 'NONE', #32886, #36575, #44732 ) ;
#17089=CARTESIAN_POINT ( 'NONE',  ( -150.5215542367829471, -193.5000000000000000, -72.19655804061974891 ) ) ;
#17090=EDGE_CURVE ( 'NONE', #25917, #41928, #26918, .T. ) ;
#17091=DIRECTION ( 'NONE',  ( 0.000000000000000000, 0.000000000000000000, 1.000000000000000000 ) ) ;
#17092=CARTESIAN_POINT ( 'NONE',  ( -34.51936650669026818, -175.3837268820161057, -124.2180546213278234 ) ) ;
#17095=CIRCLE ( 'NONE', #1118, 124.9999999999999858 ) ;
#17096=DIRECTION ( 'NONE',  ( 0.000000000000000000, 1.000000000000000000, 0.000000000000000000 ) ) ;
#17099=CARTESIAN_POINT ( 'NONE',  ( 12.99855592850622443, -183.6283474603465606, 108.8370090194294875 ) ) ;
#17101=DIRECTION ( 'NONE',  ( 0.000000000000000000, -1.000000000000000000, 0.000000000000000000 ) ) ;
#17102=VERTEX_POINT ( 'NONE', #50279 ) ;
#17103=FACE_OUTER_BOUND ( 'NONE', #6822, .T. ) ;
#17104=CIRCLE ( 'NONE', #27992, 125.0000000000000000 ) ;
#17105=VECTOR ( 'NONE', #36854, 999.9999999999998863 ) ;
#17106=LINE ( 'NONE', #29424, #22533 ) ;
#17109=DIRECTION ( 'NONE',  ( 0.000000000000000000, 0.000000000000000000, -1.000000000000000000 ) ) ;
#17112=ORIENTED_EDGE ( 'NONE', *, *, #49159, .T. ) ;
#17113=DIRECTION ( 'NONE',  ( -0.000000000000000000, 1.000000000000000000, -0.000000000000000000 ) ) ;
#17120=ORIENTED_EDGE ( 'NONE', *, *, #7892, .F. ) ;
#17121=DIRECTION ( 'NONE',  ( -0.000000000000000000, 1.000000000000000000, -0.000000000000000000 ) ) ;
#17123=DIRECTION ( 'NONE',  ( 0.000000000000000000, -0.000000000000000000, 1.000000000000000000 ) ) ;
#17125=CARTESIAN_POINT ( 'NONE',  ( -51.89154260666841623, -183.6283474603465606, 124.9534129907280970 ) ) ;
#17126=DIRECTION ( 'NONE',  ( -0.000000000000000000, -1.000000000000000000, 0.000000000000000000 ) ) ;
#17129=ADVANCED_FACE ( 'NONE', ( #22409 ), #43142, .T. ) ;
#17130=CARTESIAN_POINT ( 'NONE',  ( -172.0839188101924719, -189.7472609257535510, -18.62405380494754681 ) ) ;
#17132=DIRECTION ( 'NONE',  ( 0.000000000000000000, -1.000000000000000000, 0.000000000000000000 ) ) ;
#17133=ORIENTED_EDGE ( 'NONE', *, *, #10514, .T. ) ;
#17135=PLANE ( 'NONE',  #42890 ) ;
#17136=VECTOR ( 'NONE', #27586, 1000.000000000000000 ) ;
#17137=PLANE ( 'NONE',  #21871 ) ;
#17138=PLANE ( 'NONE',  #41724 ) ;
#17139=AXIS2_PLACEMENT_3D ( 'NONE', #21453, #17530, #36962 ) ;
#17140=PLANE ( 'NONE',  #15391 ) ;
#17141=DIRECTION ( 'NONE',  ( 0.000000000000000000, 0.000000000000000000, 1.000000000000000000 ) ) ;
#17144=CARTESIAN_POINT ( 'NONE',  ( 52.98246549829696761, -189.7472609257535510, 73.01058346660535392 ) ) ;
#17146=EDGE_LOOP ( 'NONE', ( #41694, #2385, #23378, #51127 ) ) ;
#17147=CARTESIAN_POINT ( 'NONE',  ( -153.2421220336517251, -189.7472609257535510, -66.33788548805453900 ) ) ;
#17148=CIRCLE ( 'NONE', #14598, 125.0000000000000000 ) ;
#17150=CARTESIAN_POINT ( 'NONE',  ( -75.31296732259116311, -177.1207230881787780, -121.0625654437172614 ) ) ;
#17151=VERTEX_POINT ( 'NONE', #23945 ) ;
#17152=ORIENTED_EDGE ( 'NONE', *, *, #22179, .T. ) ;
#17153=ORIENTED_EDGE ( 'NONE', *, *, #48831, .F. ) ;
#17154=PLANE ( 'NONE',  #34267 ) ;
#17156=CARTESIAN_POINT ( 'NONE',  ( -170.9669310976187830, -175.3837268820161057, -24.93467037017131105 ) ) ;
#17157=VERTEX_POINT ( 'NONE', #19739 ) ;
#17158=FACE_OUTER_BOUND ( 'NONE', #1195, .T. ) ;
#17159=DIRECTION ( 'NONE',  ( 0.000000000000000000, 0.000000000000000000, 1.000000000000000000 ) ) ;
#17160=ORIENTED_EDGE ( 'NONE', *, *, #16170, .F. ) ;
#17161=DIRECTION ( 'NONE',  ( 0.000000000000000000, 0.000000000000000000, 1.000000000000000000 ) ) ;
#17162=VECTOR ( 'NONE', #15881, 1000.000000000000114 ) ;
#17163=ORIENTED_EDGE ( 'NONE', *, *, #46193, .F. ) ;
#17165=VERTEX_POINT ( 'NONE', #39451 ) ;
#17167=EDGE_CURVE ( 'NONE', #29891, #44801, #47626, .T. ) ;
#17168=CARTESIAN_POINT ( 'NONE',  ( -164.6073096293132494, -193.5000000000000000, 43.47841891815210147 ) ) ;
#17169=CARTESIAN_POINT ( 'NONE',  ( -48.47912675150885065, -189.7472609257535510, 6.938893903907228378E-15 ) ) ;
#17170=FACE_OUTER_BOUND ( 'NONE', #13506, .T. ) ;
#17171=VECTOR ( 'NONE', #9561, 1000.000000000000000 ) ;
#17173=ORIENTED_EDGE ( 'NONE', *, *, #17253, .T. ) ;
#17174=ORIENTED_EDGE ( 'NONE', *, *, #7668, .F. ) ;
#17175=LINE ( 'NONE', #5094, #34846 ) ;
#17176=CARTESIAN_POINT ( 'NONE',  ( -155.0851258170080769, -177.1207230881787780, 63.33473559879987391 ) ) ;
#17177=ORIENTED_EDGE ( 'NONE', *, *, #23912, .T. ) ;
#17178=CARTESIAN_POINT ( 'NONE',  ( -145.4373324222574126, -175.3837268820161057, -78.89300572996837957 ) ) ;
#17179=LINE ( 'NONE', #12694, #22883 ) ;
#17182=DIRECTION ( 'NONE',  ( -0.000000000000000000, 1.000000000000000000, 0.000000000000000000 ) ) ;
#17183=VECTOR ( 'NONE', #48775, 1000.000000000000000 ) ;
#17184=ADVANCED_FACE ( 'NONE', ( #39205 ), #15830, .F. ) ;
#17187=ORIENTED_EDGE ( 'NONE', *, *, #6971, .F. ) ;
#17189=ORIENTED_EDGE ( 'NONE', *, *, #49158, .F. ) ;
#17192=CARTESIAN_POINT ( 'NONE',  ( -48.47912675150885065, -175.3837268820161057, 6.938893903907228378E-15 ) ) ;
#17193=ORIENTED_EDGE ( 'NONE', *, *, #9226, .T. ) ;
#17195=DIRECTION ( 'NONE',  ( 0.000000000000000000, -1.000000000000000000, 0.000000000000000000 ) ) ;
#17196=DIRECTION ( 'NONE',  ( 0.000000000000000000, -1.000000000000000000, 0.000000000000000000 ) ) ;
#17198=ORIENTED_EDGE ( 'NONE', *, *, #39121, .T. ) ;
#17199=DIRECTION ( 'NONE',  ( 0.2348860457809775482, 0.000000000000000000, 0.9720229140804121926 ) ) ;
#17200=ORIENTED_EDGE ( 'NONE', *, *, #8864, .F. ) ;
#17201=ORIENTED_EDGE ( 'NONE', *, *, #22086, .T. ) ;
#17202=EDGE_CURVE ( 'NONE', #23608, #47014, #18116, .T. ) ;
#17203=CARTESIAN_POINT ( 'NONE',  ( 61.38599058177057799, -189.7472609257535510, 59.62093586438192006 ) ) ;
#17204=DIRECTION ( 'NONE',  ( 0.000000000000000000, 0.000000000000000000, 1.000000000000000000 ) ) ;
#17206=CIRCLE ( 'NONE', #26412, 15.00000000000000000 ) ;
#17207=AXIS2_PLACEMENT_3D ( 'NONE', #15854, #39989, #39723 ) ;
#17208=ORIENTED_EDGE ( 'NONE', *, *, #16071, .F. ) ;
#17212=CARTESIAN_POINT ( 'NONE',  ( 33.25242634436025213, -189.7472609257535510, -94.57776286494160445 ) ) ;
#17214=DIRECTION ( 'NONE',  ( 0.4031234292879665171, 0.000000000000000000, 0.9151456172430210145 ) ) ;
#17215=AXIS2_PLACEMENT_3D ( 'NONE', #25693, #13868, #21494 ) ;
#17217=DIRECTION ( 'NONE',  ( -0.000000000000000000, 1.000000000000000000, -0.000000000000000000 ) ) ;
#17218=DIRECTION ( 'NONE',  ( -0.9027978299657387629, 0.000000000000000000, -0.4300652022765304450 ) ) ;
#17219=VECTOR ( 'NONE', #18254, 1000.000000000000000 ) ;
#17220=FACE_OUTER_BOUND ( 'NONE', #22074, .T. ) ;
#17221=CIRCLE ( 'NONE', #32278, 125.0000000000000000 ) ;
#17223=ORIENTED_EDGE ( 'NONE', *, *, #36956, .T. ) ;
#17224=ORIENTED_EDGE ( 'NONE', *, *, #22852, .F. ) ;
#17225=ORIENTED_EDGE ( 'NONE', *, *, #47788, .F. ) ;
#17226=CARTESIAN_POINT ( 'NONE',  ( 28.02885774092382221, -189.7472609257535510, 98.85104101073332572 ) ) ;
#17227=DIRECTION ( 'NONE',  ( 0.000000000000000000, 0.000000000000000000, 1.000000000000000000 ) ) ;
#17229=DIRECTION ( 'NONE',  ( 0.000000000000000000, -0.000000000000000000, -1.000000000000000000 ) ) ;
#17230=ORIENTED_EDGE ( 'NONE', *, *, #30765, .T. ) ;
#17231=EDGE_CURVE ( 'NONE', #25859, #38149, #36290, .T. ) ;
#17232=EDGE_CURVE ( 'NONE', #4651, #23372, #15298, .T. ) ;
#17234=DIRECTION ( 'NONE',  ( 0.000000000000000000, 0.000000000000000000, -1.000000000000000000 ) ) ;
#17235=EDGE_LOOP ( 'NONE', ( #31305, #6523, #44038, #30955 ) ) ;
#17239=DIRECTION ( 'NONE',  ( 0.000000000000000000, 1.000000000000000000, -0.000000000000000000 ) ) ;
#17240=AXIS2_PLACEMENT_3D ( 'NONE', #22603, #50984, #18903 ) ;
#17241=VECTOR ( 'NONE', #23461, 1000.000000000000000 ) ;
#17242=DIRECTION ( 'NONE',  ( -0.000000000000000000, 1.000000000000000000, -0.000000000000000000 ) ) ;
#17247=DIRECTION ( 'NONE',  ( 0.000000000000000000, 0.000000000000000000, -1.000000000000000000 ) ) ;
#17248=VERTEX_POINT ( 'NONE', #44186 ) ;
#17251=VERTEX_POINT ( 'NONE', #4243 ) ;
#17253=EDGE_CURVE ( 'NONE', #48345, #32062, #20263, .T. ) ;
#17254=AXIS2_PLACEMENT_3D ( 'NONE', #17757, #21947, #32984 ) ;
#17255=DIRECTION ( 'NONE',  ( 0.000000000000000000, -0.000000000000000000, 1.000000000000000000 ) ) ;
#17257=AXIS2_PLACEMENT_3D ( 'NONE', #50448, #29939, #45999 ) ;
#17260=DIRECTION ( 'NONE',  ( 0.000000000000000000, 0.000000000000000000, 1.000000000000000000 ) ) ;
#17261=FACE_OUTER_BOUND ( 'NONE', #8525, .T. ) ;
#17262=CIRCLE ( 'NONE', #47453, 124.9999999999999858 ) ;
#17263=DIRECTION ( 'NONE',  ( 0.000000000000000000, 0.000000000000000000, -1.000000000000000000 ) ) ;
#17266=VECTOR ( 'NONE', #32263, 1000.000000000000000 ) ;
#17268=EDGE_LOOP ( 'NONE', ( #51582, #19668, #18867, #43535 ) ) ;
#17270=VERTEX_POINT ( 'NONE', #11852 ) ;
#17272=ORIENTED_EDGE ( 'NONE', *, *, #15396, .T. ) ;
#17273=FACE_OUTER_BOUND ( 'NONE', #27730, .T. ) ;
#17274=ORIENTED_EDGE ( 'NONE', *, *, #10555, .F. ) ;
#17275=CARTESIAN_POINT ( 'NONE',  ( -53.47502265695599277, -177.1207230881787780, -123.9001241957025883 ) ) ;
#17276=AXIS2_PLACEMENT_3D ( 'NONE', #3667, #37556, #1550 ) ;
#17280=AXIS2_PLACEMENT_3D ( 'NONE', #7428, #35007, #27109 ) ;
#17281=VECTOR ( 'NONE', #38447, 1000.000000000000000 ) ;
#17282=DIRECTION ( 'NONE',  ( 0.000000000000000000, 0.000000000000000000, 1.000000000000000000 ) ) ;
#17283=EDGE_LOOP ( 'NONE', ( #32210, #13014, #5152, #31773 ) ) ;
#17285=EDGE_LOOP ( 'NONE', ( #50865, #15632, #6986, #50957 ) ) ;
#17286=EDGE_CURVE ( 'NONE', #19435, #44506, #43917, .T. ) ;
#17287=FACE_OUTER_BOUND ( 'NONE', #16308, .T. ) ;
#17288=CARTESIAN_POINT ( 'NONE',  ( -158.1873290247468447, -177.1207230881787780, 57.79541595648306185 ) ) ;
#17290=CIRCLE ( 'NONE', #4674, 125.0000000000000000 ) ;
#17292=VECTOR ( 'NONE', #19824, 1000.000000000000000 ) ;
#17293=CARTESIAN_POINT ( 'NONE',  ( 26.70958190211000982, -189.7472609257535510, -99.85818990449013199 ) ) ;
#17294=DIRECTION ( 'NONE',  ( 0.000000000000000000, -0.000000000000000000, -1.000000000000000000 ) ) ;
#17296=EDGE_CURVE ( 'NONE', #20535, #23501, #36039, .T. ) ;
#17297=EDGE_CURVE ( 'NONE', #39416, #37656, #46668, .T. ) ;
#17298=ADVANCED_FACE ( 'NONE', ( #48918 ), #24732, .T. ) ;
#17299=VECTOR ( 'NONE', #6955, 1000.000000000000114 ) ;
#17300=EDGE_CURVE ( 'NONE', #5586, #12962, #4767, .T. ) ;
#17301=VECTOR ( 'NONE', #26416, 999.9999999999998863 ) ;
#17302=FACE_OUTER_BOUND ( 'NONE', #39612, .T. ) ;
#17303=DIRECTION ( 'NONE',  ( -0.9151456172430237901, 0.000000000000000000, 0.4031234292879600778 ) ) ;
#17304=ORIENTED_EDGE ( 'NONE', *, *, #20244, .F. ) ;
#17305=CARTESIAN_POINT ( 'NONE',  ( -137.9639882952644143, -193.5000000000000000, 87.27805883780241913 ) ) ;
#17307=ORIENTED_EDGE ( 'NONE', *, *, #6478, .T. ) ;
#17309=EDGE_CURVE ( 'NONE', #20792, #34352, #25508, .T. ) ;
#17310=ORIENTED_EDGE ( 'NONE', *, *, #7257, .T. ) ;
#17312=VERTEX_POINT ( 'NONE', #9233 ) ;
#17313=DIRECTION ( 'NONE',  ( 0.000000000000000000, -1.000000000000000000, 0.000000000000000000 ) ) ;
#17314=PLANE ( 'NONE',  #37628 ) ;
#17316=ADVANCED_FACE ( 'NONE', ( #44709 ), #40484, .F. ) ;
#17317=CARTESIAN_POINT ( 'NONE',  ( -156.7610986364826999, -183.6283474603465606, -62.45009659481510766 ) ) ;
#17319=EDGE_CURVE ( 'NONE', #7465, #1427, #20520, .T. ) ;
#17320=ORIENTED_EDGE ( 'NONE', *, *, #7257, .F. ) ;
#17321=DIRECTION ( 'NONE',  ( 0.000000000000000000, 0.000000000000000000, 1.000000000000000000 ) ) ;
#17324=AXIS2_PLACEMENT_3D ( 'NONE', #16477, #12767, #28795 ) ;
#17327=CARTESIAN_POINT ( 'NONE',  ( -166.1003692892502102, -177.1207230881787780, -42.31126686685033889 ) ) ;
#17328=EDGE_LOOP ( 'NONE', ( #21348, #18535, #46165, #15180 ) ) ;
#17330=CARTESIAN_POINT ( 'NONE',  ( -47.82630463331832971, -175.3837268820161057, -0.7575112421616121416 ) ) ;
#17331=VECTOR ( 'NONE', #44, 1000.000000000000227 ) ;
#17332=ADVANCED_FACE ( 'NONE', ( #28917 ), #37605, .T. ) ;
#17336=CARTESIAN_POINT ( 'NONE',  ( -142.3192003680973130, -183.6283474603465606, 82.57748230379306165 ) ) ;
#17337=CARTESIAN_POINT ( 'NONE',  ( -49.42645310536304493, -183.6283474603465606, 0.3202698538628349079 ) ) ;
#17340=DIRECTION ( 'NONE',  ( -0.000000000000000000, 1.000000000000000000, -0.000000000000000000 ) ) ;
#17344=VECTOR ( 'NONE', #33595, 1000.000000000000114 ) ;
#17345=CARTESIAN_POINT ( 'NONE',  ( -11.17913199888832487, -175.3837268820161057, 119.3051146910914468 ) ) ;
#17346=DIRECTION ( 'NONE',  ( 0.000000000000000000, -0.000000000000000000, 1.000000000000000000 ) ) ;
#17348=CARTESIAN_POINT ( 'NONE',  ( -47.47956591500005885, -189.7472609257535510, -0.02963332782254939762 ) ) ;
#17349=CIRCLE ( 'NONE', #1378, 125.0000000000000000 ) ;
#17350=VERTEX_POINT ( 'NONE', #49176 ) ;
#17352=AXIS2_PLACEMENT_3D ( 'NONE', #32614, #16601, #8695 ) ;
#17353=LINE ( 'NONE', #30200, #21733 ) ;
#17358=CARTESIAN_POINT ( 'NONE',  ( 26.70958190211001337, -193.5000000000000000, -99.85818990449013199 ) ) ;
#17359=DIRECTION ( 'NONE',  ( -0.9266896074318291543, 0.000000000000000000, -0.3758275821142488260 ) ) ;
#17361=CARTESIAN_POINT ( 'NONE',  ( 69.14211578623219623, -183.6283474603465606, 42.31126686685117022 ) ) ;
#17362=VERTEX_POINT ( 'NONE', #44452 ) ;
#17365=VECTOR ( 'NONE', #2193, 1000.000000000000000 ) ;
#17367=PLANE ( 'NONE',  #10004 ) ;
#17368=VECTOR ( 'NONE', #7277, 1000.000000000000000 ) ;
#17370=EDGE_LOOP ( 'NONE', ( #4569, #36396, #3898, #29179 ) ) ;
#17372=ADVANCED_FACE ( 'NONE', ( #29191 ), #37069, .T. ) ;
#17373=EDGE_CURVE ( 'NONE', #8813, #40221, #5554, .T. ) ;
#17375=EDGE_LOOP ( 'NONE', ( #43409, #22465, #1645, #36516 ) ) ;
#17376=FACE_OUTER_BOUND ( 'NONE', #23919, .T. ) ;
#17377=DIRECTION ( 'NONE',  ( 0.000000000000000000, 0.000000000000000000, 1.000000000000000000 ) ) ;
#17378=VERTEX_POINT ( 'NONE', #5296 ) ;
#17379=CIRCLE ( 'NONE', #19051, 125.0000000000000000 ) ;
#17380=AXIS2_PLACEMENT_3D ( 'NONE', #49232, #9287, #33957 ) ;
#17382=VECTOR ( 'NONE', #21653, 1000.000000000000000 ) ;
#17383=ORIENTED_EDGE ( 'NONE', *, *, #29858, .F. ) ;
#17384=DIRECTION ( 'NONE',  ( 0.000000000000000000, 0.000000000000000000, -1.000000000000000000 ) ) ;
#17387=DIRECTION ( 'NONE',  ( 0.000000000000000000, 0.000000000000000000, -1.000000000000000000 ) ) ;
#17388=DIRECTION ( 'NONE',  ( 0.000000000000000000, 0.000000000000000000, 1.000000000000000000 ) ) ;
#17389=ORIENTED_EDGE ( 'NONE', *, *, #35627, .F. ) ;
#17390=EDGE_LOOP ( 'NONE', ( #40555, #1984, #47194, #2697 ) ) ;
#17392=CARTESIAN_POINT ( 'NONE',  ( -169.9131040279660283, -193.5000000000000000, 29.64437826672835996 ) ) ;
#17393=DIRECTION ( 'NONE',  ( -0.000000000000000000, 1.000000000000000000, -0.000000000000000000 ) ) ;
#17398=FACE_OUTER_BOUND ( 'NONE', #18281, .T. ) ;
#17399=LINE ( 'NONE', #7988, #24300 ) ;
#17400=LINE ( 'NONE', #41533, #21559 ) ;
#17401=ORIENTED_EDGE ( 'NONE', *, *, #19487, .T. ) ;
#17404=EDGE_CURVE ( 'NONE', #49012, #37757, #14214, .T. ) ;
#17405=CARTESIAN_POINT ( 'NONE',  ( 70.98542830588607444, -193.5000000000000000, -36.78613984829961936 ) ) ;
#17406=VERTEX_POINT ( 'NONE', #2624 ) ;
#17407=VECTOR ( 'NONE', #48783, 1000.000000000000114 ) ;
#17409=DIRECTION ( 'NONE',  ( -0.000000000000000000, 1.000000000000000000, -0.000000000000000000 ) ) ;
#17410=CARTESIAN_POINT ( 'NONE',  ( -164.8312043469690593, -183.6283474603465606, -42.87565520599201818 ) ) ;
#17411=VECTOR ( 'NONE', #45779, 1000.000000000000114 ) ;
#17412=CARTESIAN_POINT ( 'NONE',  ( -36.09284319799462537, -183.6283474603465606, 124.3848060646152618 ) ) ;
#17413=DIRECTION ( 'NONE',  ( -0.9027978299657416494, 0.000000000000000000, -0.4300652022765245608 ) ) ;
#17414=CARTESIAN_POINT ( 'NONE',  ( -139.4082623311986993, -193.5000000000000000, 84.30834960113001841 ) ) ;
#17418=CARTESIAN_POINT ( 'NONE',  ( -84.82349129030166068, -175.3837268820161057, -119.5996955107802222 ) ) ;
#17419=DIRECTION ( 'NONE',  ( 0.000000000000000000, 1.000000000000000000, -0.000000000000000000 ) ) ;
#17420=VERTEX_POINT ( 'NONE', #41805 ) ;
#17421=VECTOR ( 'NONE', #17762, 1000.000000000000341 ) ;
#17423=DIRECTION ( 'NONE',  ( 0.4031234292879792847, 0.000000000000000000, -0.9151456172430153524 ) ) ;
#17424=VECTOR ( 'NONE', #36077, 1000.000000000000114 ) ;
#17425=VECTOR ( 'NONE', #22656, 1000.000000000000000 ) ;
#17427=DIRECTION ( 'NONE',  ( 0.000000000000000000, 1.000000000000000000, 0.000000000000000000 ) ) ;
#17428=VERTEX_POINT ( 'NONE', #18411 ) ;
#17429=VERTEX_POINT ( 'NONE', #14468 ) ;
#17430=ORIENTED_EDGE ( 'NONE', *, *, #50380, .F. ) ;
#17432=ADVANCED_FACE ( 'NONE', ( #34677 ), #46787, .F. ) ;
#17433=CARTESIAN_POINT ( 'NONE',  ( 59.00260725618641544, -183.6283474603465606, -63.81752780152991278 ) ) ;
#17434=DIRECTION ( 'NONE',  ( 0.000000000000000000, 0.000000000000000000, 1.000000000000000000 ) ) ;
#17436=LINE ( 'NONE', #33457, #21839 ) ;
#17439=VERTEX_POINT ( 'NONE', #5826 ) ;
#17440=CIRCLE ( 'NONE', #33368, 125.0000000000000000 ) ;
#17441=CARTESIAN_POINT ( 'NONE',  ( 27.50603775690335695, -175.3837268820161057, -99.25348746834811209 ) ) ;
#17442=VERTEX_POINT ( 'NONE', #29972 ) ;
#17444=CIRCLE ( 'NONE', #5700, 125.0000000000000000 ) ;
#17445=VERTEX_POINT ( 'NONE', #38369 ) ;
#17446=DIRECTION ( 'NONE',  ( 0.000000000000000000, 1.000000000000000000, 0.000000000000000000 ) ) ;
#17447=LINE ( 'NONE', #41324, #48997 ) ;
#17448=CARTESIAN_POINT ( 'NONE',  ( -123.8574911141017623, -189.7472609257535510, 98.45863302693528851 ) ) ;
#17449=EDGE_LOOP ( 'NONE', ( #37952, #16853, #25170, #39428 ) ) ;
#17450=VECTOR ( 'NONE', #3313, 1000.000000000000000 ) ;
#17452=CARTESIAN_POINT ( 'NONE',  ( -37.67038537088846084, -177.1207230881787780, -124.5318076226586612 ) ) ;
#17455=VERTEX_POINT ( 'NONE', #18664 ) ;
#17456=ADVANCED_FACE ( 'NONE', ( #50727 ), #45747, .F. ) ;
#17457=DIRECTION ( 'NONE',  ( 0.000000000000000000, 0.000000000000000000, 1.000000000000000000 ) ) ;
#17458=AXIS2_PLACEMENT_3D ( 'NONE', #48385, #12370, #28397 ) ;
#17459=ORIENTED_EDGE ( 'NONE', *, *, #9874, .T. ) ;
#17461=PLANE ( 'NONE',  #11320 ) ;
#17462=EDGE_CURVE ( 'NONE', #41184, #16398, #18147, .T. ) ;
#17463=AXIS2_PLACEMENT_3D ( 'NONE', #2866, #13930, #38085 ) ;
#17465=LINE ( 'NONE', #8252, #532 ) ;
#17466=ORIENTED_EDGE ( 'NONE', *, *, #40559, .T. ) ;
#17467=LINE ( 'NONE', #49523, #45558 ) ;
#17470=CARTESIAN_POINT ( 'NONE',  ( -15.48416040178638831, -177.1207230881787780, 119.5301634136914970 ) ) ;
#17472=DIRECTION ( 'NONE',  ( -0.000000000000000000, 1.000000000000000000, -0.000000000000000000 ) ) ;
#17473=EDGE_CURVE ( 'NONE', #16711, #33847, #33904, .T. ) ;
#17474=DIRECTION ( 'NONE',  ( 0.4566292373937077542, 0.000000000000000000, 0.8896570909947499883 ) ) ;
#17477=ORIENTED_EDGE ( 'NONE', *, *, #10714, .F. ) ;
#17478=ORIENTED_EDGE ( 'NONE', *, *, #17550, .T. ) ;
#17479=VECTOR ( 'NONE', #9098, 1000.000000000000000 ) ;
#17481=LINE ( 'NONE', #29283, #24332 ) ;
#17482=FACE_OUTER_BOUND ( 'NONE', #21959, .T. ) ;
#17484=AXIS2_PLACEMENT_3D ( 'NONE', #20560, #44487, #20049 ) ;
#17485=VERTEX_POINT ( 'NONE', #50219 ) ;
#17487=ADVANCED_FACE ( 'NONE', ( #42051 ), #26274, .T. ) ;
#17492=EDGE_LOOP ( 'NONE', ( #1464, #36600, #18939, #47511 ) ) ;
#17495=EDGE_CURVE ( 'NONE', #32338, #26523, #4726, .T. ) ;
#17496=DIRECTION ( 'NONE',  ( 0.000000000000000000, -1.000000000000000000, -0.000000000000000000 ) ) ;
#17497=CARTESIAN_POINT ( 'NONE',  ( -15.81236726369125023, -177.1207230881787780, -120.6560517527615417 ) ) ;
#17499=VERTEX_POINT ( 'NONE', #22859 ) ;
#17500=ORIENTED_EDGE ( 'NONE', *, *, #2230, .T. ) ;
#17502=CARTESIAN_POINT ( 'NONE',  ( 27.23560471289044571, -175.3837268820161057, 99.45993886622845537 ) ) ;
#17505=DIRECTION ( 'NONE',  ( 0.000000000000000000, 0.000000000000000000, -1.000000000000000000 ) ) ;
#17506=LINE ( 'NONE', #16728, #17183 ) ;
#17508=EDGE_LOOP ( 'NONE', ( #9320, #39508, #5858, #17015 ) ) ;
#17510=ORIENTED_EDGE ( 'NONE', *, *, #43523, .F. ) ;
#17511=VECTOR ( 'NONE', #49513, 1000.000000000000000 ) ;
#17512=ORIENTED_EDGE ( 'NONE', *, *, #15568, .F. ) ;
#17514=DIRECTION ( 'NONE',  ( 0.1182731709213523247, 0.000000000000000000, 0.9929810960135185827 ) ) ;
#17515=AXIS2_PLACEMENT_3D ( 'NONE', #28903, #33886, #9724 ) ;
#17518=CIRCLE ( 'NONE', #46888, 125.0000000000000000 ) ;
#17520=CARTESIAN_POINT ( 'NONE',  ( -101.0675409952199999, -177.1207230881787780, 113.3995532942341100 ) ) ;
#17522=LINE ( 'NONE', #37729, #30886 ) ;
#17524=CARTESIAN_POINT ( 'NONE',  ( 76.48781641346532467, -189.7472609257535510, 2.874563619424060246 ) ) ;
#17525=AXIS2_PLACEMENT_3D ( 'NONE', #24635, #24383, #40387 ) ;
#17527=CARTESIAN_POINT ( 'NONE',  ( -49.47517659412407198, -193.5000000000000000, 0.08879589532293177823 ) ) ;
#17529=CARTESIAN_POINT ( 'NONE',  ( -33.52607327456454556, -193.5000000000000000, -124.1024020384603119 ) ) ;
#17530=DIRECTION ( 'NONE',  ( 0.000000000000000000, 1.000000000000000000, 0.000000000000000000 ) ) ;
#17532=CARTESIAN_POINT ( 'NONE',  ( -48.47912675150885065, -175.3837268820161057, 6.938893903907228378E-15 ) ) ;
#17533=VECTOR ( 'NONE', #10250, 1000.000000000000000 ) ;
#17535=FACE_BOUND ( 'NONE', #32838, .T. ) ;
#17536=ORIENTED_EDGE ( 'NONE', *, *, #18432, .F. ) ;
#17537=DIRECTION ( 'NONE',  ( 0.000000000000000000, 0.000000000000000000, 1.000000000000000000 ) ) ;
#17538=ORIENTED_EDGE ( 'NONE', *, *, #43998, .T. ) ;
#17539=EDGE_CURVE ( 'NONE', #34512, #37437, #10501, .T. ) ;
#17541=EDGE_CURVE ( 'NONE', #38180, #13416, #14830, .T. ) ;
#17542=CARTESIAN_POINT ( 'NONE',  ( -82.67254833784559764, -183.6283474603465606, -120.2323164553483963 ) ) ;
#17543=VERTEX_POINT ( 'NONE', #26534 ) ;
#17545=AXIS2_PLACEMENT_3D ( 'NONE', #24473, #40492, #35516 ) ;
#17546=CARTESIAN_POINT ( 'NONE',  ( 75.48825557695654709, -189.7472609257535510, 2.844930291601486694 ) ) ;
#17548=ORIENTED_EDGE ( 'NONE', *, *, #25840, .F. ) ;
#17549=AXIS2_PLACEMENT_3D ( 'NONE', #27284, #15476, #48043 ) ;
#17550=EDGE_CURVE ( 'NONE', #32204, #22697, #42572, .T. ) ;
#17551=CARTESIAN_POINT ( 'NONE',  ( 4.109287492203100634, -193.5000000000000000, -113.3995532942336979 ) ) ;
#17552=EDGE_LOOP ( 'NONE', ( #36814, #49850, #13308, #11156 ) ) ;
#17554=ADVANCED_FACE ( 'NONE', ( #6586 ), #38623, .T. ) ;
#17557=CARTESIAN_POINT ( 'NONE',  ( -47.57632892154310866, -177.1207230881787780, -0.4300652022765113491 ) ) ;
#17558=EDGE_CURVE ( 'NONE', #18768, #1472, #1609, .T. ) ;
#17560=CARTESIAN_POINT ( 'NONE',  ( -47.97059563285962724, -175.3837268820161057, -0.8610436117673480050 ) ) ;
#17562=DIRECTION ( 'NONE',  ( 0.6528221181905227155, 0.000000000000000000, -0.7575112421616191360 ) ) ;
#17563=EDGE_LOOP ( 'NONE', ( #40645, #48314, #26568, #36586 ) ) ;
#17565=DIRECTION ( 'NONE',  ( -0.000000000000000000, 1.000000000000000000, -0.000000000000000000 ) ) ;
#17568=DIRECTION ( 'NONE',  ( 0.000000000000000000, 0.000000000000000000, 1.000000000000000000 ) ) ;
#17570=ORIENTED_EDGE ( 'NONE', *, *, #42635, .T. ) ;
#17571=ORIENTED_EDGE ( 'NONE', *, *, #17952, .F. ) ;
#17572=CARTESIAN_POINT ( 'NONE',  ( 26.10278175629141373, -193.5000000000000000, -99.06333546307678262 ) ) ;
#17574=ORIENTED_EDGE ( 'NONE', *, *, #5082, .T. ) ;
#17575=DIRECTION ( 'NONE',  ( 0.000000000000000000, 0.000000000000000000, 1.000000000000000000 ) ) ;
#17576=LINE ( 'NONE', #50407, #22587 ) ;
#17578=DIRECTION ( 'NONE',  ( 0.000000000000000000, 1.000000000000000000, -0.000000000000000000 ) ) ;
#17579=ORIENTED_EDGE ( 'NONE', *, *, #4421, .F. ) ;
#17581=CYLINDRICAL_SURFACE ( 'NONE', #33777, 124.9999999999999858 ) ;
#17583=AXIS2_PLACEMENT_3D ( 'NONE', #14680, #23590, #47523 ) ;
#17585=DIRECTION ( 'NONE',  ( -0.1182731709213660498, 0.000000000000000000, 0.9929810960135169173 ) ) ;
#17586=ORIENTED_EDGE ( 'NONE', *, *, #18530, .F. ) ;
#17588=AXIS2_PLACEMENT_3D ( 'NONE', #50639, #29879, #50137 ) ;
#17589=DIRECTION ( 'NONE',  ( 0.000000000000000000, -1.000000000000000000, -0.000000000000000000 ) ) ;
#17590=CARTESIAN_POINT ( 'NONE',  ( 67.42090074966655777, -189.7472609257535510, -46.82076062204440348 ) ) ;
#17591=DIRECTION ( 'NONE',  ( -0.7765238627180482966, 0.000000000000000000, 0.6300878435817038881 ) ) ;
#17593=CARTESIAN_POINT ( 'NONE',  ( 14.94072793302542124, -189.7472609257535510, 107.7168604805791574 ) ) ;
#17594=CARTESIAN_POINT ( 'NONE',  ( -133.8011377042516301, -193.5000000000000000, -91.35181687837437892 ) ) ;
#17595=DIRECTION ( 'NONE',  ( 0.9890401873221633666, 0.000000000000000000, 0.1476465640024850756 ) ) ;
#17596=VERTEX_POINT ( 'NONE', #35195 ) ;
#17598=PLANE ( 'NONE',  #10979 ) ;
#17599=CARTESIAN_POINT ( 'NONE',  ( -115.7878797639662025, -193.5000000000000000, -104.1428419024399545 ) ) ;
#17603=ORIENTED_EDGE ( 'NONE', *, *, #43159, .T. ) ;
#17604=ORIENTED_EDGE ( 'NONE', *, *, #38767, .T. ) ;
#17607=DIRECTION ( 'NONE',  ( -0.9266896074318370369, 0.000000000000000000, 0.3758275821142292306 ) ) ;
#17609=DIRECTION ( 'NONE',  ( 1.000000000000000000, 0.000000000000000000, -0.000000000000000000 ) ) ;
#17611=LINE ( 'NONE', #21801, #51444 ) ;
#17612=EDGE_CURVE ( 'NONE', #48961, #5269, #9755, .T. ) ;
#17615=CARTESIAN_POINT ( 'NONE',  ( -143.2689064740322351, -193.5000000000000000, -79.94433946042764205 ) ) ;
#17616=ORIENTED_EDGE ( 'NONE', *, *, #6983, .T. ) ;
#17617=EDGE_CURVE ( 'NONE', #16239, #46127, #47303, .T. ) ;
#17618=DIRECTION ( 'NONE',  ( 0.000000000000000000, 0.000000000000000000, 1.000000000000000000 ) ) ;
#17620=EDGE_CURVE ( 'NONE', #47120, #23170, #23121, .T. ) ;
#17621=DIRECTION ( 'NONE',  ( 0.000000000000000000, -1.000000000000000000, 0.000000000000000000 ) ) ;
#17623=CIRCLE ( 'NONE', #44429, 125.0000000000000000 ) ;
#17624=ORIENTED_EDGE ( 'NONE', *, *, #18392, .F. ) ;
#17625=PLANE ( 'NONE',  #24212 ) ;
#17626=EDGE_CURVE ( 'NONE', #49035, #45874, #27573, .T. ) ;
#17627=ORIENTED_EDGE ( 'NONE', *, *, #394, .F. ) ;
#17629=DIRECTION ( 'NONE',  ( 0.000000000000000000, -1.000000000000000000, 0.000000000000000000 ) ) ;
#17631=DIRECTION ( 'NONE',  ( 0.000000000000000000, 0.000000000000000000, -1.000000000000000000 ) ) ;
#17632=CARTESIAN_POINT ( 'NONE',  ( 31.28129687248616619, -177.1207230881787780, 96.24590808611479531 ) ) ;
#17633=ORIENTED_EDGE ( 'NONE', *, *, #27334, .F. ) ;
#17635=ORIENTED_EDGE ( 'NONE', *, *, #46418, .F. ) ;
#17636=CARTESIAN_POINT ( 'NONE',  ( -81.47409310123212833, -177.1207230881787780, -119.5301634136912412 ) ) ;
#17637=ORIENTED_EDGE ( 'NONE', *, *, #30337, .T. ) ;
#17638=DIRECTION ( 'NONE',  ( 0.000000000000000000, 0.000000000000000000, -1.000000000000000000 ) ) ;
#17639=CARTESIAN_POINT ( 'NONE',  ( -47.87232660569025455, -189.7472609257535510, -0.7948544414133454916 ) ) ;
#17641=ORIENTED_EDGE ( 'NONE', *, *, #16828, .T. ) ;
#17642=EDGE_CURVE ( 'NONE', #41498, #48626, #3145, .T. ) ;
#17644=AXIS2_PLACEMENT_3D ( 'NONE', #17557, #28827, #17800 ) ;
#17646=DIRECTION ( 'NONE',  ( 0.000000000000000000, 0.000000000000000000, 1.000000000000000000 ) ) ;
#17647=CARTESIAN_POINT ( 'NONE',  ( 71.15591247552653442, -177.1207230881787780, 36.22785377504035154 ) ) ;
#17648=DIRECTION ( 'NONE',  ( 0.8757349421956345248, 0.000000000000000000, 0.4827922027307490205 ) ) ;
#17649=VERTEX_POINT ( 'NONE', #43854 ) ;
#17650=DIRECTION ( 'NONE',  ( -0.08879589532293158394, 0.000000000000000000, -0.9960498426152172291 ) ) ;
#17651=CARTESIAN_POINT ( 'NONE',  ( -49.25565061422688728, -193.5000000000000000, -0.6300878435817132139 ) ) ;
#17652=LINE ( 'NONE', #41023, #46118 ) ;
#17655=CARTESIAN_POINT ( 'NONE',  ( 27.23560471289043861, -189.7472609257535510, 99.45993886622846958 ) ) ;
#17656=CARTESIAN_POINT ( 'NONE',  ( -169.9883746053192795, -193.5000000000000000, -24.72869175143020115 ) ) ;
#17657=EDGE_CURVE ( 'NONE', #1828, #27213, #23382, .T. ) ;
#17658=DIRECTION ( 'NONE',  ( -0.6749830015182196608, 0.000000000000000000, 0.7378332790417189146 ) ) ;
#17659=ORIENTED_EDGE ( 'NONE', *, *, #46479, .T. ) ;
#17661=DIRECTION ( 'NONE',  ( -0.000000000000000000, 1.000000000000000000, -0.000000000000000000 ) ) ;
#17663=EDGE_CURVE ( 'NONE', #47785, #27930, #34942, .T. ) ;
#17664=CARTESIAN_POINT ( 'NONE',  ( 76.46082103836691601, -189.7472609257535510, 3.874202661595774533 ) ) ;
#17666=EDGE_CURVE ( 'NONE', #563, #40551, #31506, .T. ) ;
#17667=EDGE_CURVE ( 'NONE', #22277, #4055, #46960, .T. ) ;
#17668=ADVANCED_FACE ( 'NONE', ( #26710 ), #42995, .T. ) ;
#17670=FACE_OUTER_BOUND ( 'NONE', #30615, .T. ) ;
#17673=ORIENTED_EDGE ( 'NONE', *, *, #50433, .F. ) ;
#17675=PLANE ( 'NONE',  #19042 ) ;
#17676=EDGE_CURVE ( 'NONE', #38746, #47822, #34340, .T. ) ;
#17677=VECTOR ( 'NONE', #27157, 1000.000000000000000 ) ;
#17680=FACE_OUTER_BOUND ( 'NONE', #20116, .T. ) ;
#17681=ORIENTED_EDGE ( 'NONE', *, *, #9317, .F. ) ;
#17682=ORIENTED_EDGE ( 'NONE', *, *, #38374, .F. ) ;
#17684=ORIENTED_EDGE ( 'NONE', *, *, #38759, .T. ) ;
#17685=DIRECTION ( 'NONE',  ( 0.000000000000000000, -1.000000000000000000, 0.000000000000000000 ) ) ;
#17686=EDGE_CURVE ( 'NONE', #20713, #50002, #50632, .T. ) ;
#17687=DIRECTION ( 'NONE',  ( 0.000000000000000000, 0.000000000000000000, 1.000000000000000000 ) ) ;
#17688=DIRECTION ( 'NONE',  ( 0.000000000000000000, 0.000000000000000000, 1.000000000000000000 ) ) ;
#17689=EDGE_LOOP ( 'NONE', ( #19228, #24454, #31874, #24478 ) ) ;
#17692=FACE_OUTER_BOUND ( 'NONE', #14991, .T. ) ;
#17695=DIRECTION ( 'NONE',  ( -0.2920567706369764371, 0.000000000000000000, 0.9564009842765223146 ) ) ;
#17696=ORIENTED_EDGE ( 'NONE', *, *, #31700, .T. ) ;
#17697=DIRECTION ( 'NONE',  ( 0.000000000000000000, 0.000000000000000000, 1.000000000000000000 ) ) ;
#17698=ORIENTED_EDGE ( 'NONE', *, *, #38951, .T. ) ;
#17699=LINE ( 'NONE', #37909, #38356 ) ;
#17700=DIRECTION ( 'NONE',  ( 0.000000000000000000, -1.000000000000000000, 0.000000000000000000 ) ) ;
#17701=DIRECTION ( 'NONE',  ( 0.000000000000000000, 0.000000000000000000, -1.000000000000000000 ) ) ;
#17703=ORIENTED_EDGE ( 'NONE', *, *, #35594, .T. ) ;
#17704=ORIENTED_EDGE ( 'NONE', *, *, #42744, .T. ) ;
#17705=DIRECTION ( 'NONE',  ( 0.000000000000000000, -1.000000000000000000, -0.000000000000000000 ) ) ;
#17706=DIRECTION ( 'NONE',  ( 0.000000000000000000, 0.000000000000000000, -1.000000000000000000 ) ) ;
#17709=CIRCLE ( 'NONE', #47071, 125.0000000000000000 ) ;
#17710=ORIENTED_EDGE ( 'NONE', *, *, #42030, .F. ) ;
#17711=DIRECTION ( 'NONE',  ( -0.000000000000000000, 1.000000000000000000, -0.000000000000000000 ) ) ;
#17712=CARTESIAN_POINT ( 'NONE',  ( -85.14888725715766782, -189.7472609257535510, 119.5003291395398719 ) ) ;
#17714=ORIENTED_EDGE ( 'NONE', *, *, #27782, .F. ) ;
#17715=PLANE ( 'NONE',  #583 ) ;
#17716=ORIENTED_EDGE ( 'NONE', *, *, #40767, .F. ) ;
#17717=DIRECTION ( 'NONE',  ( 0.9960498426152165630, 0.000000000000000000, 0.08879589532293852283 ) ) ;
#17719=CARTESIAN_POINT ( 'NONE',  ( 6.039888445539284056, -193.5000000000000000, 111.3726929437940498 ) ) ;
#17721=DIRECTION ( 'NONE',  ( 0.000000000000000000, 0.000000000000000000, 1.000000000000000000 ) ) ;
#17722=CARTESIAN_POINT ( 'NONE',  ( -49.30901192927172616, -189.7472609257535510, -123.9972451320097093 ) ) ;
#17723=DIRECTION ( 'NONE',  ( 0.000000000000000000, 0.000000000000000000, 1.000000000000000000 ) ) ;
#17727=CARTESIAN_POINT ( 'NONE',  ( -48.47912675150885065, -177.1207230881787780, 6.938893903907228378E-15 ) ) ;
#17728=ORIENTED_EDGE ( 'NONE', *, *, #24054, .F. ) ;
#17730=CARTESIAN_POINT ( 'NONE',  ( -130.7087404384255080, -193.5000000000000000, -94.14505102712755047 ) ) ;
#17731=FACE_OUTER_BOUND ( 'NONE', #5250, .T. ) ;
#17732=ORIENTED_EDGE ( 'NONE', *, *, #24726, .F. ) ;
#17733=VERTEX_POINT ( 'NONE', #50899 ) ;
#17737=DIRECTION ( 'NONE',  ( 0.000000000000000000, 1.000000000000000000, 0.000000000000000000 ) ) ;
#17739=ORIENTED_EDGE ( 'NONE', *, *, #38223, .T. ) ;
#17746=ORIENTED_EDGE ( 'NONE', *, *, #29928, .T. ) ;
#17747=EDGE_CURVE ( 'NONE', #47759, #21174, #17349, .T. ) ;
#17748=VECTOR ( 'NONE', #4930, 1000.000000000000000 ) ;
#17749=EDGE_LOOP ( 'NONE', ( #17062, #12835, #36686, #31294 ) ) ;
#17750=CARTESIAN_POINT ( 'NONE',  ( 6.443011874827240248, -177.1207230881787780, 112.2878385610370771 ) ) ;
#17755=ORIENTED_EDGE ( 'NONE', *, *, #15276, .F. ) ;
#17756=ORIENTED_EDGE ( 'NONE', *, *, #8503, .T. ) ;
#17757=CARTESIAN_POINT ( 'NONE',  ( -48.47912675150885065, -189.7472609257535510, 6.938893903907228378E-15 ) ) ;
#17758=ORIENTED_EDGE ( 'NONE', *, *, #27825, .T. ) ;
#17760=AXIS2_PLACEMENT_3D ( 'NONE', #594, #8472, #39740 ) ;
#17762=DIRECTION ( 'NONE',  ( -0.9646355819083556327, 0.000000000000000000, -0.2635871660690782825 ) ) ;
#17765=ORIENTED_EDGE ( 'NONE', *, *, #2217, .T. ) ;
#17767=ORIENTED_EDGE ( 'NONE', *, *, #2505, .F. ) ;
#17772=AXIS2_PLACEMENT_3D ( 'NONE', #19071, #35092, #19330 ) ;
#17773=CARTESIAN_POINT ( 'NONE',  ( -238.7407812814481076, -193.5000000000000000, -9.999999999999987566 ) ) ;
#17774=CARTESIAN_POINT ( 'NONE',  ( 53.56330073376472001, -193.5000000000000000, 72.19655804062048787 ) ) ;
#17775=DIRECTION ( 'NONE',  ( 0.000000000000000000, -1.000000000000000000, 0.000000000000000000 ) ) ;
#17776=EDGE_CURVE ( 'NONE', #51281, #49340, #32386, .T. ) ;
#17777=VECTOR ( 'NONE', #6204, 999.9999999999998863 ) ;
#17779=AXIS2_PLACEMENT_3D ( 'NONE', #20548, #5579, #17141 ) ;
#17780=DIRECTION ( 'NONE',  ( -0.000000000000000000, 1.000000000000000000, -0.000000000000000000 ) ) ;
#17782=ORIENTED_EDGE ( 'NONE', *, *, #13134, .F. ) ;
#17783=DIRECTION ( 'NONE',  ( 0.000000000000000000, 0.000000000000000000, 1.000000000000000000 ) ) ;
#17784=VERTEX_POINT ( 'NONE', #6499 ) ;
#17785=ORIENTED_EDGE ( 'NONE', *, *, #27298, .T. ) ;
#17786=CARTESIAN_POINT ( 'NONE',  ( 67.66641500972446011, -193.5000000000000000, 46.20836643931067300 ) ) ;
#17787=EDGE_LOOP ( 'NONE', ( #9522, #47857, #13560, #23688 ) ) ;
#17788=VECTOR ( 'NONE', #19280, 1000.000000000000114 ) ;
#17789=CARTESIAN_POINT ( 'NONE',  ( -34.51936650669026818, -189.7472609257535510, -124.2180546213278234 ) ) ;
#17790=AXIS2_PLACEMENT_3D ( 'NONE', #38789, #7778, #43531 ) ;
#17791=CARTESIAN_POINT ( 'NONE',  ( -166.9492939735806090, -193.5000000000000000, 39.87254040532603483 ) ) ;
#17792=DIRECTION ( 'NONE',  ( 0.000000000000000000, 0.000000000000000000, -1.000000000000000000 ) ) ;
#17794=ADVANCED_FACE ( 'NONE', ( #42747 ), #42209, .T. ) ;
#17796=ORIENTED_EDGE ( 'NONE', *, *, #19737, .F. ) ;
#17797=EDGE_LOOP ( 'NONE', ( #24222, #50606, #47913, #47549 ) ) ;
#17799=CARTESIAN_POINT ( 'NONE',  ( -48.47912675150885065, -189.7472609257535510, 6.938893903907228378E-15 ) ) ;
#17800=DIRECTION ( 'NONE',  ( 0.000000000000000000, 0.000000000000000000, -1.000000000000000000 ) ) ;
#17801=SURFACE_STYLE_USAGE ( .BOTH. , #22250 ) ;
#17803=DIRECTION ( 'NONE',  ( 0.000000000000000000, 0.000000000000000000, 1.000000000000000000 ) ) ;
#17806=CIRCLE ( 'NONE', #48763, 125.0000000000000000 ) ;
#17808=DIRECTION ( 'NONE',  ( -0.000000000000000000, 1.000000000000000000, -0.000000000000000000 ) ) ;
#17809=CARTESIAN_POINT ( 'NONE',  ( -48.47912675150885065, -177.1207230881787780, 6.938893903907228378E-15 ) ) ;
#17810=ORIENTED_EDGE ( 'NONE', *, *, #51396, .F. ) ;
#17811=DIRECTION ( 'NONE',  ( 0.000000000000000000, 0.000000000000000000, -1.000000000000000000 ) ) ;
#17812=VERTEX_POINT ( 'NONE', #34079 ) ;
#17813=ORIENTED_EDGE ( 'NONE', *, *, #5676, .T. ) ;
#17816=DIRECTION ( 'NONE',  ( 0.000000000000000000, -1.000000000000000000, 0.000000000000000000 ) ) ;
#17818=EDGE_CURVE ( 'NONE', #44900, #27780, #45929, .T. ) ;
#17822=DIRECTION ( 'NONE',  ( 0.000000000000000000, 0.000000000000000000, -1.000000000000000000 ) ) ;
#17824=AXIS2_PLACEMENT_3D ( 'NONE', #20487, #36013, #36513 ) ;
#17826=ADVANCED_FACE ( 'NONE', ( #22525 ), #30136, .T. ) ;
#17831=AXIS2_PLACEMENT_3D ( 'NONE', #26131, #5406, #45866 ) ;
#17832=DIRECTION ( 'NONE',  ( 0.000000000000000000, 1.000000000000000000, 0.000000000000000000 ) ) ;
#17833=ORIENTED_EDGE ( 'NONE', *, *, #8173, .T. ) ;
#17834=DIRECTION ( 'NONE',  ( -0.000000000000000000, 0.000000000000000000, -1.000000000000000000 ) ) ;
#17835=DIRECTION ( 'NONE',  ( -0.8610436117673621048, 0.000000000000000000, 0.5085311186492095237 ) ) ;
#17836=LINE ( 'NONE', #4985, #49817 ) ;
#17843=ORIENTED_EDGE ( 'NONE', *, *, #46587, .F. ) ;
#17844=EDGE_CURVE ( 'NONE', #50110, #25185, #22772, .T. ) ;
#17845=CARTESIAN_POINT ( 'NONE',  ( -15.24927435600542402, -177.1207230881787780, 120.5021863277718950 ) ) ;
#17847=DIRECTION ( 'NONE',  ( 0.000000000000000000, 0.000000000000000000, -1.000000000000000000 ) ) ;
#17849=ORIENTED_EDGE ( 'NONE', *, *, #13850, .T. ) ;
#17850=CARTESIAN_POINT ( 'NONE',  ( 58.45385938022562300, -177.1207230881787780, 62.78108192022012446 ) ) ;
#17851=VERTEX_POINT ( 'NONE', #7523 ) ;
#17852=VECTOR ( 'NONE', #15526, 1000.000000000000000 ) ;
#17853=PLANE ( 'NONE',  #5815 ) ;
#17855=CARTESIAN_POINT ( 'NONE',  ( -49.44376233341720450, -193.5000000000000000, -0.2635871660690713436 ) ) ;
#17856=EDGE_CURVE ( 'NONE', #5586, #31784, #35360, .T. ) ;
#17858=PLANE ( 'NONE',  #35295 ) ;
#17859=VECTOR ( 'NONE', #47526, 1000.000000000000000 ) ;
#17861=VECTOR ( 'NONE', #29573, 1000.000000000000000 ) ;
#17863=EDGE_LOOP ( 'NONE', ( #23219, #38330, #4217, #17152 ) ) ;
#17864=LINE ( 'NONE', #33879, #51925 ) ;
#17866=AXIS2_PLACEMENT_3D ( 'NONE', #45112, #5892, #37144 ) ;
#17867=ORIENTED_EDGE ( 'NONE', *, *, #6310, .F. ) ;
#17871=DIRECTION ( 'NONE',  ( 0.000000000000000000, -0.000000000000000000, 1.000000000000000000 ) ) ;
#17872=CARTESIAN_POINT ( 'NONE',  ( 74.68865188374466868, -193.5000000000000000, 14.34663989163627562 ) ) ;
#17873=ORIENTED_EDGE ( 'NONE', *, *, #25153, .T. ) ;
#17874=CARTESIAN_POINT ( 'NONE',  ( -40.90423906728908321, -175.3837268820161057, -124.7702732086912221 ) ) ;
#17875=FACE_OUTER_BOUND ( 'NONE', #47456, .T. ) ;
#17877=CARTESIAN_POINT ( 'NONE',  ( -105.7090724259148118, -193.5000000000000000, 111.1293539894142839 ) ) ;
#17878=VERTEX_POINT ( 'NONE', #39555 ) ;
#17879=CARTESIAN_POINT ( 'NONE',  ( 4.109287492203100634, -177.1207230881787780, -113.3995532942336979 ) ) ;
#17880=VECTOR ( 'NONE', #31721, 1000.000000000000000 ) ;
#17881=ORIENTED_EDGE ( 'NONE', *, *, #7337, .F. ) ;
#17882=EDGE_CURVE ( 'NONE', #46508, #4562, #51170, .T. ) ;
#17883=EDGE_CURVE ( 'NONE', #10308, #7533, #11961, .T. ) ;
#17888=ORIENTED_EDGE ( 'NONE', *, *, #12234, .T. ) ;
#17889=AXIS2_PLACEMENT_3D ( 'NONE', #42918, #27142, #50317 ) ;
#17890=DIRECTION ( 'NONE',  ( -0.000000000000000000, 1.000000000000000000, -0.000000000000000000 ) ) ;
#17892=PLANE ( 'NONE',  #37076 ) ;
#17893=LINE ( 'NONE', #49952, #23165 ) ;
#17896=DIRECTION ( 'NONE',  ( 0.000000000000000000, -1.000000000000000000, 0.000000000000000000 ) ) ;
#17901=ADVANCED_FACE ( 'NONE', ( #15932 ), #3833, .T. ) ;
#17904=AXIS2_PLACEMENT_3D ( 'NONE', #4095, #1101, #31933 ) ;
#17905=CARTESIAN_POINT ( 'NONE',  ( -48.82732838694325750, -189.7472609257535510, 0.9374196611341252261 ) ) ;
#17906=ADVANCED_FACE ( 'NONE', ( #24321 ), #32199, .F. ) ;
#17907=LINE ( 'NONE', #49708, #46410 ) ;
#17908=ORIENTED_EDGE ( 'NONE', *, *, #51554, .F. ) ;
#17910=ADVANCED_FACE ( 'NONE', ( #51418 ), #12221, .F. ) ;
#17912=FACE_OUTER_BOUND ( 'NONE', #37775, .T. ) ;
#17913=EDGE_CURVE ( 'NONE', #16796, #3069, #27483, .T. ) ;
#17914=FACE_OUTER_BOUND ( 'NONE', #39913, .T. ) ;
#17916=CIRCLE ( 'NONE', #50620, 125.0000000000000000 ) ;
#17918=CARTESIAN_POINT ( 'NONE',  ( -49.46816693883101124, -193.5000000000000000, -0.1476465640024848536 ) ) ;
#17919=DIRECTION ( 'NONE',  ( -0.000000000000000000, 1.000000000000000000, -0.000000000000000000 ) ) ;
#17920=CARTESIAN_POINT ( 'NONE',  ( -48.47912675150885065, -183.6283474603465606, 6.938893903907228378E-15 ) ) ;
#17922=ORIENTED_EDGE ( 'NONE', *, *, #45979, .T. ) ;
#17923=AXIS2_PLACEMENT_3D ( 'NONE', #18855, #23068, #51452 ) ;
#17924=DIRECTION ( 'NONE',  ( 0.000000000000000000, 0.000000000000000000, 1.000000000000000000 ) ) ;
#17925=CARTESIAN_POINT ( 'NONE',  ( -172.0602536473422504, -193.5000000000000000, -10.18383939837523755 ) ) ;
#17926=ORIENTED_EDGE ( 'NONE', *, *, #19844, .F. ) ;
#17927=ADVANCED_FACE ( 'NONE', ( #27734 ), #8296, .T. ) ;
#17928=ORIENTED_EDGE ( 'NONE', *, *, #52010, .T. ) ;
#17930=LINE ( 'NONE', #21878, #44330 ) ;
#17931=CYLINDRICAL_SURFACE ( 'NONE', #32825, 125.0000000000000000 ) ;
#17932=PLANE ( 'NONE',  #36374 ) ;
#17933=VECTOR ( 'NONE', #30534, 1000.000000000000000 ) ;
#17936=CARTESIAN_POINT ( 'NONE',  ( -48.47912675150885065, -175.3837268820161057, 6.938893903907228378E-15 ) ) ;
#17937=DIRECTION ( 'NONE',  ( -0.000000000000000000, 1.000000000000000000, -0.000000000000000000 ) ) ;
#17938=DIRECTION ( 'NONE',  ( 0.000000000000000000, 0.000000000000000000, -1.000000000000000000 ) ) ;
#17940=VECTOR ( 'NONE', #11211, 1000.000000000000000 ) ;
#17942=VERTEX_POINT ( 'NONE', #47979 ) ;
#17946=ADVANCED_FACE ( 'NONE', ( #47215 ), #44029, .T. ) ;
#17950=CARTESIAN_POINT ( 'NONE',  ( 18.00181100848376303, -177.1207230881787780, -105.8550183720733742 ) ) ;
#17951=LINE ( 'NONE', #49508, #20701 ) ;
#17952=EDGE_CURVE ( 'NONE', #50350, #12133, #51778, .T. ) ;
#17955=CARTESIAN_POINT ( 'NONE',  ( -8.169009709621407822, -183.6283474603465606, 118.3219948448695504 ) ) ;
#17956=DIRECTION ( 'NONE',  ( 0.000000000000000000, -1.000000000000000000, 0.000000000000000000 ) ) ;
#17957=VERTEX_POINT ( 'NONE', #31421 ) ;
#17958=EDGE_CURVE ( 'NONE', #33929, #24680, #47462, .T. ) ;
#17961=ORIENTED_EDGE ( 'NONE', *, *, #52008, .T. ) ;
#17962=DIRECTION ( 'NONE',  ( -0.9027978299657477557, 0.000000000000000000, 0.4300652022765115712 ) ) ;
#17963=EDGE_CURVE ( 'NONE', #20252, #45739, #391, .T. ) ;
#17964=CARTESIAN_POINT ( 'NONE',  ( -164.6246685127424882, -175.3837268820161057, -46.20836643930982035 ) ) ;
#17966=ADVANCED_FACE ( 'NONE', ( #32722 ), #33237, .T. ) ;
#17969=ORIENTED_EDGE ( 'NONE', *, *, #17612, .T. ) ;
#17971=CARTESIAN_POINT ( 'NONE',  ( 5.542374969221969039, -193.5000000000000000, 112.7238987608088365 ) ) ;
#17972=DIRECTION ( 'NONE',  ( 0.000000000000000000, -1.000000000000000000, 0.000000000000000000 ) ) ;
#17978=VECTOR ( 'NONE', #32532, 1000.000000000000227 ) ;
#17982=LINE ( 'NONE', #34760, #17012 ) ;
#17985=DIRECTION ( 'NONE',  ( -0.9027978299657387629, 0.000000000000000000, -0.4300652022765304450 ) ) ;
#17987=ORIENTED_EDGE ( 'NONE', *, *, #18778, .F. ) ;
#17991=ORIENTED_EDGE ( 'NONE', *, *, #32991, .T. ) ;
#17992=PLANE ( 'NONE',  #11341 ) ;
#17996=VECTOR ( 'NONE', #35832, 1000.000000000000114 ) ;
#17999=CARTESIAN_POINT ( 'NONE',  ( -161.4184887245413904, -177.1207230881787780, 51.19472891551358629 ) ) ;
#18001=ORIENTED_EDGE ( 'NONE', *, *, #37233, .T. ) ;
#18004=DIRECTION ( 'NONE',  ( 0.000000000000000000, -1.000000000000000000, 0.000000000000000000 ) ) ;
#18006=CARTESIAN_POINT ( 'NONE',  ( -118.4510020108455706, -189.7472609257535510, 103.5805805771131105 ) ) ;
#18007=CARTESIAN_POINT ( 'NONE',  ( 48.47907891923915713, -193.5000000000000000, 78.89300572996904748 ) ) ;
#18008=EDGE_LOOP ( 'NONE', ( #34136, #41151, #43954, #37754 ) ) ;
#18009=EDGE_CURVE ( 'NONE', #16186, #32301, #541, .T. ) ;
#18013=ADVANCED_FACE ( 'NONE', ( #37182 ), #8799, .T. ) ;
#18014=ORIENTED_EDGE ( 'NONE', *, *, #1500, .F. ) ;
#18017=CARTESIAN_POINT ( 'NONE',  ( -157.5429198988176438, -193.5000000000000000, 61.07445476073480961 ) ) ;
#18020=CARTESIAN_POINT ( 'NONE',  ( -6.081033889300858419, -175.3837268820161057, -116.5264228893325651 ) ) ;
#18026=DIRECTION ( 'NONE',  ( 0.000000000000000000, 0.000000000000000000, -1.000000000000000000 ) ) ;
#18028=ORIENTED_EDGE ( 'NONE', *, *, #38400, .F. ) ;
#18029=CIRCLE ( 'NONE', #7916, 125.0000000000000000 ) ;
#18032=FACE_OUTER_BOUND ( 'NONE', #51962, .T. ) ;
#18033=DIRECTION ( 'NONE',  ( -0.2348860457809842095, 0.000000000000000000, 0.9720229140804107493 ) ) ;
#18035=VECTOR ( 'NONE', #28301, 1000.000000000000000 ) ;
#18036=EDGE_CURVE ( 'NONE', #46272, #7639, #12325, .T. ) ;
#18038=ORIENTED_EDGE ( 'NONE', *, *, #45435, .T. ) ;
#18039=VECTOR ( 'NONE', #26781, 1000.000000000000000 ) ;
#18041=ORIENTED_EDGE ( 'NONE', *, *, #44644, .F. ) ;
#18043=DIRECTION ( 'NONE',  ( 0.9473263538541899509, 0.000000000000000000, 0.3202698538628415692 ) ) ;
#18044=VERTEX_POINT ( 'NONE', #21154 ) ;
#18046=LINE ( 'NONE', #34575, #43571 ) ;
#18048=ORIENTED_EDGE ( 'NONE', *, *, #35305, .T. ) ;
#18050=DIRECTION ( 'NONE',  ( 0.000000000000000000, -1.000000000000000000, -0.000000000000000000 ) ) ;
#18052=VERTEX_POINT ( 'NONE', #28508 ) ;
#18053=VERTEX_POINT ( 'NONE', #29298 ) ;
#18054=ORIENTED_EDGE ( 'NONE', *, *, #41136, .F. ) ;
#18055=CARTESIAN_POINT ( 'NONE',  ( -48.47912675150885065, -183.6283474603465606, 6.938893903907228378E-15 ) ) ;
#18056=DIRECTION ( 'NONE',  ( 0.6300878435817148793, 0.000000000000000000, -0.7765238627180394149 ) ) ;
#18060=CARTESIAN_POINT ( 'NONE',  ( -15.81236726369125023, -177.1207230881787780, -120.6560517527615417 ) ) ;
#18062=VERTEX_POINT ( 'NONE', #8537 ) ;
#18063=AXIS2_PLACEMENT_3D ( 'NONE', #30423, #50170, #6263 ) ;
#18064=EDGE_CURVE ( 'NONE', #9404, #21667, #45349, .T. ) ;
#18066=CARTESIAN_POINT ( 'NONE',  ( -48.47912675150885065, -189.7472609257535510, 6.938893903907228378E-15 ) ) ;
#18067=ORIENTED_EDGE ( 'NONE', *, *, #39063, .T. ) ;
#18069=ORIENTED_EDGE ( 'NONE', *, *, #48803, .T. ) ;
#18070=ORIENTED_EDGE ( 'NONE', *, *, #51554, .T. ) ;
#18071=CARTESIAN_POINT ( 'NONE',  ( 52.98246549829695340, -193.5000000000000000, 73.01058346660533971 ) ) ;
#18072=CIRCLE ( 'NONE', #49970, 125.0000000000000000 ) ;
#18074=DIRECTION ( 'NONE',  ( -0.000000000000000000, 1.000000000000000000, -0.000000000000000000 ) ) ;
#18075=CIRCLE ( 'NONE', #6341, 124.9999999999999858 ) ;
#18076=ORIENTED_EDGE ( 'NONE', *, *, #30466, .F. ) ;
#18077=LINE ( 'NONE', #34103, #24524 ) ;
#18079=ORIENTED_EDGE ( 'NONE', *, *, #37242, .F. ) ;
#18083=VECTOR ( 'NONE', #1831, 1000.000000000000114 ) ;
#18085=CARTESIAN_POINT ( 'NONE',  ( -13.05859477122062273, -189.7472609257535510, -118.8334608768479796 ) ) ;
#18086=DIRECTION ( 'NONE',  ( -0.9473263538541876194, 0.000000000000000000, -0.3202698538628486746 ) ) ;
#18087=EDGE_CURVE ( 'NONE', #21790, #36146, #26580, .T. ) ;
#18088=CARTESIAN_POINT ( 'NONE',  ( -48.98765787015808115, -189.7472609257535510, 0.8610436117673582190 ) ) ;
#18089=VERTEX_POINT ( 'NONE', #29550 ) ;
#18090=PLANE ( 'NONE',  #48366 ) ;
#18091=CARTESIAN_POINT ( 'NONE',  ( -41.90263914168912152, -175.3837268820161057, -124.8268793598473536 ) ) ;
#18093=DIRECTION ( 'NONE',  ( 0.000000000000000000, 0.000000000000000000, -1.000000000000000000 ) ) ;
#18095=ORIENTED_EDGE ( 'NONE', *, *, #45847, .F. ) ;
#18097=CARTESIAN_POINT ( 'NONE',  ( 74.48795740376233709, -193.5000000000000000, -15.97798378892164806 ) ) ;
#18101=VECTOR ( 'NONE', #31068, 1000.000000000000000 ) ;
#18103=VECTOR ( 'NONE', #22412, 1000.000000000000000 ) ;
#18105=DIRECTION ( 'NONE',  ( -0.000000000000000000, -1.000000000000000000, 0.000000000000000000 ) ) ;
#18107=LINE ( 'NONE', #45712, #28759 ) ;
#18108=EDGE_CURVE ( 'NONE', #38792, #8523, #49552, .T. ) ;
#18109=ORIENTED_EDGE ( 'NONE', *, *, #51972, .F. ) ;
#18110=DIRECTION ( 'NONE',  ( 0.000000000000000000, 0.000000000000000000, 1.000000000000000000 ) ) ;
#18111=CARTESIAN_POINT ( 'NONE',  ( -166.9492939735806090, -175.3837268820161057, 39.87254040532603483 ) ) ;
#18114=AXIS2_PLACEMENT_3D ( 'NONE', #18637, #9988, #13920 ) ;
#18116=CIRCLE ( 'NONE', #31532, 125.0000000000000000 ) ;
#18118=ORIENTED_EDGE ( 'NONE', *, *, #16740, .F. ) ;
#18121=ORIENTED_EDGE ( 'NONE', *, *, #26390, .F. ) ;
#18122=CIRCLE ( 'NONE', #41586, 125.0000000000000000 ) ;
#18123=DIRECTION ( 'NONE',  ( 0.000000000000000000, 0.000000000000000000, 1.000000000000000000 ) ) ;
#18124=VERTEX_POINT ( 'NONE', #17999 ) ;
#18128=DIRECTION ( 'NONE',  ( 0.4031234292879730674, 0.000000000000000000, -0.9151456172430181280 ) ) ;
#18130=ORIENTED_EDGE ( 'NONE', *, *, #2522, .T. ) ;
#18131=PLANE ( 'NONE',  #30043 ) ;
#18133=VERTEX_POINT ( 'NONE', #21934 ) ;
#18135=VECTOR ( 'NONE', #13634, 1000.000000000000000 ) ;
#18137=VECTOR ( 'NONE', #26537, 1000.000000000000000 ) ;
#18138=ORIENTED_EDGE ( 'NONE', *, *, #4612, .T. ) ;
#18139=CARTESIAN_POINT ( 'NONE',  ( -51.89154260666836649, -177.1207230881787780, 124.9534129907280970 ) ) ;
#18140=ORIENTED_EDGE ( 'NONE', *, *, #49738, .F. ) ;
#18141=CIRCLE ( 'NONE', #45828, 125.0000000000000000 ) ;
#18142=DIRECTION ( 'NONE',  ( -0.000000000000000000, 1.000000000000000000, -0.000000000000000000 ) ) ;
#18143=CARTESIAN_POINT ( 'NONE',  ( -118.1688136093591908, -189.7472609257535510, -103.7706487676296803 ) ) ;
#18144=DIRECTION ( 'NONE',  ( 0.000000000000000000, 0.000000000000000000, 1.000000000000000000 ) ) ;
#18145=ORIENTED_EDGE ( 'NONE', *, *, #45214, .T. ) ;
#18147=LINE ( 'NONE', #6833, #18977 ) ;
#18149=DIRECTION ( 'NONE',  ( -0.4566292373937200777, 0.000000000000000000, 0.8896570909947436601 ) ) ;
#18151=EDGE_LOOP ( 'NONE', ( #2403, #3405, #6895, #3758 ) ) ;
#18152=CIRCLE ( 'NONE', #41653, 125.0000000000000000 ) ;
#18154=DIRECTION ( 'NONE',  ( 0.000000000000000000, 0.000000000000000000, 1.000000000000000000 ) ) ;
#18158=VECTOR ( 'NONE', #11685, 999.9999999999998863 ) ;
#18159=CARTESIAN_POINT ( 'NONE',  ( -23.25236516653334107, -193.5000000000000000, -121.4073237908566512 ) ) ;
#18164=CARTESIAN_POINT ( 'NONE',  ( 27.50603775690333563, -193.5000000000000000, -99.25348746834811209 ) ) ;
#18167=ORIENTED_EDGE ( 'NONE', *, *, #26595, .T. ) ;
#18168=DIRECTION ( 'NONE',  ( -0.000000000000000000, 1.000000000000000000, -0.000000000000000000 ) ) ;
#18169=DIRECTION ( 'NONE',  ( 0.000000000000000000, 1.000000000000000000, -0.000000000000000000 ) ) ;
#18170=CARTESIAN_POINT ( 'NONE',  ( -4.525132525065792777, -189.7472609257535510, 115.9484881370938325 ) ) ;
#18172=AXIS2_PLACEMENT_3D ( 'NONE', #36710, #9375, #48806 ) ;
#18173=AXIS2_PLACEMENT_3D ( 'NONE', #51978, #48550, #12525 ) ;
#18174=CYLINDRICAL_SURFACE ( 'NONE', #37082, 125.0000000000000000 ) ;
#18175=DIRECTION ( 'NONE',  ( -0.2920567706369628924, 0.000000000000000000, -0.9564009842765264224 ) ) ;
#18177=AXIS2_PLACEMENT_3D ( 'NONE', #18674, #15245, #22091 ) ;
#18179=ADVANCED_FACE ( 'NONE', ( #29809 ), #30855, .T. ) ;
#18180=ADVANCED_FACE ( 'NONE', ( #14062 ), #5921, .T. ) ;
#18182=DIRECTION ( 'NONE',  ( 0.9266896074318317078, 0.000000000000000000, 0.3758275821142421647 ) ) ;
#18184=EDGE_LOOP ( 'NONE', ( #17987, #43629, #2658, #27472 ) ) ;
#18188=CARTESIAN_POINT ( 'NONE',  ( 60.19403481868998540, -175.3837268820161057, -59.71720175837096178 ) ) ;
#18189=CIRCLE ( 'NONE', #50909, 125.0000000000000000 ) ;
#18190=VECTOR ( 'NONE', #14936, 1000.000000000000114 ) ;
#18192=FACE_OUTER_BOUND ( 'NONE', #115, .T. ) ;
#18193=AXIS2_PLACEMENT_3D ( 'NONE', #46636, #10621, #27928 ) ;
#18194=DIRECTION ( 'NONE',  ( -0.000000000000000000, 1.000000000000000000, -0.000000000000000000 ) ) ;
#18196=ADVANCED_FACE ( 'NONE', ( #49805 ), #37707, .F. ) ;
#18197=VECTOR ( 'NONE', #33188, 1000.000000000000000 ) ;
#18198=DIRECTION ( 'NONE',  ( 0.000000000000000000, 0.000000000000000000, 1.000000000000000000 ) ) ;
#18201=CARTESIAN_POINT ( 'NONE',  ( -84.53143451966460020, -189.7472609257535510, -118.6432945265037091 ) ) ;
#18202=EDGE_LOOP ( 'NONE', ( #718, #14248, #23594, #22272 ) ) ;
#18205=ORIENTED_EDGE ( 'NONE', *, *, #28860, .F. ) ;
#18206=CARTESIAN_POINT ( 'NONE',  ( 38.48673058372652633, -175.3837268820161057, 88.39086586114804334 ) ) ;
#18207=EDGE_CURVE ( 'NONE', #25337, #46929, #40833, .T. ) ;
#18208=ORIENTED_EDGE ( 'NONE', *, *, #13394, .F. ) ;
#18209=DIRECTION ( 'NONE',  ( 0.000000000000000000, 0.000000000000000000, 1.000000000000000000 ) ) ;
#18210=DIRECTION ( 'NONE',  ( -0.7378332790417333475, 0.000000000000000000, 0.6749830015182038956 ) ) ;
#18212=AXIS2_PLACEMENT_3D ( 'NONE', #50874, #50611, #14881 ) ;
#18213=VERTEX_POINT ( 'NONE', #38210 ) ;
#18215=CIRCLE ( 'NONE', #34148, 125.0000000000000000 ) ;
#18218=CARTESIAN_POINT ( 'NONE',  ( -48.47912675150885065, -183.6283474603465606, 6.938893903907228378E-15 ) ) ;
#18219=VECTOR ( 'NONE', #42141, 1000.000000000000000 ) ;
#18224=CARTESIAN_POINT ( 'NONE',  ( -137.2261550162226911, -193.5000000000000000, 86.60307583628420502 ) ) ;
#18226=VECTOR ( 'NONE', #11966, 1000.000000000000114 ) ;
#18227=CARTESIAN_POINT ( 'NONE',  ( -48.77118352214583297, -193.5000000000000000, 0.9564009842765270886 ) ) ;
#18230=VERTEX_POINT ( 'NONE', #6437 ) ;
#18232=VECTOR ( 'NONE', #24746, 1000.000000000000000 ) ;
#18234=DIRECTION ( 'NONE',  ( -0.1476465640024779702, 0.000000000000000000, -0.9890401873221644768 ) ) ;
#18235=CARTESIAN_POINT ( 'NONE',  ( 72.05536924052412928, -175.3837268820161057, 33.11246405730899056 ) ) ;
#18236=VERTEX_POINT ( 'NONE', #22464 ) ;
#18237=FACE_OUTER_BOUND ( 'NONE', #18558, .T. ) ;
#18241=DIRECTION ( 'NONE',  ( -0.000000000000000000, 1.000000000000000000, -0.000000000000000000 ) ) ;
#18242=CARTESIAN_POINT ( 'NONE',  ( -63.09433862318517328, -193.5000000000000000, -124.1426420773539405 ) ) ;
#18243=CARTESIAN_POINT ( 'NONE',  ( 64.72501964220592185, -189.7472609257535510, 53.00774697410174952 ) ) ;
#18245=ADVANCED_FACE ( 'NONE', ( #42684 ), #30578, .T. ) ;
#18246=ORIENTED_EDGE ( 'NONE', *, *, #35255, .F. ) ;
#18247=EDGE_CURVE ( 'NONE', #4695, #16186, #47917, .T. ) ;
#18248=EDGE_CURVE ( 'NONE', #47058, #22690, #6936, .T. ) ;
#18249=DIRECTION ( 'NONE',  ( 0.000000000000000000, 0.000000000000000000, -1.000000000000000000 ) ) ;
#18251=FACE_OUTER_BOUND ( 'NONE', #16811, .T. ) ;
#18252=CIRCLE ( 'NONE', #30803, 125.0000000000000000 ) ;
#18253=ORIENTED_EDGE ( 'NONE', *, *, #44940, .T. ) ;
#18254=DIRECTION ( 'NONE',  ( -0.000000000000000000, 1.000000000000000000, -0.000000000000000000 ) ) ;
#18255=EDGE_CURVE ( 'NONE', #23736, #32626, #43960, .T. ) ;
#18256=ORIENTED_EDGE ( 'NONE', *, *, #4731, .F. ) ;
#18258=CARTESIAN_POINT ( 'NONE',  ( -54.99637373343401237, -175.3837268820161057, 123.8286356280830773 ) ) ;
#18259=CIRCLE ( 'NONE', #3123, 125.0000000000000000 ) ;
#18260=EDGE_CURVE ( 'NONE', #22800, #27646, #47671, .T. ) ;
#18262=CARTESIAN_POINT ( 'NONE',  ( -41.90263914168912152, -193.5000000000000000, -124.8268793598473536 ) ) ;
#18264=VERTEX_POINT ( 'NONE', #40008 ) ;
#18266=VERTEX_POINT ( 'NONE', #22968 ) ;
#18268=CARTESIAN_POINT ( 'NONE',  ( -51.83230197877470147, -183.6283474603465606, 123.9551692589637639 ) ) ;
#18271=VECTOR ( 'NONE', #22397, 1000.000000000000000 ) ;
#18272=AXIS2_PLACEMENT_3D ( 'NONE', #16984, #25381, #45367 ) ;
#18273=LINE ( 'NONE', #25882, #46349 ) ;
#18275=ORIENTED_EDGE ( 'NONE', *, *, #1857, .T. ) ;
#18276=ADVANCED_FACE ( 'NONE', ( #11653 ), #11894, .T. ) ;
#18277=CIRCLE ( 'NONE', #47650, 125.0000000000000000 ) ;
#18278=LINE ( 'NONE', #994, #23188 ) ;
#18280=VERTEX_POINT ( 'NONE', #35820 ) ;
#18281=EDGE_LOOP ( 'NONE', ( #5528, #5645, #48580, #12805 ) ) ;
#18288=ORIENTED_EDGE ( 'NONE', *, *, #26613, .T. ) ;
#18290=ORIENTED_EDGE ( 'NONE', *, *, #23464, .T. ) ;
#18292=AXIS2_PLACEMENT_3D ( 'NONE', #1917, #17956, #41865 ) ;
#18293=VECTOR ( 'NONE', #36225, 1000.000000000000000 ) ;
#18294=CARTESIAN_POINT ( 'NONE',  ( -48.07600332222088468, -177.1207230881787780, 0.9151456172430280089 ) ) ;
#18296=CIRCLE ( 'NONE', #28361, 125.0000000000000000 ) ;
#18297=DIRECTION ( 'NONE',  ( 0.7378332790417239107, 0.000000000000000000, 0.6749830015182142207 ) ) ;
#18299=CARTESIAN_POINT ( 'NONE',  ( -78.41101675714241992, -189.7472609257535510, -120.3332351033023286 ) ) ;
#18300=CARTESIAN_POINT ( 'NONE',  ( 21.21056010634070432, -189.7472609257535510, 103.7706487676302061 ) ) ;
#18301=PLANE ( 'NONE',  #23603 ) ;
#18302=EDGE_CURVE ( 'NONE', #26407, #46129, #51113, .T. ) ;
#18303=EDGE_LOOP ( 'NONE', ( #4852, #9195, #50509, #47940 ) ) ;
#18307=EDGE_CURVE ( 'NONE', #8754, #10566, #47608, .T. ) ;
#18309=EDGE_CURVE ( 'NONE', #5120, #19493, #15869, .T. ) ;
#18310=PLANE ( 'NONE',  #33011 ) ;
#18311=ADVANCED_FACE ( 'NONE', ( #3261 ), #15100, .T. ) ;
#18313=EDGE_CURVE ( 'NONE', #27750, #4, #23235, .T. ) ;
#18314=AXIS2_PLACEMENT_3D ( 'NONE', #282, #16857, #32613 ) ;
#18317=LINE ( 'NONE', #14623, #33826 ) ;
#18318=VERTEX_POINT ( 'NONE', #47400 ) ;
#18319=PLANE ( 'NONE',  #42555 ) ;
#18320=DIRECTION ( 'NONE',  ( -0.3482016354344059095, 0.000000000000000000, 0.9374196611341183427 ) ) ;
#18321=DIRECTION ( 'NONE',  ( 0.000000000000000000, 0.000000000000000000, 1.000000000000000000 ) ) ;
#18322=VERTEX_POINT ( 'NONE', #51599 ) ;
#18323=ORIENTED_EDGE ( 'NONE', *, *, #48386, .F. ) ;
#18324=ORIENTED_EDGE ( 'NONE', *, *, #14585, .F. ) ;
#18327=CARTESIAN_POINT ( 'NONE',  ( 52.98246549829695340, -175.3837268820161057, 73.01058346660533971 ) ) ;
#18328=AXIS2_PLACEMENT_3D ( 'NONE', #48003, #20934, #12517 ) ;
#18330=AXIS2_PLACEMENT_3D ( 'NONE', #523, #36023, #40213 ) ;
#18331=SURFACE_STYLE_FILL_AREA ( #38276 ) ;
#18332=CARTESIAN_POINT ( 'NONE',  ( 66.49421114223471818, -189.7472609257535510, -46.44493303993017719 ) ) ;
#18334=ORIENTED_EDGE ( 'NONE', *, *, #21872, .T. ) ;
#18335=AXIS2_PLACEMENT_3D ( 'NONE', #2421, #18448, #10049 ) ;
#18337=ADVANCED_FACE ( 'NONE', ( #28957 ), #9014, .T. ) ;
#18339=ORIENTED_EDGE ( 'NONE', *, *, #25885, .F. ) ;
#18341=ORIENTED_EDGE ( 'NONE', *, *, #3686, .T. ) ;
#18342=VECTOR ( 'NONE', #47142, 1000.000000000000000 ) ;
#18345=ORIENTED_EDGE ( 'NONE', *, *, #29205, .F. ) ;
#18346=CARTESIAN_POINT ( 'NONE',  ( 64.72501964220592185, -193.5000000000000000, 53.00774697410174952 ) ) ;
#18348=CARTESIAN_POINT ( 'NONE',  ( 71.44208735029286572, -183.6283474603465606, 35.26900067126700833 ) ) ;
#18350=ORIENTED_EDGE ( 'NONE', *, *, #19340, .F. ) ;
#18352=ORIENTED_EDGE ( 'NONE', *, *, #13172, .T. ) ;
#18353=VECTOR ( 'NONE', #35440, 1000.000000000000000 ) ;
#18354=ORIENTED_EDGE ( 'NONE', *, *, #35155, .F. ) ;
#18355=CARTESIAN_POINT ( 'NONE',  ( -119.6907301311197216, -183.6283474603465606, 101.5140743725400370 ) ) ;
#18357=EDGE_LOOP ( 'NONE', ( #38942, #37998, #37791, #15185 ) ) ;
#18358=CARTESIAN_POINT ( 'NONE',  ( -162.7543581613524282, -177.1207230881787780, 50.65739320402011003 ) ) ;
#18359=LINE ( 'NONE', #14664, #32298 ) ;
#18361=CARTESIAN_POINT ( 'NONE',  ( -118.1688136093591908, -189.7472609257535510, -103.7706487676296803 ) ) ;
#18364=DIRECTION ( 'NONE',  ( 0.000000000000000000, 0.000000000000000000, 1.000000000000000000 ) ) ;
#18370=CYLINDRICAL_SURFACE ( 'NONE', #49920, 125.0000000000000000 ) ;
#18372=CARTESIAN_POINT ( 'NONE',  ( 56.77503207194101265, -189.7472609257535510, -67.42819922234311036 ) ) ;
#18373=ORIENTED_EDGE ( 'NONE', *, *, #22119, .T. ) ;
#18374=EDGE_CURVE ( 'NONE', #27011, #30763, #39186, .T. ) ;
#18377=ORIENTED_EDGE ( 'NONE', *, *, #243, .T. ) ;
#18381=DIRECTION ( 'NONE',  ( 0.000000000000000000, 1.000000000000000000, 0.000000000000000000 ) ) ;
#18384=ORIENTED_EDGE ( 'NONE', *, *, #11574, .F. ) ;
#18385=VECTOR ( 'NONE', #11733, 1000.000000000000000 ) ;
#18386=LINE ( 'NONE', #33877, #42447 ) ;
#18388=CARTESIAN_POINT ( 'NONE',  ( -48.24424070572787571, -189.7472609257535510, 0.9720229140804191870 ) ) ;
#18389=VERTEX_POINT ( 'NONE', #20839 ) ;
#18390=ADVANCED_FACE ( 'NONE', ( #36865 ), #33171, .T. ) ;
#18392=EDGE_CURVE ( 'NONE', #48065, #27409, #12146, .T. ) ;
#18393=CARTESIAN_POINT ( 'NONE',  ( -25.55153130240594450, -193.5000000000000000, 122.8793122007210599 ) ) ;
#18395=ORIENTED_EDGE ( 'NONE', *, *, #41373, .F. ) ;
#18397=CARTESIAN_POINT ( 'NONE',  ( -49.44376233341720450, -193.5000000000000000, -0.2635871660690713436 ) ) ;
#18398=ORIENTED_EDGE ( 'NONE', *, *, #6416, .F. ) ;
#18399=AXIS2_PLACEMENT_3D ( 'NONE', #45990, #9981, #13393 ) ;
#18400=DIRECTION ( 'NONE',  ( -0.5338233779648003940, 0.000000000000000000, 0.8455960035018199594 ) ) ;
#18401=ORIENTED_EDGE ( 'NONE', *, *, #15929, .F. ) ;
#18402=DIRECTION ( 'NONE',  ( 0.000000000000000000, 0.000000000000000000, -1.000000000000000000 ) ) ;
#18403=AXIS2_PLACEMENT_3D ( 'NONE', #30144, #33821, #22534 ) ;
#18405=DIRECTION ( 'NONE',  ( -0.000000000000000000, 1.000000000000000000, -0.000000000000000000 ) ) ;
#18406=CARTESIAN_POINT ( 'NONE',  ( -49.40581635894069024, -183.6283474603465606, 0.3758275821142362250 ) ) ;
#18407=DIRECTION ( 'NONE',  ( 0.000000000000000000, 1.000000000000000000, 0.000000000000000000 ) ) ;
#18411=CARTESIAN_POINT ( 'NONE',  ( -62.43888699632653072, -189.7472609257535510, 124.2180546213279229 ) ) ;
#18412=ORIENTED_EDGE ( 'NONE', *, *, #6092, .T. ) ;
#18413=CYLINDRICAL_SURFACE ( 'NONE', #11071, 125.0000000000000000 ) ;
#18414=DIRECTION ( 'NONE',  ( 0.000000000000000000, 0.000000000000000000, 1.000000000000000000 ) ) ;
#18419=CARTESIAN_POINT ( 'NONE',  ( -48.47912675150885065, -189.7472609257535510, 6.938893903907228378E-15 ) ) ;
#18421=EDGE_LOOP ( 'NONE', ( #15056, #10855, #1265, #51220 ) ) ;
#18424=CIRCLE ( 'NONE', #43580, 125.0000000000000000 ) ;
#18426=DIRECTION ( 'NONE',  ( 0.000000000000000000, -1.000000000000000000, 0.000000000000000000 ) ) ;
#18427=EDGE_LOOP ( 'NONE', ( #43202, #6486, #20449, #20374 ) ) ;
#18428=LINE ( 'NONE', #51266, #26492 ) ;
#18430=DIRECTION ( 'NONE',  ( 0.8294056854502049880, 0.000000000000000000, -0.5586467658036476935 ) ) ;
#18431=DIRECTION ( 'NONE',  ( 0.6068001458185945385, 0.000000000000000000, -0.7948544414133523750 ) ) ;
#18432=EDGE_CURVE ( 'NONE', #22639, #7756, #16899, .T. ) ;
#18433=VERTEX_POINT ( 'NONE', #17156 ) ;
#18434=FACE_OUTER_BOUND ( 'NONE', #17390, .T. ) ;
#18436=AXIS2_PLACEMENT_3D ( 'NONE', #5963, #14114, #46173 ) ;
#18438=DIRECTION ( 'NONE',  ( 0.000000000000000000, 1.000000000000000000, -0.000000000000000000 ) ) ;
#18440=AXIS2_PLACEMENT_3D ( 'NONE', #26327, #11315, #27352 ) ;
#18442=CARTESIAN_POINT ( 'NONE',  ( -48.47912675150885065, -189.7472609257535510, 6.938893903907228378E-15 ) ) ;
#18443=CARTESIAN_POINT ( 'NONE',  ( 76.46082103836691601, -189.7472609257535510, 3.874202661595774533 ) ) ;
#18444=ORIENTED_EDGE ( 'NONE', *, *, #32478, .T. ) ;
#18445=EDGE_LOOP ( 'NONE', ( #26535, #13929, #12875, #13535 ) ) ;
#18446=EDGE_LOOP ( 'NONE', ( #32893, #28570, #15431, #23420 ) ) ;
#18447=EDGE_CURVE ( 'NONE', #9912, #9410, #29965, .T. ) ;
#18448=DIRECTION ( 'NONE',  ( -0.4827922027307427477, 0.000000000000000000, -0.8757349421956379665 ) ) ;
#18449=CARTESIAN_POINT ( 'NONE',  ( -47.92047998570519951, -193.5000000000000000, -0.8294056854501942189 ) ) ;
#18450=DIRECTION ( 'NONE',  ( -0.000000000000000000, 1.000000000000000000, -0.000000000000000000 ) ) ;
#18451=ORIENTED_EDGE ( 'NONE', *, *, #24305, .T. ) ;
#18452=AXIS2_PLACEMENT_3D ( 'NONE', #23806, #4106, #28262 ) ;
#18454=CARTESIAN_POINT ( 'NONE',  ( -27.18512803868275540, -189.7472609257535510, -123.1729094355498262 ) ) ;
#18455=DIRECTION ( 'NONE',  ( -0.3202698538628487301, 0.000000000000000000, 0.9473263538541877304 ) ) ;
#18456=DIRECTION ( 'NONE',  ( 0.9374196611341183427, 0.000000000000000000, 0.3482016354344059095 ) ) ;
#18457=ORIENTED_EDGE ( 'NONE', *, *, #3295, .F. ) ;
#18458=CYLINDRICAL_SURFACE ( 'NONE', #31460, 125.0000000000000000 ) ;
#18462=DIRECTION ( 'NONE',  ( 0.000000000000000000, 0.000000000000000000, -1.000000000000000000 ) ) ;
#18463=DIRECTION ( 'NONE',  ( -0.000000000000000000, 1.000000000000000000, -0.000000000000000000 ) ) ;
#18469=VERTEX_POINT ( 'NONE', #37113 ) ;
#18470=CARTESIAN_POINT ( 'NONE',  ( -145.0195698084541505, -193.5000000000000000, 79.40367028273128369 ) ) ;
#18471=CARTESIAN_POINT ( 'NONE',  ( 116.9235303384055840, -213.5000000000000000, -9.999999999999971578 ) ) ;
#18472=EDGE_CURVE ( 'NONE', #43321, #43010, #24772, .T. ) ;
#18474=LINE ( 'NONE', #15305, #14993 ) ;
#18476=EDGE_CURVE ( 'NONE', #18911, #23451, #50127, .T. ) ;
#18479=DIRECTION ( 'NONE',  ( 0.000000000000000000, 0.000000000000000000, -1.000000000000000000 ) ) ;
#18480=ORIENTED_EDGE ( 'NONE', *, *, #40393, .F. ) ;
#18485=PLANE ( 'NONE',  #47403 ) ;
#18486=PLANE ( 'NONE',  #8982 ) ;
#18487=EDGE_CURVE ( 'NONE', #7752, #15492, #34167, .T. ) ;
#18488=EDGE_CURVE ( 'NONE', #33164, #7438, #29135, .T. ) ;
#18489=ADVANCED_FACE ( 'NONE', ( #44489 ), #45290, .F. ) ;
#18490=VECTOR ( 'NONE', #43192, 999.9999999999998863 ) ;
#18492=AXIS2_PLACEMENT_3D ( 'NONE', #42072, #18169, #26295 ) ;
#18497=CARTESIAN_POINT ( 'NONE',  ( -48.93575598890255662, -193.5000000000000000, -0.8896570909947461026 ) ) ;
#18500=ORIENTED_EDGE ( 'NONE', *, *, #46210, .F. ) ;
#18503=DIRECTION ( 'NONE',  ( -0.000000000000000000, 1.000000000000000000, -0.000000000000000000 ) ) ;
#18505=VECTOR ( 'NONE', #50964, 1000.000000000000000 ) ;
#18506=CARTESIAN_POINT ( 'NONE',  ( 76.47090317495664635, -193.5000000000000000, -3.534122433557446374 ) ) ;
#18508=CARTESIAN_POINT ( 'NONE',  ( -161.4019114581580823, -193.5000000000000000, 53.60452120946281696 ) ) ;
#18509=DIRECTION ( 'NONE',  ( -0.000000000000000000, 1.000000000000000000, -0.000000000000000000 ) ) ;
#18510=DIRECTION ( 'NONE',  ( 0.02963332782256331357, 0.000000000000000000, -0.9995608365087942371 ) ) ;
#18512=ORIENTED_EDGE ( 'NONE', *, *, #39092, .T. ) ;
#18513=ORIENTED_EDGE ( 'NONE', *, *, #19285, .T. ) ;
#18514=VERTEX_POINT ( 'NONE', #48135 ) ;
#18515=CARTESIAN_POINT ( 'NONE',  ( -48.47912675150885065, -173.5000000000000284, 6.938893903907228378E-15 ) ) ;
#18516=DIRECTION ( 'NONE',  ( -0.000000000000000000, 1.000000000000000000, -0.000000000000000000 ) ) ;
#18518=CARTESIAN_POINT ( 'NONE',  ( 43.63512310656542326, -193.5000000000000000, 84.49831343337136502 ) ) ;
#18521=CARTESIAN_POINT ( 'NONE',  ( 70.20858612167234014, -177.1207230881787780, 35.90758392117750475 ) ) ;
#18523=CIRCLE ( 'NONE', #10150, 125.0000000000000000 ) ;
#18524=ORIENTED_EDGE ( 'NONE', *, *, #8802, .T. ) ;
#18525=EDGE_LOOP ( 'NONE', ( #27917, #27959, #39002, #43174 ) ) ;
#18526=DIRECTION ( 'NONE',  ( -0.2348860457809911206, 0.000000000000000000, 0.9720229140804089729 ) ) ;
#18527=CARTESIAN_POINT ( 'NONE',  ( 61.06976976088564157, -189.7472609257535510, -60.19999396110169698 ) ) ;
#18530=EDGE_CURVE ( 'NONE', #20432, #28789, #41753, .T. ) ;
#18531=DIRECTION ( 'NONE',  ( -0.000000000000000000, 1.000000000000000000, -0.000000000000000000 ) ) ;
#18532=EDGE_CURVE ( 'NONE', #35, #50678, #3991, .T. ) ;
#18533=EDGE_CURVE ( 'NONE', #36997, #48106, #44263, .T. ) ;
#18535=ORIENTED_EDGE ( 'NONE', *, *, #27958, .T. ) ;
#18536=CARTESIAN_POINT ( 'NONE',  ( -49.47517659412406488, -189.7472609257535510, -0.08879589532293878651 ) ) ;
#18537=VERTEX_POINT ( 'NONE', #20801 ) ;
#18541=ORIENTED_EDGE ( 'NONE', *, *, #2462, .F. ) ;
#18544=CYLINDRICAL_SURFACE ( 'NONE', #20459, 125.0000000000000000 ) ;
#18545=CARTESIAN_POINT ( 'NONE',  ( -1.230335819511603423, -177.1207230881787780, 115.7261930397108216 ) ) ;
#18548=EDGE_CURVE ( 'NONE', #7465, #23874, #44190, .T. ) ;
#18550=EDGE_LOOP ( 'NONE', ( #441, #47418, #27584, #28933 ) ) ;
#18552=LINE ( 'NONE', #23281, #26452 ) ;
#18554=AXIS2_PLACEMENT_3D ( 'NONE', #24363, #3415, #26558 ) ;
#18555=EDGE_CURVE ( 'NONE', #16914, #12681, #12637, .T. ) ;
#18556=ORIENTED_EDGE ( 'NONE', *, *, #48887, .T. ) ;
#18557=CARTESIAN_POINT ( 'NONE',  ( 7.859956736328458149, -189.7472609257535510, -111.5836353223468649 ) ) ;
#18558=EDGE_LOOP ( 'NONE', ( #26023, #25953, #33240, #42220 ) ) ;
#18559=VECTOR ( 'NONE', #2466, 1000.000000000000227 ) ;
#18560=DIRECTION ( 'NONE',  ( 0.000000000000000000, 0.000000000000000000, -1.000000000000000000 ) ) ;
#18561=ORIENTED_EDGE ( 'NONE', *, *, #43964, .T. ) ;
#18562=FACE_OUTER_BOUND ( 'NONE', #6648, .T. ) ;
#18564=ORIENTED_EDGE ( 'NONE', *, *, #45888, .F. ) ;
#18568=EDGE_CURVE ( 'NONE', #10098, #2552, #1072, .T. ) ;
#18572=FACE_OUTER_BOUND ( 'NONE', #49505, .T. ) ;
#18577=PLANE ( 'NONE',  #23879 ) ;
#18578=ORIENTED_EDGE ( 'NONE', *, *, #38060, .T. ) ;
#18579=DIRECTION ( 'NONE',  ( -0.000000000000000000, 1.000000000000000000, -0.000000000000000000 ) ) ;
#18580=ADVANCED_FACE ( 'NONE', ( #28922 ), #36294, .T. ) ;
#18581=ORIENTED_EDGE ( 'NONE', *, *, #32534, .T. ) ;
#18583=ORIENTED_EDGE ( 'NONE', *, *, #38464, .F. ) ;
#18586=ORIENTED_EDGE ( 'NONE', *, *, #42917, .F. ) ;
#18589=EDGE_CURVE ( 'NONE', #34528, #13215, #36831, .T. ) ;
#18590=EDGE_CURVE ( 'NONE', #4651, #50992, #16866, .T. ) ;
#18592=ADVANCED_FACE ( 'NONE', ( #44984 ), #21056, .F. ) ;
#18595=ORIENTED_EDGE ( 'NONE', *, *, #44573, .T. ) ;
#18597=AXIS2_PLACEMENT_3D ( 'NONE', #42445, #42181, #50352 ) ;
#18598=ORIENTED_EDGE ( 'NONE', *, *, #18830, .F. ) ;
#18599=ADVANCED_FACE ( 'NONE', ( #10020 ), #25778, .T. ) ;
#18601=DIRECTION ( 'NONE',  ( 0.9027978299657446470, 0.000000000000000000, -0.4300652022765183435 ) ) ;
#18603=ADVANCED_FACE ( 'NONE', ( #5559 ), #49182, .T. ) ;
#18604=CARTESIAN_POINT ( 'NONE',  ( -77.03256798524179771, -175.3837268820161057, 121.6951149130964751 ) ) ;
#18605=VERTEX_POINT ( 'NONE', #13431 ) ;
#18610=EDGE_CURVE ( 'NONE', #895, #23734, #13243, .T. ) ;
#18611=ORIENTED_EDGE ( 'NONE', *, *, #40393, .T. ) ;
#18612=PLANE ( 'NONE',  #22977 ) ;
#18613=CARTESIAN_POINT ( 'NONE',  ( -172.1341525481709880, -189.7472609257535510, 18.28755301364335750 ) ) ;
#18616=CARTESIAN_POINT ( 'NONE',  ( -166.8403286750647680, -175.3837268820161057, -40.19484891389966918 ) ) ;
#18620=CARTESIAN_POINT ( 'NONE',  ( 64.86941505090324256, -183.6283474603465606, -50.28156562190504530 ) ) ;
#18623=VERTEX_POINT ( 'NONE', #33910 ) ;
#18626=EDGE_CURVE ( 'NONE', #4562, #50065, #29048, .T. ) ;
#18629=DIRECTION ( 'NONE',  ( 0.000000000000000000, 0.000000000000000000, -1.000000000000000000 ) ) ;
#18633=AXIS2_PLACEMENT_3D ( 'NONE', #49255, #45323, #41345 ) ;
#18636=AXIS2_PLACEMENT_3D ( 'NONE', #7935, #19765, #23472 ) ;
#18637=CARTESIAN_POINT ( 'NONE',  ( 75.27070168362158142, -189.7472609257535510, 17.63462396184792524 ) ) ;
#18639=ORIENTED_EDGE ( 'NONE', *, *, #27084, .F. ) ;
#18640=DIRECTION ( 'NONE',  ( 0.9473263538541899509, 0.000000000000000000, 0.3202698538628415692 ) ) ;
#18641=EDGE_LOOP ( 'NONE', ( #8972, #31436, #17698, #45940 ) ) ;
#18642=FACE_OUTER_BOUND ( 'NONE', #18947, .T. ) ;
#18644=DIRECTION ( 'NONE',  ( 0.000000000000000000, 1.000000000000000000, 0.000000000000000000 ) ) ;
#18645=CARTESIAN_POINT ( 'NONE',  ( -136.5246168469702468, -177.1207230881787780, 87.31661597576147926 ) ) ;
#18646=ORIENTED_EDGE ( 'NONE', *, *, #29102, .F. ) ;
#18647=DIRECTION ( 'NONE',  ( 0.000000000000000000, 0.000000000000000000, 1.000000000000000000 ) ) ;
#18649=VERTEX_POINT ( 'NONE', #26033 ) ;
#18650=VECTOR ( 'NONE', #46225, 1000.000000000000227 ) ;
#18654=CARTESIAN_POINT ( 'NONE',  ( -140.1460956102404509, -193.5000000000000000, 84.98333260264821831 ) ) ;
#18656=EDGE_CURVE ( 'NONE', #18469, #4360, #29197, .T. ) ;
#18658=CARTESIAN_POINT ( 'NONE',  ( -48.59739992243022755, -193.5000000000000000, 0.9929810960135230236 ) ) ;
#18659=CARTESIAN_POINT ( 'NONE',  ( -49.13194886969936448, -177.1207230881787780, -0.7575112421616214675 ) ) ;
#18661=ORIENTED_EDGE ( 'NONE', *, *, #6310, .T. ) ;
#18662=ORIENTED_EDGE ( 'NONE', *, *, #39133, .F. ) ;
#18663=ADVANCED_FACE ( 'NONE', ( #29447 ), #45251, .T. ) ;
#18664=CARTESIAN_POINT ( 'NONE',  ( -173.3294908491238004, -183.6283474603465606, -6.114457023560984972 ) ) ;
#18665=VERTEX_POINT ( 'NONE', #37335 ) ;
#18666=DIRECTION ( 'NONE',  ( -0.000000000000000000, 1.000000000000000000, -0.000000000000000000 ) ) ;
#18668=ORIENTED_EDGE ( 'NONE', *, *, #47422, .T. ) ;
#18669=CARTESIAN_POINT ( 'NONE',  ( -47.87232660569026166, -193.5000000000000000, 0.7948544414133635883 ) ) ;
#18670=CARTESIAN_POINT ( 'NONE',  ( -141.2664123866436796, -189.7472609257535510, -83.75869879877495805 ) ) ;
#18671=DIRECTION ( 'NONE',  ( 0.000000000000000000, -0.000000000000000000, -1.000000000000000000 ) ) ;
#18674=CARTESIAN_POINT ( 'NONE',  ( 61.06976976088562026, -175.3837268820161057, -60.19999396110170409 ) ) ;
#18675=VERTEX_POINT ( 'NONE', #45499 ) ;
#18676=DIRECTION ( 'NONE',  ( 0.000000000000000000, 0.000000000000000000, 1.000000000000000000 ) ) ;
#18678=CIRCLE ( 'NONE', #42971, 125.0000000000000000 ) ;
#18679=CARTESIAN_POINT ( 'NONE',  ( -48.77118352214581876, -183.6283474603465606, -0.9564009842765195391 ) ) ;
#18680=EDGE_LOOP ( 'NONE', ( #31530, #41725, #5143, #32974 ) ) ;
#18681=DIRECTION ( 'NONE',  ( -0.000000000000000000, 1.000000000000000000, -0.000000000000000000 ) ) ;
#18682=CARTESIAN_POINT ( 'NONE',  ( -173.4460699164830260, -193.5000000000000000, -2.874563619423202265 ) ) ;
#18684=DIRECTION ( 'NONE',  ( 0.000000000000000000, 1.000000000000000000, -0.000000000000000000 ) ) ;
#18686=ORIENTED_EDGE ( 'NONE', *, *, #22852, .T. ) ;
#18688=VECTOR ( 'NONE', #48474, 1000.000000000000114 ) ;
#18689=ADVANCED_FACE ( 'NONE', ( #33418 ), #38106, .F. ) ;
#18690=AXIS2_PLACEMENT_3D ( 'NONE', #29586, #30361, #25646 ) ;
#18691=CARTESIAN_POINT ( 'NONE',  ( -48.47912675150885065, -175.3837268820161057, 6.938893903907228378E-15 ) ) ;
#18698=LINE ( 'NONE', #22375, #9553 ) ;
#18699=ORIENTED_EDGE ( 'NONE', *, *, #20842, .T. ) ;
#18700=ORIENTED_EDGE ( 'NONE', *, *, #8990, .F. ) ;
#18704=PLANE ( 'NONE',  #41257 ) ;
#18705=DIRECTION ( 'NONE',  ( -0.000000000000000000, 1.000000000000000000, -0.000000000000000000 ) ) ;
#18706=ORIENTED_EDGE ( 'NONE', *, *, #33972, .T. ) ;
#18707=AXIS2_PLACEMENT_3D ( 'NONE', #21279, #29670, #13648 ) ;
#18708=LINE ( 'NONE', #18964, #36781 ) ;
#18710=DIRECTION ( 'NONE',  ( -0.000000000000000000, -1.000000000000000000, 0.000000000000000000 ) ) ;
#18713=DIRECTION ( 'NONE',  ( 0.000000000000000000, 0.000000000000000000, -1.000000000000000000 ) ) ;
#18714=ORIENTED_EDGE ( 'NONE', *, *, #48615, .T. ) ;
#18715=FACE_OUTER_BOUND ( 'NONE', #6268, .T. ) ;
#18719=LINE ( 'NONE', #26078, #17933 ) ;
#18720=PLANE ( 'NONE',  #13995 ) ;
#18721=CIRCLE ( 'NONE', #38848, 125.0000000000000000 ) ;
#18722=AXIS2_PLACEMENT_3D ( 'NONE', #38594, #3110, #26500 ) ;
#18724=ORIENTED_EDGE ( 'NONE', *, *, #14747, .T. ) ;
#18726=CARTESIAN_POINT ( 'NONE',  ( 24.07160180756802248, -193.5000000000000000, 100.5610240384924481 ) ) ;
#18729=LINE ( 'NONE', #3222, #8124 ) ;
#18730=LINE ( 'NONE', #3719, #12233 ) ;
#18733=VECTOR ( 'NONE', #11754, 1000.000000000000227 ) ;
#18734=CARTESIAN_POINT ( 'NONE',  ( -172.4728835572423975, -193.5000000000000000, 1.322128892812079792 ) ) ;
#18735=ORIENTED_EDGE ( 'NONE', *, *, #30099, .T. ) ;
#18736=CARTESIAN_POINT ( 'NONE',  ( -49.42645310536304493, -189.7472609257535510, 0.3202698538628349079 ) ) ;
#18737=VERTEX_POINT ( 'NONE', #30485 ) ;
#18738=DIRECTION ( 'NONE',  ( 0.08879589532293853671, 0.000000000000000000, -0.9960498426152166740 ) ) ;
#18739=DIRECTION ( 'NONE',  ( -0.000000000000000000, 1.000000000000000000, -0.000000000000000000 ) ) ;
#18740=EDGE_CURVE ( 'NONE', #36297, #22714, #15641, .T. ) ;
#18741=ORIENTED_EDGE ( 'NONE', *, *, #36983, .T. ) ;
#18743=DIRECTION ( 'NONE',  ( -0.9646355819083556327, 0.000000000000000000, -0.2635871660690782825 ) ) ;
#18745=CARTESIAN_POINT ( 'NONE',  ( -64.08700758308646073, -175.3837268820161057, -124.0217483183786982 ) ) ;
#18747=VERTEX_POINT ( 'NONE', #18670 ) ;
#18751=DIRECTION ( 'NONE',  ( 0.000000000000000000, 0.000000000000000000, -1.000000000000000000 ) ) ;
#18754=CARTESIAN_POINT ( 'NONE',  ( -49.08592689732745384, -177.1207230881787780, 0.7948544414133550395 ) ) ;
#18755=ADVANCED_FACE ( 'NONE', ( #51000 ), #3659, .F. ) ;
#18756=AXIS2_PLACEMENT_3D ( 'NONE', #34480, #34732, #50013 ) ;
#18759=EDGE_LOOP ( 'NONE', ( #11779, #12010, #16611, #36616 ) ) ;
#18760=LINE ( 'NONE', #10616, #40711 ) ;
#18761=ORIENTED_EDGE ( 'NONE', *, *, #10878, .F. ) ;
#18763=LINE ( 'NONE', #10358, #41814 ) ;
#18764=DIRECTION ( 'NONE',  ( -0.000000000000000000, 1.000000000000000000, -0.000000000000000000 ) ) ;
#18768=VERTEX_POINT ( 'NONE', #46529 ) ;
#18769=EDGE_CURVE ( 'NONE', #4233, #29477, #49339, .T. ) ;
#18770=DIRECTION ( 'NONE',  ( -4.884776371667510679E-16, 0.000000000000000000, -1.000000000000000000 ) ) ;
#18771=PLANE ( 'NONE',  #48691 ) ;
#18772=PLANE ( 'NONE',  #28717 ) ;
#18773=DIRECTION ( 'NONE',  ( 0.1768902751225666370, 0.000000000000000000, 0.9842305779475979399 ) ) ;
#18774=VECTOR ( 'NONE', #46997, 1000.000000000000000 ) ;
#18777=CARTESIAN_POINT ( 'NONE',  ( -107.1845112550870027, -183.6283474603465606, 109.2239789693437331 ) ) ;
#18778=EDGE_CURVE ( 'NONE', #48253, #16384, #18277, .T. ) ;
#18780=EDGE_LOOP ( 'NONE', ( #25056, #50447, #16020, #10248 ) ) ;
#18784=DIRECTION ( 'NONE',  ( 0.000000000000000000, 0.000000000000000000, -1.000000000000000000 ) ) ;
#18785=DIRECTION ( 'NONE',  ( 0.000000000000000000, 1.000000000000000000, -0.000000000000000000 ) ) ;
#18787=DIRECTION ( 'NONE',  ( 0.000000000000000000, -0.000000000000000000, -1.000000000000000000 ) ) ;
#18789=ORIENTED_EDGE ( 'NONE', *, *, #36507, .T. ) ;
#18790=CARTESIAN_POINT ( 'NONE',  ( -163.3872488209693472, -177.1207230881787780, -49.20491319441547517 ) ) ;
#18791=ORIENTED_EDGE ( 'NONE', *, *, #970, .F. ) ;
#18792=CARTESIAN_POINT ( 'NONE',  ( -88.23625491228469286, -193.5000000000000000, 118.5089480183148254 ) ) ;
#18793=CARTESIAN_POINT ( 'NONE',  ( -5.732832253866456007, -175.3837268820161057, -117.4638425504666657 ) ) ;
#18794=EDGE_CURVE ( 'NONE', #45161, #36997, #27050, .T. ) ;
#18795=ORIENTED_EDGE ( 'NONE', *, *, #17232, .T. ) ;
#18796=DIRECTION ( 'NONE',  ( 0.000000000000000000, -1.000000000000000000, 0.000000000000000000 ) ) ;
#18797=DIRECTION ( 'NONE',  ( 0.4031234292879730674, 0.000000000000000000, -0.9151456172430181280 ) ) ;
#18798=CARTESIAN_POINT ( 'NONE',  ( -48.47912675150885065, -193.5000000000000000, -0.9999999999999931166 ) ) ;
#18801=DIRECTION ( 'NONE',  ( -0.000000000000000000, 1.000000000000000000, -0.000000000000000000 ) ) ;
#18802=DIRECTION ( 'NONE',  ( -0.9266896074318291543, 0.000000000000000000, -0.3758275821142488260 ) ) ;
#18803=ORIENTED_EDGE ( 'NONE', *, *, #51891, .T. ) ;
#18804=VECTOR ( 'NONE', #24785, 999.9999999999998863 ) ;
#18807=CARTESIAN_POINT ( 'NONE',  ( 72.05536924052414349, -189.7472609257535510, 33.11246405730899056 ) ) ;
#18808=ORIENTED_EDGE ( 'NONE', *, *, #50403, .F. ) ;
#18809=LINE ( 'NONE', #10673, #6700 ) ;
#18810=ORIENTED_EDGE ( 'NONE', *, *, #47163, .F. ) ;
#18811=DIRECTION ( 'NONE',  ( -0.000000000000000000, 1.000000000000000000, -0.000000000000000000 ) ) ;
#18813=ORIENTED_EDGE ( 'NONE', *, *, #436, .F. ) ;
#18815=EDGE_CURVE ( 'NONE', #26252, #46287, #11276, .T. ) ;
#18817=CARTESIAN_POINT ( 'NONE',  ( 69.99104047056319189, -189.7472609257535510, -39.87254040532513955 ) ) ;
#18820=ORIENTED_EDGE ( 'NONE', *, *, #28177, .F. ) ;
#18821=EDGE_LOOP ( 'NONE', ( #45596, #5425, #42176, #32931 ) ) ;
#18822=VERTEX_POINT ( 'NONE', #35451 ) ;
#18824=DIRECTION ( 'NONE',  ( 0.05924062789371441901, 0.000000000000000000, -0.9982437317643214625 ) ) ;
#18827=DIRECTION ( 'NONE',  ( -0.000000000000000000, 1.000000000000000000, -0.000000000000000000 ) ) ;
#18830=EDGE_CURVE ( 'NONE', #50211, #25917, #35201, .T. ) ;
#18832=EDGE_LOOP ( 'NONE', ( #36355, #37709, #16743, #31218 ) ) ;
#18833=CARTESIAN_POINT ( 'NONE',  ( -48.71401279728982558, -177.1207230881787780, -0.9720229140804069745 ) ) ;
#18834=ORIENTED_EDGE ( 'NONE', *, *, #26882, .F. ) ;
#18835=ORIENTED_EDGE ( 'NONE', *, *, #33442, .F. ) ;
#18837=CARTESIAN_POINT ( 'NONE',  ( -131.1972941934623975, -193.5000000000000000, 92.37913469314125336 ) ) ;
#18838=CARTESIAN_POINT ( 'NONE',  ( 42.10477485469927927, -177.1207230881787780, 86.13684908212515268 ) ) ;
#18839=VECTOR ( 'NONE', #4234, 1000.000000000000000 ) ;
#18840=EDGE_CURVE ( 'NONE', #31544, #16791, #47529, .T. ) ;
#18841=VECTOR ( 'NONE', #1792, 1000.000000000000000 ) ;
#18844=ORIENTED_EDGE ( 'NONE', *, *, #48513, .T. ) ;
#18846=VERTEX_POINT ( 'NONE', #14475 ) ;
#18849=CARTESIAN_POINT ( 'NONE',  ( -99.02518858244150124, -175.3837268820161057, 114.3245189510261497 ) ) ;
#18852=ORIENTED_EDGE ( 'NONE', *, *, #16040, .T. ) ;
#18854=DIRECTION ( 'NONE',  ( 0.000000000000000000, 0.000000000000000000, 1.000000000000000000 ) ) ;
#18855=CARTESIAN_POINT ( 'NONE',  ( -87.28630321566649286, -193.5000000000000000, 118.8234112238818341 ) ) ;
#18856=LINE ( 'NONE', #43036, #38815 ) ;
#18858=VECTOR ( 'NONE', #16905, 1000.000000000000000 ) ;
#18859=DIRECTION ( 'NONE',  ( 0.000000000000000000, -0.000000000000000000, 1.000000000000000000 ) ) ;
#18860=DIRECTION ( 'NONE',  ( -0.000000000000000000, 1.000000000000000000, -0.000000000000000000 ) ) ;
#18861=CARTESIAN_POINT ( 'NONE',  ( -8.169009709621407822, -193.5000000000000000, 118.3219948448695504 ) ) ;
#18862=ORIENTED_EDGE ( 'NONE', *, *, #24708, .F. ) ;
#18863=CARTESIAN_POINT ( 'NONE',  ( 76.21810084846656252, -183.6283474603465606, -8.694908215727989997 ) ) ;
#18864=CARTESIAN_POINT ( 'NONE',  ( -170.4669447856608997, -193.5000000000000000, 22.25084316132122453 ) ) ;
#18865=ORIENTED_EDGE ( 'NONE', *, *, #40185, .F. ) ;
#18866=CARTESIAN_POINT ( 'NONE',  ( -172.0839188101925004, -193.5000000000000000, -18.62405380494756812 ) ) ;
#18867=ORIENTED_EDGE ( 'NONE', *, *, #51118, .F. ) ;
#18869=FACE_OUTER_BOUND ( 'NONE', #47016, .T. ) ;
#18870=AXIS2_PLACEMENT_3D ( 'NONE', #23333, #11480, #31197 ) ;
#18871=FACE_BOUND ( 'NONE', #16689, .T. ) ;
#18872=CARTESIAN_POINT ( 'NONE',  ( -47.57632892154311577, -175.3837268820161057, 0.4300652022765314997 ) ) ;
#18873=CARTESIAN_POINT ( 'NONE',  ( -160.2705093830644216, -177.1207230881787780, -55.92572546981521242 ) ) ;
#18875=AXIS2_PLACEMENT_3D ( 'NONE', #20404, #32229, #31454 ) ;
#18876=EDGE_CURVE ( 'NONE', #9572, #44523, #23628, .T. ) ;
#18877=EDGE_CURVE ( 'NONE', #28248, #6855, #24941, .T. ) ;
#18878=EDGE_CURVE ( 'NONE', #30289, #23283, #40179, .T. ) ;
#18879=PLANE ( 'NONE',  #38639 ) ;
#18880=VERTEX_POINT ( 'NONE', #16271 ) ;
#18881=VECTOR ( 'NONE', #11235, 1000.000000000000114 ) ;
#18884=CARTESIAN_POINT ( 'NONE',  ( 73.32083127613157103, -183.6283474603465606, 28.10285082451656535 ) ) ;
#18886=ADVANCED_FACE ( 'NONE', ( #12319 ), #24670, .T. ) ;
#18888=DIRECTION ( 'NONE',  ( 0.000000000000000000, 0.000000000000000000, 1.000000000000000000 ) ) ;
#18891=VECTOR ( 'NONE', #3204, 1000.000000000000000 ) ;
#18893=VECTOR ( 'NONE', #23605, 1000.000000000000000 ) ;
#18896=ORIENTED_EDGE ( 'NONE', *, *, #38484, .F. ) ;
#18897=CARTESIAN_POINT ( 'NONE',  ( 74.00867759460086859, -189.7472609257535510, 24.93467037017222410 ) ) ;
#18900=EDGE_CURVE ( 'NONE', #10499, #40286, #52038, .T. ) ;
#18901=LINE ( 'NONE', #19168, #23150 ) ;
#18903=DIRECTION ( 'NONE',  ( 0.000000000000000000, 0.000000000000000000, -1.000000000000000000 ) ) ;
#18904=ORIENTED_EDGE ( 'NONE', *, *, #43924, .T. ) ;
#18905=EDGE_CURVE ( 'NONE', #1914, #28854, #2204, .T. ) ;
#18906=FACE_OUTER_BOUND ( 'NONE', #21106, .T. ) ;
#18907=VERTEX_POINT ( 'NONE', #8128 ) ;
#18908=DIRECTION ( 'NONE',  ( 0.000000000000000000, 1.000000000000000000, 0.000000000000000000 ) ) ;
#18909=CARTESIAN_POINT ( 'NONE',  ( -67.10529315269987194, -193.5000000000000000, -122.5936119678274281 ) ) ;
#18911=VERTEX_POINT ( 'NONE', #24170 ) ;
#18912=ADVANCED_FACE ( 'NONE', ( #47826 ), #19956, .T. ) ;
#18919=DIRECTION ( 'NONE',  ( 0.000000000000000000, 0.000000000000000000, 1.000000000000000000 ) ) ;
#18923=CARTESIAN_POINT ( 'NONE',  ( -49.45768324380835423, -175.3837268820161057, 0.2059786187410958813 ) ) ;
#18924=VECTOR ( 'NONE', #17661, 1000.000000000000000 ) ;
#18925=VERTEX_POINT ( 'NONE', #51769 ) ;
#18927=CYLINDRICAL_SURFACE ( 'NONE', #16227, 125.0000000000000000 ) ;
#18929=CARTESIAN_POINT ( 'NONE',  ( -127.4665351220365892, -177.1207230881787780, -96.88131563365291754 ) ) ;
#18932=ORIENTED_EDGE ( 'NONE', *, *, #21, .F. ) ;
#18934=CARTESIAN_POINT ( 'NONE',  ( 71.18041382641612813, -189.7472609257535510, -32.52067927015755089 ) ) ;
#18935=AXIS2_PLACEMENT_3D ( 'NONE', #33105, #45223, #20496 ) ;
#18939=ORIENTED_EDGE ( 'NONE', *, *, #37816, .T. ) ;
#18942=PLANE ( 'NONE',  #10321 ) ;
#18943=DIRECTION ( 'NONE',  ( 0.000000000000000000, -1.000000000000000000, 0.000000000000000000 ) ) ;
#18944=FACE_OUTER_BOUND ( 'NONE', #36022, .T. ) ;
#18946=DIRECTION ( 'NONE',  ( -0.000000000000000000, 1.000000000000000000, -0.000000000000000000 ) ) ;
#18947=EDGE_LOOP ( 'NONE', ( #49311, #32126, #21727, #10926 ) ) ;
#18953=DIRECTION ( 'NONE',  ( 0.3482016354343928088, 0.000000000000000000, 0.9374196611341231167 ) ) ;
#18955=ORIENTED_EDGE ( 'NONE', *, *, #4011, .T. ) ;
#18956=AXIS2_PLACEMENT_3D ( 'NONE', #23635, #47577, #11560 ) ;
#18957=VERTEX_POINT ( 'NONE', #765 ) ;
#18963=ORIENTED_EDGE ( 'NONE', *, *, #15279, .T. ) ;
#18964=CARTESIAN_POINT ( 'NONE',  ( 34.98161733638499982, -193.5000000000000000, -91.70840728318313495 ) ) ;
#18966=CARTESIAN_POINT ( 'NONE',  ( -6.081033889300861972, -193.5000000000000000, -116.5264228893325509 ) ) ;
#18967=LINE ( 'NONE', #7134, #22429 ) ;
#18969=ADVANCED_FACE ( 'NONE', ( #9177 ), #19685, .F. ) ;
#18972=DIRECTION ( 'NONE',  ( 0.000000000000000000, -1.000000000000000000, 0.000000000000000000 ) ) ;
#18973=ORIENTED_EDGE ( 'NONE', *, *, #40704, .F. ) ;
#18975=ORIENTED_EDGE ( 'NONE', *, *, #16404, .T. ) ;
#18976=DIRECTION ( 'NONE',  ( 0.000000000000000000, 0.000000000000000000, -1.000000000000000000 ) ) ;
#18977=VECTOR ( 'NONE', #34174, 1000.000000000000000 ) ;
#18978=DIRECTION ( 'NONE',  ( -0.000000000000000000, 1.000000000000000000, -0.000000000000000000 ) ) ;
#18979=CARTESIAN_POINT ( 'NONE',  ( -104.3615810019516630, -189.7472609257535510, 110.6939782313525455 ) ) ;
#18980=CYLINDRICAL_SURFACE ( 'NONE', #48347, 125.0000000000000000 ) ;
#18982=EDGE_CURVE ( 'NONE', #48695, #39147, #25729, .T. ) ;
#18984=ORIENTED_EDGE ( 'NONE', *, *, #17090, .F. ) ;
#18986=DIRECTION ( 'NONE',  ( 0.9982437317643210184, 0.000000000000000000, 0.05924062789372143423 ) ) ;
#18987=ORIENTED_EDGE ( 'NONE', *, *, #28681, .F. ) ;
#18989=CARTESIAN_POINT ( 'NONE',  ( -49.03777351731249468, -175.3837268820161057, -0.8294056854502022125 ) ) ;
#18990=EDGE_LOOP ( 'NONE', ( #47829, #41191, #50160, #5289 ) ) ;
#18992=PLANE ( 'NONE',  #13901 ) ;
#18993=VERTEX_POINT ( 'NONE', #17327 ) ;
#18995=VERTEX_POINT ( 'NONE', #21257 ) ;
#18997=AXIS2_PLACEMENT_3D ( 'NONE', #168, #48794, #32227 ) ;
#18998=FACE_OUTER_BOUND ( 'NONE', #2318, .T. ) ;
#18999=ORIENTED_EDGE ( 'NONE', *, *, #40726, .T. ) ;
#19000=AXIS2_PLACEMENT_3D ( 'NONE', #34618, #29641, #34112 ) ;
#19001=AXIS2_PLACEMENT_3D ( 'NONE', #22785, #18579, #22258 ) ;
#19005=ORIENTED_EDGE ( 'NONE', *, *, #4131, .T. ) ;
#19006=CARTESIAN_POINT ( 'NONE',  ( -91.22542124915045747, -175.3837268820161057, 117.4638425504669783 ) ) ;
#19007=AXIS2_PLACEMENT_3D ( 'NONE', #40812, #1127, #45047 ) ;
#19008=VECTOR ( 'NONE', #43923, 1000.000000000000000 ) ;
#19009=DIRECTION ( 'NONE',  ( -0.000000000000000000, 1.000000000000000000, -0.000000000000000000 ) ) ;
#19010=DIRECTION ( 'NONE',  ( -0.000000000000000000, 1.000000000000000000, -0.000000000000000000 ) ) ;
#19014=ORIENTED_EDGE ( 'NONE', *, *, #29331, .F. ) ;
#19016=ADVANCED_FACE ( 'NONE', ( #13890 ), #45190, .F. ) ;
#19017=CARTESIAN_POINT ( 'NONE',  ( -151.4272465800706016, -193.5000000000000000, 70.89911581792887318 ) ) ;
#19019=VECTOR ( 'NONE', #51889, 1000.000000000000000 ) ;
#19021=VERTEX_POINT ( 'NONE', #22024 ) ;
#19022=ORIENTED_EDGE ( 'NONE', *, *, #47365, .F. ) ;
#19023=DIRECTION ( 'NONE',  ( 0.02963332782254913048, 0.000000000000000000, 0.9995608365087946812 ) ) ;
#19024=AXIS2_PLACEMENT_3D ( 'NONE', #26010, #37591, #22065 ) ;
#19025=ORIENTED_EDGE ( 'NONE', *, *, #39677, .T. ) ;
#19027=DIRECTION ( 'NONE',  ( 0.000000000000000000, 1.000000000000000000, -0.000000000000000000 ) ) ;
#19030=ORIENTED_EDGE ( 'NONE', *, *, #32193, .F. ) ;
#19031=ORIENTED_EDGE ( 'NONE', *, *, #18876, .F. ) ;
#19032=ORIENTED_EDGE ( 'NONE', *, *, #10584, .F. ) ;
#19033=DIRECTION ( 'NONE',  ( -0.000000000000000000, 1.000000000000000000, -0.000000000000000000 ) ) ;
#19034=DIRECTION ( 'NONE',  ( 0.000000000000000000, 1.000000000000000000, 0.000000000000000000 ) ) ;
#19035=VECTOR ( 'NONE', #43226, 1000.000000000000000 ) ;
#19037=VECTOR ( 'NONE', #42391, 1000.000000000000000 ) ;
#19038=EDGE_CURVE ( 'NONE', #4051, #49012, #14159, .T. ) ;
#19040=FACE_OUTER_BOUND ( 'NONE', #12823, .T. ) ;
#19042=AXIS2_PLACEMENT_3D ( 'NONE', #13714, #1098, #33443 ) ;
#19044=ADVANCED_FACE ( 'NONE', ( #37278 ), #29644, .T. ) ;
#19046=EDGE_LOOP ( 'NONE', ( #18076, #671, #31236, #26618 ) ) ;
#19047=VECTOR ( 'NONE', #22673, 1000.000000000000000 ) ;
#19049=PLANE ( 'NONE',  #47432 ) ;
#19050=CYLINDRICAL_SURFACE ( 'NONE', #35907, 125.0000000000000000 ) ;
#19051=AXIS2_PLACEMENT_3D ( 'NONE', #37612, #2109, #21846 ) ;
#19053=AXIS2_PLACEMENT_3D ( 'NONE', #6645, #27632, #23182 ) ;
#19054=VECTOR ( 'NONE', #2696, 1000.000000000000114 ) ;
#19055=CARTESIAN_POINT ( 'NONE',  ( 55.03325008324584644, -183.6283474603465606, -70.07273251429357686 ) ) ;
#19059=EDGE_CURVE ( 'NONE', #10177, #12033, #9954, .T. ) ;
#19061=CIRCLE ( 'NONE', #25773, 125.0000000000000000 ) ;
#19063=DIRECTION ( 'NONE',  ( 0.000000000000000000, 0.000000000000000000, 1.000000000000000000 ) ) ;
#19064=DIRECTION ( 'NONE',  ( 0.8896570909947499883, 0.000000000000000000, -0.4566292373937077542 ) ) ;
#19065=VERTEX_POINT ( 'NONE', #29385 ) ;
#19066=CARTESIAN_POINT ( 'NONE',  ( -162.3451783319732726, -177.1207230881787780, 51.57055649762781968 ) ) ;
#19067=FACE_OUTER_BOUND ( 'NONE', #40791, .T. ) ;
#19068=LINE ( 'NONE', #43743, #1347 ) ;
#19069=CARTESIAN_POINT ( 'NONE',  ( -172.0042974347349229, -193.5000000000000000, 10.84123789944660210 ) ) ;
#19070=EDGE_CURVE ( 'NONE', #32782, #22041, #8091, .T. ) ;
#19071=CARTESIAN_POINT ( 'NONE',  ( -48.47912675150885065, -175.3837268820161057, 6.938893903907228378E-15 ) ) ;
#19077=ORIENTED_EDGE ( 'NONE', *, *, #17676, .T. ) ;
#19079=VERTEX_POINT ( 'NONE', #50166 ) ;
#19082=ADVANCED_FACE ( 'NONE', ( #17067 ), #37018, .T. ) ;
#19083=ORIENTED_EDGE ( 'NONE', *, *, #27480, .T. ) ;
#19084=LINE ( 'NONE', #23288, #48643 ) ;
#19085=VECTOR ( 'NONE', #23492, 1000.000000000000114 ) ;
#19086=EDGE_CURVE ( 'NONE', #7533, #11977, #31603, .T. ) ;
#19091=ORIENTED_EDGE ( 'NONE', *, *, #46435, .F. ) ;
#19092=CARTESIAN_POINT ( 'NONE',  ( -173.4291566779743050, -193.5000000000000000, 3.534122433558352760 ) ) ;
#19096=VERTEX_POINT ( 'NONE', #10446 ) ;
#19097=VERTEX_POINT ( 'NONE', #47947 ) ;
#19099=VECTOR ( 'NONE', #23666, 1000.000000000000000 ) ;
#19101=CARTESIAN_POINT ( 'NONE',  ( -31.47951320919343488, -193.5000000000000000, -122.8300162461135301 ) ) ;
#19102=EDGE_CURVE ( 'NONE', #49449, #19466, #14827, .T. ) ;
#19103=LINE ( 'NONE', #11198, #44433 ) ;
#19106=ORIENTED_EDGE ( 'NONE', *, *, #9108, .T. ) ;
#19107=LINE ( 'NONE', #31433, #43386 ) ;
#19109=CARTESIAN_POINT ( 'NONE',  ( -48.71401279728984690, -189.7472609257535510, 0.9720229140804159673 ) ) ;
#19112=VERTEX_POINT ( 'NONE', #18604 ) ;
#19113=VECTOR ( 'NONE', #31504, 1000.000000000000114 ) ;
#19115=PLANE ( 'NONE',  #47646 ) ;
#19116=AXIS2_PLACEMENT_3D ( 'NONE', #20112, #44809, #134 ) ;
#19118=DIRECTION ( 'NONE',  ( 0.3482016354343995812, 0.000000000000000000, -0.9374196611341205632 ) ) ;
#19119=ORIENTED_EDGE ( 'NONE', *, *, #14094, .T. ) ;
#19120=CARTESIAN_POINT ( 'NONE',  ( -161.6832731452239500, -189.7472609257535510, -53.00774697410101055 ) ) ;
#19122=EDGE_LOOP ( 'NONE', ( #30374, #13165, #49229, #24774 ) ) ;
#19124=AXIS2_PLACEMENT_3D ( 'NONE', #31417, #23796, #27477 ) ;
#19125=FACE_OUTER_BOUND ( 'NONE', #15227, .T. ) ;
#19127=CIRCLE ( 'NONE', #21647, 125.0000000000000000 ) ;
#19128=PLANE ( 'NONE',  #21514 ) ;
#19129=DIRECTION ( 'NONE',  ( 0.6528221181905174975, 0.000000000000000000, 0.7575112421616236880 ) ) ;
#19132=DIRECTION ( 'NONE',  ( 0.000000000000000000, 0.000000000000000000, -1.000000000000000000 ) ) ;
#19134=DIRECTION ( 'NONE',  ( -0.000000000000000000, 1.000000000000000000, -0.000000000000000000 ) ) ;
#19135=DIRECTION ( 'NONE',  ( 0.5085311186492273983, 0.000000000000000000, -0.8610436117673514467 ) ) ;
#19139=CARTESIAN_POINT ( 'NONE',  ( -173.1763543514842070, -193.5000000000000000, 8.694908215728892387 ) ) ;
#19143=EDGE_CURVE ( 'NONE', #31601, #43746, #2248, .T. ) ;
#19144=ORIENTED_EDGE ( 'NONE', *, *, #50049, .F. ) ;
#19146=AXIS2_PLACEMENT_3D ( 'NONE', #30807, #14271, #6894 ) ;
#19148=AXIS2_PLACEMENT_3D ( 'NONE', #25136, #22214, #17247 ) ;
#19149=EDGE_CURVE ( 'NONE', #39380, #16176, #39777, .T. ) ;
#19150=FACE_BOUND ( 'NONE', #1426, .T. ) ;
#19152=ORIENTED_EDGE ( 'NONE', *, *, #47711, .F. ) ;
#19153=AXIS2_PLACEMENT_3D ( 'NONE', #30852, #7192, #42925 ) ;
#19155=ORIENTED_EDGE ( 'NONE', *, *, #16890, .F. ) ;
#19156=ORIENTED_EDGE ( 'NONE', *, *, #24591, .F. ) ;
#19159=ORIENTED_EDGE ( 'NONE', *, *, #2739, .F. ) ;
#19160=CARTESIAN_POINT ( 'NONE',  ( -146.8460685364478593, -177.1207230881787780, 75.49882471933935335 ) ) ;
#19163=LINE ( 'NONE', #34911, #16513 ) ;
#19166=CARTESIAN_POINT ( 'NONE',  ( 55.92943606843918047, -175.3837268820161057, -66.89437584437831674 ) ) ;
#19167=ORIENTED_EDGE ( 'NONE', *, *, #4640, .F. ) ;
#19168=CARTESIAN_POINT ( 'NONE',  ( -18.54723674587610205, -193.5000000000000000, 120.3332351033025844 ) ) ;
#19169=EDGE_LOOP ( 'NONE', ( #34146, #51321, #45173, #23659 ) ) ;
#19170=LINE ( 'NONE', #39630, #49958 ) ;
#19171=EDGE_LOOP ( 'NONE', ( #32409, #11215, #7846, #31781 ) ) ;
#19173=VERTEX_POINT ( 'NONE', #10717 ) ;
#19176=ORIENTED_EDGE ( 'NONE', *, *, #33377, .F. ) ;
#19178=EDGE_CURVE ( 'NONE', #19715, #24408, #40486, .T. ) ;
#19179=VERTEX_POINT ( 'NONE', #19816 ) ;
#19181=CIRCLE ( 'NONE', #30090, 125.0000000000000000 ) ;
#19185=CARTESIAN_POINT ( 'NONE',  ( -25.55153130240594450, -193.5000000000000000, 122.8793122007210599 ) ) ;
#19186=DIRECTION ( 'NONE',  ( 0.000000000000000000, 0.000000000000000000, -1.000000000000000000 ) ) ;
#19187=DIRECTION ( 'NONE',  ( -0.000000000000000000, 1.000000000000000000, 0.000000000000000000 ) ) ;
#19188=AXIS2_PLACEMENT_3D ( 'NONE', #9211, #29680, #44689 ) ;
#19189=DIRECTION ( 'NONE',  ( -0.000000000000000000, 1.000000000000000000, -0.000000000000000000 ) ) ;
#19190=EDGE_CURVE ( 'NONE', #16507, #35850, #29924, .T. ) ;
#19191=EDGE_CURVE ( 'NONE', #4441, #10029, #37461, .T. ) ;
#19192=ORIENTED_EDGE ( 'NONE', *, *, #42726, .T. ) ;
#19193=EDGE_CURVE ( 'NONE', #36633, #38465, #14409, .T. ) ;
#19195=DIRECTION ( 'NONE',  ( -0.7765238627180349740, 0.000000000000000000, -0.6300878435817203194 ) ) ;
#19196=DIRECTION ( 'NONE',  ( 0.000000000000000000, 0.000000000000000000, -1.000000000000000000 ) ) ;
#19198=LINE ( 'NONE', #14738, #11985 ) ;
#19199=VERTEX_POINT ( 'NONE', #6782 ) ;
#19200=VECTOR ( 'NONE', #30917, 1000.000000000000000 ) ;
#19202=EDGE_CURVE ( 'NONE', #27293, #44533, #14661, .T. ) ;
#19203=CARTESIAN_POINT ( 'NONE',  ( -109.0835867659424565, -177.1207230881787780, -109.3256576763154726 ) ) ;
#19206=EDGE_LOOP ( 'NONE', ( #17635, #35639, #8933, #21008 ) ) ;
#19207=ORIENTED_EDGE ( 'NONE', *, *, #18656, .F. ) ;
#19208=EDGE_CURVE ( 'NONE', #39811, #44661, #36110, .T. ) ;
#19209=EDGE_CURVE ( 'NONE', #49503, #41529, #39993, .T. ) ;
#19211=EDGE_CURVE ( 'NONE', #9678, #39413, #32166, .T. ) ;
#19213=CARTESIAN_POINT ( 'NONE',  ( -48.47912675150885065, -175.3837268820161057, 6.938893903907228378E-15 ) ) ;
#19214=EDGE_CURVE ( 'NONE', #31341, #6500, #26993, .T. ) ;
#19216=CARTESIAN_POINT ( 'NONE',  ( -47.66663987350317200, -193.5000000000000000, -0.5829794791144634614 ) ) ;
#19217=DIRECTION ( 'NONE',  ( -0.000000000000000000, 1.000000000000000000, -0.000000000000000000 ) ) ;
#19218=ADVANCED_FACE ( 'NONE', ( #23063 ), #26475, .F. ) ;
#19221=ORIENTED_EDGE ( 'NONE', *, *, #47787, .F. ) ;
#19224=ORIENTED_EDGE ( 'NONE', *, *, #48522, .T. ) ;
#19225=DIRECTION ( 'NONE',  ( -0.000000000000000000, 1.000000000000000000, -0.000000000000000000 ) ) ;
#19226=AXIS2_PLACEMENT_3D ( 'NONE', #46763, #10751, #42028 ) ;
#19228=ORIENTED_EDGE ( 'NONE', *, *, #47422, .F. ) ;
#19229=ADVANCED_FACE ( 'NONE', ( #2571 ), #12450, .F. ) ;
#19230=CARTESIAN_POINT ( 'NONE',  ( 76.46082103836693022, -175.3837268820161057, 3.874202661595785635 ) ) ;
#19231=CARTESIAN_POINT ( 'NONE',  ( -47.53180039765466347, -183.6283474603465606, 0.3202698538628485636 ) ) ;
#19235=VERTEX_POINT ( 'NONE', #25327 ) ;
#19236=CARTESIAN_POINT ( 'NONE',  ( -78.00521078983979351, -175.3837268820161057, 121.4627941443857111 ) ) ;
#19237=VERTEX_POINT ( 'NONE', #24289 ) ;
#19238=FACE_OUTER_BOUND ( 'NONE', #9580, .T. ) ;
#19239=VERTEX_POINT ( 'NONE', #36366 ) ;
#19240=DIRECTION ( 'NONE',  ( -0.000000000000000000, -1.000000000000000000, 0.000000000000000000 ) ) ;
#19242=FACE_OUTER_BOUND ( 'NONE', #46035, .T. ) ;
#19243=CARTESIAN_POINT ( 'NONE',  ( -49.08592689732743963, -193.5000000000000000, -0.7948544414133539293 ) ) ;
#19244=ORIENTED_EDGE ( 'NONE', *, *, #11696, .F. ) ;
#19246=EDGE_CURVE ( 'NONE', #41165, #50970, #4312, .T. ) ;
#19250=PLANE ( 'NONE',  #34260 ) ;
#19251=ORIENTED_EDGE ( 'NONE', *, *, #51913, .T. ) ;
#19252=LINE ( 'NONE', #47630, #42522 ) ;
#19253=CYLINDRICAL_SURFACE ( 'NONE', #23166, 125.0000000000000000 ) ;
#19254=EDGE_CURVE ( 'NONE', #23051, #23027, #8766, .T. ) ;
#19256=ADVANCED_FACE ( 'NONE', ( #33202 ), #45320, .T. ) ;
#19257=ORIENTED_EDGE ( 'NONE', *, *, #30184, .T. ) ;
#19258=EDGE_CURVE ( 'NONE', #16764, #18124, #17465, .T. ) ;
#19261=EDGE_CURVE ( 'NONE', #21480, #35003, #24804, .T. ) ;
#19262=ORIENTED_EDGE ( 'NONE', *, *, #24652, .T. ) ;
#19263=DIRECTION ( 'NONE',  ( 0.000000000000000000, 0.000000000000000000, -1.000000000000000000 ) ) ;
#19265=CIRCLE ( 'NONE', #28462, 125.0000000000000000 ) ;
#19266=FACE_OUTER_BOUND ( 'NONE', #38225, .T. ) ;
#19268=DIRECTION ( 'NONE',  ( 0.000000000000000000, -0.000000000000000000, 1.000000000000000000 ) ) ;
#19269=EDGE_LOOP ( 'NONE', ( #10585, #52018, #4776, #10374 ) ) ;
#19271=CARTESIAN_POINT ( 'NONE',  ( -155.9608607592036833, -177.1207230881787780, 63.81752780153064464 ) ) ;
#19272=PLANE ( 'NONE',  #37345 ) ;
#19274=ADVANCED_FACE ( 'NONE', ( #40819 ), #1137, .T. ) ;
#19275=EDGE_CURVE ( 'NONE', #31327, #25704, #27398, .T. ) ;
#19277=EDGE_CURVE ( 'NONE', #21480, #12830, #5108, .T. ) ;
#19278=CARTESIAN_POINT ( 'NONE',  ( -159.8192355313504720, -193.5000000000000000, -56.81883646197830018 ) ) ;
#19279=DIRECTION ( 'NONE',  ( 0.000000000000000000, 0.000000000000000000, -1.000000000000000000 ) ) ;
#19280=DIRECTION ( 'NONE',  ( 0.9266896074318317078, 0.000000000000000000, 0.3758275821142421647 ) ) ;
#19281=ORIENTED_EDGE ( 'NONE', *, *, #5502, .F. ) ;
#19282=EDGE_CURVE ( 'NONE', #16977, #28018, #12963, .T. ) ;
#19285=EDGE_CURVE ( 'NONE', #46248, #36451, #28471, .T. ) ;
#19288=ORIENTED_EDGE ( 'NONE', *, *, #24520, .F. ) ;
#19289=VERTEX_POINT ( 'NONE', #25080 ) ;
#19290=PLANE ( 'NONE',  #34053 ) ;
#19292=CARTESIAN_POINT ( 'NONE',  ( -48.82732838694323618, -175.3837268820161057, -0.9374196611341184537 ) ) ;
#19294=LINE ( 'NONE', #7194, #25288 ) ;
#19295=CARTESIAN_POINT ( 'NONE',  ( -164.2512865680372727, -175.3837268820161057, -47.13604789772046644 ) ) ;
#19296=EDGE_LOOP ( 'NONE', ( #16165, #10718, #35579, #42822 ) ) ;
#19297=ORIENTED_EDGE ( 'NONE', *, *, #2266, .F. ) ;
#19298=ORIENTED_EDGE ( 'NONE', *, *, #1794, .F. ) ;
#19300=DIRECTION ( 'NONE',  ( 0.000000000000000000, -1.000000000000000000, 0.000000000000000000 ) ) ;
#19303=CIRCLE ( 'NONE', #48675, 125.0000000000000000 ) ;
#19305=CARTESIAN_POINT ( 'NONE',  ( -164.0008810331606526, -189.7472609257535510, 47.74645837849825369 ) ) ;
#19310=PLANE ( 'NONE',  #5468 ) ;
#19311=CARTESIAN_POINT ( 'NONE',  ( -123.4791267515088435, -173.5000000000000284, 70.00000000000000000 ) ) ;
#19312=VERTEX_POINT ( 'NONE', #20875 ) ;
#19315=EDGE_CURVE ( 'NONE', #31987, #3363, #34131, .T. ) ;
#19316=DIRECTION ( 'NONE',  ( 0.000000000000000000, 0.000000000000000000, -1.000000000000000000 ) ) ;
#19319=CARTESIAN_POINT ( 'NONE',  ( 76.04209377433248562, -193.5000000000000000, -10.93003379476866677 ) ) ;
#19320=AXIS2_PLACEMENT_3D ( 'NONE', #42424, #37964, #10366 ) ;
#19322=VERTEX_POINT ( 'NONE', #33481 ) ;
#19324=DIRECTION ( 'NONE',  ( 0.000000000000000000, 0.000000000000000000, 1.000000000000000000 ) ) ;
#19325=ORIENTED_EDGE ( 'NONE', *, *, #26989, .T. ) ;
#19329=LINE ( 'NONE', #47438, #19035 ) ;
#19330=DIRECTION ( 'NONE',  ( 0.000000000000000000, 0.000000000000000000, -1.000000000000000000 ) ) ;
#19332=VERTEX_POINT ( 'NONE', #28217 ) ;
#19333=AXIS2_PLACEMENT_3D ( 'NONE', #31750, #11246, #27789 ) ;
#19336=CARTESIAN_POINT ( 'NONE',  ( -133.8011377042516301, -183.6283474603465606, -91.35181687837437892 ) ) ;
#19338=VERTEX_POINT ( 'NONE', #22680 ) ;
#19339=CARTESIAN_POINT ( 'NONE',  ( 67.42090074966655777, -193.5000000000000000, -46.82076062204441058 ) ) ;
#19340=EDGE_CURVE ( 'NONE', #9665, #17851, #21907, .T. ) ;
#19342=ORIENTED_EDGE ( 'NONE', *, *, #30773, .T. ) ;
#19343=DIRECTION ( 'NONE',  ( -0.000000000000000000, 1.000000000000000000, -0.000000000000000000 ) ) ;
#19344=DIRECTION ( 'NONE',  ( -0.000000000000000000, 1.000000000000000000, -0.000000000000000000 ) ) ;
#19345=ORIENTED_EDGE ( 'NONE', *, *, #24963, .T. ) ;
#19346=DIRECTION ( 'NONE',  ( 0.000000000000000000, 0.000000000000000000, 1.000000000000000000 ) ) ;
#19348=DIRECTION ( 'NONE',  ( 0.000000000000000000, 1.000000000000000000, 0.000000000000000000 ) ) ;
#19350=ORIENTED_EDGE ( 'NONE', *, *, #30108, .F. ) ;
#19352=AXIS2_PLACEMENT_3D ( 'NONE', #13965, #18684, #29721 ) ;
#19353=ORIENTED_EDGE ( 'NONE', *, *, #45281, .T. ) ;
#19357=CARTESIAN_POINT ( 'NONE',  ( -171.6469053867624837, -183.6283474603465606, -14.34663989163548514 ) ) ;
#19364=ORIENTED_EDGE ( 'NONE', *, *, #45271, .F. ) ;
#19365=VECTOR ( 'NONE', #389, 1000.000000000000114 ) ;
#19366=CARTESIAN_POINT ( 'NONE',  ( -170.8336150310144887, -193.5000000000000000, 25.58083653558494319 ) ) ;
#19367=DIRECTION ( 'NONE',  ( -0.9027978299657446470, 0.000000000000000000, 0.4300652022765183435 ) ) ;
#19368=CYLINDRICAL_SURFACE ( 'NONE', #34696, 124.9999999999999858 ) ;
#19370=LINE ( 'NONE', #19882, #51117 ) ;
#19372=CARTESIAN_POINT ( 'NONE',  ( -11.17913199888832843, -193.5000000000000000, 119.3051146910914326 ) ) ;
#19373=EDGE_LOOP ( 'NONE', ( #31446, #37903, #44913, #20329 ) ) ;
#19374=VERTEX_POINT ( 'NONE', #38175 ) ;
#19375=CARTESIAN_POINT ( 'NONE',  ( -170.7635349987907603, -193.5000000000000000, -25.91377046305877130 ) ) ;
#19377=DIRECTION ( 'NONE',  ( -0.9960498426152158968, 0.000000000000000000, -0.08879589532294571153 ) ) ;
#19380=DIRECTION ( 'NONE',  ( -0.9842305779475992722, 0.000000000000000000, 0.1768902751225592818 ) ) ;
#19381=DIRECTION ( 'NONE',  ( -0.000000000000000000, 1.000000000000000000, -0.000000000000000000 ) ) ;
#19382=EDGE_LOOP ( 'NONE', ( #45076, #1371, #40195, #8287 ) ) ;
#19384=DIRECTION ( 'NONE',  ( 0.8610436117673514467, 0.000000000000000000, 0.5085311186492273983 ) ) ;
#19385=AXIS2_PLACEMENT_3D ( 'NONE', #51785, #15516, #39411 ) ;
#19386=CARTESIAN_POINT ( 'NONE',  ( -171.9128728525929262, -175.3837268820161057, 11.83705339977325011 ) ) ;
#19387=ORIENTED_EDGE ( 'NONE', *, *, #41, .F. ) ;
#19389=DIRECTION ( 'NONE',  ( -0.000000000000000000, 1.000000000000000000, -0.000000000000000000 ) ) ;
#19391=ORIENTED_EDGE ( 'NONE', *, *, #38603, .F. ) ;
#19393=EDGE_LOOP ( 'NONE', ( #23992, #44077, #5066, #3546, #9528, #43061 ) ) ;
#19394=CARTESIAN_POINT ( 'NONE',  ( 68.21542617880035664, -193.5000000000000000, 41.93543928473692972 ) ) ;
#19395=VECTOR ( 'NONE', #13470, 1000.000000000000000 ) ;
#19396=FACE_BOUND ( 'NONE', #1065, .T. ) ;
#19397=LINE ( 'NONE', #30968, #17859 ) ;
#19398=CARTESIAN_POINT ( 'NONE',  ( 58.45385938022562300, -193.5000000000000000, 62.78108192022012446 ) ) ;
#19399=VERTEX_POINT ( 'NONE', #29516 ) ;
#19400=VERTEX_POINT ( 'NONE', #45570 ) ;
#19405=EDGE_CURVE ( 'NONE', #47822, #51761, #1417, .T. ) ;
#19406=VECTOR ( 'NONE', #33290, 1000.000000000000000 ) ;
#19413=LINE ( 'NONE', #50982, #5566 ) ;
#19414=ORIENTED_EDGE ( 'NONE', *, *, #22584, .T. ) ;
#19415=FACE_OUTER_BOUND ( 'NONE', #38672, .T. ) ;
#19416=ORIENTED_EDGE ( 'NONE', *, *, #28865, .T. ) ;
#19417=EDGE_CURVE ( 'NONE', #28664, #15304, #5630, .T. ) ;
#19419=ORIENTED_EDGE ( 'NONE', *, *, #10349, .T. ) ;
#19420=DIRECTION ( 'NONE',  ( -0.9564009842765223146, 0.000000000000000000, -0.2920567706369764371 ) ) ;
#19421=DIRECTION ( 'NONE',  ( 0.000000000000000000, 1.000000000000000000, 0.000000000000000000 ) ) ;
#19423=VECTOR ( 'NONE', #35095, 1000.000000000000000 ) ;
#19424=EDGE_CURVE ( 'NONE', #25561, #45202, #6660, .T. ) ;
#19425=CARTESIAN_POINT ( 'NONE',  ( -155.4465502054561057, -183.6283474603465606, 64.67588669375881238 ) ) ;
#19427=DIRECTION ( 'NONE',  ( -0.2348860457809775482, 0.000000000000000000, -0.9720229140804121926 ) ) ;
#19428=EDGE_CURVE ( 'NONE', #4116, #11641, #33979, .T. ) ;
#19430=AXIS2_PLACEMENT_3D ( 'NONE', #43462, #18764, #30854 ) ;
#19431=DIRECTION ( 'NONE',  ( -0.000000000000000000, 1.000000000000000000, -0.000000000000000000 ) ) ;
#19433=DIRECTION ( 'NONE',  ( 0.9890401873221633666, 0.000000000000000000, 0.1476465640024850756 ) ) ;
#19435=VERTEX_POINT ( 'NONE', #10077 ) ;
#19436=CARTESIAN_POINT ( 'NONE',  ( 55.35935253854128746, -193.5000000000000000, 69.58857822035042773 ) ) ;
#19437=DIRECTION ( 'NONE',  ( 0.9995608365087942371, 0.000000000000000000, 0.02963332782256331357 ) ) ;
#19438=LINE ( 'NONE', #38893, #22919 ) ;
#19440=FACE_OUTER_BOUND ( 'NONE', #14167, .T. ) ;
#19441=DIRECTION ( 'NONE',  ( 0.000000000000000000, 0.000000000000000000, -1.000000000000000000 ) ) ;
#19443=VECTOR ( 'NONE', #29193, 1000.000000000000000 ) ;
#19444=LINE ( 'NONE', #39917, #40329 ) ;
#19450=CIRCLE ( 'NONE', #25313, 125.0000000000000000 ) ;
#19452=PLANE ( 'NONE',  #16991 ) ;
#19454=CARTESIAN_POINT ( 'NONE',  ( -68.21229068036657850, -177.1207230881787780, -123.4325817657429809 ) ) ;
#19457=ORIENTED_EDGE ( 'NONE', *, *, #32333, .T. ) ;
#19458=AXIS2_PLACEMENT_3D ( 'NONE', #17075, #28867, #44916 ) ;
#19460=VECTOR ( 'NONE', #33822, 1000.000000000000000 ) ;
#19461=ORIENTED_EDGE ( 'NONE', *, *, #32750, .F. ) ;
#19462=CARTESIAN_POINT ( 'NONE',  ( -136.1415351158078693, -175.3837268820161057, -89.10837311819173578 ) ) ;
#19463=EDGE_CURVE ( 'NONE', #17942, #42649, #26094, .T. ) ;
#19464=ADVANCED_FACE ( 'NONE', ( #13502 ), #17715, .F. ) ;
#19465=CARTESIAN_POINT ( 'NONE',  ( -140.5933766095837427, -193.5000000000000000, -84.49831343337065448 ) ) ;
#19466=VERTEX_POINT ( 'NONE', #34750 ) ;
#19469=CARTESIAN_POINT ( 'NONE',  ( -141.2664123866436512, -175.3837268820161057, -83.75869879877495805 ) ) ;
#19470=DIRECTION ( 'NONE',  ( 0.000000000000000000, 0.000000000000000000, -1.000000000000000000 ) ) ;
#19474=DIRECTION ( 'NONE',  ( 0.000000000000000000, 0.000000000000000000, 1.000000000000000000 ) ) ;
#19476=ORIENTED_EDGE ( 'NONE', *, *, #2368, .F. ) ;
#19480=DIRECTION ( 'NONE',  ( -0.000000000000000000, 1.000000000000000000, 0.000000000000000000 ) ) ;
#19481=DIRECTION ( 'NONE',  ( 0.000000000000000000, 1.000000000000000000, -0.000000000000000000 ) ) ;
#19484=VECTOR ( 'NONE', #13395, 1000.000000000000000 ) ;
#19486=LINE ( 'NONE', #10839, #12190 ) ;
#19487=EDGE_CURVE ( 'NONE', #46212, #51398, #2285, .T. ) ;
#19489=VERTEX_POINT ( 'NONE', #29771 ) ;
#19490=DIRECTION ( 'NONE',  ( 0.000000000000000000, 0.000000000000000000, 1.000000000000000000 ) ) ;
#19491=CARTESIAN_POINT ( 'NONE',  ( -41.96187976958284338, -193.5000000000000000, -123.8286356280830205 ) ) ;
#19493=VERTEX_POINT ( 'NONE', #50543 ) ;
#19495=AXIS2_PLACEMENT_3D ( 'NONE', #6862, #46555, #15265 ) ;
#19497=AXIS2_PLACEMENT_3D ( 'NONE', #41658, #42171, #6194 ) ;
#19498=ORIENTED_EDGE ( 'NONE', *, *, #44416, .F. ) ;
#19499=DIRECTION ( 'NONE',  ( -0.5829794791144820021, 0.000000000000000000, 0.8124868780056742068 ) ) ;
#19501=VECTOR ( 'NONE', #28800, 1000.000000000000000 ) ;
#19505=DIRECTION ( 'NONE',  ( 0.000000000000000000, 0.000000000000000000, 1.000000000000000000 ) ) ;
#19506=DIRECTION ( 'NONE',  ( -0.000000000000000000, 1.000000000000000000, -0.000000000000000000 ) ) ;
#19507=CARTESIAN_POINT ( 'NONE',  ( 69.66827051661184100, -193.5000000000000000, -40.81902153125260213 ) ) ;
#19509=DIRECTION ( 'NONE',  ( -0.000000000000000000, 1.000000000000000000, -0.000000000000000000 ) ) ;
#19511=DIRECTION ( 'NONE',  ( -0.000000000000000000, 1.000000000000000000, -0.000000000000000000 ) ) ;
#19515=DIRECTION ( 'NONE',  ( 0.000000000000000000, 0.000000000000000000, 1.000000000000000000 ) ) ;
#19517=DIRECTION ( 'NONE',  ( 0.000000000000000000, 0.000000000000000000, 1.000000000000000000 ) ) ;
#19518=ORIENTED_EDGE ( 'NONE', *, *, #32956, .T. ) ;
#19519=ORIENTED_EDGE ( 'NONE', *, *, #11512, .F. ) ;
#19520=CARTESIAN_POINT ( 'NONE',  ( 69.25251857196690253, -175.3837268820161057, 38.92640747825683434 ) ) ;
#19522=CYLINDRICAL_SURFACE ( 'NONE', #15829, 125.0000000000000000 ) ;
#19527=CARTESIAN_POINT ( 'NONE',  ( 5.015379008610418410, -177.1207230881787780, -112.9749434763326690 ) ) ;
#19529=ORIENTED_EDGE ( 'NONE', *, *, #37821, .T. ) ;
#19532=EDGE_CURVE ( 'NONE', #27011, #44148, #47639, .T. ) ;
#19534=DIRECTION ( 'NONE',  ( 0.5085311186492154079, 0.000000000000000000, 0.8610436117673585521 ) ) ;
#19535=CARTESIAN_POINT ( 'NONE',  ( -118.1688136093591908, -175.3837268820161057, -103.7706487676296661 ) ) ;
#19536=AXIS2_PLACEMENT_3D ( 'NONE', #10925, #23786, #15916 ) ;
#19538=VECTOR ( 'NONE', #38187, 1000.000000000000000 ) ;
#19539=EDGE_CURVE ( 'NONE', #16914, #45874, #32475, .T. ) ;
#19540=CARTESIAN_POINT ( 'NONE',  ( 51.05451324771860300, -177.1207230881787780, 75.61781872352698031 ) ) ;
#19542=ORIENTED_EDGE ( 'NONE', *, *, #35982, .F. ) ;
#19545=CIRCLE ( 'NONE', #50586, 125.0000000000000000 ) ;
#19546=EDGE_CURVE ( 'NONE', #50678, #9782, #35018, .T. ) ;
#19549=EDGE_CURVE ( 'NONE', #16711, #25060, #38358, .T. ) ;
#19550=ORIENTED_EDGE ( 'NONE', *, *, #13571, .T. ) ;
#19552=VERTEX_POINT ( 'NONE', #46868 ) ;
#19554=EDGE_CURVE ( 'NONE', #11654, #28777, #43679, .T. ) ;
#19557=CARTESIAN_POINT ( 'NONE',  ( -66.64622755927948106, -177.1207230881787780, 123.6727797384707515 ) ) ;
#19558=VECTOR ( 'NONE', #44339, 1000.000000000000000 ) ;
#19559=ADVANCED_FACE ( 'NONE', ( #11625 ), #15842, .T. ) ;
#19561=CARTESIAN_POINT ( 'NONE',  ( -145.2888470698896981, -189.7472609257535510, -77.48473115145237955 ) ) ;
#19566=ORIENTED_EDGE ( 'NONE', *, *, #5746, .T. ) ;
#19568=DIRECTION ( 'NONE',  ( 0.6749830015182142207, 0.000000000000000000, -0.7378332790417239107 ) ) ;
#19570=CYLINDRICAL_SURFACE ( 'NONE', #9751, 125.0000000000000000 ) ;
#19572=CARTESIAN_POINT ( 'NONE',  ( -151.9915035862630646, -193.5000000000000000, 70.07273251429430161 ) ) ;
#19573=AXIS2_PLACEMENT_3D ( 'NONE', #14229, #18426, #2118 ) ;
#19575=AXIS2_PLACEMENT_3D ( 'NONE', #31158, #42740, #10678 ) ;
#19579=ORIENTED_EDGE ( 'NONE', *, *, #9348, .F. ) ;
#19580=CIRCLE ( 'NONE', #50615, 125.0000000000000000 ) ;
#19582=FACE_OUTER_BOUND ( 'NONE', #1579, .T. ) ;
#19585=DIRECTION ( 'NONE',  ( -0.4031234292879730674, 0.000000000000000000, 0.9151456172430181280 ) ) ;
#19589=LINE ( 'NONE', #23793, #44411 ) ;
#19590=DIRECTION ( 'NONE',  ( 0.000000000000000000, 0.000000000000000000, -1.000000000000000000 ) ) ;
#19594=AXIS2_PLACEMENT_3D ( 'NONE', #41280, #6077, #25517 ) ;
#19595=ADVANCED_FACE ( 'NONE', ( #10850 ), #47371, .T. ) ;
#19596=EDGE_CURVE ( 'NONE', #32204, #50157, #43933, .T. ) ;
#19599=ORIENTED_EDGE ( 'NONE', *, *, #46315, .F. ) ;
#19600=ORIENTED_EDGE ( 'NONE', *, *, #27276, .T. ) ;
#19601=VECTOR ( 'NONE', #29650, 1000.000000000000000 ) ;
#19604=ADVANCED_FACE ( 'NONE', ( #7163 ), #3726, .F. ) ;
#19605=DIRECTION ( 'NONE',  ( 0.9027978299657416494, 0.000000000000000000, 0.4300652022765245608 ) ) ;
#19606=FACE_OUTER_BOUND ( 'NONE', #17863, .T. ) ;
#19607=FACE_OUTER_BOUND ( 'NONE', #28701, .T. ) ;
#19608=DIRECTION ( 'NONE',  ( 0.000000000000000000, 1.000000000000000000, 0.000000000000000000 ) ) ;
#19609=CARTESIAN_POINT ( 'NONE',  ( 72.31641062551800303, -193.5000000000000000, 32.14713283941990341 ) ) ;
#19611=VECTOR ( 'NONE', #18210, 1000.000000000000000 ) ;
#19613=ORIENTED_EDGE ( 'NONE', *, *, #43325, .T. ) ;
#19614=FACE_OUTER_BOUND ( 'NONE', #39892, .T. ) ;
#19617=EDGE_CURVE ( 'NONE', #23894, #39687, #9825, .T. ) ;
#19620=CARTESIAN_POINT ( 'NONE',  ( -36.15208382588832592, -183.6283474603465606, 123.3865623328509145 ) ) ;
#19621=DIRECTION ( 'NONE',  ( 0.000000000000000000, -0.000000000000000000, -1.000000000000000000 ) ) ;
#19623=ORIENTED_EDGE ( 'NONE', *, *, #9224, .T. ) ;
#19625=ORIENTED_EDGE ( 'NONE', *, *, #13849, .F. ) ;
#19626=EDGE_CURVE ( 'NONE', #29948, #21402, #41702, .T. ) ;
#19627=ORIENTED_EDGE ( 'NONE', *, *, #49427, .F. ) ;
#19630=DIRECTION ( 'NONE',  ( 0.9890401873221644768, 0.000000000000000000, -0.1476465640024779702 ) ) ;
#19632=VECTOR ( 'NONE', #28355, 1000.000000000000000 ) ;
#19634=FACE_OUTER_BOUND ( 'NONE', #40190, .T. ) ;
#19635=DIRECTION ( 'NONE',  ( -0.000000000000000000, 1.000000000000000000, -0.000000000000000000 ) ) ;
#19636=ORIENTED_EDGE ( 'NONE', *, *, #8160, .T. ) ;
#19637=CARTESIAN_POINT ( 'NONE',  ( -75.31296732259117732, -193.5000000000000000, -121.0625654437172614 ) ) ;
#19638=FACE_OUTER_BOUND ( 'NONE', #40612, .T. ) ;
#19639=AXIS2_PLACEMENT_3D ( 'NONE', #15966, #4380, #12527 ) ;
#19641=VERTEX_POINT ( 'NONE', #20810 ) ;
#19642=DIRECTION ( 'NONE',  ( 0.000000000000000000, -0.000000000000000000, 1.000000000000000000 ) ) ;
#19646=CIRCLE ( 'NONE', #1147, 125.0000000000000000 ) ;
#19647=ORIENTED_EDGE ( 'NONE', *, *, #47245, .F. ) ;
#19648=FACE_BOUND ( 'NONE', #10067, .T. ) ;
#19649=CARTESIAN_POINT ( 'NONE',  ( 1.150725574412418739, -189.7472609257535510, -114.7252272087845881 ) ) ;
#19651=EDGE_CURVE ( 'NONE', #14780, #25092, #29206, .T. ) ;
#19652=DIRECTION ( 'NONE',  ( -0.000000000000000000, 1.000000000000000000, -0.000000000000000000 ) ) ;
#19653=ORIENTED_EDGE ( 'NONE', *, *, #34748, .F. ) ;
#19654=ORIENTED_EDGE ( 'NONE', *, *, #20694, .T. ) ;
#19656=ORIENTED_EDGE ( 'NONE', *, *, #29160, .T. ) ;
#19658=CIRCLE ( 'NONE', #4553, 125.0000000000000000 ) ;
#19659=CARTESIAN_POINT ( 'NONE',  ( -19.51863976943889512, -189.7472609257535510, 120.5706864261536992 ) ) ;
#19660=VECTOR ( 'NONE', #23062, 1000.000000000000000 ) ;
#19663=CARTESIAN_POINT ( 'NONE',  ( -62.43888699632653783, -189.7472609257535510, 124.2180546213279371 ) ) ;
#19664=ORIENTED_EDGE ( 'NONE', *, *, #43345, .F. ) ;
#19665=CARTESIAN_POINT ( 'NONE',  ( -88.78924379339714790, -177.1207230881787780, -118.3219948448692520 ) ) ;
#19668=ORIENTED_EDGE ( 'NONE', *, *, #9328, .F. ) ;
#19669=EDGE_CURVE ( 'NONE', #44484, #20620, #45263, .T. ) ;
#19670=DIRECTION ( 'NONE',  ( -0.000000000000000000, 1.000000000000000000, -0.000000000000000000 ) ) ;
#19673=ORIENTED_EDGE ( 'NONE', *, *, #3577, .F. ) ;
#19674=CYLINDRICAL_SURFACE ( 'NONE', #38486, 124.9999999999999858 ) ;
#19678=VECTOR ( 'NONE', #19869, 1000.000000000000000 ) ;
#19679=VERTEX_POINT ( 'NONE', #33143 ) ;
#19681=ORIENTED_EDGE ( 'NONE', *, *, #8986, .F. ) ;
#19682=CARTESIAN_POINT ( 'NONE',  ( -48.47912675150885065, -189.7472609257535510, 6.938893903907228378E-15 ) ) ;
#19683=PLANE ( 'NONE',  #2189 ) ;
#19684=DIRECTION ( 'NONE',  ( 0.000000000000000000, 1.000000000000000000, -0.000000000000000000 ) ) ;
#19685=PLANE ( 'NONE',  #39145 ) ;
#19686=DIRECTION ( 'NONE',  ( 0.000000000000000000, 0.000000000000000000, 1.000000000000000000 ) ) ;
#19687=DIRECTION ( 'NONE',  ( -0.9960498426152158968, 0.000000000000000000, -0.08879589532294571153 ) ) ;
#19688=VERTEX_POINT ( 'NONE', #16344 ) ;
#19689=EDGE_CURVE ( 'NONE', #37889, #23392, #36565, .T. ) ;
#19691=CARTESIAN_POINT ( 'NONE',  ( 66.73972540229262052, -175.3837268820161057, 45.83253885719641829 ) ) ;
#19692=FACE_OUTER_BOUND ( 'NONE', #19382, .T. ) ;
#19695=VECTOR ( 'NONE', #21302, 1000.000000000000114 ) ;
#19697=DIRECTION ( 'NONE',  ( 0.7575112421616145841, 0.000000000000000000, 0.6528221181905280446 ) ) ;
#19700=ORIENTED_EDGE ( 'NONE', *, *, #2741, .F. ) ;
#19702=AXIS2_PLACEMENT_3D ( 'NONE', #15458, #50679, #47514 ) ;
#19703=EDGE_CURVE ( 'NONE', #5112, #18389, #50126, .T. ) ;
#19704=CARTESIAN_POINT ( 'NONE',  ( 75.10200014432447801, -193.5000000000000000, 10.18383939837614349 ) ) ;
#19705=DIRECTION ( 'NONE',  ( -0.000000000000000000, 1.000000000000000000, -0.000000000000000000 ) ) ;
#19706=AXIS2_PLACEMENT_3D ( 'NONE', #47290, #46769, #42553 ) ;
#19708=FACE_OUTER_BOUND ( 'NONE', #23853, .T. ) ;
#19709=VECTOR ( 'NONE', #44806, 1000.000000000000000 ) ;
#19712=CIRCLE ( 'NONE', #3775, 125.0000000000000000 ) ;
#19714=ORIENTED_EDGE ( 'NONE', *, *, #37869, .F. ) ;
#19715=VERTEX_POINT ( 'NONE', #32101 ) ;
#19718=CARTESIAN_POINT ( 'NONE',  ( 43.63512310656542326, -175.3837268820161057, 84.49831343337136502 ) ) ;
#19719=ORIENTED_EDGE ( 'NONE', *, *, #25254, .T. ) ;
#19720=PLANE ( 'NONE',  #9099 ) ;
#19726=EDGE_CURVE ( 'NONE', #779, #10952, #32630, .T. ) ;
#19727=CARTESIAN_POINT ( 'NONE',  ( -170.0502155641509319, -193.5000000000000000, -29.07697310430878090 ) ) ;
#19728=AXIS2_PLACEMENT_3D ( 'NONE', #15763, #43596, #12034 ) ;
#19729=ORIENTED_EDGE ( 'NONE', *, *, #46148, .F. ) ;
#19731=ORIENTED_EDGE ( 'NONE', *, *, #28066, .F. ) ;
#19732=AXIS2_PLACEMENT_3D ( 'NONE', #36424, #425, #31328 ) ;
#19734=CARTESIAN_POINT ( 'NONE',  ( -142.3192003680973414, -183.6283474603465606, 82.57748230379304744 ) ) ;
#19737=EDGE_CURVE ( 'NONE', #42695, #48318, #21062, .T. ) ;
#19738=EDGE_LOOP ( 'NONE', ( #8940, #9474, #42855, #19777 ) ) ;
#19739=CARTESIAN_POINT ( 'NONE',  ( 48.33059356687144970, -189.7472609257535510, 77.48473115145309009 ) ) ;
#19740=CARTESIAN_POINT ( 'NONE',  ( 141.7825277784304205, -213.5000000000000000, 41.45482488023466772 ) ) ;
#19741=DIRECTION ( 'NONE',  ( 0.1182731709213730997, 0.000000000000000000, -0.9929810960135161402 ) ) ;
#19742=ORIENTED_EDGE ( 'NONE', *, *, #35478, .T. ) ;
#19743=VECTOR ( 'NONE', #9930, 1000.000000000000114 ) ;
#19744=LINE ( 'NONE', #51833, #9819 ) ;
#19746=VECTOR ( 'NONE', #1041, 1000.000000000000000 ) ;
#19747=CARTESIAN_POINT ( 'NONE',  ( 76.47090317495664635, -189.7472609257535510, -3.534122433557455256 ) ) ;
#19748=VERTEX_POINT ( 'NONE', #32876 ) ;
#19749=FACE_OUTER_BOUND ( 'NONE', #9143, .T. ) ;
#19750=VECTOR ( 'NONE', #2370, 1000.000000000000000 ) ;
#19753=ORIENTED_EDGE ( 'NONE', *, *, #20244, .T. ) ;
#19754=DIRECTION ( 'NONE',  ( 0.000000000000000000, 1.000000000000000000, 0.000000000000000000 ) ) ;
#19756=FACE_OUTER_BOUND ( 'NONE', #51469, .T. ) ;
#19757=DIRECTION ( 'NONE',  ( 0.000000000000000000, 0.000000000000000000, -1.000000000000000000 ) ) ;
#19758=CARTESIAN_POINT ( 'NONE',  ( 17.15229921100055321, -177.1207230881787780, -106.3838142112212779 ) ) ;
#19759=EDGE_CURVE ( 'NONE', #19237, #42041, #47606, .T. ) ;
#19760=CARTESIAN_POINT ( 'NONE',  ( 15.29189835570547551, -193.5000000000000000, 106.3450133598704213 ) ) ;
#19764=AXIS2_PLACEMENT_3D ( 'NONE', #46228, #22813, #2835 ) ;
#19765=DIRECTION ( 'NONE',  ( -0.02963332782255633305, 0.000000000000000000, -0.9995608365087944591 ) ) ;
#19766=DIRECTION ( 'NONE',  ( -0.000000000000000000, 1.000000000000000000, -0.000000000000000000 ) ) ;
#19767=DIRECTION ( 'NONE',  ( 0.000000000000000000, 0.000000000000000000, 1.000000000000000000 ) ) ;
#19769=CIRCLE ( 'NONE', #49992, 125.0000000000000000 ) ;
#19770=VECTOR ( 'NONE', #26557, 1000.000000000000114 ) ;
#19771=ORIENTED_EDGE ( 'NONE', *, *, #31630, .T. ) ;
#19773=ADVANCED_FACE ( 'NONE', ( #1082 ), #40239, .T. ) ;
#19774=EDGE_CURVE ( 'NONE', #49340, #6620, #44994, .T. ) ;
#19775=DIRECTION ( 'NONE',  ( -0.000000000000000000, 1.000000000000000000, -0.000000000000000000 ) ) ;
#19776=VERTEX_POINT ( 'NONE', #36050 ) ;
#19777=ORIENTED_EDGE ( 'NONE', *, *, #23713, .T. ) ;
#19778=EDGE_CURVE ( 'NONE', #6620, #19239, #25431, .T. ) ;
#19779=CIRCLE ( 'NONE', #3856, 125.0000000000000000 ) ;
#19780=VERTEX_POINT ( 'NONE', #48147 ) ;
#19784=EDGE_CURVE ( 'NONE', #18133, #10779, #4254, .T. ) ;
#19785=CARTESIAN_POINT ( 'NONE',  ( 1.150725574412418739, -189.7472609257535510, -114.7252272087845881 ) ) ;
#19786=VECTOR ( 'NONE', #39963, 1000.000000000000114 ) ;
#19787=DIRECTION ( 'NONE',  ( 1.000000000000000000, -0.000000000000000000, 6.978251959525016136E-17 ) ) ;
#19788=VERTEX_POINT ( 'NONE', #4519 ) ;
#19789=EDGE_LOOP ( 'NONE', ( #220, #3003, #8518, #22082 ) ) ;
#19796=DIRECTION ( 'NONE',  ( -0.5085311186492273983, 0.000000000000000000, 0.8610436117673514467 ) ) ;
#19799=LINE ( 'NONE', #51888, #45809 ) ;
#19801=VERTEX_POINT ( 'NONE', #22102 ) ;
#19802=ORIENTED_EDGE ( 'NONE', *, *, #40156, .T. ) ;
#19804=LINE ( 'NONE', #7981, #42434 ) ;
#19805=AXIS2_PLACEMENT_3D ( 'NONE', #41472, #38309, #17834 ) ;
#19806=CARTESIAN_POINT ( 'NONE',  ( -47.87232660569026166, -183.6283474603465606, 0.7948544414133635883 ) ) ;
#19808=CARTESIAN_POINT ( 'NONE',  ( 70.19984492582109681, -175.3837268820161057, 39.24667733211968823 ) ) ;
#19809=AXIS2_PLACEMENT_3D ( 'NONE', #2627, #30236, #18414 ) ;
#19810=VECTOR ( 'NONE', #31577, 1000.000000000000114 ) ;
#19811=DIRECTION ( 'NONE',  ( -0.000000000000000000, 1.000000000000000000, -0.000000000000000000 ) ) ;
#19812=CARTESIAN_POINT ( 'NONE',  ( -49.21696003055057389, -175.3837268820161057, -0.6749830015182127774 ) ) ;
#19815=ORIENTED_EDGE ( 'NONE', *, *, #32115, .T. ) ;
#19816=CARTESIAN_POINT ( 'NONE',  ( -167.6453766917639427, -177.1207230881787780, 37.74128873232410086 ) ) ;
#19817=CYLINDRICAL_SURFACE ( 'NONE', #22118, 125.0000000000000000 ) ;
#19818=VECTOR ( 'NONE', #13521, 1000.000000000000000 ) ;
#19819=CARTESIAN_POINT ( 'NONE',  ( -66.64622755927948106, -177.1207230881787780, 123.6727797384707515 ) ) ;
#19824=DIRECTION ( 'NONE',  ( -0.000000000000000000, 1.000000000000000000, -0.000000000000000000 ) ) ;
#19825=EDGE_CURVE ( 'NONE', #35, #4302, #247, .T. ) ;
#19826=CARTESIAN_POINT ( 'NONE',  ( 67.29469129333651267, -183.6283474603465606, -44.41421852208627996 ) ) ;
#19828=EDGE_CURVE ( 'NONE', #37488, #48517, #34646, .T. ) ;
#19829=VECTOR ( 'NONE', #50379, 1000.000000000000000 ) ;
#19830=CARTESIAN_POINT ( 'NONE',  ( -91.84482189527193441, -175.3837268820161057, -117.2365833888816553 ) ) ;
#19832=ORIENTED_EDGE ( 'NONE', *, *, #38305, .F. ) ;
#19835=ORIENTED_EDGE ( 'NONE', *, *, #47844, .T. ) ;
#19836=ORIENTED_EDGE ( 'NONE', *, *, #7513, .T. ) ;
#19837=ADVANCED_FACE ( 'NONE', ( #46292 ), #22360, .T. ) ;
#19839=CARTESIAN_POINT ( 'NONE',  ( 67.66641500972446011, -189.7472609257535510, 46.20836643931067300 ) ) ;
#19841=ADVANCED_FACE ( 'NONE', ( #2395 ), #41819, .T. ) ;
#19842=VERTEX_POINT ( 'NONE', #5840 ) ;
#19843=CARTESIAN_POINT ( 'NONE',  ( 21.49274850782854074, -175.3837268820161057, -103.5805805771126700 ) ) ;
#19844=EDGE_CURVE ( 'NONE', #22714, #5997, #17907, .T. ) ;
#19845=EDGE_CURVE ( 'NONE', #30580, #22041, #29456, .T. ) ;
#19846=FACE_OUTER_BOUND ( 'NONE', #12592, .T. ) ;
#19850=CARTESIAN_POINT ( 'NONE',  ( 57.31108707223382481, -193.5000000000000000, -66.58401203837755133 ) ) ;
#19852=EDGE_LOOP ( 'NONE', ( #5421, #3926, #32550, #31090 ) ) ;
#19855=AXIS2_PLACEMENT_3D ( 'NONE', #33828, #51181, #36155 ) ;
#19857=LINE ( 'NONE', #32721, #38669 ) ;
#19859=ORIENTED_EDGE ( 'NONE', *, *, #43907, .F. ) ;
#19860=ORIENTED_EDGE ( 'NONE', *, *, #32422, .F. ) ;
#19861=ORIENTED_EDGE ( 'NONE', *, *, #24700, .F. ) ;
#19864=AXIS2_PLACEMENT_3D ( 'NONE', #43424, #38683, #30809 ) ;
#19866=DIRECTION ( 'NONE',  ( 0.8455960035018311727, 0.000000000000000000, -0.5338233779647826305 ) ) ;
#19869=DIRECTION ( 'NONE',  ( -0.000000000000000000, 1.000000000000000000, -0.000000000000000000 ) ) ;
#19871=VECTOR ( 'NONE', #9590, 1000.000000000000114 ) ;
#19873=VECTOR ( 'NONE', #43346, 1000.000000000000000 ) ;
#19874=DIRECTION ( 'NONE',  ( -0.4566292373937018145, 0.000000000000000000, -0.8896570909947529859 ) ) ;
#19875=ORIENTED_EDGE ( 'NONE', *, *, #9317, .T. ) ;
#19876=DIRECTION ( 'NONE',  ( -0.8124868780056783146, 0.000000000000000000, -0.5829794791144762289 ) ) ;
#19877=ORIENTED_EDGE ( 'NONE', *, *, #45602, .T. ) ;
#19878=ORIENTED_EDGE ( 'NONE', *, *, #38110, .T. ) ;
#19879=CARTESIAN_POINT ( 'NONE',  ( -70.75782287548091176, -175.3837268820161057, 122.9986166548864901 ) ) ;
#19880=CARTESIAN_POINT ( 'NONE',  ( -87.88805327685030022, -183.6283474603465606, 117.5715283571807106 ) ) ;
#19882=CARTESIAN_POINT ( 'NONE',  ( -163.4524646452520926, -193.5000000000000000, 46.44493303993097300 ) ) ;
#19883=ORIENTED_EDGE ( 'NONE', *, *, #23780, .T. ) ;
#19884=CARTESIAN_POINT ( 'NONE',  ( -11.17913199888832843, -189.7472609257535510, 119.3051146910914326 ) ) ;
#19885=ORIENTED_EDGE ( 'NONE', *, *, #11773, .T. ) ;
#19887=ORIENTED_EDGE ( 'NONE', *, *, #46863, .F. ) ;
#19888=AXIS2_PLACEMENT_3D ( 'NONE', #3542, #7236, #39291 ) ;
#19889=VECTOR ( 'NONE', #5053, 1000.000000000000000 ) ;
#19890=PLANE ( 'NONE',  #25709 ) ;
#19891=LINE ( 'NONE', #3870, #48261 ) ;
#19893=ADVANCED_FACE ( 'NONE', ( #10273 ), #14486, .T. ) ;
#19894=EDGE_CURVE ( 'NONE', #3648, #24784, #45763, .T. ) ;
#19895=CARTESIAN_POINT ( 'NONE',  ( -169.6464974000608379, -175.3837268820161057, 26.35287080855539088 ) ) ;
#19896=CYLINDRICAL_SURFACE ( 'NONE', #42158, 125.0000000000000000 ) ;
#19901=ADVANCED_FACE ( 'NONE', ( #26289 ), #37346, .F. ) ;
#19902=FACE_BOUND ( 'NONE', #16925, .T. ) ;
#19903=ORIENTED_EDGE ( 'NONE', *, *, #51636, .T. ) ;
#19905=CIRCLE ( 'NONE', #28300, 125.0000000000000000 ) ;
#19907=VECTOR ( 'NONE', #50011, 1000.000000000000000 ) ;
#19909=ORIENTED_EDGE ( 'NONE', *, *, #4144, .T. ) ;
#19910=DIRECTION ( 'NONE',  ( 0.000000000000000000, 0.000000000000000000, 1.000000000000000000 ) ) ;
#19912=VERTEX_POINT ( 'NONE', #31012 ) ;
#19914=FACE_OUTER_BOUND ( 'NONE', #26215, .T. ) ;
#19915=EDGE_CURVE ( 'NONE', #4854, #48288, #35460, .T. ) ;
#19916=FACE_BOUND ( 'NONE', #16155, .T. ) ;
#19917=PLANE ( 'NONE',  #50612 ) ;
#19918=ORIENTED_EDGE ( 'NONE', *, *, #23774, .T. ) ;
#19919=EDGE_CURVE ( 'NONE', #20876, #4233, #19438, .T. ) ;
#19921=VERTEX_POINT ( 'NONE', #51263 ) ;
#19922=EDGE_CURVE ( 'NONE', #32747, #37279, #7105, .T. ) ;
#19923=ORIENTED_EDGE ( 'NONE', *, *, #7051, .F. ) ;
#19924=LINE ( 'NONE', #16245, #35128 ) ;
#19927=ORIENTED_EDGE ( 'NONE', *, *, #48803, .F. ) ;
#19928=CARTESIAN_POINT ( 'NONE',  ( -73.70588833648351113, -193.5000000000000000, 121.4073237908568359 ) ) ;
#19929=CARTESIAN_POINT ( 'NONE',  ( -48.47912675150885065, -177.1207230881787780, 6.938893903907228378E-15 ) ) ;
#19933=ORIENTED_EDGE ( 'NONE', *, *, #3995, .F. ) ;
#19934=CARTESIAN_POINT ( 'NONE',  ( -150.5215542367829471, -189.7472609257535510, -72.19655804061974891 ) ) ;
#19936=EDGE_LOOP ( 'NONE', ( #33633, #28807, #22547, #16969 ) ) ;
#19937=AXIS2_PLACEMENT_3D ( 'NONE', #41899, #31095, #2723 ) ;
#19938=ORIENTED_EDGE ( 'NONE', *, *, #18313, .T. ) ;
#19940=VECTOR ( 'NONE', #41144, 1000.000000000000341 ) ;
#19943=LINE ( 'NONE', #20195, #50779 ) ;
#19944=ORIENTED_EDGE ( 'NONE', *, *, #37514, .F. ) ;
#19945=AXIS2_PLACEMENT_3D ( 'NONE', #27314, #10782, #3402 ) ;
#19946=DIRECTION ( 'NONE',  ( 0.000000000000000000, 0.000000000000000000, 1.000000000000000000 ) ) ;
#19947=EDGE_LOOP ( 'NONE', ( #39515, #8117 ) ) ;
#19950=ORIENTED_EDGE ( 'NONE', *, *, #14700, .F. ) ;
#19951=AXIS2_PLACEMENT_3D ( 'NONE', #33113, #16848, #36807 ) ;
#19952=VERTEX_POINT ( 'NONE', #23140 ) ;
#19954=CARTESIAN_POINT ( 'NONE',  ( -172.2289551866394106, -193.5000000000000000, -17.63462396184707970 ) ) ;
#19956=PLANE ( 'NONE',  #4012 ) ;
#19960=EDGE_CURVE ( 'NONE', #11395, #32749, #3623, .T. ) ;
#19961=ADVANCED_FACE ( 'NONE', ( #39154 ), #3410, .T. ) ;
#19963=CARTESIAN_POINT ( 'NONE',  ( 72.14504940832446778, -193.5000000000000000, -32.78426643622660208 ) ) ;
#19964=LINE ( 'NONE', #51780, #39900 ) ;
#19965=DIRECTION ( 'NONE',  ( 0.9720229140804089729, 0.000000000000000000, 0.2348860457809911206 ) ) ;
#19970=VECTOR ( 'NONE', #38719, 1000.000000000000000 ) ;
#19972=CARTESIAN_POINT ( 'NONE',  ( -65.65563056894596627, -183.6283474603465606, 123.8142468240612999 ) ) ;
#19975=VERTEX_POINT ( 'NONE', #15787 ) ;
#19976=AXIS2_PLACEMENT_3D ( 'NONE', #31355, #23729, #27925 ) ;
#19977=DIRECTION ( 'NONE',  ( 0.8610436117673514467, 0.000000000000000000, 0.5085311186492273983 ) ) ;
#19978=DIRECTION ( 'NONE',  ( 0.4031234292879665171, 0.000000000000000000, 0.9151456172430210145 ) ) ;
#19979=EDGE_CURVE ( 'NONE', #32000, #32301, #47317, .T. ) ;
#19982=ORIENTED_EDGE ( 'NONE', *, *, #41070, .F. ) ;
#19984=EDGE_CURVE ( 'NONE', #36830, #43678, #22097, .T. ) ;
#19985=VECTOR ( 'NONE', #28327, 1000.000000000000000 ) ;
#19988=ORIENTED_EDGE ( 'NONE', *, *, #32339, .F. ) ;
#19989=DIRECTION ( 'NONE',  ( 0.000000000000000000, 0.000000000000000000, 1.000000000000000000 ) ) ;
#19991=DIRECTION ( 'NONE',  ( 0.9473263538541876194, 0.000000000000000000, 0.3202698538628486746 ) ) ;
#19992=DIRECTION ( 'NONE',  ( -0.000000000000000000, 1.000000000000000000, -0.000000000000000000 ) ) ;
#19993=AXIS2_PLACEMENT_3D ( 'NONE', #38681, #26083, #2944 ) ;
#19994=CARTESIAN_POINT ( 'NONE',  ( -49.40581635894068313, -189.7472609257535510, -0.3758275821142418316 ) ) ;
#19997=VECTOR ( 'NONE', #7740, 1000.000000000000000 ) ;
#19998=VECTOR ( 'NONE', #25237, 1000.000000000000000 ) ;
#20001=CARTESIAN_POINT ( 'NONE',  ( -48.47912675150883643, -189.7472609257535510, -125.0000000000000000 ) ) ;
#20002=AXIS2_PLACEMENT_3D ( 'NONE', #39675, #28382, #48109 ) ;
#20003=EDGE_LOOP ( 'NONE', ( #13719, #35136, #13982, #6551 ) ) ;
#20006=FACE_OUTER_BOUND ( 'NONE', #17268, .T. ) ;
#20007=LINE ( 'NONE', #39202, #26499 ) ;
#20008=ORIENTED_EDGE ( 'NONE', *, *, #26463, .F. ) ;
#20016=CARTESIAN_POINT ( 'NONE',  ( -48.47912675150885065, -189.7472609257535510, 6.938893903907228378E-15 ) ) ;
#20017=CARTESIAN_POINT ( 'NONE',  ( -127.4665351220365892, -177.1207230881787780, -96.88131563365291754 ) ) ;
#20018=ORIENTED_EDGE ( 'NONE', *, *, #20873, .F. ) ;
#20019=EDGE_CURVE ( 'NONE', #3372, #13063, #14527, .T. ) ;
#20022=AXIS2_PLACEMENT_3D ( 'NONE', #4694, #8378, #44638 ) ;
#20023=ORIENTED_EDGE ( 'NONE', *, *, #31937, .T. ) ;
#20024=CARTESIAN_POINT ( 'NONE',  ( 76.43863189440992301, -175.3837268820161057, -4.533605064403313456 ) ) ;
#20025=ORIENTED_EDGE ( 'NONE', *, *, #13441, .F. ) ;
#20026=EDGE_CURVE ( 'NONE', #7370, #26319, #19198, .T. ) ;
#20028=DIRECTION ( 'NONE',  ( 0.000000000000000000, 1.000000000000000000, 0.000000000000000000 ) ) ;
#20030=CARTESIAN_POINT ( 'NONE',  ( -48.24424070572786860, -189.7472609257535510, -0.9720229140804037549 ) ) ;
#20031=DIRECTION ( 'NONE',  ( -0.9982437317643214625, 0.000000000000000000, -0.05924062789371441901 ) ) ;
#20033=VECTOR ( 'NONE', #14800, 1000.000000000000000 ) ;
#20035=CARTESIAN_POINT ( 'NONE',  ( -47.97059563285963435, -193.5000000000000000, 0.8610436117673654355 ) ) ;
#20036=EDGE_CURVE ( 'NONE', #6126, #20552, #50610, .T. ) ;
#20037=CYLINDRICAL_SURFACE ( 'NONE', #3754, 125.0000000000000000 ) ;
#20038=DIRECTION ( 'NONE',  ( -0.8124868780056742068, 0.000000000000000000, -0.5829794791144820021 ) ) ;
#20039=VERTEX_POINT ( 'NONE', #51011 ) ;
#20040=CIRCLE ( 'NONE', #13336, 125.0000000000000000 ) ;
#20041=ORIENTED_EDGE ( 'NONE', *, *, #25265, .T. ) ;
#20043=CARTESIAN_POINT ( 'NONE',  ( -49.29161362951453640, -193.5000000000000000, 0.5829794791144718991 ) ) ;
#20045=AXIS2_PLACEMENT_3D ( 'NONE', #5718, #1754, #41433 ) ;
#20046=ORIENTED_EDGE ( 'NONE', *, *, #23052, .F. ) ;
#20047=ORIENTED_EDGE ( 'NONE', *, *, #1601, .T. ) ;
#20048=DIRECTION ( 'NONE',  ( 0.000000000000000000, 0.000000000000000000, -1.000000000000000000 ) ) ;
#20049=DIRECTION ( 'NONE',  ( 0.9890401873221623674, 0.000000000000000000, 0.1476465640024917925 ) ) ;
#20050=LINE ( 'NONE', #51873, #6014 ) ;
#20051=DIRECTION ( 'NONE',  ( 0.000000000000000000, 0.000000000000000000, -1.000000000000000000 ) ) ;
#20053=EDGE_LOOP ( 'NONE', ( #20610, #27981, #35047, #7122 ) ) ;
#20055=VECTOR ( 'NONE', #19118, 1000.000000000000227 ) ;
#20056=CARTESIAN_POINT ( 'NONE',  ( 51.65665342072241373, -177.1207230881787780, 74.81861753132420745 ) ) ;
#20057=PLANE ( 'NONE',  #26024 ) ;
#20059=DIRECTION ( 'NONE',  ( 0.000000000000000000, -0.000000000000000000, 1.000000000000000000 ) ) ;
#20061=VERTEX_POINT ( 'NONE', #46802 ) ;
#20066=CARTESIAN_POINT ( 'NONE',  ( -111.3295483157475445, -193.5000000000000000, 108.0501018472332504 ) ) ;
#20067=EDGE_CURVE ( 'NONE', #49029, #3029, #20396, .T. ) ;
#20068=ORIENTED_EDGE ( 'NONE', *, *, #19275, .F. ) ;
#20071=PLANE ( 'NONE',  #45790 ) ;
#20072=DIRECTION ( 'NONE',  ( 0.6965510290629932655, 0.000000000000000000, 0.7175072570443347120 ) ) ;
#20076=COLOUR_RGB ( '', 0.09019608, 0.27058824, 0.51372549) ;
#20077=DIRECTION ( 'NONE',  ( 0.000000000000000000, -0.000000000000000000, -1.000000000000000000 ) ) ;
#20078=DIRECTION ( 'NONE',  ( 0.5586467658036415873, 0.000000000000000000, 0.8294056854502090959 ) ) ;
#20082=ADVANCED_FACE ( 'NONE', ( #19692 ), #39653, .T. ) ;
#20084=VERTEX_POINT ( 'NONE', #43099 ) ;
#20085=CARTESIAN_POINT ( 'NONE',  ( 70.68712318874649725, -193.5000000000000000, -37.74128873232327663 ) ) ;
#20089=DIRECTION ( 'NONE',  ( 0.000000000000000000, 1.000000000000000000, -0.000000000000000000 ) ) ;
#20092=DIRECTION ( 'NONE',  ( 0.000000000000000000, -0.000000000000000000, 1.000000000000000000 ) ) ;
#20094=CARTESIAN_POINT ( 'NONE',  ( -169.9131040279660567, -183.6283474603465606, 29.64437826672833864 ) ) ;
#20098=ORIENTED_EDGE ( 'NONE', *, *, #46858, .T. ) ;
#20099=EDGE_LOOP ( 'NONE', ( #29940, #33579, #8228, #32092 ) ) ;
#20101=DIRECTION ( 'NONE',  ( 0.000000000000000000, -0.000000000000000000, -1.000000000000000000 ) ) ;
#20102=ORIENTED_EDGE ( 'NONE', *, *, #3213, .F. ) ;
#20103=ORIENTED_EDGE ( 'NONE', *, *, #16335, .F. ) ;
#20104=DIRECTION ( 'NONE',  ( 0.000000000000000000, 0.000000000000000000, 1.000000000000000000 ) ) ;
#20105=PLANE ( 'NONE',  #11702 ) ;
#20107=CIRCLE ( 'NONE', #5847, 125.0000000000000000 ) ;
#20109=LINE ( 'NONE', #32192, #28678 ) ;
#20111=CARTESIAN_POINT ( 'NONE',  ( 47.04848625005566731, -183.6283474603465606, 80.61932246194658092 ) ) ;
#20112=CARTESIAN_POINT ( 'NONE',  ( -48.47912675150885065, -175.3837268820161057, 6.938893903907228378E-15 ) ) ;
#20113=FACE_OUTER_BOUND ( 'NONE', #48483, .T. ) ;
#20116=EDGE_LOOP ( 'NONE', ( #51617, #48604, #32705, #21517 ) ) ;
#20117=ORIENTED_EDGE ( 'NONE', *, *, #38493, .T. ) ;
#20120=FACE_OUTER_BOUND ( 'NONE', #5482, .T. ) ;
#20124=ADVANCED_FACE ( 'NONE', ( #16558 ), #48344, .T. ) ;
#20125=EDGE_CURVE ( 'NONE', #41700, #25155, #44409, .T. ) ;
#20126=ADVANCED_FACE ( 'NONE', ( #4715 ), #40688, .T. ) ;
#20129=DIRECTION ( 'NONE',  ( 0.000000000000000000, 1.000000000000000000, -0.000000000000000000 ) ) ;
#20130=ORIENTED_EDGE ( 'NONE', *, *, #2947, .T. ) ;
#20131=DIRECTION ( 'NONE',  ( 0.000000000000000000, 1.000000000000000000, 0.000000000000000000 ) ) ;
#20135=CARTESIAN_POINT ( 'NONE',  ( -47.66663987350317910, -193.5000000000000000, 0.5829794791144832233 ) ) ;
#20136=EDGE_CURVE ( 'NONE', #33417, #47120, #18721, .T. ) ;
#20137=FACE_OUTER_BOUND ( 'NONE', #14316, .T. ) ;
#20140=VERTEX_POINT ( 'NONE', #28086 ) ;
#20141=EDGE_CURVE ( 'NONE', #51271, #8740, #31310, .T. ) ;
#20142=DIRECTION ( 'NONE',  ( 0.000000000000000000, -1.000000000000000000, 0.000000000000000000 ) ) ;
#20143=VERTEX_POINT ( 'NONE', #24176 ) ;
#20144=EDGE_CURVE ( 'NONE', #19332, #11775, #49792, .T. ) ;
#20145=ORIENTED_EDGE ( 'NONE', *, *, #6285, .T. ) ;
#20146=DIRECTION ( 'NONE',  ( 0.000000000000000000, 0.000000000000000000, 1.000000000000000000 ) ) ;
#20147=EDGE_CURVE ( 'NONE', #13215, #32692, #16207, .T. ) ;
#20148=VECTOR ( 'NONE', #10543, 1000.000000000000114 ) ;
#20150=DIRECTION ( 'NONE',  ( 0.000000000000000000, -1.000000000000000000, 0.000000000000000000 ) ) ;
#20153=CARTESIAN_POINT ( 'NONE',  ( -5.113431607746556473, -175.3837268820161057, 117.2365833888819679 ) ) ;
#20155=CARTESIAN_POINT ( 'NONE',  ( -153.7737137892885073, -189.7472609257535510, -65.49088066501643368 ) ) ;
#20157=FACE_BOUND ( 'NONE', #45741, .T. ) ;
#20159=DIRECTION ( 'NONE',  ( 0.000000000000000000, 0.000000000000000000, -1.000000000000000000 ) ) ;
#20160=CARTESIAN_POINT ( 'NONE',  ( -49.25565061422690150, -189.7472609257535510, 0.6300878435817109935 ) ) ;
#20161=ORIENTED_EDGE ( 'NONE', *, *, #29663, .T. ) ;
#20163=ORIENTED_EDGE ( 'NONE', *, *, #11956, .T. ) ;
#20164=ADVANCED_FACE ( 'NONE', ( #12059 ), #24679, .T. ) ;
#20165=VECTOR ( 'NONE', #599, 1000.000000000000000 ) ;
#20166=VECTOR ( 'NONE', #41546, 1000.000000000000000 ) ;
#20167=CARTESIAN_POINT ( 'NONE',  ( -158.3442440847887269, -193.5000000000000000, -59.62093586438114556 ) ) ;
#20168=FACE_BOUND ( 'NONE', #13408, .T. ) ;
#20169=DIRECTION ( 'NONE',  ( 0.000000000000000000, 1.000000000000000000, 0.000000000000000000 ) ) ;
#20171=CARTESIAN_POINT ( 'NONE',  ( -21.46839590530488451, -193.5000000000000000, 122.0467960216650738 ) ) ;
#20172=ORIENTED_EDGE ( 'NONE', *, *, #29455, .T. ) ;
#20173=EDGE_LOOP ( 'NONE', ( #19221, #7679, #37925, #47216 ) ) ;
#20174=EDGE_CURVE ( 'NONE', #42501, #13947, #37025, .T. ) ;
#20176=VECTOR ( 'NONE', #19652, 1000.000000000000000 ) ;
#20177=ORIENTED_EDGE ( 'NONE', *, *, #10895, .F. ) ;
#20179=CARTESIAN_POINT ( 'NONE',  ( 67.87295084395105960, -177.1207230881787780, 42.87565520599286373 ) ) ;
#20182=EDGE_CURVE ( 'NONE', #35111, #17063, #33083, .T. ) ;
#20186=FACE_OUTER_BOUND ( 'NONE', #44837, .T. ) ;
#20190=EDGE_LOOP ( 'NONE', ( #10435, #26782, #37687, #13821 ) ) ;
#20191=ORIENTED_EDGE ( 'NONE', *, *, #6409, .T. ) ;
#20192=EDGE_CURVE ( 'NONE', #15949, #45202, #28872, .T. ) ;
#20193=DIRECTION ( 'NONE',  ( -0.000000000000000000, 1.000000000000000000, -0.000000000000000000 ) ) ;
#20195=CARTESIAN_POINT ( 'NONE',  ( -173.4724443937511751, -193.5000000000000000, 1.292495564989516454 ) ) ;
#20197=VERTEX_POINT ( 'NONE', #21528 ) ;
#20198=DIRECTION ( 'NONE',  ( 0.9151456172430153524, 0.000000000000000000, 0.4031234292879792847 ) ) ;
#20200=EDGE_CURVE ( 'NONE', #32592, #50673, #41759, .T. ) ;
#20201=PLANE ( 'NONE',  #6543 ) ;
#20202=CARTESIAN_POINT ( 'NONE',  ( -134.2540868116286958, -189.7472609257535510, 89.54698061029652933 ) ) ;
#20206=CIRCLE ( 'NONE', #3429, 125.0000000000000000 ) ;
#20207=ORIENTED_EDGE ( 'NONE', *, *, #51956, .F. ) ;
#20210=EDGE_CURVE ( 'NONE', #9746, #41712, #5248, .T. ) ;
#20212=CARTESIAN_POINT ( 'NONE',  ( 48.69345348225014902, -175.3837268820161057, -78.62880929222872339 ) ) ;
#20213=CARTESIAN_POINT ( 'NONE',  ( -107.6930423737362190, -183.6283474603465606, 110.0850225811110761 ) ) ;
#20215=EDGE_CURVE ( 'NONE', #48966, #28239, #22035, .T. ) ;
#20218=CARTESIAN_POINT ( 'NONE',  ( -173.0003472773501301, -189.7472609257535510, 10.93003379476953896 ) ) ;
#20219=PLANE ( 'NONE',  #3840 ) ;
#20220=EDGE_CURVE ( 'NONE', #12568, #2342, #18189, .T. ) ;
#20221=DIRECTION ( 'NONE',  ( 0.7765238627180349740, 0.000000000000000000, 0.6300878435817203194 ) ) ;
#20225=LINE ( 'NONE', #28876, #42860 ) ;
#20227=ORIENTED_EDGE ( 'NONE', *, *, #25178, .F. ) ;
#20228=ORIENTED_EDGE ( 'NONE', *, *, #30897, .F. ) ;
#20229=ORIENTED_EDGE ( 'NONE', *, *, #7635, .F. ) ;
#20230=EDGE_CURVE ( 'NONE', #1228, #30377, #10606, .T. ) ;
#20231=EDGE_CURVE ( 'NONE', #25977, #44982, #37801, .T. ) ;
#20233=DIRECTION ( 'NONE',  ( 0.7948544414133565938, 0.000000000000000000, -0.6068001458185890984 ) ) ;
#20234=LINE ( 'NONE', #39422, #11115 ) ;
#20235=LINE ( 'NONE', #24970, #1038 ) ;
#20237=ORIENTED_EDGE ( 'NONE', *, *, #36577, .F. ) ;
#20239=EDGE_LOOP ( 'NONE', ( #29190, #22818, #10532, #51371 ) ) ;
#20242=ORIENTED_EDGE ( 'NONE', *, *, #19059, .F. ) ;
#20243=DIRECTION ( 'NONE',  ( 0.000000000000000000, -1.000000000000000000, 0.000000000000000000 ) ) ;
#20244=EDGE_CURVE ( 'NONE', #46197, #27750, #25724, .T. ) ;
#20245=EDGE_CURVE ( 'NONE', #50634, #8813, #49393, .T. ) ;
#20246=ORIENTED_EDGE ( 'NONE', *, *, #18302, .F. ) ;
#20248=DIRECTION ( 'NONE',  ( 0.000000000000000000, 1.000000000000000000, -0.000000000000000000 ) ) ;
#20250=CARTESIAN_POINT ( 'NONE',  ( -105.2524431885210987, -193.5000000000000000, 110.2396968984195382 ) ) ;
#20251=DIRECTION ( 'NONE',  ( -0.000000000000000000, 1.000000000000000000, -0.000000000000000000 ) ) ;
#20252=VERTEX_POINT ( 'NONE', #41220 ) ;
#20253=CIRCLE ( 'NONE', #42909, 125.0000000000000000 ) ;
#20256=CARTESIAN_POINT ( 'NONE',  ( 74.28166149629942083, -175.3837268820161057, 17.48697739784543259 ) ) ;
#20258=FACE_OUTER_BOUND ( 'NONE', #29873, .T. ) ;
#20260=PLANE ( 'NONE',  #40872 ) ;
#20261=CARTESIAN_POINT ( 'NONE',  ( 17.98688506184922176, -193.5000000000000000, 104.6823626202124586 ) ) ;
#20263=LINE ( 'NONE', #11334, #6382 ) ;
#20264=LINE ( 'NONE', #40485, #39574 ) ;
#20267=DIRECTION ( 'NONE',  ( 0.8757349421956345248, 0.000000000000000000, 0.4827922027307490205 ) ) ;
#20268=CARTESIAN_POINT ( 'NONE',  ( -48.24424070572786860, -175.3837268820161057, -0.9720229140804037549 ) ) ;
#20272=CARTESIAN_POINT ( 'NONE',  ( -103.4012653778457462, -193.5000000000000000, -112.2878385610366649 ) ) ;
#20278=ORIENTED_EDGE ( 'NONE', *, *, #51904, .T. ) ;
#20280=CARTESIAN_POINT ( 'NONE',  ( -49.44376233341721161, -193.5000000000000000, 0.2635871660690650709 ) ) ;
#20282=CARTESIAN_POINT ( 'NONE',  ( -82.67254833784559764, -193.5000000000000000, -120.2323164553483963 ) ) ;
#20285=PLANE ( 'NONE',  #17088 ) ;
#20286=AXIS2_PLACEMENT_3D ( 'NONE', #10300, #50513, #51286 ) ;
#20287=DIRECTION ( 'NONE',  ( 0.000000000000000000, -1.000000000000000000, 0.000000000000000000 ) ) ;
#20289=CARTESIAN_POINT ( 'NONE',  ( -167.1580984288390823, -189.7472609257535510, -39.24667733211878584 ) ) ;
#20290=VERTEX_POINT ( 'NONE', #34124 ) ;
#20292=DIRECTION ( 'NONE',  ( 0.000000000000000000, 0.000000000000000000, 1.000000000000000000 ) ) ;
#20293=DIRECTION ( 'NONE',  ( 0.000000000000000000, -1.000000000000000000, -0.000000000000000000 ) ) ;
#20294=VERTEX_POINT ( 'NONE', #25465 ) ;
#20295=EDGE_LOOP ( 'NONE', ( #18145, #34670, #24405, #14174 ) ) ;
#20297=CARTESIAN_POINT ( 'NONE',  ( 71.97629403264902237, -183.6283474603465606, -29.43839964798649333 ) ) ;
#20298=CIRCLE ( 'NONE', #4367, 124.9999999999999858 ) ;
#20299=ADVANCED_FACE ( 'NONE', ( #41481 ), #33608, .F. ) ;
#20301=CARTESIAN_POINT ( 'NONE',  ( -48.98765787015805984, -189.7472609257535510, -0.8610436117673551104 ) ) ;
#20302=AXIS2_PLACEMENT_3D ( 'NONE', #4576, #32170, #48992 ) ;
#20304=ORIENTED_EDGE ( 'NONE', *, *, #14110, .F. ) ;
#20305=EDGE_LOOP ( 'NONE', ( #37159, #17230, #5456, #20145 ) ) ;
#20306=CARTESIAN_POINT ( 'NONE',  ( 48.69345348225014902, -175.3837268820161057, -78.62880929222872339 ) ) ;
#20308=CARTESIAN_POINT ( 'NONE',  ( -157.8637630444124795, -193.5000000000000000, -60.49794494914009135 ) ) ;
#20311=DIRECTION ( 'NONE',  ( -0.000000000000000000, -1.000000000000000000, 0.000000000000000000 ) ) ;
#20312=ORIENTED_EDGE ( 'NONE', *, *, #23713, .F. ) ;
#20313=DIRECTION ( 'NONE',  ( -0.000000000000000000, 1.000000000000000000, 0.000000000000000000 ) ) ;
#20315=DIRECTION ( 'NONE',  ( 0.000000000000000000, 0.000000000000000000, -1.000000000000000000 ) ) ;
#20316=CARTESIAN_POINT ( 'NONE',  ( -121.1142239062970418, -193.5000000000000000, 101.7307360698549132 ) ) ;
#20317=AXIS2_PLACEMENT_3D ( 'NONE', #45776, #25801, #41832 ) ;
#20319=VERTEX_POINT ( 'NONE', #29656 ) ;
#20322=VECTOR ( 'NONE', #604, 1000.000000000000114 ) ;
#20323=CARTESIAN_POINT ( 'NONE',  ( -48.47912675150885065, -183.6283474603465606, 6.938893903907228378E-15 ) ) ;
#20324=DIRECTION ( 'NONE',  ( 0.000000000000000000, 0.000000000000000000, 1.000000000000000000 ) ) ;
#20325=ORIENTED_EDGE ( 'NONE', *, *, #15114, .T. ) ;
#20326=EDGE_CURVE ( 'NONE', #2316, #23737, #41655, .T. ) ;
#20328=DIRECTION ( 'NONE',  ( 0.3482016354343928088, 0.000000000000000000, 0.9374196611341231167 ) ) ;
#20329=ORIENTED_EDGE ( 'NONE', *, *, #45493, .F. ) ;
#20330=DIRECTION ( 'NONE',  ( -0.000000000000000000, 1.000000000000000000, -0.000000000000000000 ) ) ;
#20331=ORIENTED_EDGE ( 'NONE', *, *, #9347, .T. ) ;
#20332=DIRECTION ( 'NONE',  ( 0.8896570909947436601, 0.000000000000000000, 0.4566292373937200777 ) ) ;
#20333=ORIENTED_EDGE ( 'NONE', *, *, #48755, .F. ) ;
#20334=DIRECTION ( 'NONE',  ( -0.000000000000000000, 1.000000000000000000, -0.000000000000000000 ) ) ;
#20335=FACE_BOUND ( 'NONE', #45707, .T. ) ;
#20339=VECTOR ( 'NONE', #38814, 1000.000000000000000 ) ;
#20340=DIRECTION ( 'NONE',  ( -0.000000000000000000, 1.000000000000000000, -0.000000000000000000 ) ) ;
#20342=DIRECTION ( 'NONE',  ( 0.000000000000000000, -0.000000000000000000, -1.000000000000000000 ) ) ;
#20343=EDGE_CURVE ( 'NONE', #210, #11500, #16502, .T. ) ;
#20344=CARTESIAN_POINT ( 'NONE',  ( -96.65280530915693191, -183.6283474603465606, -115.3442529744087466 ) ) ;
#20345=CIRCLE ( 'NONE', #5295, 125.0000000000000000 ) ;
#20346=ORIENTED_EDGE ( 'NONE', *, *, #46117, .F. ) ;
#20347=DIRECTION ( 'NONE',  ( 0.000000000000000000, -0.000000000000000000, -1.000000000000000000 ) ) ;
#20348=ORIENTED_EDGE ( 'NONE', *, *, #6026, .F. ) ;
#20349=EDGE_LOOP ( 'NONE', ( #45410, #1650, #28695, #13457 ) ) ;
#20352=PLANE ( 'NONE',  #45475 ) ;
#20353=VERTEX_POINT ( 'NONE', #19386 ) ;
#20354=ORIENTED_EDGE ( 'NONE', *, *, #5598, .F. ) ;
#20356=VECTOR ( 'NONE', #49145, 1000.000000000000000 ) ;
#20357=AXIS2_PLACEMENT_3D ( 'NONE', #49826, #6713, #9611 ) ;
#20358=EDGE_CURVE ( 'NONE', #32858, #39920, #51457, .T. ) ;
#20360=AXIS2_PLACEMENT_3D ( 'NONE', #33791, #26155, #13830 ) ;
#20361=AXIS2_PLACEMENT_3D ( 'NONE', #51522, #47591, #51028 ) ;
#20364=CARTESIAN_POINT ( 'NONE',  ( -48.88225018079680950, -177.1207230881787780, -0.9151456172430169067 ) ) ;
#20365=ORIENTED_EDGE ( 'NONE', *, *, #40345, .F. ) ;
#20366=DIRECTION ( 'NONE',  ( 0.000000000000000000, 0.000000000000000000, 1.000000000000000000 ) ) ;
#20367=DIRECTION ( 'NONE',  ( -0.000000000000000000, 1.000000000000000000, -0.000000000000000000 ) ) ;
#20368=ADVANCED_FACE ( 'NONE', ( #31207 ), #39082, .F. ) ;
#20369=CARTESIAN_POINT ( 'NONE',  ( 59.29945538372744807, -193.5000000000000000, 63.31490529818492519 ) ) ;
#20374=ORIENTED_EDGE ( 'NONE', *, *, #17818, .T. ) ;
#20378=PLANE ( 'NONE',  #30988 ) ;
#20382=ORIENTED_EDGE ( 'NONE', *, *, #48, .F. ) ;
#20388=ORIENTED_EDGE ( 'NONE', *, *, #4258, .T. ) ;
#20389=CARTESIAN_POINT ( 'NONE',  ( 61.06976976088562026, -193.5000000000000000, -60.19999396110170409 ) ) ;
#20390=EDGE_CURVE ( 'NONE', #10059, #32964, #27397, .T. ) ;
#20392=DIRECTION ( 'NONE',  ( -0.2635871660690648488, 0.000000000000000000, -0.9646355819083595184 ) ) ;
#20393=CARTESIAN_POINT ( 'NONE',  ( -78.41101675714243413, -193.5000000000000000, -120.3332351033023286 ) ) ;
#20394=ORIENTED_EDGE ( 'NONE', *, *, #14238, .F. ) ;
#20396=CIRCLE ( 'NONE', #5304, 125.0000000000000000 ) ;
#20397=ORIENTED_EDGE ( 'NONE', *, *, #49697, .F. ) ;
#20401=VECTOR ( 'NONE', #8889, 1000.000000000000000 ) ;
#20402=CARTESIAN_POINT ( 'NONE',  ( 76.47090317495664635, -175.3837268820161057, -3.534122433557446374 ) ) ;
#20403=DIRECTION ( 'NONE',  ( -0.4300652022765304450, 0.000000000000000000, 0.9027978299657387629 ) ) ;
#20404=CARTESIAN_POINT ( 'NONE',  ( -153.7332855749581881, -189.7472609257535510, 67.42819922234390617 ) ) ;
#20406=LINE ( 'NONE', #32501, #48053 ) ;
#20408=ORIENTED_EDGE ( 'NONE', *, *, #10525, .T. ) ;
#20409=DIRECTION ( 'NONE',  ( -0.4566292373937140270, 0.000000000000000000, 0.8896570909947467687 ) ) ;
#20410=LINE ( 'NONE', #36431, #13143 ) ;
#20411=CARTESIAN_POINT ( 'NONE',  ( 72.12732647922463514, -177.1207230881787780, 28.81338593824055749 ) ) ;
#20412=FACE_BOUND ( 'NONE', #45069, .T. ) ;
#20413=ORIENTED_EDGE ( 'NONE', *, *, #2432, .F. ) ;
#20415=VECTOR ( 'NONE', #38634, 1000.000000000000000 ) ;
#20417=EDGE_CURVE ( 'NONE', #50110, #39155, #8090, .T. ) ;
#20418=EDGE_LOOP ( 'NONE', ( #38524, #12295, #9741, #42561 ) ) ;
#20420=CARTESIAN_POINT ( 'NONE',  ( -107.6930423737362190, -193.5000000000000000, 110.0850225811110761 ) ) ;
#20422=VECTOR ( 'NONE', #33445, 1000.000000000000114 ) ;
#20423=CARTESIAN_POINT ( 'NONE',  ( 74.31448861501726810, -177.1207230881787780, -23.38221600314288651 ) ) ;
#20424=FACE_BOUND ( 'NONE', #36166, .T. ) ;
#20425=FACE_OUTER_BOUND ( 'NONE', #10842, .T. ) ;
#20427=EDGE_CURVE ( 'NONE', #8625, #17957, #38832, .T. ) ;
#20428=CARTESIAN_POINT ( 'NONE',  ( 37.29583330861160562, -175.3837268820161057, -89.54698061029594669 ) ) ;
#20429=VECTOR ( 'NONE', #18463, 1000.000000000000000 ) ;
#20430=ORIENTED_EDGE ( 'NONE', *, *, #27606, .F. ) ;
#20431=EDGE_CURVE ( 'NONE', #10147, #47473, #30953, .T. ) ;
#20432=VERTEX_POINT ( 'NONE', #23582 ) ;
#20433=DIRECTION ( 'NONE',  ( -0.000000000000000000, 1.000000000000000000, -0.000000000000000000 ) ) ;
#20434=AXIS2_PLACEMENT_3D ( 'NONE', #23049, #51966, #31962 ) ;
#20435=EDGE_CURVE ( 'NONE', #16247, #14954, #21533, .T. ) ;
#20437=CARTESIAN_POINT ( 'NONE',  ( -149.1282321233095445, -193.5000000000000000, -72.42760398749011586 ) ) ;
#20439=DIRECTION ( 'NONE',  ( 0.000000000000000000, 0.000000000000000000, 1.000000000000000000 ) ) ;
#20441=FACE_OUTER_BOUND ( 'NONE', #23089, .T. ) ;
#20442=FACE_OUTER_BOUND ( 'NONE', #44775, .T. ) ;
#20443=ORIENTED_EDGE ( 'NONE', *, *, #34639, .F. ) ;
#20444=DIRECTION ( 'NONE',  ( 0.000000000000000000, 1.000000000000000000, 0.000000000000000000 ) ) ;
#20445=CARTESIAN_POINT ( 'NONE',  ( -142.3192003680973130, -183.6283474603465606, 82.57748230379306165 ) ) ;
#20448=DIRECTION ( 'NONE',  ( -0.7575112421616284619, 0.000000000000000000, 0.6528221181905119463 ) ) ;
#20449=ORIENTED_EDGE ( 'NONE', *, *, #21815, .T. ) ;
#20451=VECTOR ( 'NONE', #44346, 1000.000000000000114 ) ;
#20452=ORIENTED_EDGE ( 'NONE', *, *, #8460, .F. ) ;
#20454=CARTESIAN_POINT ( 'NONE',  ( -140.0851925571752474, -193.5000000000000000, 83.57229767764225414 ) ) ;
#20455=VERTEX_POINT ( 'NONE', #6544 ) ;
#20456=LINE ( 'NONE', #476, #21616 ) ;
#20457=CARTESIAN_POINT ( 'NONE',  ( -92.16375985330356002, -193.5000000000000000, 117.1181148702521710 ) ) ;
#20458=ORIENTED_EDGE ( 'NONE', *, *, #8818, .T. ) ;
#20459=AXIS2_PLACEMENT_3D ( 'NONE', #2263, #42184, #14878 ) ;
#20461=FACE_OUTER_BOUND ( 'NONE', #20418, .T. ) ;
#20463=CARTESIAN_POINT ( 'NONE',  ( -169.9883746053192795, -175.3837268820161057, -24.72869175143020826 ) ) ;
#20465=CARTESIAN_POINT ( 'NONE',  ( -48.47912675150885065, -189.7472609257535510, 6.938893903907228378E-15 ) ) ;
#20468=DIRECTION ( 'NONE',  ( -0.8757349421956412971, 0.000000000000000000, 0.4827922027307366970 ) ) ;
#20469=AXIS2_PLACEMENT_3D ( 'NONE', #26449, #14134, #11200 ) ;
#20471=FACE_OUTER_BOUND ( 'NONE', #12522, .T. ) ;
#20472=DIRECTION ( 'NONE',  ( 0.000000000000000000, 0.000000000000000000, -1.000000000000000000 ) ) ;
#20474=CARTESIAN_POINT ( 'NONE',  ( 61.06976976088562026, -175.3837268820161057, -60.19999396110170409 ) ) ;
#20475=EDGE_CURVE ( 'NONE', #45648, #36788, #35152, .T. ) ;
#20476=DIRECTION ( 'NONE',  ( 0.000000000000000000, 0.000000000000000000, -1.000000000000000000 ) ) ;
#20477=CARTESIAN_POINT ( 'NONE',  ( -53.47502265695602119, -177.1207230881787780, -124.9001241957025883 ) ) ;
#20478=ADVANCED_FACE ( 'NONE', ( #3356, #50677, #26486, #31464, #30682, #51207, #15196, #43297, #26751, #11492, #43560, #6794, #22817, #20157, #12780, #48283, #32765, #48558, #20676, #12263, #176, #24364, #28297, #44349, #28031, #15719, #24881, #23841, #4388, #3876, #28806, #8340, #36712, #40369, #31979, #44594, #43808, #8844, #24614, #31734, #16224, #4650, #44855, #47772, #40128, #28550, #7809, #48810, #16485, #20412, #4145, #11747, #20949, #36435, #32507, #715, #434, #12533, #8583, #39852, #40628, #48019, #40900, #19902, #4925, #16760, #24117, #51714, #15971, #44073, #8073, #12002, #35935, #27773, #51986, #36180, #32238, #13569, #41682, #49586, #959, #45904, #17009, #29067, #41419, #33796, #49061, #9379, #5707, #33018, #25404, #37482, #13044, #45133, #25150, #45645, #41164, #36968, #49843, #17535, #9122, #29592, #21199, #5184, #37741, #9897 ), #45386, .T. ) ;
#20481=EDGE_LOOP ( 'NONE', ( #49731, #35441, #12968, #17843 ) ) ;
#20483=FACE_OUTER_BOUND ( 'NONE', #25128, .T. ) ;
#20484=EDGE_CURVE ( 'NONE', #13937, #41128, #21724, .T. ) ;
#20486=CARTESIAN_POINT ( 'NONE',  ( -80.17897391495031911, -193.5000000000000000, 120.9136869416132498 ) ) ;
#20487=CARTESIAN_POINT ( 'NONE',  ( -48.47912675150885065, -183.6283474603465606, 6.938893903907228378E-15 ) ) ;
#20488=ORIENTED_EDGE ( 'NONE', *, *, #35247, .F. ) ;
#20489=VECTOR ( 'NONE', #33345, 1000.000000000000000 ) ;
#20492=DIRECTION ( 'NONE',  ( 0.000000000000000000, -0.000000000000000000, 1.000000000000000000 ) ) ;
#20493=ORIENTED_EDGE ( 'NONE', *, *, #46917, .T. ) ;
#20494=AXIS2_PLACEMENT_3D ( 'NONE', #5371, #17195, #890 ) ;
#20496=DIRECTION ( 'NONE',  ( 0.9473263538541946138, 0.000000000000000000, -0.3202698538628279690 ) ) ;
#20499=EDGE_LOOP ( 'NONE', ( #28916, #5367, #18001, #46275 ) ) ;
#20503=EDGE_CURVE ( 'NONE', #17442, #46449, #50086, .T. ) ;
#20504=DIRECTION ( 'NONE',  ( 0.08879589532292483933, 0.000000000000000000, 0.9960498426152178952 ) ) ;
#20505=DIRECTION ( 'NONE',  ( 0.6528221181905174975, 0.000000000000000000, 0.7575112421616236880 ) ) ;
#20506=CARTESIAN_POINT ( 'NONE',  ( 69.66827051661184100, -175.3837268820161057, -40.81902153125259503 ) ) ;
#20507=FACE_OUTER_BOUND ( 'NONE', #39218, .T. ) ;
#20508=ORIENTED_EDGE ( 'NONE', *, *, #48145, .T. ) ;
#20509=LINE ( 'NONE', #28645, #48279 ) ;
#20511=LINE ( 'NONE', #24455, #36457 ) ;
#20512=CARTESIAN_POINT ( 'NONE',  ( -92.16375985330357423, -175.3837268820161057, 117.1181148702521710 ) ) ;
#20515=FACE_OUTER_BOUND ( 'NONE', #1122, .T. ) ;
#20518=EDGE_CURVE ( 'NONE', #47358, #37325, #11908, .T. ) ;
#20520=LINE ( 'NONE', #12896, #50873 ) ;
#20521=DIRECTION ( 'NONE',  ( 0.000000000000000000, -0.000000000000000000, -1.000000000000000000 ) ) ;
#20522=( LENGTH_UNIT ( ) NAMED_UNIT ( * ) SI_UNIT ( .MILLI., .METRE. ) );
#20524=LINE ( 'NONE', #20802, #39947 ) ;
#20526=CARTESIAN_POINT ( 'NONE',  ( -49.29161362951453640, -175.3837268820161057, 0.5829794791144718991 ) ) ;
#20528=ORIENTED_EDGE ( 'NONE', *, *, #14910, .F. ) ;
#20529=CARTESIAN_POINT ( 'NONE',  ( -47.50057025920934706, -183.6283474603465606, -0.2059786187410884151 ) ) ;
#20530=CARTESIAN_POINT ( 'NONE',  ( -1.230335819511603423, -183.6283474603465606, 115.7261930397108216 ) ) ;
#20531=CIRCLE ( 'NONE', #19702, 125.0000000000000000 ) ;
#20534=CARTESIAN_POINT ( 'NONE',  ( -172.5669052183642123, -177.1207230881787780, 15.07392567185553567 ) ) ;
#20535=VERTEX_POINT ( 'NONE', #24006 ) ;
#20536=LINE ( 'NONE', #8201, #6362 ) ;
#20537=CARTESIAN_POINT ( 'NONE',  ( 30.05499637021959813, -177.1207230881787780, -97.24912084693207248 ) ) ;
#20538=AXIS2_PLACEMENT_3D ( 'NONE', #22321, #38352, #17377 ) ;
#20541=CARTESIAN_POINT ( 'NONE',  ( -166.9492939735806090, -189.7472609257535510, 39.87254040532606325 ) ) ;
#20543=EDGE_CURVE ( 'NONE', #18993, #41471, #16664, .T. ) ;
#20544=CIRCLE ( 'NONE', #2915, 125.0000000000000000 ) ;
#20545=ADVANCED_FACE ( 'NONE', ( #9028 ), #5087, .T. ) ;
#20546=CARTESIAN_POINT ( 'NONE',  ( 69.14211578623219623, -177.1207230881787780, 42.31126686685117022 ) ) ;
#20547=EDGE_CURVE ( 'NONE', #37656, #36987, #40802, .T. ) ;
#20548=CARTESIAN_POINT ( 'NONE',  ( -48.47912675150885065, -189.7472609257535510, 6.938893903907228378E-15 ) ) ;
#20552=VERTEX_POINT ( 'NONE', #20855 ) ;
#20554=CARTESIAN_POINT ( 'NONE',  ( -140.8230258362169707, -193.5000000000000000, 84.24728067916045404 ) ) ;
#20556=ORIENTED_EDGE ( 'NONE', *, *, #27879, .T. ) ;
#20558=EDGE_CURVE ( 'NONE', #32896, #51992, #43977, .T. ) ;
#20560=CARTESIAN_POINT ( 'NONE',  ( 75.27070168362158142, -193.5000000000000000, 17.63462396184792524 ) ) ;
#20561=CIRCLE ( 'NONE', #22251, 125.0000000000000000 ) ;
#20564=DIRECTION ( 'NONE',  ( -0.000000000000000000, 1.000000000000000000, 0.000000000000000000 ) ) ;
#20566=ORIENTED_EDGE ( 'NONE', *, *, #30592, .T. ) ;
#20567=VERTEX_POINT ( 'NONE', #48192 ) ;
#20568=AXIS2_PLACEMENT_3D ( 'NONE', #41762, #42258, #30192 ) ;
#20571=CARTESIAN_POINT ( 'NONE',  ( 55.03325008324586776, -177.1207230881787780, -70.07273251429357686 ) ) ;
#20573=ORIENTED_EDGE ( 'NONE', *, *, #7628, .T. ) ;
#20575=PLANE ( 'NONE',  #38817 ) ;
#20579=LINE ( 'NONE', #31890, #2032 ) ;
#20580=EDGE_LOOP ( 'NONE', ( #35854, #21381, #19257, #44428 ) ) ;
#20581=DIRECTION ( 'NONE',  ( -0.000000000000000000, 1.000000000000000000, -0.000000000000000000 ) ) ;
#20582=AXIS2_PLACEMENT_3D ( 'NONE', #13160, #32854, #28908 ) ;
#20583=FACE_OUTER_BOUND ( 'NONE', #30403, .T. ) ;
#20586=ORIENTED_EDGE ( 'NONE', *, *, #45124, .F. ) ;
#20587=ORIENTED_EDGE ( 'NONE', *, *, #8664, .F. ) ;
#20588=DIRECTION ( 'NONE',  ( 0.000000000000000000, 0.000000000000000000, 1.000000000000000000 ) ) ;
#20590=ORIENTED_EDGE ( 'NONE', *, *, #19960, .T. ) ;
#20591=DIRECTION ( 'NONE',  ( 0.000000000000000000, -0.000000000000000000, -1.000000000000000000 ) ) ;
#20593=ORIENTED_EDGE ( 'NONE', *, *, #7976, .T. ) ;
#20596=VERTEX_POINT ( 'NONE', #32672 ) ;
#20600=CARTESIAN_POINT ( 'NONE',  ( -77.03256798524175508, -175.3837268820161057, 121.6951149130964893 ) ) ;
#20602=AXIS2_PLACEMENT_3D ( 'NONE', #48199, #8244, #28460 ) ;
#20604=DIRECTION ( 'NONE',  ( 0.000000000000000000, -1.000000000000000000, -0.000000000000000000 ) ) ;
#20608=EDGE_CURVE ( 'NONE', #26111, #21667, #24272, .T. ) ;
#20610=ORIENTED_EDGE ( 'NONE', *, *, #29162, .T. ) ;
#20611=CARTESIAN_POINT ( 'NONE',  ( 67.42090074966655777, -175.3837268820161057, -46.82076062204441058 ) ) ;
#20612=ORIENTED_EDGE ( 'NONE', *, *, #51304, .T. ) ;
#20614=ORIENTED_EDGE ( 'NONE', *, *, #21085, .F. ) ;
#20615=CIRCLE ( 'NONE', #9708, 125.0000000000000000 ) ;
#20616=DIRECTION ( 'NONE',  ( -0.000000000000000000, 1.000000000000000000, -0.000000000000000000 ) ) ;
#20617=CARTESIAN_POINT ( 'NONE',  ( -48.88225018079680950, -193.5000000000000000, -0.9151456172430169067 ) ) ;
#20618=ORIENTED_EDGE ( 'NONE', *, *, #29861, .T. ) ;
#20619=CIRCLE ( 'NONE', #41577, 125.0000000000000000 ) ;
#20620=VERTEX_POINT ( 'NONE', #25061 ) ;
#20621=DIRECTION ( 'NONE',  ( -0.8124868780056742068, 0.000000000000000000, -0.5829794791144820021 ) ) ;
#20623=VECTOR ( 'NONE', #3515, 1000.000000000000227 ) ;
#20624=CARTESIAN_POINT ( 'NONE',  ( -173.4460699164830260, -189.7472609257535510, -2.874563619423202265 ) ) ;
#20625=ORIENTED_EDGE ( 'NONE', *, *, #48396, .F. ) ;
#20627=ADVANCED_FACE ( 'NONE', ( #21101 ), #37123, .F. ) ;
#20630=DIRECTION ( 'NONE',  ( 0.000000000000000000, -1.000000000000000000, 0.000000000000000000 ) ) ;
#20631=DIRECTION ( 'NONE',  ( 0.000000000000000000, -0.000000000000000000, 1.000000000000000000 ) ) ;
#20632=DIRECTION ( 'NONE',  ( 0.000000000000000000, -0.000000000000000000, -1.000000000000000000 ) ) ;
#20634=ORIENTED_EDGE ( 'NONE', *, *, #20141, .F. ) ;
#20636=EDGE_LOOP ( 'NONE', ( #29770, #33103, #36156, #25469 ) ) ;
#20637=DIRECTION ( 'NONE',  ( 0.000000000000000000, 0.000000000000000000, -1.000000000000000000 ) ) ;
#20638=LINE ( 'NONE', #32976, #35210 ) ;
#20639=CIRCLE ( 'NONE', #50028, 125.0000000000000000 ) ;
#20640=DIRECTION ( 'NONE',  ( 0.000000000000000000, -1.000000000000000000, 0.000000000000000000 ) ) ;
#20643=PLANE ( 'NONE',  #5410 ) ;
#20644=ORIENTED_EDGE ( 'NONE', *, *, #19424, .T. ) ;
#20645=VECTOR ( 'NONE', #14275, 1000.000000000000000 ) ;
#20646=EDGE_CURVE ( 'NONE', #32529, #32483, #40539, .T. ) ;
#20647=VERTEX_POINT ( 'NONE', #614 ) ;
#20648=DIRECTION ( 'NONE',  ( 0.8896570909947436601, 0.000000000000000000, 0.4566292373937200777 ) ) ;
#20649=ORIENTED_EDGE ( 'NONE', *, *, #20125, .T. ) ;
#20653=DIRECTION ( 'NONE',  ( -0.000000000000000000, 1.000000000000000000, 0.000000000000000000 ) ) ;
#20657=ORIENTED_EDGE ( 'NONE', *, *, #49497, .T. ) ;
#20658=DIRECTION ( 'NONE',  ( 0.000000000000000000, 0.000000000000000000, 1.000000000000000000 ) ) ;
#20660=ORIENTED_EDGE ( 'NONE', *, *, #8574, .T. ) ;
#20661=ADVANCED_FACE ( 'NONE', ( #33466 ), #13227, .T. ) ;
#20662=AXIS2_PLACEMENT_3D ( 'NONE', #6974, #51148, #14879 ) ;
#20663=VERTEX_POINT ( 'NONE', #30283 ) ;
#20667=CARTESIAN_POINT ( 'NONE',  ( 141.7825277784304205, -213.5000000000000000, -41.45482488023466061 ) ) ;
#20669=LINE ( 'NONE', #171, #28715 ) ;
#20672=EDGE_LOOP ( 'NONE', ( #42544, #28032, #24839, #10548 ) ) ;
#20675=PLANE ( 'NONE',  #48796 ) ;
#20676=FACE_BOUND ( 'NONE', #18525, .T. ) ;
#20677=VERTEX_POINT ( 'NONE', #5611 ) ;
#20678=EDGE_CURVE ( 'NONE', #14148, #10828, #34161, .T. ) ;
#20679=CIRCLE ( 'NONE', #49200, 125.0000000000000000 ) ;
#20681=CARTESIAN_POINT ( 'NONE',  ( -47.53180039765465636, -175.3837268820161057, -0.3202698538628280800 ) ) ;
#20682=ORIENTED_EDGE ( 'NONE', *, *, #40585, .T. ) ;
#20683=AXIS2_PLACEMENT_3D ( 'NONE', #25264, #8975, #33913 ) ;
#20686=DIRECTION ( 'NONE',  ( 0.3202698538628279690, 0.000000000000000000, 0.9473263538541946138 ) ) ;
#20687=ORIENTED_EDGE ( 'NONE', *, *, #34716, .F. ) ;
#20688=DIRECTION ( 'NONE',  ( 0.000000000000000000, 0.000000000000000000, 1.000000000000000000 ) ) ;
#20689=CIRCLE ( 'NONE', #30733, 125.0000000000000000 ) ;
#20690=FACE_BOUND ( 'NONE', #20481, .T. ) ;
#20692=CARTESIAN_POINT ( 'NONE',  ( -49.30901192927175458, -189.7472609257535510, -124.9972451320097093 ) ) ;
#20693=VERTEX_POINT ( 'NONE', #26337 ) ;
#20694=EDGE_CURVE ( 'NONE', #35744, #21107, #48425, .T. ) ;
#20696=AXIS2_PLACEMENT_3D ( 'NONE', #32425, #37404, #28729 ) ;
#20698=DIRECTION ( 'NONE',  ( 0.000000000000000000, 1.000000000000000000, 0.000000000000000000 ) ) ;
#20699=ORIENTED_EDGE ( 'NONE', *, *, #43908, .F. ) ;
#20701=VECTOR ( 'NONE', #25559, 1000.000000000000114 ) ;
#20702=CARTESIAN_POINT ( 'NONE',  ( -84.19171550243319757, -193.5000000000000000, 119.7898618611247628 ) ) ;
#20705=CARTESIAN_POINT ( 'NONE',  ( -47.66663987350317910, -193.5000000000000000, 0.5829794791144832233 ) ) ;
#20707=DIRECTION ( 'NONE',  ( 0.4566292373937077542, 0.000000000000000000, 0.8896570909947499883 ) ) ;
#20708=CARTESIAN_POINT ( 'NONE',  ( -92.78132261338707565, -175.3837268820161057, -116.8859077982276773 ) ) ;
#20709=DIRECTION ( 'NONE',  ( 0.1182731709213592358, 0.000000000000000000, 0.9929810960135178055 ) ) ;
#20710=ORIENTED_EDGE ( 'NONE', *, *, #33779, .F. ) ;
#20713=VERTEX_POINT ( 'NONE', #45548 ) ;
#20715=EDGE_LOOP ( 'NONE', ( #23135, #45406, #5841, #19529 ) ) ;
#20717=PLANE ( 'NONE',  #35735 ) ;
#20720=ORIENTED_EDGE ( 'NONE', *, *, #49954, .T. ) ;
#20721=VECTOR ( 'NONE', #47747, 1000.000000000000000 ) ;
#20722=ADVANCED_FACE ( 'NONE', ( #1391 ), #37386, .F. ) ;
#20723=CARTESIAN_POINT ( 'NONE',  ( -146.2338470511239450, -177.1207230881787780, 76.29032973288700248 ) ) ;
#20724=CARTESIAN_POINT ( 'NONE',  ( -165.5546359831674295, -193.5000000000000000, 43.79868877201493405 ) ) ;
#20725=VERTEX_POINT ( 'NONE', #42105 ) ;
#20728=VERTEX_POINT ( 'NONE', #33185 ) ;
#20729=EDGE_LOOP ( 'NONE', ( #38869, #1982, #13486, #685 ) ) ;
#20730=CARTESIAN_POINT ( 'NONE',  ( -48.47912675150885065, -189.7472609257535510, 6.938893903907228378E-15 ) ) ;
#20731=VECTOR ( 'NONE', #39560, 1000.000000000000000 ) ;
#20733=AXIS2_PLACEMENT_3D ( 'NONE', #20213, #484, #48071 ) ;
#20734=DIRECTION ( 'NONE',  ( 0.000000000000000000, 0.000000000000000000, 1.000000000000000000 ) ) ;
#20736=ORIENTED_EDGE ( 'NONE', *, *, #313, .F. ) ;
#20737=CIRCLE ( 'NONE', #33347, 125.0000000000000000 ) ;
#20738=VECTOR ( 'NONE', #8198, 1000.000000000000114 ) ;
#20739=FACE_OUTER_BOUND ( 'NONE', #12440, .T. ) ;
#20740=DIRECTION ( 'NONE',  ( 0.000000000000000000, -1.000000000000000000, 0.000000000000000000 ) ) ;
#20741=ADVANCED_FACE ( 'NONE', ( #13482 ), #25307, .T. ) ;
#20742=VECTOR ( 'NONE', #37375, 1000.000000000000000 ) ;
#20743=DIRECTION ( 'NONE',  ( 0.000000000000000000, 0.000000000000000000, 1.000000000000000000 ) ) ;
#20747=CARTESIAN_POINT ( 'NONE',  ( -48.47912675150885065, -175.3837268820161057, 6.938893903907228378E-15 ) ) ;
#20749=ORIENTED_EDGE ( 'NONE', *, *, #35944, .F. ) ;
#20750=EDGE_CURVE ( 'NONE', #8060, #36650, #41582, .T. ) ;
#20751=DIRECTION ( 'NONE',  ( -0.2348860457809842095, 0.000000000000000000, 0.9720229140804107493 ) ) ;
#20752=DIRECTION ( 'NONE',  ( 0.7378332790417285736, 0.000000000000000000, -0.6749830015182091136 ) ) ;
#20754=ORIENTED_EDGE ( 'NONE', *, *, #32711, .F. ) ;
#20757=VECTOR ( 'NONE', #8429, 1000.000000000000000 ) ;
#20759=CIRCLE ( 'NONE', #21597, 125.0000000000000000 ) ;
#20764=ORIENTED_EDGE ( 'NONE', *, *, #25967, .F. ) ;
#20767=ORIENTED_EDGE ( 'NONE', *, *, #6019, .T. ) ;
#20768=CARTESIAN_POINT ( 'NONE',  ( -43.48323084606168720, -177.1207230881787780, 123.9001241957026167 ) ) ;
#20769=VERTEX_POINT ( 'NONE', #29248 ) ;
#20771=AXIS2_PLACEMENT_3D ( 'NONE', #16125, #334, #32395 ) ;
#20772=ORIENTED_EDGE ( 'NONE', *, *, #22111, .F. ) ;
#20773=DIRECTION ( 'NONE',  ( -0.1768902751225733261, 0.000000000000000000, 0.9842305779475966077 ) ) ;
#20774=AXIS2_PLACEMENT_3D ( 'NONE', #45951, #34101, #5748 ) ;
#20776=CARTESIAN_POINT ( 'NONE',  ( 14.94072793302542124, -175.3837268820161057, 107.7168604805791716 ) ) ;
#20778=FACE_OUTER_BOUND ( 'NONE', #49087, .T. ) ;
#20780=EDGE_LOOP ( 'NONE', ( #7536, #40978, #19875, #33866 ) ) ;
#20781=PLANE ( 'NONE',  #50798 ) ;
#20783=DIRECTION ( 'NONE',  ( 0.6965510290629882695, 0.000000000000000000, 0.7175072570443395970 ) ) ;
#20784=FACE_OUTER_BOUND ( 'NONE', #10018, .T. ) ;
#20785=ORIENTED_EDGE ( 'NONE', *, *, #31266, .F. ) ;
#20786=EDGE_CURVE ( 'NONE', #19679, #40406, #17699, .T. ) ;
#20788=EDGE_CURVE ( 'NONE', #31046, #22971, #7310, .T. ) ;
#20789=DIRECTION ( 'NONE',  ( 0.000000000000000000, -1.000000000000000000, 0.000000000000000000 ) ) ;
#20790=DIRECTION ( 'NONE',  ( 0.2059786187410889424, 0.000000000000000000, 0.9785564922995060311 ) ) ;
#20791=DIRECTION ( 'NONE',  ( 0.000000000000000000, -0.000000000000000000, -1.000000000000000000 ) ) ;
#20792=VERTEX_POINT ( 'NONE', #45805 ) ;
#20793=ADVANCED_FACE ( 'NONE', ( #38430 ), #21363, .T. ) ;
#20794=DIRECTION ( 'NONE',  ( 0.000000000000000000, -1.000000000000000000, 0.000000000000000000 ) ) ;
#20795=VECTOR ( 'NONE', #39517, 1000.000000000000114 ) ;
#20796=DIRECTION ( 'NONE',  ( 0.000000000000000000, 1.000000000000000000, 0.000000000000000000 ) ) ;
#20798=DIRECTION ( 'NONE',  ( 0.1182731709213660498, 0.000000000000000000, -0.9929810960135169173 ) ) ;
#20799=ORIENTED_EDGE ( 'NONE', *, *, #19894, .F. ) ;
#20800=EDGE_CURVE ( 'NONE', #33685, #1866, #41858, .T. ) ;
#20801=CARTESIAN_POINT ( 'NONE',  ( -86.93810158023210022, -183.6283474603465606, 117.8859915627477335 ) ) ;
#20802=CARTESIAN_POINT ( 'NONE',  ( 32.99469856375239374, -189.7472609257535510, 94.79987230212019256 ) ) ;
#20805=CYLINDRICAL_SURFACE ( 'NONE', #43342, 125.0000000000000000 ) ;
#20806=VERTEX_POINT ( 'NONE', #30799 ) ;
#20807=EDGE_CURVE ( 'NONE', #39429, #44939, #34999, .T. ) ;
#20808=CARTESIAN_POINT ( 'NONE',  ( 75.60865171534661044, -183.6283474603465606, -15.07392567185467236 ) ) ;
#20810=CARTESIAN_POINT ( 'NONE',  ( -110.8210171970983566, -175.3837268820161057, 107.1890582354659074 ) ) ;
#20811=ORIENTED_EDGE ( 'NONE', *, *, #26882, .T. ) ;
#20813=ADVANCED_FACE ( 'NONE', ( #7420 ), #3449, .T. ) ;
#20815=CARTESIAN_POINT ( 'NONE',  ( 75.02564229359539638, -193.5000000000000000, -19.27620354518634826 ) ) ;
#20816=EDGE_CURVE ( 'NONE', #20956, #13540, #14865, .T. ) ;
#20817=PLANE ( 'NONE',  #51248 ) ;
#20818=DIRECTION ( 'NONE',  ( 0.000000000000000000, -0.000000000000000000, -1.000000000000000000 ) ) ;
#20819=CARTESIAN_POINT ( 'NONE',  ( -48.65601702663143868, -183.6283474603465606, 0.9842305779476024918 ) ) ;
#20820=LINE ( 'NONE', #21070, #48096 ) ;
#20821=AXIS2_PLACEMENT_3D ( 'NONE', #40729, #24989, #17631 ) ;
#20823=LINE ( 'NONE', #36848, #45508 ) ;
#20824=FACE_OUTER_BOUND ( 'NONE', #5629, .T. ) ;
#20825=ORIENTED_EDGE ( 'NONE', *, *, #29783, .F. ) ;
#20827=DIRECTION ( 'NONE',  ( 0.000000000000000000, 0.000000000000000000, -1.000000000000000000 ) ) ;
#20829=LINE ( 'NONE', #41301, #17105 ) ;
#20830=ORIENTED_EDGE ( 'NONE', *, *, #45143, .T. ) ;
#20831=VECTOR ( 'NONE', #16327, 1000.000000000000000 ) ;
#20832=VECTOR ( 'NONE', #3339, 1000.000000000000227 ) ;
#20834=AXIS2_PLACEMENT_3D ( 'NONE', #14255, #35238, #11062 ) ;
#20835=ORIENTED_EDGE ( 'NONE', *, *, #39177, .F. ) ;
#20836=DIRECTION ( 'NONE',  ( 0.000000000000000000, 1.000000000000000000, 0.000000000000000000 ) ) ;
#20837=AXIS2_PLACEMENT_3D ( 'NONE', #48368, #3965, #19989 ) ;
#20838=DIRECTION ( 'NONE',  ( -0.9266896074318291543, 0.000000000000000000, -0.3758275821142488260 ) ) ;
#20839=CARTESIAN_POINT ( 'NONE',  ( -33.64434644548591535, -175.3837268820161057, -123.1094209424468033 ) ) ;
#20841=ORIENTED_EDGE ( 'NONE', *, *, #47800, .T. ) ;
#20842=EDGE_CURVE ( 'NONE', #42630, #13937, #44214, .T. ) ;
#20845=FACE_OUTER_BOUND ( 'NONE', #14108, .T. ) ;
#20847=DIRECTION ( 'NONE',  ( -0.000000000000000000, 1.000000000000000000, 0.000000000000000000 ) ) ;
#20849=DIRECTION ( 'NONE',  ( -0.7378332790417189146, 0.000000000000000000, -0.6749830015182196608 ) ) ;
#20850=VERTEX_POINT ( 'NONE', #42631 ) ;
#20851=ADVANCED_FACE ( 'NONE', ( #51550 ), #10567, .F. ) ;
#20855=CARTESIAN_POINT ( 'NONE',  ( 66.49421114223471818, -175.3837268820161057, -46.44493303993017719 ) ) ;
#20856=DIRECTION ( 'NONE',  ( -0.000000000000000000, 1.000000000000000000, -0.000000000000000000 ) ) ;
#20860=ORIENTED_EDGE ( 'NONE', *, *, #41249, .F. ) ;
#20861=ORIENTED_EDGE ( 'NONE', *, *, #12487, .T. ) ;
#20862=DIRECTION ( 'NONE',  ( -0.000000000000000000, 1.000000000000000000, 0.000000000000000000 ) ) ;
#20864=ORIENTED_EDGE ( 'NONE', *, *, #29619, .F. ) ;
#20865=EDGE_CURVE ( 'NONE', #28928, #10952, #29958, .T. ) ;
#20866=EDGE_CURVE ( 'NONE', #664, #35703, #31049, .T. ) ;
#20872=CARTESIAN_POINT ( 'NONE',  ( -149.9407190013151592, -189.7472609257535510, -73.01058346660460074 ) ) ;
#20873=EDGE_CURVE ( 'NONE', #24589, #51222, #35250, .T. ) ;
#20874=ORIENTED_EDGE ( 'NONE', *, *, #22775, .T. ) ;
#20875=CARTESIAN_POINT ( 'NONE',  ( -84.85683048652070681, -175.3837268820161057, 118.5439281552633446 ) ) ;
#20876=VERTEX_POINT ( 'NONE', #23441 ) ;
#20877=FACE_BOUND ( 'NONE', #6953, .T. ) ;
#20879=VECTOR ( 'NONE', #6197, 1000.000000000000000 ) ;
#20880=EDGE_CURVE ( 'NONE', #15236, #4741, #13201, .T. ) ;
#20881=CIRCLE ( 'NONE', #16687, 125.0000000000000000 ) ;
#20882=CARTESIAN_POINT ( 'NONE',  ( -47.74129347246712740, -177.1207230881787780, -0.6749830015182022303 ) ) ;
#20883=ORIENTED_EDGE ( 'NONE', *, *, #25001, .T. ) ;
#20884=AXIS2_PLACEMENT_3D ( 'NONE', #2855, #26004, #18888 ) ;
#20886=CARTESIAN_POINT ( 'NONE',  ( -48.65601702663143868, -177.1207230881787780, 0.9842305779476024918 ) ) ;
#20889=DIRECTION ( 'NONE',  ( 0.2920567706369764371, 0.000000000000000000, -0.9564009842765223146 ) ) ;
#20896=CARTESIAN_POINT ( 'NONE',  ( -40.24578378811990831, -175.3837268820161057, 124.7285535218268251 ) ) ;
#20897=LINE ( 'NONE', #44537, #51328 ) ;
#20898=VERTEX_POINT ( 'NONE', #39956 ) ;
#20899=ORIENTED_EDGE ( 'NONE', *, *, #34716, .T. ) ;
#20900=CARTESIAN_POINT ( 'NONE',  ( -169.2746641285359317, -175.3837268820161057, -32.14713283941908628 ) ) ;
#20901=VECTOR ( 'NONE', #46208, 1000.000000000000000 ) ;
#20903=LINE ( 'NONE', #17212, #14272 ) ;
#20904=EDGE_LOOP ( 'NONE', ( #44251, #46713, #29700, #50699 ) ) ;
#20905=CARTESIAN_POINT ( 'NONE',  ( 5.542374969221976144, -177.1207230881787780, 112.7238987608088365 ) ) ;
#20906=VERTEX_POINT ( 'NONE', #23939 ) ;
#20908=LINE ( 'NONE', #35887, #51835 ) ;
#20909=CARTESIAN_POINT ( 'NONE',  ( 8.448131207122532516, -175.3837268820161057, 111.2847127925100352 ) ) ;
#20912=ORIENTED_EDGE ( 'NONE', *, *, #38113, .F. ) ;
#20913=VERTEX_POINT ( 'NONE', #31835 ) ;
#20914=DIRECTION ( 'NONE',  ( -0.000000000000000000, 1.000000000000000000, 0.000000000000000000 ) ) ;
#20915=DIRECTION ( 'NONE',  ( 0.2920567706369694982, 0.000000000000000000, 0.9564009842765243130 ) ) ;
#20916=AXIS2_PLACEMENT_3D ( 'NONE', #46487, #41771, #18110 ) ;
#20920=ORIENTED_EDGE ( 'NONE', *, *, #8992, .F. ) ;
#20921=AXIS2_PLACEMENT_3D ( 'NONE', #11719, #11449, #51680 ) ;
#20922=EDGE_CURVE ( 'NONE', #22789, #7887, #20737, .T. ) ;
#20923=ADVANCED_FACE ( 'NONE', ( #8693 ), #36540, .T. ) ;
#20928=ORIENTED_EDGE ( 'NONE', *, *, #6478, .F. ) ;
#20929=DIRECTION ( 'NONE',  ( 0.000000000000000000, -1.000000000000000000, 0.000000000000000000 ) ) ;
#20931=PLANE ( 'NONE',  #36380 ) ;
#20932=DIRECTION ( 'NONE',  ( -0.000000000000000000, 1.000000000000000000, -0.000000000000000000 ) ) ;
#20933=ORIENTED_EDGE ( 'NONE', *, *, #30054, .T. ) ;
#20934=DIRECTION ( 'NONE',  ( 0.000000000000000000, 1.000000000000000000, 0.000000000000000000 ) ) ;
#20935=ORIENTED_EDGE ( 'NONE', *, *, #31586, .F. ) ;
#20936=AXIS2_PLACEMENT_3D ( 'NONE', #13692, #39770, #41275 ) ;
#20937=ORIENTED_EDGE ( 'NONE', *, *, #23345, .F. ) ;
#20939=EDGE_CURVE ( 'NONE', #20353, #13271, #51807, .T. ) ;
#20942=DIRECTION ( 'NONE',  ( 0.000000000000000000, -1.000000000000000000, -0.000000000000000000 ) ) ;
#20943=PLANE ( 'NONE',  #44722 ) ;
#20944=ORIENTED_EDGE ( 'NONE', *, *, #30841, .T. ) ;
#20945=LINE ( 'NONE', #13040, #12072 ) ;
#20949=FACE_BOUND ( 'NONE', #9955, .T. ) ;
#20950=EDGE_LOOP ( 'NONE', ( #7611, #35482, #50743, #15452 ) ) ;
#20951=VECTOR ( 'NONE', #30627, 1000.000000000000000 ) ;
#20952=CARTESIAN_POINT ( 'NONE',  ( -63.09433862318517328, -175.3837268820161057, -124.1426420773539405 ) ) ;
#20956=VERTEX_POINT ( 'NONE', #12096 ) ;
#20957=PLANE ( 'NONE',  #45604 ) ;
#20960=DIRECTION ( 'NONE',  ( 0.000000000000000000, 1.000000000000000000, -0.000000000000000000 ) ) ;
#20963=ORIENTED_EDGE ( 'NONE', *, *, #34609, .F. ) ;
#20966=ORIENTED_EDGE ( 'NONE', *, *, #38706, .T. ) ;
#20967=CIRCLE ( 'NONE', #17644, 125.0000000000000000 ) ;
#20970=CARTESIAN_POINT ( 'NONE',  ( -172.3334410065085649, -193.5000000000000000, -6.025661128238022357 ) ) ;
#20971=VERTEX_POINT ( 'NONE', #16072 ) ;
#20972=DIRECTION ( 'NONE',  ( -0.7378332790417189146, 0.000000000000000000, -0.6749830015182196608 ) ) ;
#20973=CARTESIAN_POINT ( 'NONE',  ( 30.50828161901820224, -177.1207230881787780, 96.88131563365348597 ) ) ;
#20974=CARTESIAN_POINT ( 'NONE',  ( -106.2948367055610106, -189.7472609257535510, -110.8257356506552185 ) ) ;
#20975=ADVANCED_FACE ( 'NONE', ( #4500 ), #540, .T. ) ;
#20976=DIRECTION ( 'NONE',  ( 0.7765238627180437447, 0.000000000000000000, -0.6300878435817094392 ) ) ;
#20977=CARTESIAN_POINT ( 'NONE',  ( 55.35935253854128035, -183.6283474603465606, 69.58857822035041352 ) ) ;
#20979=DIRECTION ( 'NONE',  ( 0.000000000000000000, 0.000000000000000000, -1.000000000000000000 ) ) ;
#20980=LINE ( 'NONE', #15755, #49926 ) ;
#20981=ORIENTED_EDGE ( 'NONE', *, *, #38282, .F. ) ;
#20982=VERTEX_POINT ( 'NONE', #43910 ) ;
#20984=PLANE ( 'NONE',  #29847 ) ;
#20987=VERTEX_POINT ( 'NONE', #5483 ) ;
#20988=DIRECTION ( 'NONE',  ( 0.000000000000000000, -1.000000000000000000, 0.000000000000000000 ) ) ;
#20989=DIRECTION ( 'NONE',  ( -0.4031234292879792847, 0.000000000000000000, 0.9151456172430153524 ) ) ;
#20990=VERTEX_POINT ( 'NONE', #51821 ) ;
#20991=CARTESIAN_POINT ( 'NONE',  ( 59.80284513346456521, -177.1207230881787780, 62.45009659481583952 ) ) ;
#20992=EDGE_LOOP ( 'NONE', ( #21074, #20799, #47687, #30195 ) ) ;
#20993=EDGE_LOOP ( 'NONE', ( #36037, #8962, #25889, #4189 ) ) ;
#20995=DIRECTION ( 'NONE',  ( 0.4300652022765115712, 0.000000000000000000, 0.9027978299657477557 ) ) ;
#20996=EDGE_CURVE ( 'NONE', #34425, #38590, #27873, .T. ) ;
#20998=EDGE_LOOP ( 'NONE', ( #7127, #40677, #38449, #37004 ) ) ;
#20999=FACE_OUTER_BOUND ( 'NONE', #48407, .T. ) ;
#21001=DIRECTION ( 'NONE',  ( 0.000000000000000000, -1.000000000000000000, 0.000000000000000000 ) ) ;
#21005=VECTOR ( 'NONE', #11659, 1000.000000000000000 ) ;
#21006=CIRCLE ( 'NONE', #26953, 125.0000000000000000 ) ;
#21008=ORIENTED_EDGE ( 'NONE', *, *, #48263, .T. ) ;
#21010=DIRECTION ( 'NONE',  ( 0.000000000000000000, -1.000000000000000000, 0.000000000000000000 ) ) ;
#21011=FACE_OUTER_BOUND ( 'NONE', #4276, .T. ) ;
#21012=EDGE_LOOP ( 'NONE', ( #35322, #8379, #4965, #10066 ) ) ;
#21016=AXIS2_PLACEMENT_3D ( 'NONE', #22053, #49918, #29413 ) ;
#21017=FACE_OUTER_BOUND ( 'NONE', #17283, .T. ) ;
#21026=EDGE_CURVE ( 'NONE', #18514, #17157, #29130, .T. ) ;
#21027=ORIENTED_EDGE ( 'NONE', *, *, #13185, .F. ) ;
#21029=ORIENTED_EDGE ( 'NONE', *, *, #27908, .T. ) ;
#21032=EDGE_CURVE ( 'NONE', #18605, #2316, #16319, .T. ) ;
#21034=AXIS2_PLACEMENT_3D ( 'NONE', #2963, #13766, #31860 ) ;
#21041=CARTESIAN_POINT ( 'NONE',  ( -166.2107720749849022, -189.7472609257535510, -38.92640747825594616 ) ) ;
#21042=ORIENTED_EDGE ( 'NONE', *, *, #30492, .F. ) ;
#21043=DIRECTION ( 'NONE',  ( 0.000000000000000000, -1.000000000000000000, -0.000000000000000000 ) ) ;
#21044=CARTESIAN_POINT ( 'NONE',  ( -48.36085358058748085, -175.3837268820161057, -0.9929810960135100339 ) ) ;
#21045=ORIENTED_EDGE ( 'NONE', *, *, #16040, .F. ) ;
#21047=CARTESIAN_POINT ( 'NONE',  ( -108.0638572795232335, -183.6283474603465606, 108.7464374498172504 ) ) ;
#21049=ORIENTED_EDGE ( 'NONE', *, *, #2224, .F. ) ;
#21052=CARTESIAN_POINT ( 'NONE',  ( -164.6246685127424882, -175.3837268820161057, -46.20836643930983456 ) ) ;
#21053=VECTOR ( 'NONE', #23540, 1000.000000000000114 ) ;
#21055=ADVANCED_FACE ( 'NONE', ( #20258 ), #32334, .T. ) ;
#21056=PLANE ( 'NONE',  #45144 ) ;
#21058=CARTESIAN_POINT ( 'NONE',  ( -48.47912675150885065, -175.3837268820161057, 6.938893903907228378E-15 ) ) ;
#21060=VERTEX_POINT ( 'NONE', #44445 ) ;
#21062=LINE ( 'NONE', #32360, #18232 ) ;
#21065=FACE_OUTER_BOUND ( 'NONE', #12076, .T. ) ;
#21066=AXIS2_PLACEMENT_3D ( 'NONE', #31015, #46808, #23401 ) ;
#21067=FACE_OUTER_BOUND ( 'NONE', #15548, .T. ) ;
#21070=CARTESIAN_POINT ( 'NONE',  ( 2.669657140899374337, -193.5000000000000000, 114.0561348912355868 ) ) ;
#21071=CARTESIAN_POINT ( 'NONE',  ( -63.43218022845228887, -193.5000000000000000, 124.1024020384604540 ) ) ;
#21072=CARTESIAN_POINT ( 'NONE',  ( -47.50057025920934706, -193.5000000000000000, -0.2059786187410884151 ) ) ;
#21074=ORIENTED_EDGE ( 'NONE', *, *, #2219, .F. ) ;
#21077=EDGE_CURVE ( 'NONE', #49045, #3432, #9935, .T. ) ;
#21078=DIRECTION ( 'NONE',  ( 0.000000000000000000, 0.000000000000000000, -1.000000000000000000 ) ) ;
#21081=ORIENTED_EDGE ( 'NONE', *, *, #29301, .F. ) ;
#21082=VECTOR ( 'NONE', #42615, 999.9999999999998863 ) ;
#21083=VERTEX_POINT ( 'NONE', #42231 ) ;
#21084=DIRECTION ( 'NONE',  ( 0.000000000000000000, -1.000000000000000000, 0.000000000000000000 ) ) ;
#21085=EDGE_CURVE ( 'NONE', #32877, #6126, #25954, .T. ) ;
#21086=PLANE ( 'NONE',  #48823 ) ;
#21087=DIRECTION ( 'NONE',  ( 0.8757349421956379665, 0.000000000000000000, -0.4827922027307427477 ) ) ;
#21088=ORIENTED_EDGE ( 'NONE', *, *, #2287, .F. ) ;
#21089=ORIENTED_EDGE ( 'NONE', *, *, #33016, .T. ) ;
#21090=EDGE_CURVE ( 'NONE', #5101, #27694, #22266, .T. ) ;
#21091=DIRECTION ( 'NONE',  ( 0.08879589532292483933, 0.000000000000000000, 0.9960498426152178952 ) ) ;
#21092=CARTESIAN_POINT ( 'NONE',  ( -49.46816693883101124, -189.7472609257535510, -0.1476465640024848536 ) ) ;
#21094=EDGE_CURVE ( 'NONE', #38778, #8625, #42766, .T. ) ;
#21097=PLANE ( 'NONE',  #47362 ) ;
#21101=FACE_OUTER_BOUND ( 'NONE', #16345, .T. ) ;
#21102=LINE ( 'NONE', #25062, #22312 ) ;
#21103=AXIS2_PLACEMENT_3D ( 'NONE', #5947, #38750, #30109 ) ;
#21104=CARTESIAN_POINT ( 'NONE',  ( -48.47912675150885065, -175.3837268820161057, 6.938893903907228378E-15 ) ) ;
#21105=AXIS2_PLACEMENT_3D ( 'NONE', #37230, #1219, #22693 ) ;
#21106=EDGE_LOOP ( 'NONE', ( #43987, #16220, #30489, #47609 ) ) ;
#21107=VERTEX_POINT ( 'NONE', #26200 ) ;
#21109=CARTESIAN_POINT ( 'NONE',  ( 46.31065297101394407, -193.5000000000000000, 79.94433946042836681 ) ) ;
#21111=DIRECTION ( 'NONE',  ( 0.000000000000000000, -1.000000000000000000, 0.000000000000000000 ) ) ;
#21112=DIRECTION ( 'NONE',  ( -0.000000000000000000, 1.000000000000000000, -0.000000000000000000 ) ) ;
#21115=VECTOR ( 'NONE', #31147, 1000.000000000000000 ) ;
#21117=VERTEX_POINT ( 'NONE', #14147 ) ;
#21120=VECTOR ( 'NONE', #48582, 1000.000000000000000 ) ;
#21121=FACE_OUTER_BOUND ( 'NONE', #13384, .T. ) ;
#21122=ORIENTED_EDGE ( 'NONE', *, *, #24731, .T. ) ;
#21123=CARTESIAN_POINT ( 'NONE',  ( 73.87536152799695799, -175.3837268820161057, -25.58083653558413673 ) ) ;
#21126=DIRECTION ( 'NONE',  ( 0.000000000000000000, 1.000000000000000000, 0.000000000000000000 ) ) ;
#21127=EDGE_LOOP ( 'NONE', ( #22702, #28232, #50520, #29766 ) ) ;
#21130=ADVANCED_FACE ( 'NONE', ( #33836 ), #38292, .T. ) ;
#21131=ORIENTED_EDGE ( 'NONE', *, *, #36983, .F. ) ;
#21137=ORIENTED_EDGE ( 'NONE', *, *, #45317, .T. ) ;
#21138=EDGE_CURVE ( 'NONE', #31867, #21525, #14901, .T. ) ;
#21139=DIRECTION ( 'NONE',  ( 0.000000000000000000, 0.000000000000000000, 1.000000000000000000 ) ) ;
#21140=ADVANCED_FACE ( 'NONE', ( #42497 ), #2311, .T. ) ;
#21141=AXIS2_PLACEMENT_3D ( 'NONE', #23462, #27124, #35275 ) ;
#21145=DIRECTION ( 'NONE',  ( 0.9785564922995046988, 0.000000000000000000, -0.2059786187410953262 ) ) ;
#21146=EDGE_LOOP ( 'NONE', ( #44772, #33022, #850, #18130 ) ) ;
#21147=DIRECTION ( 'NONE',  ( -0.000000000000000000, 1.000000000000000000, -0.000000000000000000 ) ) ;
#21149=ORIENTED_EDGE ( 'NONE', *, *, #33660, .F. ) ;
#21151=LINE ( 'NONE', #49016, #30027 ) ;
#21154=CARTESIAN_POINT ( 'NONE',  ( 61.06976976088564157, -189.7472609257535510, -60.19999396110169698 ) ) ;
#21155=VERTEX_POINT ( 'NONE', #50655 ) ;
#21157=VERTEX_POINT ( 'NONE', #38801 ) ;
#21159=ORIENTED_EDGE ( 'NONE', *, *, #16, .T. ) ;
#21161=CARTESIAN_POINT ( 'NONE',  ( -171.2727421180348415, -193.5000000000000000, 23.38221600314377113 ) ) ;
#21162=CIRCLE ( 'NONE', #8585, 125.0000000000000000 ) ;
#21163=AXIS2_PLACEMENT_3D ( 'NONE', #31174, #47224, #23310 ) ;
#21164=EDGE_CURVE ( 'NONE', #43502, #39314, #50981, .T. ) ;
#21166=CARTESIAN_POINT ( 'NONE',  ( 73.66680038934278230, -189.7472609257535510, -26.55884942729568365 ) ) ;
#21168=EDGE_CURVE ( 'NONE', #3689, #38204, #23296, .T. ) ;
#21170=EDGE_CURVE ( 'NONE', #25060, #16474, #8053, .T. ) ;
#21171=ORIENTED_EDGE ( 'NONE', *, *, #24411, .T. ) ;
#21174=VERTEX_POINT ( 'NONE', #19620 ) ;
#21177=CIRCLE ( 'NONE', #48036, 125.0000000000000000 ) ;
#21180=CARTESIAN_POINT ( 'NONE',  ( 26.62880456707186383, -175.3837268820161057, 98.66508442481512020 ) ) ;
#21181=EDGE_LOOP ( 'NONE', ( #9363, #416, #1423, #3137 ) ) ;
#21183=ORIENTED_EDGE ( 'NONE', *, *, #46846, .T. ) ;
#21184=ADVANCED_FACE ( 'NONE', ( #31185 ), #11469, .T. ) ;
#21186=EDGE_LOOP ( 'NONE', ( #48858, #44491, #40443, #33396 ) ) ;
#21188=LINE ( 'NONE', #24353, #6033 ) ;
#21189=ORIENTED_EDGE ( 'NONE', *, *, #44246, .T. ) ;
#21190=CARTESIAN_POINT ( 'NONE',  ( -47.60339180931321579, -183.6283474603465606, -0.4827922027307358088 ) ) ;
#21192=CARTESIAN_POINT ( 'NONE',  ( -173.1763543514842070, -193.5000000000000000, 8.694908215728892387 ) ) ;
#21193=ORIENTED_EDGE ( 'NONE', *, *, #12262, .T. ) ;
#21194=CARTESIAN_POINT ( 'NONE',  ( -69.77312546433407192, -193.5000000000000000, 123.1729094355500109 ) ) ;
#21199=FACE_BOUND ( 'NONE', #18421, .T. ) ;
#21200=VERTEX_POINT ( 'NONE', #39333 ) ;
#21204=ORIENTED_EDGE ( 'NONE', *, *, #33669, .T. ) ;
#21205=DIRECTION ( 'NONE',  ( 0.000000000000000000, 1.000000000000000000, -0.000000000000000000 ) ) ;
#21207=ORIENTED_EDGE ( 'NONE', *, *, #32883, .T. ) ;
#21209=DIRECTION ( 'NONE',  ( 0.1182731709213730997, 0.000000000000000000, -0.9929810960135161402 ) ) ;
#21211=ORIENTED_EDGE ( 'NONE', *, *, #14382, .T. ) ;
#21212=ADVANCED_FACE ( 'NONE', ( #26981 ), #19115, .T. ) ;
#21213=ADVANCED_FACE ( 'NONE', ( #20137 ), #31439, .T. ) ;
#21214=CARTESIAN_POINT ( 'NONE',  ( -74.51199343215203896, -177.1207230881787780, -122.2591094863194598 ) ) ;
#21215=CARTESIAN_POINT ( 'NONE',  ( 63.82222181224017277, -193.5000000000000000, 52.57768177182522606 ) ) ;
#21216=CARTESIAN_POINT ( 'NONE',  ( -49.21696003055058810, -189.7472609257535510, 0.6749830015182108900 ) ) ;
#21217=ORIENTED_EDGE ( 'NONE', *, *, #39035, .F. ) ;
#21218=AXIS2_PLACEMENT_3D ( 'NONE', #12523, #28790, #44841 ) ;
#21219=DIRECTION ( 'NONE',  ( 0.000000000000000000, 0.000000000000000000, -1.000000000000000000 ) ) ;
#21220=ORIENTED_EDGE ( 'NONE', *, *, #25192, .F. ) ;
#21221=ORIENTED_EDGE ( 'NONE', *, *, #18248, .F. ) ;
#21222=AXIS2_PLACEMENT_3D ( 'NONE', #32582, #44676, #45216 ) ;
#21223=ORIENTED_EDGE ( 'NONE', *, *, #5424, .T. ) ;
#21224=CARTESIAN_POINT ( 'NONE',  ( -126.2322430781613605, -177.1207230881787780, 97.87467957288053810 ) ) ;
#21227=VERTEX_POINT ( 'NONE', #39573 ) ;
#21228=CARTESIAN_POINT ( 'NONE',  ( -155.9608607592036833, -193.5000000000000000, 63.81752780153064464 ) ) ;
#21230=DIRECTION ( 'NONE',  ( -0.000000000000000000, 1.000000000000000000, -0.000000000000000000 ) ) ;
#21231=VERTEX_POINT ( 'NONE', #51693 ) ;
#21233=AXIS2_PLACEMENT_3D ( 'NONE', #29604, #29083, #45151 ) ;
#21234=ADVANCED_FACE ( 'NONE', ( #35131 ), #31961, .T. ) ;
#21235=CARTESIAN_POINT ( 'NONE',  ( 75.78974234412359579, -193.5000000000000000, 13.49993235881449394 ) ) ;
#21236=DIRECTION ( 'NONE',  ( 0.000000000000000000, 0.000000000000000000, -1.000000000000000000 ) ) ;
#21237=ORIENTED_EDGE ( 'NONE', *, *, #41764, .T. ) ;
#21239=LINE ( 'NONE', #41720, #4600 ) ;
#21240=ORIENTED_EDGE ( 'NONE', *, *, #41356, .F. ) ;
#21242=EDGE_LOOP ( 'NONE', ( #6798, #3332, #40078, #13123 ) ) ;
#21243=FACE_OUTER_BOUND ( 'NONE', #26879, .T. ) ;
#21244=ORIENTED_EDGE ( 'NONE', *, *, #11162, .F. ) ;
#21245=LINE ( 'NONE', #41456, #32297 ) ;
#21246=ORIENTED_EDGE ( 'NONE', *, *, #6987, .T. ) ;
#21249=CARTESIAN_POINT ( 'NONE',  ( -2.700932609314997457, -183.6283474603465606, -116.3157639405751809 ) ) ;
#21251=PLANE ( 'NONE',  #47701 ) ;
#21252=ORIENTED_EDGE ( 'NONE', *, *, #8935, .F. ) ;
#21257=CARTESIAN_POINT ( 'NONE',  ( -172.4792251663439231, -177.1207230881787780, 0.3215015308249278281 ) ) ;
#21259=VECTOR ( 'NONE', #5836, 1000.000000000000114 ) ;
#21260=CARTESIAN_POINT ( 'NONE',  ( -143.3583119192899744, -177.1207230881787780, -81.38144888055202841 ) ) ;
#21267=DIRECTION ( 'NONE',  ( 0.2348860457809842095, 0.000000000000000000, -0.9720229140804107493 ) ) ;
#21268=ORIENTED_EDGE ( 'NONE', *, *, #25165, .T. ) ;
#21270=CARTESIAN_POINT ( 'NONE',  ( 40.30419662299490113, -183.6283474603465606, -87.99159897727903967 ) ) ;
#21271=ORIENTED_EDGE ( 'NONE', *, *, #43053, .T. ) ;
#21273=ORIENTED_EDGE ( 'NONE', *, *, #42247, .F. ) ;
#21274=VECTOR ( 'NONE', #39692, 1000.000000000000000 ) ;
#21275=VERTEX_POINT ( 'NONE', #7284 ) ;
#21277=AXIS2_PLACEMENT_3D ( 'NONE', #22269, #25700, #13878 ) ;
#21279=CARTESIAN_POINT ( 'NONE',  ( -48.47912675150885065, -213.5000000000000000, 6.938893903907228378E-15 ) ) ;
#21280=DIRECTION ( 'NONE',  ( 0.000000000000000000, 0.000000000000000000, 1.000000000000000000 ) ) ;
#21281=VERTEX_POINT ( 'NONE', #27754 ) ;
#21283=AXIS2_PLACEMENT_3D ( 'NONE', #19843, #7510, #28241 ) ;
#21287=DIRECTION ( 'NONE',  ( 0.000000000000000000, 0.000000000000000000, -1.000000000000000000 ) ) ;
#21288=VERTEX_POINT ( 'NONE', #19880 ) ;
#21289=EDGE_CURVE ( 'NONE', #24589, #47106, #6534, .T. ) ;
#21290=DIRECTION ( 'NONE',  ( -0.000000000000000000, -1.000000000000000000, 0.000000000000000000 ) ) ;
#21292=VERTEX_POINT ( 'NONE', #44048 ) ;
#21293=AXIS2_PLACEMENT_3D ( 'NONE', #41751, #41216, #37794 ) ;
#21294=ADVANCED_FACE ( 'NONE', ( #23046 ), #4122, .T. ) ;
#21298=CARTESIAN_POINT ( 'NONE',  ( -48.88225018079683082, -193.5000000000000000, 0.9151456172430223468 ) ) ;
#21299=ORIENTED_EDGE ( 'NONE', *, *, #10157, .F. ) ;
#21301=ORIENTED_EDGE ( 'NONE', *, *, #51189, .T. ) ;
#21302=DIRECTION ( 'NONE',  ( -0.4566292373937200777, 0.000000000000000000, 0.8896570909947436601 ) ) ;
#21304=ORIENTED_EDGE ( 'NONE', *, *, #27114, .T. ) ;
#21307=LINE ( 'NONE', #49687, #15734 ) ;
#21308=FACE_OUTER_BOUND ( 'NONE', #10048, .T. ) ;
#21309=ORIENTED_EDGE ( 'NONE', *, *, #12521, .F. ) ;
#21310=VECTOR ( 'NONE', #39616, 1000.000000000000114 ) ;
#21311=ORIENTED_EDGE ( 'NONE', *, *, #22156, .T. ) ;
#21315=DIRECTION ( 'NONE',  ( 0.000000000000000000, 0.000000000000000000, -1.000000000000000000 ) ) ;
#21316=EDGE_LOOP ( 'NONE', ( #5962, #14273, #34888, #18556 ) ) ;
#21318=CARTESIAN_POINT ( 'NONE',  ( -111.3295483157475445, -189.7472609257535510, 108.0501018472332504 ) ) ;
#21320=CARTESIAN_POINT ( 'NONE',  ( 60.58466639580034752, -189.7472609257535510, -61.07445476073404222 ) ) ;
#21322=LINE ( 'NONE', #41536, #4485 ) ;
#21323=DIRECTION ( 'NONE',  ( 0.000000000000000000, 0.000000000000000000, 1.000000000000000000 ) ) ;
#21324=EDGE_CURVE ( 'NONE', #30315, #27694, #50168, .T. ) ;
#21326=ORIENTED_EDGE ( 'NONE', *, *, #14448, .T. ) ;
#21327=LINE ( 'NONE', #49468, #4667 ) ;
#21329=VECTOR ( 'NONE', #12774, 1000.000000000000000 ) ;
#21331=DIRECTION ( 'NONE',  ( 0.000000000000000000, -0.000000000000000000, 1.000000000000000000 ) ) ;
#21333=EDGE_CURVE ( 'NONE', #33835, #43754, #40607, .T. ) ;
#21336=EDGE_CURVE ( 'NONE', #43700, #10047, #36949, .T. ) ;
#21337=DIRECTION ( 'NONE',  ( -0.1182731709213660498, 0.000000000000000000, 0.9929810960135169173 ) ) ;
#21338=FACE_OUTER_BOUND ( 'NONE', #29090, .T. ) ;
#21339=DIRECTION ( 'NONE',  ( -0.000000000000000000, 1.000000000000000000, -0.000000000000000000 ) ) ;
#21340=ORIENTED_EDGE ( 'NONE', *, *, #47378, .F. ) ;
#21343=AXIS2_PLACEMENT_3D ( 'NONE', #42426, #38730, #29819 ) ;
#21344=CARTESIAN_POINT ( 'NONE',  ( -49.38192458147459973, -175.3837268820161057, 0.4300652022765185656 ) ) ;
#21345=DIRECTION ( 'NONE',  ( -0.000000000000000000, 1.000000000000000000, -0.000000000000000000 ) ) ;
#21346=EDGE_LOOP ( 'NONE', ( #17684, #23374, #18095, #5039 ) ) ;
#21348=ORIENTED_EDGE ( 'NONE', *, *, #15728, .T. ) ;
#21349=EDGE_CURVE ( 'NONE', #23109, #18846, #48259, .T. ) ;
#21350=CARTESIAN_POINT ( 'NONE',  ( -109.0835867659424281, -183.6283474603465606, -109.3256576763155010 ) ) ;
#21351=PLANE ( 'NONE',  #22779 ) ;
#21352=DIRECTION ( 'NONE',  ( 0.000000000000000000, 0.000000000000000000, 1.000000000000000000 ) ) ;
#21353=ORIENTED_EDGE ( 'NONE', *, *, #1884, .T. ) ;
#21355=DIRECTION ( 'NONE',  ( 0.000000000000000000, 1.000000000000000000, 0.000000000000000000 ) ) ;
#21357=CARTESIAN_POINT ( 'NONE',  ( 76.46082103836693022, -175.3837268820161057, 3.874202661595785191 ) ) ;
#21358=VECTOR ( 'NONE', #38090, 1000.000000000000000 ) ;
#21359=ORIENTED_EDGE ( 'NONE', *, *, #18207, .T. ) ;
#21363=PLANE ( 'NONE',  #2284 ) ;
#21364=FACE_OUTER_BOUND ( 'NONE', #11137, .T. ) ;
#21366=AXIS2_PLACEMENT_3D ( 'NONE', #43224, #15133, #6725 ) ;
#21367=ORIENTED_EDGE ( 'NONE', *, *, #4849, .T. ) ;
#21368=ORIENTED_EDGE ( 'NONE', *, *, #3848, .T. ) ;
#21369=CARTESIAN_POINT ( 'NONE',  ( -47.57632892154310866, -175.3837268820161057, -0.4300652022765113491 ) ) ;
#21370=DIRECTION ( 'NONE',  ( -0.9266896074318291543, 0.000000000000000000, -0.3758275821142488260 ) ) ;
#21371=ORIENTED_EDGE ( 'NONE', *, *, #50286, .T. ) ;
#21375=ORIENTED_EDGE ( 'NONE', *, *, #39775, .T. ) ;
#21380=CARTESIAN_POINT ( 'NONE',  ( 2.669657140899374337, -193.5000000000000000, 114.0561348912355868 ) ) ;
#21381=ORIENTED_EDGE ( 'NONE', *, *, #26000, .F. ) ;
#21382=CARTESIAN_POINT ( 'NONE',  ( -172.3973245609188041, -193.5000000000000000, 4.503971736581664054 ) ) ;
#21383=DIRECTION ( 'NONE',  ( 0.2348860457809842095, 0.000000000000000000, -0.9720229140804107493 ) ) ;
#21384=ORIENTED_EDGE ( 'NONE', *, *, #35627, .T. ) ;
#21385=DIRECTION ( 'NONE',  ( -0.4827922027307551267, 0.000000000000000000, 0.8757349421956311941 ) ) ;
#21386=FACE_OUTER_BOUND ( 'NONE', #15415, .T. ) ;
#21387=DIRECTION ( 'NONE',  ( 0.2920567706369764371, 0.000000000000000000, -0.9564009842765223146 ) ) ;
#21389=DIRECTION ( 'NONE',  ( 0.000000000000000000, -0.000000000000000000, 1.000000000000000000 ) ) ;
#21390=ADVANCED_FACE ( 'NONE', ( #24339 ), #29315, .T. ) ;
#21391=ORIENTED_EDGE ( 'NONE', *, *, #42019, .T. ) ;
#21392=CARTESIAN_POINT ( 'NONE',  ( 29.90148147319959193, -183.6283474603465606, 96.08646119224013660 ) ) ;
#21393=VERTEX_POINT ( 'NONE', #13295 ) ;
#21394=ORIENTED_EDGE ( 'NONE', *, *, #13453, .T. ) ;
#21395=EDGE_CURVE ( 'NONE', #6231, #1159, #1187, .T. ) ;
#21396=VECTOR ( 'NONE', #22558, 1000.000000000000341 ) ;
#21398=DIRECTION ( 'NONE',  ( 0.3482016354343995812, 0.000000000000000000, -0.9374196611341205632 ) ) ;
#21399=ORIENTED_EDGE ( 'NONE', *, *, #22045, .F. ) ;
#21401=AXIS2_PLACEMENT_3D ( 'NONE', #40117, #31200, #35657 ) ;
#21402=VERTEX_POINT ( 'NONE', #28526 ) ;
#21404=DIRECTION ( 'NONE',  ( 0.000000000000000000, 0.000000000000000000, 1.000000000000000000 ) ) ;
#21405=ORIENTED_EDGE ( 'NONE', *, *, #42569, .T. ) ;
#21406=DIRECTION ( 'NONE',  ( -0.02963332782257007553, 0.000000000000000000, 0.9995608365087941261 ) ) ;
#21410=DIRECTION ( 'NONE',  ( 0.000000000000000000, 0.000000000000000000, 1.000000000000000000 ) ) ;
#21411=AXIS2_PLACEMENT_3D ( 'NONE', #25601, #30319, #30072 ) ;
#21413=CIRCLE ( 'NONE', #44945, 125.0000000000000000 ) ;
#21415=EDGE_LOOP ( 'NONE', ( #42370, #22868, #14802, #17739 ) ) ;
#21416=VERTEX_POINT ( 'NONE', #44569 ) ;
#21417=ORIENTED_EDGE ( 'NONE', *, *, #19038, .T. ) ;
#21419=PLANE ( 'NONE',  #24937 ) ;
#21420=CARTESIAN_POINT ( 'NONE',  ( 2.066935079424583765, -193.5000000000000000, -114.3245189510257802 ) ) ;
#21421=DIRECTION ( 'NONE',  ( -0.000000000000000000, -1.000000000000000000, 0.000000000000000000 ) ) ;
#21422=PLANE ( 'NONE',  #33110 ) ;
#21424=ORIENTED_EDGE ( 'NONE', *, *, #39292, .T. ) ;
#21425=CARTESIAN_POINT ( 'NONE',  ( -149.5539421794694306, -175.3837268820161057, 73.54509967498654532 ) ) ;
#21426=ORIENTED_EDGE ( 'NONE', *, *, #48800, .T. ) ;
#21427=EDGE_LOOP ( 'NONE', ( #30208, #9803, #6205, #3643 ) ) ;
#21429=DIRECTION ( 'NONE',  ( -0.000000000000000000, 1.000000000000000000, -0.000000000000000000 ) ) ;
#21433=ADVANCED_FACE ( 'NONE', ( #12242 ), #48784, .T. ) ;
#21435=ADVANCED_FACE ( 'NONE', ( #4902 ), #940, .T. ) ;
#21436=ADVANCED_FACE ( 'NONE', ( #32989 ), #49039, .T. ) ;
#21437=CARTESIAN_POINT ( 'NONE',  ( -41.90263914168910730, -189.7472609257535510, -124.8268793598473536 ) ) ;
#21439=DIRECTION ( 'NONE',  ( 0.000000000000000000, 0.000000000000000000, 1.000000000000000000 ) ) ;
#21441=VECTOR ( 'NONE', #6984, 1000.000000000000000 ) ;
#21447=VECTOR ( 'NONE', #41451, 1000.000000000000000 ) ;
#21449=ORIENTED_EDGE ( 'NONE', *, *, #11248, .F. ) ;
#21450=EDGE_CURVE ( 'NONE', #14876, #43567, #38503, .T. ) ;
#21451=VECTOR ( 'NONE', #34145, 1000.000000000000000 ) ;
#21452=CARTESIAN_POINT ( 'NONE',  ( -142.3192003680973130, -177.1207230881787780, 82.57748230379306165 ) ) ;
#21453=CARTESIAN_POINT ( 'NONE',  ( -21.46839590530488451, -183.6283474603465606, 122.0467960216650738 ) ) ;
#21454=FACE_OUTER_BOUND ( 'NONE', #15618, .T. ) ;
#21455=ADVANCED_FACE ( 'NONE', ( #33776 ), #9871, .T. ) ;
#21460=VECTOR ( 'NONE', #12166, 1000.000000000000000 ) ;
#21468=LINE ( 'NONE', #29599, #10359 ) ;
#21469=EDGE_LOOP ( 'NONE', ( #5905, #22377, #2753, #5870 ) ) ;
#21473=DIRECTION ( 'NONE',  ( 0.000000000000000000, -1.000000000000000000, 0.000000000000000000 ) ) ;
#21475=CIRCLE ( 'NONE', #46688, 125.0000000000000000 ) ;
#21476=CARTESIAN_POINT ( 'NONE',  ( -48.47912675150885065, -183.6283474603465606, 6.938893903907228378E-15 ) ) ;
#21478=EDGE_LOOP ( 'NONE', ( #18904, #19387, #34294, #7744 ) ) ;
#21480=VERTEX_POINT ( 'NONE', #10127 ) ;
#21482=CARTESIAN_POINT ( 'NONE',  ( 34.93559171950835918, -193.5000000000000000, -93.09664195018497423 ) ) ;
#21484=AXIS2_PLACEMENT_3D ( 'NONE', #15553, #35253, #39694 ) ;
#21485=DIRECTION ( 'NONE',  ( 0.000000000000000000, -1.000000000000000000, 0.000000000000000000 ) ) ;
#21486=AXIS2_PLACEMENT_3D ( 'NONE', #15381, #48487, #43223 ) ;
#21487=CARTESIAN_POINT ( 'NONE',  ( -95.18697522258266019, -193.5000000000000000, 115.9455772817713353 ) ) ;
#21488=CARTESIAN_POINT ( 'NONE',  ( 73.66680038934278230, -193.5000000000000000, -26.55884942729568365 ) ) ;
#21489=CIRCLE ( 'NONE', #48309, 125.0000000000000000 ) ;
#21494=DIRECTION ( 'NONE',  ( 0.9995608365087946812, 0.000000000000000000, -0.02963332782254913048 ) ) ;
#21495=ORIENTED_EDGE ( 'NONE', *, *, #49419, .T. ) ;
#21497=ORIENTED_EDGE ( 'NONE', *, *, #47933, .T. ) ;
#21499=CARTESIAN_POINT ( 'NONE',  ( -15.24927435600542047, -183.6283474603465606, 120.5021863277719092 ) ) ;
#21500=ORIENTED_EDGE ( 'NONE', *, *, #1460, .F. ) ;
#21501=EDGE_CURVE ( 'NONE', #25767, #39566, #38230, .T. ) ;
#21502=PLANE ( 'NONE',  #15434 ) ;
#21503=EDGE_CURVE ( 'NONE', #38453, #13810, #44303, .T. ) ;
#21506=EDGE_LOOP ( 'NONE', ( #44300, #7525, #46685, #24467 ) ) ;
#21507=DIRECTION ( 'NONE',  ( 0.3202698538628416247, 0.000000000000000000, -0.9473263538541900619 ) ) ;
#21508=ORIENTED_EDGE ( 'NONE', *, *, #25349, .F. ) ;
#21509=EDGE_CURVE ( 'NONE', #19400, #50173, #19127, .T. ) ;
#21510=ORIENTED_EDGE ( 'NONE', *, *, #39485, .F. ) ;
#21512=VECTOR ( 'NONE', #29333, 1000.000000000000000 ) ;
#21514=AXIS2_PLACEMENT_3D ( 'NONE', #43031, #30673, #50667 ) ;
#21515=DIRECTION ( 'NONE',  ( 0.000000000000000000, 1.000000000000000000, 0.000000000000000000 ) ) ;
#21517=ORIENTED_EDGE ( 'NONE', *, *, #36402, .T. ) ;
#21518=CIRCLE ( 'NONE', #50895, 125.0000000000000000 ) ;
#21520=CARTESIAN_POINT ( 'NONE',  ( -48.71401279728984690, -183.6283474603465606, 0.9720229140804159673 ) ) ;
#21521=CIRCLE ( 'NONE', #32375, 125.0000000000000000 ) ;
#21522=FACE_OUTER_BOUND ( 'NONE', #49776, .T. ) ;
#21524=ADVANCED_FACE ( 'NONE', ( #6460 ), #21952, .T. ) ;
#21525=VERTEX_POINT ( 'NONE', #42169 ) ;
#21526=CARTESIAN_POINT ( 'NONE',  ( -164.2512865680372727, -189.7472609257535510, -47.13604789772048775 ) ) ;
#21528=CARTESIAN_POINT ( 'NONE',  ( -172.4728835572423975, -183.6283474603465606, 1.322128892812083123 ) ) ;
#21529=ORIENTED_EDGE ( 'NONE', *, *, #12799, .F. ) ;
#21532=AXIS2_PLACEMENT_3D ( 'NONE', #41624, #29011, #1160 ) ;
#21533=CIRCLE ( 'NONE', #36639, 125.0000000000000000 ) ;
#21535=DIRECTION ( 'NONE',  ( -0.000000000000000000, 1.000000000000000000, -0.000000000000000000 ) ) ;
#21536=EDGE_CURVE ( 'NONE', #24293, #41262, #30347, .T. ) ;
#21537=LINE ( 'NONE', #21793, #3595 ) ;
#21540=VECTOR ( 'NONE', #43084, 1000.000000000000114 ) ;
#21541=ORIENTED_EDGE ( 'NONE', *, *, #45914, .T. ) ;
#21543=AXIS2_PLACEMENT_3D ( 'NONE', #21104, #45808, #17701 ) ;
#21545=AXIS2_PLACEMENT_3D ( 'NONE', #21822, #37837, #2363 ) ;
#21547=CARTESIAN_POINT ( 'NONE',  ( -48.47912675150885065, -175.3837268820161057, 6.938893903907228378E-15 ) ) ;
#21548=CARTESIAN_POINT ( 'NONE',  ( -143.2689064740322067, -177.1207230881787780, -79.94433946042767047 ) ) ;
#21549=CARTESIAN_POINT ( 'NONE',  ( -48.47912675150885065, -175.3837268820161057, 6.938893903907228378E-15 ) ) ;
#21550=DIRECTION ( 'NONE',  ( -0.9720229140804139689, 0.000000000000000000, 0.2348860457809708036 ) ) ;
#21551=ORIENTED_EDGE ( 'NONE', *, *, #30337, .F. ) ;
#21552=DIRECTION ( 'NONE',  ( 0.000000000000000000, -0.000000000000000000, -1.000000000000000000 ) ) ;
#21553=EDGE_CURVE ( 'NONE', #48128, #51755, #43208, .T. ) ;
#21555=DIRECTION ( 'NONE',  ( 0.000000000000000000, 0.000000000000000000, 1.000000000000000000 ) ) ;
#21557=EDGE_LOOP ( 'NONE', ( #18457, #15377, #29373, #49636 ) ) ;
#21558=CARTESIAN_POINT ( 'NONE',  ( -49.30901192927172616, -175.3837268820161057, -123.9972451320097093 ) ) ;
#21559=VECTOR ( 'NONE', #49186, 1000.000000000000114 ) ;
#21560=ORIENTED_EDGE ( 'NONE', *, *, #34404, .T. ) ;
#21562=DIRECTION ( 'NONE',  ( 0.000000000000000000, 0.000000000000000000, 1.000000000000000000 ) ) ;
#21563=ORIENTED_EDGE ( 'NONE', *, *, #36950, .T. ) ;
#21564=DIRECTION ( 'NONE',  ( 0.000000000000000000, -1.000000000000000000, 0.000000000000000000 ) ) ;
#21567=VECTOR ( 'NONE', #39815, 999.9999999999998863 ) ;
#21569=AXIS2_PLACEMENT_3D ( 'NONE', #21891, #49506, #10063 ) ;
#21570=CARTESIAN_POINT ( 'NONE',  ( -156.7610986364826999, -193.5000000000000000, -62.45009659481510766 ) ) ;
#21571=AXIS2_PLACEMENT_3D ( 'NONE', #7925, #39973, #23202 ) ;
#21573=CARTESIAN_POINT ( 'NONE',  ( -164.6246685127424882, -189.7472609257535510, -46.20836643930982035 ) ) ;
#21578=LINE ( 'NONE', #1328, #14113 ) ;
#21579=CARTESIAN_POINT ( 'NONE',  ( -96.30460367372253927, -193.5000000000000000, -114.4068333132746176 ) ) ;
#21580=FACE_OUTER_BOUND ( 'NONE', #50458, .T. ) ;
#21581=ORIENTED_EDGE ( 'NONE', *, *, #19689, .F. ) ;
#21582=VERTEX_POINT ( 'NONE', #19808 ) ;
#21585=CARTESIAN_POINT ( 'NONE',  ( -12.13476221271688615, -193.5000000000000000, 119.5996955107804638 ) ) ;
#21586=LINE ( 'NONE', #1611, #22326 ) ;
#21589=DIRECTION ( 'NONE',  ( -0.000000000000000000, 1.000000000000000000, 0.000000000000000000 ) ) ;
#21591=ORIENTED_EDGE ( 'NONE', *, *, #537, .T. ) ;
#21593=CARTESIAN_POINT ( 'NONE',  ( -122.3978016498073202, -183.6283474603465606, -100.8019320314827212 ) ) ;
#21594=DIRECTION ( 'NONE',  ( -0.1182731709213523247, 0.000000000000000000, -0.9929810960135185827 ) ) ;
#21595=ORIENTED_EDGE ( 'NONE', *, *, #23977, .T. ) ;
#21597=AXIS2_PLACEMENT_3D ( 'NONE', #37089, #49198, #43106 ) ;
#21599=DIRECTION ( 'NONE',  ( -0.000000000000000000, 1.000000000000000000, -0.000000000000000000 ) ) ;
#21600=EDGE_CURVE ( 'NONE', #27297, #47014, #11401, .T. ) ;
#21601=AXIS2_PLACEMENT_3D ( 'NONE', #38468, #14047, #2976 ) ;
#21602=DIRECTION ( 'NONE',  ( -0.4031234292879600778, 0.000000000000000000, -0.9151456172430237901 ) ) ;
#21606=AXIS2_PLACEMENT_3D ( 'NONE', #38727, #18770, #26392 ) ;
#21607=AXIS2_PLACEMENT_3D ( 'NONE', #42938, #12427, #48705 ) ;
#21609=DIRECTION ( 'NONE',  ( 0.000000000000000000, 1.000000000000000000, 0.000000000000000000 ) ) ;
#21612=AXIS2_PLACEMENT_3D ( 'NONE', #18346, #34362, #30157 ) ;
#21614=DIRECTION ( 'NONE',  ( -0.000000000000000000, 1.000000000000000000, 0.000000000000000000 ) ) ;
#21616=VECTOR ( 'NONE', #16536, 1000.000000000000000 ) ;
#21617=DIRECTION ( 'NONE',  ( -0.000000000000000000, 1.000000000000000000, -0.000000000000000000 ) ) ;
#21620=ORIENTED_EDGE ( 'NONE', *, *, #46384, .T. ) ;
#21621=CARTESIAN_POINT ( 'NONE',  ( -26.53529504715431031, -175.3837268820161057, 123.0587999703026725 ) ) ;
#21622=DIRECTION ( 'NONE',  ( -0.6300878435817094392, 0.000000000000000000, -0.7765238627180437447 ) ) ;
#21623=CARTESIAN_POINT ( 'NONE',  ( -89.73513343757494454, -193.5000000000000000, -117.9955164924467397 ) ) ;
#21624=ORIENTED_EDGE ( 'NONE', *, *, #30977, .T. ) ;
#21626=DIRECTION ( 'NONE',  ( -0.000000000000000000, 1.000000000000000000, -0.000000000000000000 ) ) ;
#21629=ORIENTED_EDGE ( 'NONE', *, *, #43369, .F. ) ;
#21631=CYLINDRICAL_SURFACE ( 'NONE', #37354, 125.0000000000000000 ) ;
#21638=CARTESIAN_POINT ( 'NONE',  ( -123.6678354051270077, -193.5000000000000000, 99.85818990449067201 ) ) ;
#21640=ORIENTED_EDGE ( 'NONE', *, *, #25312, .F. ) ;
#21642=ORIENTED_EDGE ( 'NONE', *, *, #18982, .F. ) ;
#21643=DIRECTION ( 'NONE',  ( 0.3758275821142422202, 0.000000000000000000, -0.9266896074318318188 ) ) ;
#21646=DIRECTION ( 'NONE',  ( 0.000000000000000000, 1.000000000000000000, 0.000000000000000000 ) ) ;
#21647=AXIS2_PLACEMENT_3D ( 'NONE', #42433, #42709, #21706 ) ;
#21648=ORIENTED_EDGE ( 'NONE', *, *, #21832, .T. ) ;
#21649=CARTESIAN_POINT ( 'NONE',  ( -110.8210171970983140, -193.5000000000000000, 107.1890582354659074 ) ) ;
#21651=CIRCLE ( 'NONE', #35070, 125.0000000000000000 ) ;
#21653=DIRECTION ( 'NONE',  ( -0.000000000000000000, 1.000000000000000000, -0.000000000000000000 ) ) ;
#21655=CARTESIAN_POINT ( 'NONE',  ( -82.67254833784559764, -183.6283474603465606, -120.2323164553483963 ) ) ;
#21656=DIRECTION ( 'NONE',  ( -0.000000000000000000, 1.000000000000000000, -0.000000000000000000 ) ) ;
#21658=ADVANCED_FACE ( 'NONE', ( #39519 ), #31901, .T. ) ;
#21659=ORIENTED_EDGE ( 'NONE', *, *, #17667, .F. ) ;
#21665=VERTEX_POINT ( 'NONE', #46925 ) ;
#21666=DIRECTION ( 'NONE',  ( -0.000000000000000000, 1.000000000000000000, -0.000000000000000000 ) ) ;
#21667=VERTEX_POINT ( 'NONE', #24017 ) ;
#21674=LINE ( 'NONE', #8787, #40782 ) ;
#21676=AXIS2_PLACEMENT_3D ( 'NONE', #48174, #51870, #47914 ) ;
#21678=DIRECTION ( 'NONE',  ( -0.9374196611341254481, 0.000000000000000000, 0.3482016354343867026 ) ) ;
#21679=ORIENTED_EDGE ( 'NONE', *, *, #6019, .F. ) ;
#21680=FACE_OUTER_BOUND ( 'NONE', #29747, .T. ) ;
#21681=DIRECTION ( 'NONE',  ( -0.9027978299657477557, 0.000000000000000000, 0.4300652022765115712 ) ) ;
#21685=EDGE_LOOP ( 'NONE', ( #25548, #43727, #15075, #2058 ) ) ;
#21686=ORIENTED_EDGE ( 'NONE', *, *, #3831, .F. ) ;
#21687=EDGE_LOOP ( 'NONE', ( #2567, #883, #8661, #41852 ) ) ;
#21693=DIRECTION ( 'NONE',  ( -0.000000000000000000, 1.000000000000000000, 0.000000000000000000 ) ) ;
#21698=ORIENTED_EDGE ( 'NONE', *, *, #24333, .F. ) ;
#21699=CARTESIAN_POINT ( 'NONE',  ( -48.47912675150885065, -183.6283474603465606, 6.938893903907228378E-15 ) ) ;
#21700=ORIENTED_EDGE ( 'NONE', *, *, #45218, .F. ) ;
#21702=AXIS2_PLACEMENT_3D ( 'NONE', #22932, #50797, #14278 ) ;
#21703=EDGE_CURVE ( 'NONE', #7739, #30234, #41786, .T. ) ;
#21704=DIRECTION ( 'NONE',  ( 0.000000000000000000, 1.000000000000000000, -0.000000000000000000 ) ) ;
#21706=DIRECTION ( 'NONE',  ( 0.000000000000000000, 0.000000000000000000, 1.000000000000000000 ) ) ;
#21707=AXIS2_PLACEMENT_3D ( 'NONE', #27085, #14507, #50260 ) ;
#21708=CARTESIAN_POINT ( 'NONE',  ( 19.33815737959698566, -177.1207230881787780, 105.0038855142078091 ) ) ;
#21709=FACE_OUTER_BOUND ( 'NONE', #30662, .T. ) ;
#21710=ORIENTED_EDGE ( 'NONE', *, *, #19774, .T. ) ;
#21713=ORIENTED_EDGE ( 'NONE', *, *, #6738, .F. ) ;
#21714=CARTESIAN_POINT ( 'NONE',  ( -47.66663987350317200, -193.5000000000000000, -0.5829794791144634614 ) ) ;
#21715=VECTOR ( 'NONE', #14908, 1000.000000000000000 ) ;
#21718=LINE ( 'NONE', #37736, #40751 ) ;
#21719=DIRECTION ( 'NONE',  ( 0.8124868780056742068, 0.000000000000000000, 0.5829794791144820021 ) ) ;
#21720=DIRECTION ( 'NONE',  ( 0.7575112421616236880, 0.000000000000000000, -0.6528221181905174975 ) ) ;
#21721=DIRECTION ( 'NONE',  ( 0.000000000000000000, -1.000000000000000000, 0.000000000000000000 ) ) ;
#21722=VECTOR ( 'NONE', #2037, 1000.000000000000114 ) ;
#21723=FACE_OUTER_BOUND ( 'NONE', #44660, .T. ) ;
#21724=LINE ( 'NONE', #13318, #12280 ) ;
#21726=LINE ( 'NONE', #10144, #12197 ) ;
#21727=ORIENTED_EDGE ( 'NONE', *, *, #20800, .F. ) ;
#21728=ORIENTED_EDGE ( 'NONE', *, *, #43566, .T. ) ;
#21729=DIRECTION ( 'NONE',  ( 0.9374196611341183427, 0.000000000000000000, 0.3482016354344059095 ) ) ;
#21731=DIRECTION ( 'NONE',  ( -0.000000000000000000, 1.000000000000000000, -0.000000000000000000 ) ) ;
#21732=VECTOR ( 'NONE', #11619, 1000.000000000000000 ) ;
#21733=VECTOR ( 'NONE', #37568, 1000.000000000000000 ) ;
#21734=PLANE ( 'NONE',  #1608 ) ;
#21735=DIRECTION ( 'NONE',  ( 0.000000000000000000, 0.000000000000000000, 1.000000000000000000 ) ) ;
#21737=CIRCLE ( 'NONE', #32643, 124.9999999999999858 ) ;
#21741=ORIENTED_EDGE ( 'NONE', *, *, #46082, .T. ) ;
#21743=ORIENTED_EDGE ( 'NONE', *, *, #27236, .T. ) ;
#21744=CARTESIAN_POINT ( 'NONE',  ( -48.93575598890257794, -175.3837268820161057, 0.8896570909947506545 ) ) ;
#21745=VECTOR ( 'NONE', #25925, 1000.000000000000000 ) ;
#21746=DIRECTION ( 'NONE',  ( -0.7765238627180349740, 0.000000000000000000, -0.6300878435817203194 ) ) ;
#21749=DIRECTION ( 'NONE',  ( 0.9995608365087942371, 0.000000000000000000, 0.02963332782256331357 ) ) ;
#21750=FACE_OUTER_BOUND ( 'NONE', #45108, .T. ) ;
#21752=ADVANCED_FACE ( 'NONE', ( #4307 ), #36101, .T. ) ;
#21754=AXIS2_PLACEMENT_3D ( 'NONE', #50230, #13954, #2389 ) ;
#21756=DIRECTION ( 'NONE',  ( 0.000000000000000000, 0.000000000000000000, 1.000000000000000000 ) ) ;
#21757=VERTEX_POINT ( 'NONE', #16676 ) ;
#21758=CARTESIAN_POINT ( 'NONE',  ( -48.47912675150885065, -183.6283474603465606, 6.938893903907228378E-15 ) ) ;
#21759=ORIENTED_EDGE ( 'NONE', *, *, #38703, .T. ) ;
#21761=EDGE_CURVE ( 'NONE', #51645, #35821, #40548, .T. ) ;
#21763=DIRECTION ( 'NONE',  ( -0.000000000000000000, 1.000000000000000000, 0.000000000000000000 ) ) ;
#21765=ORIENTED_EDGE ( 'NONE', *, *, #19211, .F. ) ;
#21766=EDGE_CURVE ( 'NONE', #29802, #12404, #41651, .T. ) ;
#21767=CARTESIAN_POINT ( 'NONE',  ( 21.49274850782854074, -193.5000000000000000, -103.5805805771126700 ) ) ;
#21768=DIRECTION ( 'NONE',  ( -0.000000000000000000, 1.000000000000000000, -0.000000000000000000 ) ) ;
#21771=ORIENTED_EDGE ( 'NONE', *, *, #16071, .T. ) ;
#21773=CARTESIAN_POINT ( 'NONE',  ( -48.47912675150885065, -177.1207230881787780, 6.938893903907228378E-15 ) ) ;
#21775=VECTOR ( 'NONE', #5193, 1000.000000000000227 ) ;
#21776=DIRECTION ( 'NONE',  ( 0.000000000000000000, 0.000000000000000000, 1.000000000000000000 ) ) ;
#21778=EDGE_LOOP ( 'NONE', ( #44224, #38876, #33477, #12078 ) ) ;
#21779=DIRECTION ( 'NONE',  ( 0.9890401873221654760, 0.000000000000000000, -0.1476465640024710868 ) ) ;
#21780=AXIS2_PLACEMENT_3D ( 'NONE', #23807, #23309, #3322 ) ;
#21781=DIRECTION ( 'NONE',  ( -0.000000000000000000, 1.000000000000000000, -0.000000000000000000 ) ) ;
#21782=DIRECTION ( 'NONE',  ( 0.5085311186492216251, 0.000000000000000000, -0.8610436117673548884 ) ) ;
#21784=ORIENTED_EDGE ( 'NONE', *, *, #20873, .T. ) ;
#21786=DIRECTION ( 'NONE',  ( -0.000000000000000000, 1.000000000000000000, -0.000000000000000000 ) ) ;
#21787=DIRECTION ( 'NONE',  ( -0.000000000000000000, -1.000000000000000000, 0.000000000000000000 ) ) ;
#21788=ORIENTED_EDGE ( 'NONE', *, *, #1448, .F. ) ;
#21790=VERTEX_POINT ( 'NONE', #876 ) ;
#21791=CARTESIAN_POINT ( 'NONE',  ( -49.08592689732745384, -193.5000000000000000, 0.7948544414133550395 ) ) ;
#21792=DIRECTION ( 'NONE',  ( -0.8455960035018311727, 0.000000000000000000, 0.5338233779647826305 ) ) ;
#21793=CARTESIAN_POINT ( 'NONE',  ( -173.4460699164830260, -189.7472609257535510, -2.874563619423202265 ) ) ;
#21794=ORIENTED_EDGE ( 'NONE', *, *, #13771, .F. ) ;
#21795=LINE ( 'NONE', #33363, #12828 ) ;
#21797=AXIS2_PLACEMENT_3D ( 'NONE', #21161, #41386, #49025 ) ;
#21799=CARTESIAN_POINT ( 'NONE',  ( -126.8597349762179931, -193.5000000000000000, -96.08646119223955395 ) ) ;
#21801=CARTESIAN_POINT ( 'NONE',  ( 29.40217425202905588, -193.5000000000000000, -96.49160960477044569 ) ) ;
#21802=EDGE_CURVE ( 'NONE', #40321, #50633, #34933, .T. ) ;
#21803=EDGE_CURVE ( 'NONE', #41454, #5269, #97, .T. ) ;
#21804=ADVANCED_FACE ( 'NONE', ( #36359 ), #44510, .T. ) ;
#21805=CARTESIAN_POINT ( 'NONE',  ( -129.4514457347087557, -189.7472609257535510, 95.22858582633116953 ) ) ;
#21807=FACE_OUTER_BOUND ( 'NONE', #2941, .T. ) ;
#21808=ORIENTED_EDGE ( 'NONE', *, *, #490, .T. ) ;
#21809=EDGE_CURVE ( 'NONE', #42763, #14211, #48471, .T. ) ;
#21811=ORIENTED_EDGE ( 'NONE', *, *, #27902, .F. ) ;
#21812=CARTESIAN_POINT ( 'NONE',  ( 32.59960422616972409, -175.3837268820161057, -93.82025162277999186 ) ) ;
#21813=VECTOR ( 'NONE', #8020, 1000.000000000000000 ) ;
#21814=EDGE_LOOP ( 'NONE', ( #1749, #48245, #22319, #7781 ) ) ;
#21815=EDGE_CURVE ( 'NONE', #41523, #44900, #28721, .T. ) ;
#21816=CARTESIAN_POINT ( 'NONE',  ( -145.4373324222574126, -193.5000000000000000, -78.89300572996837957 ) ) ;
#21817=VERTEX_POINT ( 'NONE', #44776 ) ;
#21818=ADVANCED_FACE ( 'NONE', ( #33196 ), #32157, .T. ) ;
#21819=EDGE_CURVE ( 'NONE', #19493, #25155, #8759, .T. ) ;
#21822=CARTESIAN_POINT ( 'NONE',  ( -48.47912675150885065, -177.1207230881787780, 6.938893903907228378E-15 ) ) ;
#21823=ORIENTED_EDGE ( 'NONE', *, *, #5448, .F. ) ;
#21824=LINE ( 'NONE', #40998, #40089 ) ;
#21826=ORIENTED_EDGE ( 'NONE', *, *, #15331, .T. ) ;
#21827=EDGE_CURVE ( 'NONE', #27512, #32747, #37456, .T. ) ;
#21829=ORIENTED_EDGE ( 'NONE', *, *, #44486, .T. ) ;
#21831=ORIENTED_EDGE ( 'NONE', *, *, #4123, .F. ) ;
#21832=EDGE_CURVE ( 'NONE', #2077, #42496, #47565, .T. ) ;
#21835=DIRECTION ( 'NONE',  ( 0.000000000000000000, 0.000000000000000000, 1.000000000000000000 ) ) ;
#21838=EDGE_CURVE ( 'NONE', #3688, #2653, #16497, .T. ) ;
#21839=VECTOR ( 'NONE', #48704, 1000.000000000000000 ) ;
#21840=VECTOR ( 'NONE', #24555, 1000.000000000000000 ) ;
#21841=DIRECTION ( 'NONE',  ( -0.8124868780056863082, 0.000000000000000000, 0.5829794791144649047 ) ) ;
#21842=DIRECTION ( 'NONE',  ( 0.000000000000000000, 0.000000000000000000, 1.000000000000000000 ) ) ;
#21843=DIRECTION ( 'NONE',  ( -0.000000000000000000, 1.000000000000000000, -0.000000000000000000 ) ) ;
#21844=ORIENTED_EDGE ( 'NONE', *, *, #10555, .T. ) ;
#21845=CARTESIAN_POINT ( 'NONE',  ( -47.70260288879081401, -193.5000000000000000, 0.6300878435817218737 ) ) ;
#21846=DIRECTION ( 'NONE',  ( 0.000000000000000000, 0.000000000000000000, -1.000000000000000000 ) ) ;
#21847=DIRECTION ( 'NONE',  ( 0.000000000000000000, 0.000000000000000000, 1.000000000000000000 ) ) ;
#21848=CARTESIAN_POINT ( 'NONE',  ( -48.18706998087188254, -193.5000000000000000, 0.9564009842765313074 ) ) ;
#21851=ADVANCED_FACE ( 'NONE', ( #22153 ), #25837, .T. ) ;
#21852=DIRECTION ( 'NONE',  ( -0.6528221181905280446, 0.000000000000000000, 0.7575112421616145841 ) ) ;
#21853=EDGE_CURVE ( 'NONE', #3589, #32593, #49763, .T. ) ;
#21854=CARTESIAN_POINT ( 'NONE',  ( -47.63353074800702558, -183.6283474603465606, -0.5338233779647817423 ) ) ;
#21856=VECTOR ( 'NONE', #34645, 1000.000000000000000 ) ;
#21859=LINE ( 'NONE', #22108, #6753 ) ;
#21860=DIRECTION ( 'NONE',  ( -0.000000000000000000, 1.000000000000000000, 0.000000000000000000 ) ) ;
#21862=CARTESIAN_POINT ( 'NONE',  ( -101.5170032742336446, -177.1207230881787780, 112.0852863853383212 ) ) ;
#21864=CARTESIAN_POINT ( 'NONE',  ( -59.16959496120700379, -177.1207230881787780, 123.5388265266452237 ) ) ;
#21869=VECTOR ( 'NONE', #33699, 1000.000000000000000 ) ;
#21870=EDGE_CURVE ( 'NONE', #9658, #8272, #10072, .T. ) ;
#21871=AXIS2_PLACEMENT_3D ( 'NONE', #33150, #49197, #4524 ) ;
#21872=EDGE_CURVE ( 'NONE', #3584, #25092, #33717, .T. ) ;
#21876=VERTEX_POINT ( 'NONE', #30038 ) ;
#21878=CARTESIAN_POINT ( 'NONE',  ( -162.7543581613524282, -183.6283474603465606, 50.65739320402011003 ) ) ;
#21879=FACE_OUTER_BOUND ( 'NONE', #1669, .T. ) ;
#21885=ORIENTED_EDGE ( 'NONE', *, *, #37390, .T. ) ;
#21888=ORIENTED_EDGE ( 'NONE', *, *, #42548, .F. ) ;
#21890=VERTEX_POINT ( 'NONE', #45563 ) ;
#21891=CARTESIAN_POINT ( 'NONE',  ( -124.1938582159088327, -193.5000000000000000, -99.45993886622791536 ) ) ;
#21892=CARTESIAN_POINT ( 'NONE',  ( 46.01898237923984425, -183.6283474603465606, -81.82363577055903647 ) ) ;
#21893=CARTESIAN_POINT ( 'NONE',  ( 53.18081239921338721, -193.5000000000000000, -72.73415134495935774 ) ) ;
#21896=EDGE_LOOP ( 'NONE', ( #39581, #28949, #42862, #27714 ) ) ;
#21898=CARTESIAN_POINT ( 'NONE',  ( -158.3442440847887269, -175.3837268820161057, -59.62093586438114556 ) ) ;
#21901=VECTOR ( 'NONE', #45825, 1000.000000000000000 ) ;
#21902=VERTEX_POINT ( 'NONE', #49516 ) ;
#21904=DIRECTION ( 'NONE',  ( -0.9646355819083556327, 0.000000000000000000, -0.2635871660690782825 ) ) ;
#21905=AXIS2_PLACEMENT_3D ( 'NONE', #28617, #21010, #44665 ) ;
#21906=VERTEX_POINT ( 'NONE', #34487 ) ;
#21907=LINE ( 'NONE', #42650, #35807 ) ;
#21908=ORIENTED_EDGE ( 'NONE', *, *, #49139, .F. ) ;
#21912=ORIENTED_EDGE ( 'NONE', *, *, #49555, .T. ) ;
#21913=CARTESIAN_POINT ( 'NONE',  ( -107.1845112550870027, -193.5000000000000000, 109.2239789693437331 ) ) ;
#21914=DIRECTION ( 'NONE',  ( 0.000000000000000000, -1.000000000000000000, 0.000000000000000000 ) ) ;
#21915=PLANE ( 'NONE',  #48411 ) ;
#21919=VERTEX_POINT ( 'NONE', #2445 ) ;
#21920=VECTOR ( 'NONE', #43519, 1000.000000000000000 ) ;
#21922=DIRECTION ( 'NONE',  ( 0.000000000000000000, -0.000000000000000000, -1.000000000000000000 ) ) ;
#21923=ORIENTED_EDGE ( 'NONE', *, *, #31118, .T. ) ;
#21925=EDGE_CURVE ( 'NONE', #4153, #26290, #2176, .T. ) ;
#21927=VERTEX_POINT ( 'NONE', #5622 ) ;
#21931=CARTESIAN_POINT ( 'NONE',  ( -173.3294908491238004, -183.6283474603465606, -6.114457023560960991 ) ) ;
#21934=CARTESIAN_POINT ( 'NONE',  ( 8.448131207122518305, -189.7472609257535510, 111.2847127925100068 ) ) ;
#21935=ORIENTED_EDGE ( 'NONE', *, *, #44612, .F. ) ;
#21936=VERTEX_POINT ( 'NONE', #9810 ) ;
#21937=VECTOR ( 'NONE', #18241, 1000.000000000000000 ) ;
#21938=ORIENTED_EDGE ( 'NONE', *, *, #26241, .T. ) ;
#21939=DIRECTION ( 'NONE',  ( 0.9785564922995032555, 0.000000000000000000, 0.2059786187411021818 ) ) ;
#21941=ADVANCED_FACE ( 'NONE', ( #37667 ), #5883, .F. ) ;
#21942=DIRECTION ( 'NONE',  ( -0.8124868780056825335, 0.000000000000000000, 0.5829794791144703447 ) ) ;
#21947=DIRECTION ( 'NONE',  ( -0.000000000000000000, 1.000000000000000000, 0.000000000000000000 ) ) ;
#21949=AXIS2_PLACEMENT_3D ( 'NONE', #12418, #20564, #15602 ) ;
#21950=LINE ( 'NONE', #49568, #17479 ) ;
#21951=EDGE_CURVE ( 'NONE', #23290, #8865, #20689, .T. ) ;
#21952=PLANE ( 'NONE',  #44170 ) ;
#21954=FACE_OUTER_BOUND ( 'NONE', #9076, .T. ) ;
#21957=EDGE_CURVE ( 'NONE', #20647, #10130, #1919, .T. ) ;
#21959=EDGE_LOOP ( 'NONE', ( #14282, #23801, #45664, #1858 ) ) ;
#21962=DIRECTION ( 'NONE',  ( 0.000000000000000000, 0.000000000000000000, -1.000000000000000000 ) ) ;
#21963=EDGE_LOOP ( 'NONE', ( #15693, #19025, #16493, #34443 ) ) ;
#21964=VECTOR ( 'NONE', #36711, 1000.000000000000000 ) ;
#21966=DIRECTION ( 'NONE',  ( 0.000000000000000000, -1.000000000000000000, 0.000000000000000000 ) ) ;
#21967=DIRECTION ( 'NONE',  ( 0.000000000000000000, 1.000000000000000000, -0.000000000000000000 ) ) ;
#21968=VECTOR ( 'NONE', #13889, 1000.000000000000000 ) ;
#21971=EDGE_CURVE ( 'NONE', #29510, #28239, #31595, .T. ) ;
#21975=FACE_OUTER_BOUND ( 'NONE', #32904, .T. ) ;
#21976=ORIENTED_EDGE ( 'NONE', *, *, #10249, .T. ) ;
#21977=ORIENTED_EDGE ( 'NONE', *, *, #25687, .T. ) ;
#21981=VECTOR ( 'NONE', #20038, 999.9999999999998863 ) ;
#21983=FACE_OUTER_BOUND ( 'NONE', #16820, .T. ) ;
#21984=VECTOR ( 'NONE', #1888, 1000.000000000000227 ) ;
#21987=CARTESIAN_POINT ( 'NONE',  ( -36.09284319799462537, -177.1207230881787780, 124.3848060646152476 ) ) ;
#21989=VERTEX_POINT ( 'NONE', #50793 ) ;
#21990=CARTESIAN_POINT ( 'NONE',  ( -14.52059121095390992, -177.1207230881787780, 119.2602935412682399 ) ) ;
#21991=CARTESIAN_POINT ( 'NONE',  ( -106.2948367055610106, -193.5000000000000000, -110.8257356506552185 ) ) ;
#21993=VERTEX_POINT ( 'NONE', #46859 ) ;
#21994=ORIENTED_EDGE ( 'NONE', *, *, #25234, .F. ) ;
#21995=DIRECTION ( 'NONE',  ( 0.000000000000000000, 0.000000000000000000, -1.000000000000000000 ) ) ;
#21996=DIRECTION ( 'NONE',  ( -0.000000000000000000, 1.000000000000000000, -0.000000000000000000 ) ) ;
#21997=EDGE_CURVE ( 'NONE', #36797, #172, #19252, .T. ) ;
#21998=DIRECTION ( 'NONE',  ( -0.000000000000000000, 1.000000000000000000, -0.000000000000000000 ) ) ;
#22000=DIRECTION ( 'NONE',  ( 0.000000000000000000, -1.000000000000000000, -0.000000000000000000 ) ) ;
#22001=CIRCLE ( 'NONE', #15289, 125.0000000000000000 ) ;
#22002=EDGE_LOOP ( 'NONE', ( #4411, #14118, #17304, #32024 ) ) ;
#22003=EDGE_CURVE ( 'NONE', #33649, #38645, #35011, .T. ) ;
#22006=VERTEX_POINT ( 'NONE', #47884 ) ;
#22007=FACE_OUTER_BOUND ( 'NONE', #26275, .T. ) ;
#22010=ORIENTED_EDGE ( 'NONE', *, *, #25783, .F. ) ;
#22011=DIRECTION ( 'NONE',  ( 0.000000000000000000, -1.000000000000000000, 0.000000000000000000 ) ) ;
#22012=ORIENTED_EDGE ( 'NONE', *, *, #47987, .T. ) ;
#22013=CARTESIAN_POINT ( 'NONE',  ( -48.93575598890255662, -177.1207230881787780, -0.8896570909947461026 ) ) ;
#22014=PLANE ( 'NONE',  #15018 ) ;
#22016=CARTESIAN_POINT ( 'NONE',  ( -48.47912675150885065, -175.3837268820161057, 6.938893903907228378E-15 ) ) ;
#22018=VECTOR ( 'NONE', #19217, 1000.000000000000000 ) ;
#22019=VECTOR ( 'NONE', #34798, 1000.000000000000000 ) ;
#22020=ORIENTED_EDGE ( 'NONE', *, *, #47791, .T. ) ;
#22022=VECTOR ( 'NONE', #708, 1000.000000000000114 ) ;
#22024=CARTESIAN_POINT ( 'NONE',  ( -94.25732089370191602, -177.1207230881787780, 116.3157639405754935 ) ) ;
#22027=CARTESIAN_POINT ( 'NONE',  ( -144.8751831225492310, -175.3837268820161057, 77.99872144864771428 ) ) ;
#22029=EDGE_CURVE ( 'NONE', #27228, #45277, #6896, .T. ) ;
#22032=ORIENTED_EDGE ( 'NONE', *, *, #16836, .F. ) ;
#22034=PLANE ( 'NONE',  #26489 ) ;
#22035=LINE ( 'NONE', #9965, #29085 ) ;
#22037=EDGE_LOOP ( 'NONE', ( #517, #15002, #21223, #1797 ) ) ;
#22041=VERTEX_POINT ( 'NONE', #2948 ) ;
#22042=CARTESIAN_POINT ( 'NONE',  ( 25.43954814678888710, -177.1207230881787780, 100.8019320314832754 ) ) ;
#22043=EDGE_CURVE ( 'NONE', #28733, #23058, #18729, .T. ) ;
#22044=ORIENTED_EDGE ( 'NONE', *, *, #12505, .T. ) ;
#22045=EDGE_CURVE ( 'NONE', #24942, #41052, #11615, .T. ) ;
#22046=AXIS2_PLACEMENT_3D ( 'NONE', #38906, #18438, #30504 ) ;
#22047=FACE_OUTER_BOUND ( 'NONE', #14944, .T. ) ;
#22049=DIRECTION ( 'NONE',  ( -0.1768902751225802927, 0.000000000000000000, 0.9842305779475953864 ) ) ;
#22050=DIRECTION ( 'NONE',  ( 0.9027978299657446470, 0.000000000000000000, -0.4300652022765183435 ) ) ;
#22051=EDGE_CURVE ( 'NONE', #51292, #24976, #50947, .T. ) ;
#22053=CARTESIAN_POINT ( 'NONE',  ( -48.47912675150885065, -177.1207230881787780, 6.938893903907228378E-15 ) ) ;
#22054=VECTOR ( 'NONE', #37753, 1000.000000000000114 ) ;
#22055=ORIENTED_EDGE ( 'NONE', *, *, #10772, .F. ) ;
#22057=ORIENTED_EDGE ( 'NONE', *, *, #46917, .F. ) ;
#22058=CARTESIAN_POINT ( 'NONE',  ( -48.18706998087188254, -193.5000000000000000, 0.9564009842765313074 ) ) ;
#22061=ORIENTED_EDGE ( 'NONE', *, *, #13146, .F. ) ;
#22062=DIRECTION ( 'NONE',  ( -0.6300878435817094392, 0.000000000000000000, -0.7765238627180437447 ) ) ;
#22064=FACE_OUTER_BOUND ( 'NONE', #44278, .T. ) ;
#22065=DIRECTION ( 'NONE',  ( 0.000000000000000000, 0.000000000000000000, 1.000000000000000000 ) ) ;
#22068=CYLINDRICAL_SURFACE ( 'NONE', #24750, 125.0000000000000000 ) ;
#22070=FACE_OUTER_BOUND ( 'NONE', #47387, .T. ) ;
#22071=VERTEX_POINT ( 'NONE', #22928 ) ;
#22072=CARTESIAN_POINT ( 'NONE',  ( -161.8276685539205744, -177.1207230881787780, 50.28156562190587664 ) ) ;
#22073=VECTOR ( 'NONE', #48214, 1000.000000000000000 ) ;
#22074=EDGE_LOOP ( 'NONE', ( #33740, #31540, #18253, #19815 ) ) ;
#22076=CARTESIAN_POINT ( 'NONE',  ( -109.9568094315246185, -177.1207230881787780, -108.8370090194290754 ) ) ;
#22077=LINE ( 'NONE', #26021, #47483 ) ;
#22078=ORIENTED_EDGE ( 'NONE', *, *, #46441, .F. ) ;
#22079=EDGE_LOOP ( 'NONE', ( #43828, #49428, #28879, #2878 ) ) ;
#22080=VECTOR ( 'NONE', #4023, 1000.000000000000000 ) ;
#22081=DIRECTION ( 'NONE',  ( -0.4827922027307427477, 0.000000000000000000, -0.8757349421956379665 ) ) ;
#22082=ORIENTED_EDGE ( 'NONE', *, *, #19539, .F. ) ;
#22083=PLANE ( 'NONE',  #45502 ) ;
#22086=EDGE_CURVE ( 'NONE', #44410, #6055, #11340, .T. ) ;
#22091=DIRECTION ( 'NONE',  ( 0.000000000000000000, -0.000000000000000000, -1.000000000000000000 ) ) ;
#22093=EDGE_CURVE ( 'NONE', #14725, #27177, #26572, .T. ) ;
#22094=ORIENTED_EDGE ( 'NONE', *, *, #34306, .T. ) ;
#22095=ADVANCED_FACE ( 'NONE', ( #6654 ), #7154, .T. ) ;
#22097=CIRCLE ( 'NONE', #17041, 125.0000000000000000 ) ;
#22098=PLANE ( 'NONE',  #22943 ) ;
#22100=DIRECTION ( 'NONE',  ( -0.1182731709213523247, 0.000000000000000000, -0.9929810960135185827 ) ) ;
#22101=ADVANCED_FACE ( 'NONE', ( #31318 ), #47361, .T. ) ;
#22102=CARTESIAN_POINT ( 'NONE',  ( 70.49476099643867144, -183.6283474603465606, 34.94873081740416865 ) ) ;
#22103=VERTEX_POINT ( 'NONE', #7664 ) ;
#22104=CIRCLE ( 'NONE', #23743, 125.0000000000000000 ) ;
#22106=EDGE_CURVE ( 'NONE', #19400, #44532, #3460, .T. ) ;
#22107=CARTESIAN_POINT ( 'NONE',  ( -106.4764934152196645, -213.5000000000000000, -110.7307791902283043 ) ) ;
#22108=CARTESIAN_POINT ( 'NONE',  ( 17.15229921100054611, -183.6283474603465606, -106.3838142112212921 ) ) ;
#22111=EDGE_CURVE ( 'NONE', #48301, #17063, #19744, .T. ) ;
#22112=EDGE_CURVE ( 'NONE', #9601, #30050, #4351, .T. ) ;
#22114=EDGE_CURVE ( 'NONE', #6993, #49807, #44557, .T. ) ;
#22116=LINE ( 'NONE', #37881, #37981 ) ;
#22117=DIRECTION ( 'NONE',  ( -0.000000000000000000, 1.000000000000000000, -0.000000000000000000 ) ) ;
#22118=AXIS2_PLACEMENT_3D ( 'NONE', #39282, #4066, #35081 ) ;
#22119=EDGE_CURVE ( 'NONE', #4209, #35348, #3569, .T. ) ;
#22120=ORIENTED_EDGE ( 'NONE', *, *, #33724, .F. ) ;
#22121=CARTESIAN_POINT ( 'NONE',  ( -2.174401709722253440, -183.6283474603465606, -115.0304316645280096 ) ) ;
#22122=EDGE_CURVE ( 'NONE', #20850, #25612, #24074, .T. ) ;
#22124=CARTESIAN_POINT ( 'NONE',  ( -49.17567778057185990, -175.3837268820161057, 0.7175072570443320474 ) ) ;
#22126=ORIENTED_EDGE ( 'NONE', *, *, #28128, .F. ) ;
#22128=ORIENTED_EDGE ( 'NONE', *, *, #4359, .F. ) ;
#22130=PLANE ( 'NONE',  #27785 ) ;
#22132=AXIS2_PLACEMENT_3D ( 'NONE', #5612, #16666, #32673 ) ;
#22133=ORIENTED_EDGE ( 'NONE', *, *, #49530, .T. ) ;
#22135=DIRECTION ( 'NONE',  ( 0.000000000000000000, -1.000000000000000000, 0.000000000000000000 ) ) ;
#22137=DIRECTION ( 'NONE',  ( 0.9473263538541876194, 0.000000000000000000, 0.3202698538628486746 ) ) ;
#22138=CARTESIAN_POINT ( 'NONE',  ( 56.77503207194100554, -175.3837268820161057, -67.42819922234311036 ) ) ;
#22141=CARTESIAN_POINT ( 'NONE',  ( -80.17897391495031911, -193.5000000000000000, 120.9136869416132498 ) ) ;
#22143=DIRECTION ( 'NONE',  ( 0.000000000000000000, 0.000000000000000000, 1.000000000000000000 ) ) ;
#22144=ORIENTED_EDGE ( 'NONE', *, *, #30976, .T. ) ;
#22147=LINE ( 'NONE', #21893, #8097 ) ;
#22148=ADVANCED_FACE ( 'NONE', ( #142 ), #43525, .T. ) ;
#22149=ORIENTED_EDGE ( 'NONE', *, *, #46754, .T. ) ;
#22150=FACE_OUTER_BOUND ( 'NONE', #28335, .T. ) ;
#22153=FACE_OUTER_BOUND ( 'NONE', #50320, .T. ) ;
#22155=EDGE_CURVE ( 'NONE', #38089, #33159, #8954, .T. ) ;
#22156=EDGE_CURVE ( 'NONE', #43203, #7649, #4794, .T. ) ;
#22157=VERTEX_POINT ( 'NONE', #31692 ) ;
#22160=ADVANCED_FACE ( 'NONE', ( #40090 ), #44033, .T. ) ;
#22161=ORIENTED_EDGE ( 'NONE', *, *, #50844, .T. ) ;
#22163=ORIENTED_EDGE ( 'NONE', *, *, #42974, .F. ) ;
#22164=CARTESIAN_POINT ( 'NONE',  ( -46.06708674231131084, -193.5000000000000000, -124.9767260852756863 ) ) ;
#22167=DIRECTION ( 'NONE',  ( -0.000000000000000000, 1.000000000000000000, -0.000000000000000000 ) ) ;
#22169=CARTESIAN_POINT ( 'NONE',  ( 24.63024857337166296, -193.5000000000000000, 101.3904297239426597 ) ) ;
#22170=VECTOR ( 'NONE', #18194, 1000.000000000000000 ) ;
#22172=DIRECTION ( 'NONE',  ( -0.000000000000000000, 1.000000000000000000, -0.000000000000000000 ) ) ;
#22175=FACE_OUTER_BOUND ( 'NONE', #19947, .T. ) ;
#22177=LINE ( 'NONE', #18243, #6045 ) ;
#22179=EDGE_CURVE ( 'NONE', #51005, #34028, #35896, .T. ) ;
#22180=ORIENTED_EDGE ( 'NONE', *, *, #40145, .F. ) ;
#22182=EDGE_CURVE ( 'NONE', #36635, #45987, #32468, .T. ) ;
#22184=ORIENTED_EDGE ( 'NONE', *, *, #19532, .T. ) ;
#22185=LINE ( 'NONE', #38473, #23910 ) ;
#22186=VERTEX_POINT ( 'NONE', #8300 ) ;
#22189=VECTOR ( 'NONE', #2674, 1000.000000000000114 ) ;
#22190=AXIS2_PLACEMENT_3D ( 'NONE', #48608, #8641, #45437 ) ;
#22191=CARTESIAN_POINT ( 'NONE',  ( -123.0610352593084400, -175.3837268820161057, 99.06333546307732263 ) ) ;
#22192=DIRECTION ( 'NONE',  ( 0.000000000000000000, 0.000000000000000000, 1.000000000000000000 ) ) ;
#22196=ORIENTED_EDGE ( 'NONE', *, *, #41593, .F. ) ;
#22198=DIRECTION ( 'NONE',  ( 0.000000000000000000, 0.000000000000000000, 1.000000000000000000 ) ) ;
#22199=DIRECTION ( 'NONE',  ( -0.5829794791144703447, 0.000000000000000000, -0.8124868780056825335 ) ) ;
#22200=LINE ( 'NONE', #26909, #44862 ) ;
#22201=VERTEX_POINT ( 'NONE', #24325 ) ;
#22202=CIRCLE ( 'NONE', #48209, 125.0000000000000000 ) ;
#22203=CARTESIAN_POINT ( 'NONE',  ( 72.31641062551800303, -189.7472609257535510, 32.14713283941990341 ) ) ;
#22207=CARTESIAN_POINT ( 'NONE',  ( -114.9451385648675767, -183.6283474603465606, -104.6823626202120181 ) ) ;
#22210=EDGE_CURVE ( 'NONE', #44850, #2592, #8036, .T. ) ;
#22211=LINE ( 'NONE', #17520, #782 ) ;
#22212=EDGE_CURVE ( 'NONE', #17102, #19374, #32727, .T. ) ;
#22214=DIRECTION ( 'NONE',  ( 0.000000000000000000, -1.000000000000000000, 0.000000000000000000 ) ) ;
#22215=ORIENTED_EDGE ( 'NONE', *, *, #45149, .F. ) ;
#22216=EDGE_LOOP ( 'NONE', ( #29883, #18167, #35614, #3262 ) ) ;
#22217=FACE_OUTER_BOUND ( 'NONE', #8390, .T. ) ;
#22218=LINE ( 'NONE', #1988, #8527 ) ;
#22219=EDGE_LOOP ( 'NONE', ( #21938, #49431, #21686, #1600 ) ) ;
#22220=AXIS2_PLACEMENT_3D ( 'NONE', #51296, #42879, #38927 ) ;
#22221=AXIS2_PLACEMENT_3D ( 'NONE', #23889, #35718, #51773 ) ;
#22222=LINE ( 'NONE', #50607, #49217 ) ;
#22224=PLANE ( 'NONE',  #31572 ) ;
#22229=ADVANCED_FACE ( 'NONE', ( #28512 ), #27740, .T. ) ;
#22230=CYLINDRICAL_SURFACE ( 'NONE', #16818, 125.0000000000000000 ) ;
#22231=ORIENTED_EDGE ( 'NONE', *, *, #1190, .F. ) ;
#22232=ORIENTED_EDGE ( 'NONE', *, *, #13966, .F. ) ;
#22233=FACE_OUTER_BOUND ( 'NONE', #321, .T. ) ;
#22234=AXIS2_PLACEMENT_3D ( 'NONE', #39264, #31626, #3770 ) ;
#22235=ORIENTED_EDGE ( 'NONE', *, *, #19070, .F. ) ;
#22236=EDGE_CURVE ( 'NONE', #11493, #46287, #46740, .T. ) ;
#22237=LINE ( 'NONE', #21214, #23460 ) ;
#22242=LINE ( 'NONE', #13585, #36124 ) ;
#22245=ORIENTED_EDGE ( 'NONE', *, *, #11556, .T. ) ;
#22246=ORIENTED_EDGE ( 'NONE', *, *, #3694, .F. ) ;
#22248=DIRECTION ( 'NONE',  ( -0.3482016354343928088, 0.000000000000000000, -0.9374196611341231167 ) ) ;
#22249=VECTOR ( 'NONE', #18086, 1000.000000000000227 ) ;
#22250=SURFACE_SIDE_STYLE ('',( #18331 ) ) ;
#22251=AXIS2_PLACEMENT_3D ( 'NONE', #26919, #17816, #18784 ) ;
#22252=LINE ( 'NONE', #5469, #37929 ) ;
#22254=EDGE_LOOP ( 'NONE', ( #33447, #698, #38783, #32077 ) ) ;
#22255=CIRCLE ( 'NONE', #21401, 125.0000000000000000 ) ;
#22256=CIRCLE ( 'NONE', #51643, 125.0000000000000000 ) ;
#22257=EDGE_CURVE ( 'NONE', #42284, #16002, #41908, .T. ) ;
#22258=DIRECTION ( 'NONE',  ( 0.000000000000000000, 0.000000000000000000, 1.000000000000000000 ) ) ;
#22262=EDGE_LOOP ( 'NONE', ( #25051, #46005, #3909, #24686 ) ) ;
#22263=CARTESIAN_POINT ( 'NONE',  ( -58.29063029684667185, -183.6283474603465606, 124.6143426664034877 ) ) ;
#22264=CIRCLE ( 'NONE', #7189, 125.0000000000000000 ) ;
#22265=ORIENTED_EDGE ( 'NONE', *, *, #20245, .T. ) ;
#22266=LINE ( 'NONE', #50921, #2328 ) ;
#22267=VECTOR ( 'NONE', #2721, 1000.000000000000000 ) ;
#22269=CARTESIAN_POINT ( 'NONE',  ( -48.30223647638627682, -193.5000000000000000, -0.9842305779475897243 ) ) ;
#22272=ORIENTED_EDGE ( 'NONE', *, *, #29337, .T. ) ;
#22273=DIRECTION ( 'NONE',  ( 0.000000000000000000, 1.000000000000000000, -0.000000000000000000 ) ) ;
#22274=VECTOR ( 'NONE', #38865, 1000.000000000000000 ) ;
#22276=CIRCLE ( 'NONE', #8843, 125.0000000000000000 ) ;
#22277=VERTEX_POINT ( 'NONE', #17226 ) ;
#22278=CARTESIAN_POINT ( 'NONE',  ( 32.49319223169170101, -189.7472609257535510, -95.22858582633061530 ) ) ;
#22281=DIRECTION ( 'NONE',  ( 0.000000000000000000, 0.000000000000000000, -1.000000000000000000 ) ) ;
#22284=DIRECTION ( 'NONE',  ( -0.000000000000000000, 1.000000000000000000, -0.000000000000000000 ) ) ;
#22285=CARTESIAN_POINT ( 'NONE',  ( -171.0948786228703398, -193.5000000000000000, -18.47640724094508258 ) ) ;
#22287=ORIENTED_EDGE ( 'NONE', *, *, #43060, .T. ) ;
#22288=PLANE ( 'NONE',  #11221 ) ;
#22290=CARTESIAN_POINT ( 'NONE',  ( -172.6359455740846442, -177.1207230881787780, -14.49428645563791562 ) ) ;
#22295=CIRCLE ( 'NONE', #27316, 125.0000000000000000 ) ;
#22297=PLANE ( 'NONE',  #2584 ) ;
#22298=ORIENTED_EDGE ( 'NONE', *, *, #34380, .T. ) ;
#22299=CARTESIAN_POINT ( 'NONE',  ( -147.0463339291296165, -177.1207230881787780, 76.87330921200147316 ) ) ;
#22301=CYLINDRICAL_SURFACE ( 'NONE', #20916, 125.0000000000000000 ) ;
#22308=PLANE ( 'NONE',  #5880 ) ;
#22309=ORIENTED_EDGE ( 'NONE', *, *, #21971, .T. ) ;
#22310=CARTESIAN_POINT ( 'NONE',  ( 50.08808042611237710, -193.5000000000000000, -76.87330921200083367 ) ) ;
#22312=VECTOR ( 'NONE', #40540, 1000.000000000000000 ) ;
#22315=LINE ( 'NONE', #10232, #9972 ) ;
#22316=ADVANCED_FACE ( 'NONE', ( #49024 ), #37963, .T. ) ;
#22317=CARTESIAN_POINT ( 'NONE',  ( -81.14588623932564815, -183.6283474603465606, 120.6560517527617833 ) ) ;
#22319=ORIENTED_EDGE ( 'NONE', *, *, #48074, .T. ) ;
#22320=CARTESIAN_POINT ( 'NONE',  ( -78.64590280292341617, -189.7472609257535510, -121.3052580173827408 ) ) ;
#22321=CARTESIAN_POINT ( 'NONE',  ( -48.47912675150885065, -183.6283474603465606, 6.938893903907228378E-15 ) ) ;
#22322=ORIENTED_EDGE ( 'NONE', *, *, #20435, .F. ) ;
#22326=VECTOR ( 'NONE', #17648, 1000.000000000000000 ) ;
#22327=ORIENTED_EDGE ( 'NONE', *, *, #20136, .F. ) ;
#22331=EDGE_CURVE ( 'NONE', #33929, #14578, #16542, .T. ) ;
#22335=ORIENTED_EDGE ( 'NONE', *, *, #43042, .T. ) ;
#22338=EDGE_CURVE ( 'NONE', #41080, #47840, #25117, .T. ) ;
#22340=ORIENTED_EDGE ( 'NONE', *, *, #8914, .T. ) ;
#22341=CARTESIAN_POINT ( 'NONE',  ( -140.8230258362169707, -175.3837268820161057, 84.24728067916045404 ) ) ;
#22342=ADVANCED_FACE ( 'NONE', ( #13282 ), #21419, .T. ) ;
#22343=DIRECTION ( 'NONE',  ( -0.000000000000000000, 1.000000000000000000, -0.000000000000000000 ) ) ;
#22344=VERTEX_POINT ( 'NONE', #17750 ) ;
#22345=EDGE_CURVE ( 'NONE', #5747, #33733, #44818, .T. ) ;
#22346=AXIS2_PLACEMENT_3D ( 'NONE', #44803, #5385, #21139 ) ;
#22347=CARTESIAN_POINT ( 'NONE',  ( -172.4728835572423975, -177.1207230881787780, 1.322128892812083123 ) ) ;
#22348=DIRECTION ( 'NONE',  ( -0.000000000000000000, 1.000000000000000000, -0.000000000000000000 ) ) ;
#22349=DIRECTION ( 'NONE',  ( 0.000000000000000000, -0.000000000000000000, 1.000000000000000000 ) ) ;
#22350=DIRECTION ( 'NONE',  ( 0.9995608365087942371, 0.000000000000000000, 0.02963332782256331357 ) ) ;
#22351=AXIS2_PLACEMENT_3D ( 'NONE', #1418, #8512, #40828 ) ;
#22353=CARTESIAN_POINT ( 'NONE',  ( -55.05561436132770581, -189.7472609257535510, 124.8268793598474105 ) ) ;
#22356=VECTOR ( 'NONE', #10939, 1000.000000000000000 ) ;
#22357=LINE ( 'NONE', #31261, #20415 ) ;
#22359=AXIS2_PLACEMENT_3D ( 'NONE', #11161, #3024, #26691 ) ;
#22360=PLANE ( 'NONE',  #30446 ) ;
#22361=ORIENTED_EDGE ( 'NONE', *, *, #1448, .T. ) ;
#22362=DIRECTION ( 'NONE',  ( 0.000000000000000000, -1.000000000000000000, 0.000000000000000000 ) ) ;
#22365=CARTESIAN_POINT ( 'NONE',  ( -0.6536498292959382894, -193.5000000000000000, 114.4068333132749160 ) ) ;
#22366=EDGE_LOOP ( 'NONE', ( #1431, #20325, #3430, #5851 ) ) ;
#22367=DIRECTION ( 'NONE',  ( 0.000000000000000000, 0.000000000000000000, -1.000000000000000000 ) ) ;
#22371=CARTESIAN_POINT ( 'NONE',  ( -49.03777351731250889, -175.3837268820161057, 0.8294056854502042109 ) ) ;
#22372=PLANE ( 'NONE',  #20317 ) ;
#22375=CARTESIAN_POINT ( 'NONE',  ( -24.23284180386169950, -193.5000000000000000, -121.6072260099953581 ) ) ;
#22377=ORIENTED_EDGE ( 'NONE', *, *, #11810, .F. ) ;
#22379=ORIENTED_EDGE ( 'NONE', *, *, #14171, .F. ) ;
#22382=FACE_OUTER_BOUND ( 'NONE', #8959, .T. ) ;
#22384=AXIS2_PLACEMENT_3D ( 'NONE', #42510, #2825, #46990 ) ;
#22388=CARTESIAN_POINT ( 'NONE',  ( 62.59443091842027940, -193.5000000000000000, -57.33816169485140790 ) ) ;
#22391=ORIENTED_EDGE ( 'NONE', *, *, #51826, .T. ) ;
#22392=EDGE_CURVE ( 'NONE', #35941, #4690, #29815, .T. ) ;
#22393=AXIS2_PLACEMENT_3D ( 'NONE', #51823, #24462, #28652 ) ;
#22396=DIRECTION ( 'NONE',  ( 0.000000000000000000, 0.000000000000000000, -1.000000000000000000 ) ) ;
#22397=DIRECTION ( 'NONE',  ( -0.000000000000000000, 1.000000000000000000, -0.000000000000000000 ) ) ;
#22398=ORIENTED_EDGE ( 'NONE', *, *, #1048, .T. ) ;
#22402=DIRECTION ( 'NONE',  ( 0.000000000000000000, 1.000000000000000000, 0.000000000000000000 ) ) ;
#22403=ORIENTED_EDGE ( 'NONE', *, *, #4421, .T. ) ;
#22404=DIRECTION ( 'NONE',  ( 0.000000000000000000, 0.000000000000000000, -1.000000000000000000 ) ) ;
#22407=DIRECTION ( 'NONE',  ( -0.3758275821142488260, 0.000000000000000000, 0.9266896074318291543 ) ) ;
#22408=EDGE_CURVE ( 'NONE', #24976, #18993, #13798, .T. ) ;
#22409=FACE_OUTER_BOUND ( 'NONE', #6115, .T. ) ;
#22410=VECTOR ( 'NONE', #17474, 1000.000000000000000 ) ;
#22412=DIRECTION ( 'NONE',  ( -0.000000000000000000, 1.000000000000000000, -0.000000000000000000 ) ) ;
#22414=EDGE_CURVE ( 'NONE', #11641, #21393, #29998, .T. ) ;
#22415=DIRECTION ( 'NONE',  ( -0.000000000000000000, 1.000000000000000000, -0.000000000000000000 ) ) ;
#22417=CARTESIAN_POINT ( 'NONE',  ( -47.63353074800703268, -177.1207230881787780, 0.5338233779648018373 ) ) ;
#22418=CIRCLE ( 'NONE', #50111, 125.0000000000000000 ) ;
#22420=EDGE_CURVE ( 'NONE', #28114, #23398, #7345, .T. ) ;
#22421=ORIENTED_EDGE ( 'NONE', *, *, #46537, .F. ) ;
#22423=DIRECTION ( 'NONE',  ( 0.000000000000000000, -0.000000000000000000, -1.000000000000000000 ) ) ;
#22427=AXIS2_PLACEMENT_3D ( 'NONE', #19092, #11186, #30378 ) ;
#22428=DIRECTION ( 'NONE',  ( -0.2348860457809911206, 0.000000000000000000, 0.9720229140804089729 ) ) ;
#22429=VECTOR ( 'NONE', #38667, 1000.000000000000000 ) ;
#22431=ORIENTED_EDGE ( 'NONE', *, *, #29493, .T. ) ;
#22434=DIRECTION ( 'NONE',  ( 0.000000000000000000, 0.000000000000000000, -1.000000000000000000 ) ) ;
#22436=CARTESIAN_POINT ( 'NONE',  ( 40.30419662299490113, -193.5000000000000000, -87.99159897727903967 ) ) ;
#22437=AXIS2_PLACEMENT_3D ( 'NONE', #854, #45024, #48440 ) ;
#22438=EDGE_CURVE ( 'NONE', #3300, #27708, #34529, .T. ) ;
#22439=ORIENTED_EDGE ( 'NONE', *, *, #6398, .F. ) ;
#22441=VECTOR ( 'NONE', #37601, 1000.000000000000000 ) ;
#22444=PLANE ( 'NONE',  #3365 ) ;
#22445=PLANE ( 'NONE',  #1007 ) ;
#22447=ORIENTED_EDGE ( 'NONE', *, *, #18247, .F. ) ;
#22448=DIRECTION ( 'NONE',  ( 0.2348860457809842095, 0.000000000000000000, -0.9720229140804107493 ) ) ;
#22449=ADVANCED_FACE ( 'NONE', ( #2488 ), #26657, .T. ) ;
#22450=FACE_OUTER_BOUND ( 'NONE', #40374, .T. ) ;
#22451=AXIS2_PLACEMENT_3D ( 'NONE', #21044, #30155, #46203 ) ;
#22453=VERTEX_POINT ( 'NONE', #50328 ) ;
#22454=FACE_OUTER_BOUND ( 'NONE', #11117, .T. ) ;
#22456=CARTESIAN_POINT ( 'NONE',  ( -48.47912675150885065, -175.3837268820161057, 6.938893903907228378E-15 ) ) ;
#22458=AXIS2_PLACEMENT_3D ( 'NONE', #4098, #32719, #8293 ) ;
#22459=ADVANCED_FACE ( 'NONE', ( #26904 ), #2732, .T. ) ;
#22460=EDGE_CURVE ( 'NONE', #18213, #47040, #30081, .T. ) ;
#22463=CARTESIAN_POINT ( 'NONE',  ( 66.42899531795131907, -193.5000000000000000, 49.20491319441622124 ) ) ;
#22464=CARTESIAN_POINT ( 'NONE',  ( -167.4530144994566285, -183.6283474603465606, -34.94873081740328757 ) ) ;
#22465=ORIENTED_EDGE ( 'NONE', *, *, #38782, .F. ) ;
#22466=EDGE_LOOP ( 'NONE', ( #52000, #6414, #1530, #10809 ) ) ;
#22468=ORIENTED_EDGE ( 'NONE', *, *, #6092, .F. ) ;
#22469=FACE_OUTER_BOUND ( 'NONE', #50113, .T. ) ;
#22470=CARTESIAN_POINT ( 'NONE',  ( -48.02249751411513756, -183.6283474603465606, -0.8896570909947397743 ) ) ;
#22472=AXIS2_PLACEMENT_3D ( 'NONE', #40999, #40470, #5021 ) ;
#22473=ADVANCED_FACE ( 'NONE', ( #22469 ), #14317, .T. ) ;
#22474=EDGE_CURVE ( 'NONE', #15796, #17439, #11131, .T. ) ;
#22475=VECTOR ( 'NONE', #26402, 999.9999999999998863 ) ;
#22476=LINE ( 'NONE', #13801, #51409 ) ;
#22478=ORIENTED_EDGE ( 'NONE', *, *, #48652, .T. ) ;
#22480=ADVANCED_FACE ( 'NONE', ( #10365 ), #30860, .F. ) ;
#22481=DIRECTION ( 'NONE',  ( -0.5586467658036594619, 0.000000000000000000, 0.8294056854501971054 ) ) ;
#22483=AXIS2_PLACEMENT_3D ( 'NONE', #32020, #19420, #35442 ) ;
#22484=ORIENTED_EDGE ( 'NONE', *, *, #3052, .T. ) ;
#22487=DIRECTION ( 'NONE',  ( -0.8294056854502011022, 0.000000000000000000, -0.5586467658036535777 ) ) ;
#22488=DIRECTION ( 'NONE',  ( -0.05924062789370006937, 0.000000000000000000, -0.9982437317643222396 ) ) ;
#22490=DIRECTION ( 'NONE',  ( -0.000000000000000000, 1.000000000000000000, -0.000000000000000000 ) ) ;
#22491=CARTESIAN_POINT ( 'NONE',  ( -140.1460956102404509, -175.3837268820161057, 84.98333260264821831 ) ) ;
#22492=ORIENTED_EDGE ( 'NONE', *, *, #40415, .T. ) ;
#22493=LINE ( 'NONE', #38508, #5780 ) ;
#22494=EDGE_CURVE ( 'NONE', #13319, #37838, #22972, .T. ) ;
#22495=EDGE_LOOP ( 'NONE', ( #34822, #15053, #43896, #31633 ) ) ;
#22498=VECTOR ( 'NONE', #24407, 1000.000000000000000 ) ;
#22499=DIRECTION ( 'NONE',  ( -0.000000000000000000, 1.000000000000000000, 0.000000000000000000 ) ) ;
#22500=ORIENTED_EDGE ( 'NONE', *, *, #9928, .T. ) ;
#22501=CIRCLE ( 'NONE', #4032, 125.0000000000000000 ) ;
#22502=DIRECTION ( 'NONE',  ( 0.4031234292879665171, 0.000000000000000000, 0.9151456172430210145 ) ) ;
#22503=CARTESIAN_POINT ( 'NONE',  ( -98.10897907742933910, -189.7472609257535510, 114.7252272087849434 ) ) ;
#22507=DIRECTION ( 'NONE',  ( 0.000000000000000000, 0.000000000000000000, 1.000000000000000000 ) ) ;
#22508=ORIENTED_EDGE ( 'NONE', *, *, #19277, .T. ) ;
#22509=VECTOR ( 'NONE', #34771, 1000.000000000000000 ) ;
#22511=ORIENTED_EDGE ( 'NONE', *, *, #32294, .T. ) ;
#22512=ORIENTED_EDGE ( 'NONE', *, *, #22093, .F. ) ;
#22515=VECTOR ( 'NONE', #4762, 1000.000000000000000 ) ;
#22516=FACE_OUTER_BOUND ( 'NONE', #7640, .T. ) ;
#22517=ORIENTED_EDGE ( 'NONE', *, *, #19428, .T. ) ;
#22518=DIRECTION ( 'NONE',  ( 0.000000000000000000, 0.000000000000000000, -1.000000000000000000 ) ) ;
#22521=CARTESIAN_POINT ( 'NONE',  ( -41.96187976958283627, -175.3837268820161057, -123.8286356280830205 ) ) ;
#22522=EDGE_CURVE ( 'NONE', #35097, #11813, #14068, .T. ) ;
#22523=EDGE_CURVE ( 'NONE', #40799, #38866, #7961, .T. ) ;
#22525=FACE_OUTER_BOUND ( 'NONE', #2600, .T. ) ;
#22526=VERTEX_POINT ( 'NONE', #20056 ) ;
#22528=ORIENTED_EDGE ( 'NONE', *, *, #29837, .T. ) ;
#22529=DIRECTION ( 'NONE',  ( -0.2920567706369628924, 0.000000000000000000, -0.9564009842765264224 ) ) ;
#22530=VECTOR ( 'NONE', #5620, 1000.000000000000000 ) ;
#22531=LINE ( 'NONE', #38546, #40255 ) ;
#22533=VECTOR ( 'NONE', #40996, 1000.000000000000000 ) ;
#22534=DIRECTION ( 'NONE',  ( 0.000000000000000000, -0.000000000000000000, 1.000000000000000000 ) ) ;
#22538=AXIS2_PLACEMENT_3D ( 'NONE', #21621, #851, #1892 ) ;
#22539=DIRECTION ( 'NONE',  ( 0.000000000000000000, -1.000000000000000000, 0.000000000000000000 ) ) ;
#22540=ORIENTED_EDGE ( 'NONE', *, *, #23560, .T. ) ;
#22541=LINE ( 'NONE', #14385, #5522 ) ;
#22542=EDGE_LOOP ( 'NONE', ( #19281, #30040, #45330, #26334 ) ) ;
#22543=AXIS2_PLACEMENT_3D ( 'NONE', #29165, #45225, #21287 ) ;
#22545=CARTESIAN_POINT ( 'NONE',  ( 63.54086012517504400, -189.7472609257535510, -53.17445600718541954 ) ) ;
#22546=EDGE_CURVE ( 'NONE', #38453, #33832, #40267, .T. ) ;
#22547=ORIENTED_EDGE ( 'NONE', *, *, #11561, .T. ) ;
#22548=CARTESIAN_POINT ( 'NONE',  ( 59.29945538372744807, -177.1207230881787780, 63.31490529818492519 ) ) ;
#22549=LINE ( 'NONE', #50155, #50650 ) ;
#22554=EDGE_CURVE ( 'NONE', #39207, #50756, #41741, .T. ) ;
#22555=AXIS2_PLACEMENT_3D ( 'NONE', #26203, #34104, #9418 ) ;
#22556=ORIENTED_EDGE ( 'NONE', *, *, #21085, .T. ) ;
#22558=DIRECTION ( 'NONE',  ( -0.9646355819083556327, 0.000000000000000000, -0.2635871660690782825 ) ) ;
#22559=DIRECTION ( 'NONE',  ( 0.7378332790417333475, 0.000000000000000000, -0.6749830015182038956 ) ) ;
#22560=ORIENTED_EDGE ( 'NONE', *, *, #32645, .T. ) ;
#22561=PLANE ( 'NONE',  #8303 ) ;
#22563=CARTESIAN_POINT ( 'NONE',  ( -89.73513343757494454, -183.6283474603465606, -117.9955164924467397 ) ) ;
#22566=CARTESIAN_POINT ( 'NONE',  ( -109.5001801941309338, -193.5000000000000000, -107.9473519284343155 ) ) ;
#22567=DIRECTION ( 'NONE',  ( 0.000000000000000000, -0.000000000000000000, 1.000000000000000000 ) ) ;
#22570=ORIENTED_EDGE ( 'NONE', *, *, #9578, .F. ) ;
#22571=AXIS2_PLACEMENT_3D ( 'NONE', #4310, #8502, #12447 ) ;
#22573=CARTESIAN_POINT ( 'NONE',  ( -171.7300019102062549, -177.1207230881787780, -20.83798868929510562 ) ) ;
#22574=AXIS2_PLACEMENT_3D ( 'NONE', #44956, #40995, #9721 ) ;
#22576=VERTEX_POINT ( 'NONE', #4284 ) ;
#22578=VERTEX_POINT ( 'NONE', #15875 ) ;
#22579=AXIS2_PLACEMENT_3D ( 'NONE', #9397, #40924, #21995 ) ;
#22582=DIRECTION ( 'NONE',  ( -0.7378332790417333475, 0.000000000000000000, 0.6749830015182038956 ) ) ;
#22583=CARTESIAN_POINT ( 'NONE',  ( -77.43961373357959133, -189.7472609257535510, -120.5706864261535145 ) ) ;
#22584=EDGE_CURVE ( 'NONE', #36852, #38638, #12424, .T. ) ;
#22585=LINE ( 'NONE', #37575, #30210 ) ;
#22586=VERTEX_POINT ( 'NONE', #51878 ) ;
#22587=VECTOR ( 'NONE', #42500, 1000.000000000000000 ) ;
#22589=ORIENTED_EDGE ( 'NONE', *, *, #39063, .F. ) ;
#22590=DIRECTION ( 'NONE',  ( -0.8610436117673621048, 0.000000000000000000, 0.5085311186492095237 ) ) ;
#22592=DIRECTION ( 'NONE',  ( -0.7765238627180437447, 0.000000000000000000, 0.6300878435817094392 ) ) ;
#22593=DIRECTION ( 'NONE',  ( 0.000000000000000000, 0.000000000000000000, 1.000000000000000000 ) ) ;
#22595=VERTEX_POINT ( 'NONE', #43714 ) ;
#22598=ORIENTED_EDGE ( 'NONE', *, *, #29619, .T. ) ;
#22599=AXIS2_PLACEMENT_3D ( 'NONE', #6803, #11506, #27533 ) ;
#22600=EDGE_CURVE ( 'NONE', #36650, #35348, #12152, .T. ) ;
#22602=ORIENTED_EDGE ( 'NONE', *, *, #5432, .T. ) ;
#22603=CARTESIAN_POINT ( 'NONE',  ( -48.47912675150885065, -175.3837268820161057, 6.938893903907228378E-15 ) ) ;
#22605=ORIENTED_EDGE ( 'NONE', *, *, #19828, .F. ) ;
#22606=CARTESIAN_POINT ( 'NONE',  ( 22.73247662810271308, -177.1207230881787780, -101.5140743725395254 ) ) ;
#22608=CARTESIAN_POINT ( 'NONE',  ( -48.47912675150885065, -183.6283474603465606, 6.938893903907228378E-15 ) ) ;
#22609=ORIENTED_EDGE ( 'NONE', *, *, #32930, .F. ) ;
#22611=DIRECTION ( 'NONE',  ( 0.9785564922995017012, 0.000000000000000000, 0.2059786187411094538 ) ) ;
#22612=ORIENTED_EDGE ( 'NONE', *, *, #28833, .T. ) ;
#22613=CARTESIAN_POINT ( 'NONE',  ( -156.7610986364826999, -177.1207230881787780, -62.45009659481509345 ) ) ;
#22614=DIRECTION ( 'NONE',  ( 0.8757349421956345248, 0.000000000000000000, 0.4827922027307490205 ) ) ;
#22615=ORIENTED_EDGE ( 'NONE', *, *, #15210, .T. ) ;
#22617=DIRECTION ( 'NONE',  ( 0.000000000000000000, -1.000000000000000000, 0.000000000000000000 ) ) ;
#22619=DIRECTION ( 'NONE',  ( -0.000000000000000000, 1.000000000000000000, -0.000000000000000000 ) ) ;
#22620=CARTESIAN_POINT ( 'NONE',  ( -43.48323084606168720, -183.6283474603465606, 124.9001241957026167 ) ) ;
#22622=EDGE_CURVE ( 'NONE', #26421, #17429, #40529, .T. ) ;
#22623=DIRECTION ( 'NONE',  ( -0.000000000000000000, 1.000000000000000000, -0.000000000000000000 ) ) ;
#22624=LINE ( 'NONE', #50741, #5542 ) ;
#22628=CARTESIAN_POINT ( 'NONE',  ( 28.62116745695382392, -177.1207230881787780, -97.11716833071837129 ) ) ;
#22630=DIRECTION ( 'NONE',  ( 0.000000000000000000, 0.000000000000000000, -1.000000000000000000 ) ) ;
#22631=EDGE_CURVE ( 'NONE', #35575, #16039, #24510, .T. ) ;
#22633=EDGE_LOOP ( 'NONE', ( #46605, #2991, #2436, #29898 ) ) ;
#22635=AXIS2_PLACEMENT_3D ( 'NONE', #43818, #48031, #12012 ) ;
#22637=FACE_OUTER_BOUND ( 'NONE', #36855, .T. ) ;
#22639=VERTEX_POINT ( 'NONE', #7469 ) ;
#22640=EDGE_CURVE ( 'NONE', #43567, #41906, #24119, .T. ) ;
#22641=LINE ( 'NONE', #5130, #5049 ) ;
#22642=EDGE_CURVE ( 'NONE', #45491, #43537, #15350, .T. ) ;
#22643=CARTESIAN_POINT ( 'NONE',  ( -0.3054481938615447034, -183.6283474603465606, 115.3442529744090592 ) ) ;
#22644=EDGE_LOOP ( 'NONE', ( #33222, #7392, #29575, #33802 ) ) ;
#22645=ORIENTED_EDGE ( 'NONE', *, *, #32772, .F. ) ;
#22649=LINE ( 'NONE', #39185, #42948 ) ;
#22650=LINE ( 'NONE', #38662, #48168 ) ;
#22652=AXIS2_PLACEMENT_3D ( 'NONE', #50638, #38274, #42215 ) ;
#22654=DIRECTION ( 'NONE',  ( -0.000000000000000000, 1.000000000000000000, -0.000000000000000000 ) ) ;
#22656=DIRECTION ( 'NONE',  ( -0.000000000000000000, 1.000000000000000000, -0.000000000000000000 ) ) ;
#22657=CARTESIAN_POINT ( 'NONE',  ( -98.71382891444390850, -189.7472609257535510, -114.4616734920523839 ) ) ;
#22661=EDGE_LOOP ( 'NONE', ( #6585, #7654, #4357, #31748 ) ) ;
#22663=ORIENTED_EDGE ( 'NONE', *, *, #15111, .F. ) ;
#22665=DIRECTION ( 'NONE',  ( -0.000000000000000000, 1.000000000000000000, -0.000000000000000000 ) ) ;
#22666=CARTESIAN_POINT ( 'NONE',  ( -91.49662025983752756, -175.3837268820161057, -116.2991637277475405 ) ) ;
#22668=ORIENTED_EDGE ( 'NONE', *, *, #46933, .F. ) ;
#22669=PLANE ( 'NONE',  #14769 ) ;
#22670=CARTESIAN_POINT ( 'NONE',  ( -94.25732089370191602, -193.5000000000000000, 116.3157639405754935 ) ) ;
#22672=ORIENTED_EDGE ( 'NONE', *, *, #7668, .T. ) ;
#22673=DIRECTION ( 'NONE',  ( -0.000000000000000000, 1.000000000000000000, -0.000000000000000000 ) ) ;
#22674=CARTESIAN_POINT ( 'NONE',  ( -129.9529520667707914, -193.5000000000000000, -94.79987230211959570 ) ) ;
#22675=ORIENTED_EDGE ( 'NONE', *, *, #8310, .F. ) ;
#22677=CARTESIAN_POINT ( 'NONE',  ( -48.47912675150885065, -189.7472609257535510, 124.0000000000000142 ) ) ;
#22680=CARTESIAN_POINT ( 'NONE',  ( 28.62116745695382392, -183.6283474603465606, -97.11716833071837129 ) ) ;
#22681=ORIENTED_EDGE ( 'NONE', *, *, #3632, .F. ) ;
#22682=LINE ( 'NONE', #15574, #28126 ) ;
#22683=CARTESIAN_POINT ( 'NONE',  ( 141.7825277784304205, -213.5000000000000000, 10.00000000000000178 ) ) ;
#22684=ORIENTED_EDGE ( 'NONE', *, *, #385, .T. ) ;
#22685=DIRECTION ( 'NONE',  ( -0.000000000000000000, 1.000000000000000000, -0.000000000000000000 ) ) ;
#22686=ADVANCED_FACE ( 'NONE', ( #47405 ), #11385, .T. ) ;
#22687=CARTESIAN_POINT ( 'NONE',  ( -48.64924157374594671, -175.3837268820161057, 124.9998842437354227 ) ) ;
#22690=VERTEX_POINT ( 'NONE', #48183 ) ;
#22692=PLANE ( 'NONE',  #40501 ) ;
#22693=DIRECTION ( 'NONE',  ( -0.5085311186492154079, 0.000000000000000000, -0.8610436117673585521 ) ) ;
#22696=ORIENTED_EDGE ( 'NONE', *, *, #15396, .F. ) ;
#22697=VERTEX_POINT ( 'NONE', #3505 ) ;
#22701=CARTESIAN_POINT ( 'NONE',  ( -48.47912675150885065, -177.1207230881787780, 6.938893903907228378E-15 ) ) ;
#22702=ORIENTED_EDGE ( 'NONE', *, *, #43042, .F. ) ;
#22703=EDGE_CURVE ( 'NONE', #29336, #51798, #12675, .T. ) ;
#22704=VECTOR ( 'NONE', #41955, 1000.000000000000000 ) ;
#22706=ORIENTED_EDGE ( 'NONE', *, *, #24677, .T. ) ;
#22708=LINE ( 'NONE', #46632, #19970 ) ;
#22709=EDGE_CURVE ( 'NONE', #44232, #27933, #48703, .T. ) ;
#22710=DIRECTION ( 'NONE',  ( 0.000000000000000000, -1.000000000000000000, 0.000000000000000000 ) ) ;
#22712=ORIENTED_EDGE ( 'NONE', *, *, #32867, .T. ) ;
#22713=ORIENTED_EDGE ( 'NONE', *, *, #24495, .T. ) ;
#22714=VERTEX_POINT ( 'NONE', #24775 ) ;
#22716=CARTESIAN_POINT ( 'NONE',  ( -127.0132498732366457, -183.6283474603465606, 97.24912084693259828 ) ) ;
#22718=LINE ( 'NONE', #18007, #7933 ) ;
#22719=ORIENTED_EDGE ( 'NONE', *, *, #19703, .F. ) ;
#22720=AXIS2_PLACEMENT_3D ( 'NONE', #44785, #36637, #44270 ) ;
#22722=CYLINDRICAL_SURFACE ( 'NONE', #24828, 9.999999999999994671 ) ;
#22723=CARTESIAN_POINT ( 'NONE',  ( 73.87536152799695799, -175.3837268820161057, -25.58083653558413317 ) ) ;
#22724=CIRCLE ( 'NONE', #29422, 125.0000000000000000 ) ;
#22725=AXIS2_PLACEMENT_3D ( 'NONE', #27328, #3671, #35464 ) ;
#22726=EDGE_LOOP ( 'NONE', ( #51446, #1725, #5536, #33067 ) ) ;
#22727=ORIENTED_EDGE ( 'NONE', *, *, #32365, .T. ) ;
#22729=FACE_OUTER_BOUND ( 'NONE', #7876, .T. ) ;
#22730=CARTESIAN_POINT ( 'NONE',  ( -47.51449116960048968, -177.1207230881787780, 0.2635871660690785045 ) ) ;
#22732=CARTESIAN_POINT ( 'NONE',  ( 72.35619569422321717, -177.1207230881787780, 27.83926365844748574 ) ) ;
#22735=CARTESIAN_POINT ( 'NONE',  ( -48.71401279728982558, -183.6283474603465606, -0.9720229140804069745 ) ) ;
#22738=LINE ( 'NONE', #18792, #22901 ) ;
#22739=VECTOR ( 'NONE', #6498, 1000.000000000000000 ) ;
#22741=EDGE_LOOP ( 'NONE', ( #38498, #26910, #897, #8417 ) ) ;
#22743=DIRECTION ( 'NONE',  ( 0.000000000000000000, -1.000000000000000000, 0.000000000000000000 ) ) ;
#22744=ADVANCED_FACE ( 'NONE', ( #14119 ), #18319, .T. ) ;
#22750=DIRECTION ( 'NONE',  ( -0.000000000000000000, 1.000000000000000000, -0.000000000000000000 ) ) ;
#22751=ORIENTED_EDGE ( 'NONE', *, *, #34535, .F. ) ;
#22752=ADVANCED_FACE ( 'NONE', ( #35107 ), #47212, .T. ) ;
#22753=CARTESIAN_POINT ( 'NONE',  ( -168.4003408533108086, -193.5000000000000000, -35.26900067126609173 ) ) ;
#22754=LINE ( 'NONE', #45710, #43882 ) ;
#22757=ORIENTED_EDGE ( 'NONE', *, *, #17296, .F. ) ;
#22758=PLANE ( 'NONE',  #6174 ) ;
#22759=ADVANCED_FACE ( 'NONE', ( #42742 ), #38265, .F. ) ;
#22760=VERTEX_POINT ( 'NONE', #51167 ) ;
#22761=ADVANCED_FACE ( 'NONE', ( #14365 ), #34073, .T. ) ;
#22762=AXIS2_PLACEMENT_3D ( 'NONE', #38960, #2969, #35037 ) ;
#22763=LINE ( 'NONE', #39547, #45308 ) ;
#22764=ORIENTED_EDGE ( 'NONE', *, *, #38871, .F. ) ;
#22765=ADVANCED_FACE ( 'NONE', ( #34578 ), #30911, .F. ) ;
#22767=CARTESIAN_POINT ( 'NONE',  ( 40.30419662299490113, -183.6283474603465606, -87.99159897727903967 ) ) ;
#22769=LINE ( 'NONE', #10935, #29124 ) ;
#22772=LINE ( 'NONE', #38781, #24087 ) ;
#22775=EDGE_CURVE ( 'NONE', #29888, #18768, #51802, .T. ) ;
#22776=VERTEX_POINT ( 'NONE', #26708 ) ;
#22777=DIRECTION ( 'NONE',  ( 0.000000000000000000, -1.000000000000000000, 0.000000000000000000 ) ) ;
#22779=AXIS2_PLACEMENT_3D ( 'NONE', #46065, #21622, #45289 ) ;
#22781=DIRECTION ( 'NONE',  ( 0.000000000000000000, 0.000000000000000000, 1.000000000000000000 ) ) ;
#22783=ORIENTED_EDGE ( 'NONE', *, *, #11179, .F. ) ;
#22784=ADVANCED_FACE ( 'NONE', ( #10412 ), #23295, .T. ) ;
#22785=CARTESIAN_POINT ( 'NONE',  ( -48.13092511607445800, -193.5000000000000000, 0.9374196611341301111 ) ) ;
#22786=ORIENTED_EDGE ( 'NONE', *, *, #18307, .F. ) ;
#22787=DIRECTION ( 'NONE',  ( -0.000000000000000000, 1.000000000000000000, -0.000000000000000000 ) ) ;
#22788=EDGE_LOOP ( 'NONE', ( #44496, #3963, #34931, #36031 ) ) ;
#22789=VERTEX_POINT ( 'NONE', #22521 ) ;
#22790=CARTESIAN_POINT ( 'NONE',  ( -48.77118352214583297, -175.3837268820161057, 0.9564009842765270886 ) ) ;
#22791=DIRECTION ( 'NONE',  ( 0.9960498426152171181, 0.000000000000000000, -0.08879589532293157006 ) ) ;
#22792=CIRCLE ( 'NONE', #12683, 125.0000000000000000 ) ;
#22793=DIRECTION ( 'NONE',  ( 0.2348860457809775482, 0.000000000000000000, 0.9720229140804121926 ) ) ;
#22794=FACE_OUTER_BOUND ( 'NONE', #41944, .T. ) ;
#22795=ORIENTED_EDGE ( 'NONE', *, *, #37697, .F. ) ;
#22799=AXIS2_PLACEMENT_3D ( 'NONE', #44733, #37095, #41293 ) ;
#22800=VERTEX_POINT ( 'NONE', #38538 ) ;
#22801=CARTESIAN_POINT ( 'NONE',  ( -130.0559183202350084, -189.7472609257535510, -93.38753978496592367 ) ) ;
#22805=DIRECTION ( 'NONE',  ( -0.3758275821142357809, 0.000000000000000000, -0.9266896074318343723 ) ) ;
#22806=CARTESIAN_POINT ( 'NONE',  ( -52.47502265695602119, -193.5000000000000000, -124.9361149384469485 ) ) ;
#22808=EDGE_CURVE ( 'NONE', #44107, #47366, #22769, .T. ) ;
#22810=DIRECTION ( 'NONE',  ( -0.000000000000000000, 1.000000000000000000, -0.000000000000000000 ) ) ;
#22813=DIRECTION ( 'NONE',  ( -0.000000000000000000, 1.000000000000000000, -0.000000000000000000 ) ) ;
#22814=AXIS2_PLACEMENT_3D ( 'NONE', #16431, #8522, #12719 ) ;
#22816=EDGE_CURVE ( 'NONE', #25410, #3029, #14900, .T. ) ;
#22817=FACE_BOUND ( 'NONE', #45239, .T. ) ;
#22818=ORIENTED_EDGE ( 'NONE', *, *, #19038, .F. ) ;
#22820=DIRECTION ( 'NONE',  ( 0.000000000000000000, 1.000000000000000000, -0.000000000000000000 ) ) ;
#22821=CARTESIAN_POINT ( 'NONE',  ( 70.98542830588607444, -183.6283474603465606, -36.78613984829962646 ) ) ;
#22822=VERTEX_POINT ( 'NONE', #43764 ) ;
#22823=DIRECTION ( 'NONE',  ( 0.000000000000000000, 0.000000000000000000, 1.000000000000000000 ) ) ;
#22825=DIRECTION ( 'NONE',  ( 0.000000000000000000, 1.000000000000000000, -0.000000000000000000 ) ) ;
#22826=ADVANCED_FACE ( 'NONE', ( #24318 ), #35358, .T. ) ;
#22827=FACE_OUTER_BOUND ( 'NONE', #6656, .T. ) ;
#22831=CARTESIAN_POINT ( 'NONE',  ( -51.89154260666836649, -193.5000000000000000, 124.9534129907280828 ) ) ;
#22834=VECTOR ( 'NONE', #29220, 1000.000000000000000 ) ;
#22835=ORIENTED_EDGE ( 'NONE', *, *, #10288, .T. ) ;
#22840=FACE_OUTER_BOUND ( 'NONE', #48924, .T. ) ;
#22846=AXIS2_PLACEMENT_3D ( 'NONE', #9519, #42342, #10045 ) ;
#22848=FACE_OUTER_BOUND ( 'NONE', #47129, .T. ) ;
#22849=ORIENTED_EDGE ( 'NONE', *, *, #2816, .F. ) ;
#22850=CARTESIAN_POINT ( 'NONE',  ( -11.80936624585915418, -193.5000000000000000, -119.5003291395395735 ) ) ;
#22852=EDGE_CURVE ( 'NONE', #41498, #26525, #32460, .T. ) ;
#22853=CARTESIAN_POINT ( 'NONE',  ( -8.169009709621407822, -177.1207230881787780, 118.3219948448695504 ) ) ;
#22855=LINE ( 'NONE', #34926, #8138 ) ;
#22856=CARTESIAN_POINT ( 'NONE',  ( 11.66870402553033337, -177.1207230881787780, 108.4360005853211248 ) ) ;
#22858=ORIENTED_EDGE ( 'NONE', *, *, #20147, .F. ) ;
#22859=CARTESIAN_POINT ( 'NONE',  ( -102.9981419485577590, -183.6283474603465606, -111.3726929437936377 ) ) ;
#22862=LINE ( 'NONE', #31002, #24846 ) ;
#22867=DIRECTION ( 'NONE',  ( -0.7765238627180349740, 0.000000000000000000, -0.6300878435817203194 ) ) ;
#22868=ORIENTED_EDGE ( 'NONE', *, *, #34821, .F. ) ;
#22870=EDGE_CURVE ( 'NONE', #8427, #39351, #12391, .T. ) ;
#22872=DIRECTION ( 'NONE',  ( 0.000000000000000000, -1.000000000000000000, 0.000000000000000000 ) ) ;
#22873=VECTOR ( 'NONE', #1881, 999.9999999999998863 ) ;
#22874=CARTESIAN_POINT ( 'NONE',  ( 46.40005841627164074, -193.5000000000000000, 81.38144888055276738 ) ) ;
#22876=DIRECTION ( 'NONE',  ( 0.000000000000000000, -1.000000000000000000, 0.000000000000000000 ) ) ;
#22879=DIRECTION ( 'NONE',  ( 0.9890401873221633666, 0.000000000000000000, 0.1476465640024850756 ) ) ;
#22881=VERTEX_POINT ( 'NONE', #35886 ) ;
#22882=CIRCLE ( 'NONE', #203, 125.0000000000000000 ) ;
#22883=VECTOR ( 'NONE', #44778, 1000.000000000000000 ) ;
#22885=DIRECTION ( 'NONE',  ( 0.000000000000000000, 1.000000000000000000, -0.000000000000000000 ) ) ;
#22886=AXIS2_PLACEMENT_3D ( 'NONE', #5904, #45836, #38705 ) ;
#22888=CARTESIAN_POINT ( 'NONE',  ( -173.1763543514842070, -177.1207230881787780, 8.694908215728892387 ) ) ;
#22889=ADVANCED_FACE ( 'NONE', ( #51668 ), #15410, .F. ) ;
#22890=DIRECTION ( 'NONE',  ( 0.000000000000000000, 0.000000000000000000, -1.000000000000000000 ) ) ;
#22891=DIRECTION ( 'NONE',  ( 0.000000000000000000, -1.000000000000000000, 0.000000000000000000 ) ) ;
#22892=EDGE_LOOP ( 'NONE', ( #24867, #20346, #37245, #5466 ) ) ;
#22896=CARTESIAN_POINT ( 'NONE',  ( -4.794493649713349015, -175.3837268820161057, -117.1181148702518726 ) ) ;
#22897=EDGE_LOOP ( 'NONE', ( #39908, #7767, #7400, #34392 ) ) ;
#22898=ORIENTED_EDGE ( 'NONE', *, *, #5434, .F. ) ;
#22899=ORIENTED_EDGE ( 'NONE', *, *, #493, .F. ) ;
#22901=VECTOR ( 'NONE', #34803, 1000.000000000000000 ) ;
#22903=CARTESIAN_POINT ( 'NONE',  ( -48.71401279728982558, -175.3837268820161057, -0.9720229140804069745 ) ) ;
#22904=CARTESIAN_POINT ( 'NONE',  ( -18.95304271317703382, -175.3837268820161057, -121.4627941443854837 ) ) ;
#22905=EDGE_LOOP ( 'NONE', ( #39440, #14276, #22560, #32048 ) ) ;
#22906=VECTOR ( 'NONE', #9579, 1000.000000000000000 ) ;
#22907=FACE_OUTER_BOUND ( 'NONE', #19936, .T. ) ;
#22908=DIRECTION ( 'NONE',  ( 0.5586467658036415873, 0.000000000000000000, 0.8294056854502090959 ) ) ;
#22909=CARTESIAN_POINT ( 'NONE',  ( 43.18784210722336070, -175.3837268820161057, -84.98333260264753619 ) ) ;
#22910=CARTESIAN_POINT ( 'NONE',  ( 76.09804998693969935, -193.5000000000000000, 10.27263529369908746 ) ) ;
#22911=ORIENTED_EDGE ( 'NONE', *, *, #12673, .T. ) ;
#22912=CARTESIAN_POINT ( 'NONE',  ( 33.25242634436026634, -175.3837268820161057, -94.57776286494161866 ) ) ;
#22916=DIRECTION ( 'NONE',  ( 0.000000000000000000, 0.000000000000000000, 1.000000000000000000 ) ) ;
#22917=CARTESIAN_POINT ( 'NONE',  ( -106.4764934152196645, -213.5000000000000000, 110.7307791902283043 ) ) ;
#22918=CARTESIAN_POINT ( 'NONE',  ( -48.77118352214581876, -193.5000000000000000, -0.9564009842765195391 ) ) ;
#22919=VECTOR ( 'NONE', #43618, 1000.000000000000000 ) ;
#22922=EDGE_CURVE ( 'NONE', #24499, #47079, #23538, .T. ) ;
#22923=ORIENTED_EDGE ( 'NONE', *, *, #7529, .F. ) ;
#22924=VECTOR ( 'NONE', #40507, 1000.000000000000000 ) ;
#22925=CARTESIAN_POINT ( 'NONE',  ( -77.43961373357964817, -193.5000000000000000, -120.5706864261535145 ) ) ;
#22926=CARTESIAN_POINT ( 'NONE',  ( -84.53143451966468547, -193.5000000000000000, -118.6432945265036949 ) ) ;
#22928=CARTESIAN_POINT ( 'NONE',  ( 44.30815888362531041, -189.7472609257535510, 83.75869879877568280 ) ) ;
#22930=ORIENTED_EDGE ( 'NONE', *, *, #5264, .F. ) ;
#22932=CARTESIAN_POINT ( 'NONE',  ( -47.60339180931321579, -189.7472609257535510, 0.4827922027307559594 ) ) ;
#22934=EDGE_CURVE ( 'NONE', #29247, #39853, #49329, .T. ) ;
#22935=LINE ( 'NONE', #2449, #32324 ) ;
#22936=ORIENTED_EDGE ( 'NONE', *, *, #16645, .F. ) ;
#22937=CARTESIAN_POINT ( 'NONE',  ( 73.32083127613157103, -193.5000000000000000, 28.10285082451656535 ) ) ;
#22938=ORIENTED_EDGE ( 'NONE', *, *, #16836, .T. ) ;
#22939=EDGE_CURVE ( 'NONE', #39920, #8260, #16180, .T. ) ;
#22940=LINE ( 'NONE', #10590, #23973 ) ;
#22941=PLANE ( 'NONE',  #8485 ) ;
#22942=ORIENTED_EDGE ( 'NONE', *, *, #13136, .T. ) ;
#22943=AXIS2_PLACEMENT_3D ( 'NONE', #10026, #44268, #45506 ) ;
#22944=DIRECTION ( 'NONE',  ( 0.000000000000000000, 1.000000000000000000, 0.000000000000000000 ) ) ;
#22945=ADVANCED_FACE ( 'NONE', ( #44548 ), #48240, .T. ) ;
#22946=PLANE ( 'NONE',  #14656 ) ;
#22947=CARTESIAN_POINT ( 'NONE',  ( -49.32472275501068282, -189.7472609257535510, 0.5338233779647895139 ) ) ;
#22948=VECTOR ( 'NONE', #37636, 1000.000000000000000 ) ;
#22949=EDGE_LOOP ( 'NONE', ( #33070, #3984, #38151, #15155 ) ) ;
#22950=LINE ( 'NONE', #19006, #35510 ) ;
#22951=PLANE ( 'NONE',  #51318 ) ;
#22953=LINE ( 'NONE', #46360, #28520 ) ;
#22955=ORIENTED_EDGE ( 'NONE', *, *, #37685, .F. ) ;
#22956=VERTEX_POINT ( 'NONE', #8025 ) ;
#22957=CARTESIAN_POINT ( 'NONE',  ( -97.70585564814139445, -189.7472609257535510, 113.8100815915419162 ) ) ;
#22958=VECTOR ( 'NONE', #7421, 1000.000000000000000 ) ;
#22960=ORIENTED_EDGE ( 'NONE', *, *, #3514, .T. ) ;
#22961=AXIS2_PLACEMENT_3D ( 'NONE', #33839, #38804, #10185 ) ;
#22963=CARTESIAN_POINT ( 'NONE',  ( -88.23625491228469286, -193.5000000000000000, 118.5089480183148254 ) ) ;
#22964=ORIENTED_EDGE ( 'NONE', *, *, #3234, .T. ) ;
#22966=CARTESIAN_POINT ( 'NONE',  ( -51.89154260666841623, -183.6283474603465606, 124.9534129907280970 ) ) ;
#22968=CARTESIAN_POINT ( 'NONE',  ( -172.9701362814535912, -175.3837268820161057, -11.26891947860193000 ) ) ;
#22969=ORIENTED_EDGE ( 'NONE', *, *, #5838, .T. ) ;
#22971=VERTEX_POINT ( 'NONE', #24064 ) ;
#22972=LINE ( 'NONE', #2994, #45097 ) ;
#22973=CARTESIAN_POINT ( 'NONE',  ( -164.0008810331606526, -193.5000000000000000, 47.74645837849825369 ) ) ;
#22975=DIRECTION ( 'NONE',  ( 0.000000000000000000, -1.000000000000000000, 0.000000000000000000 ) ) ;
#22976=DIRECTION ( 'NONE',  ( 0.000000000000000000, 1.000000000000000000, 0.000000000000000000 ) ) ;
#22977=AXIS2_PLACEMENT_3D ( 'NONE', #30427, #34878, #2055 ) ;
#22979=EDGE_CURVE ( 'NONE', #19952, #5285, #40079, .T. ) ;
#22980=EDGE_CURVE ( 'NONE', #2758, #23170, #39310, .T. ) ;
#22981=DIRECTION ( 'NONE',  ( 0.000000000000000000, -1.000000000000000000, 0.000000000000000000 ) ) ;
#22982=DIRECTION ( 'NONE',  ( 0.000000000000000000, 0.000000000000000000, -1.000000000000000000 ) ) ;
#22984=ORIENTED_EDGE ( 'NONE', *, *, #50593, .T. ) ;
#22985=ORIENTED_EDGE ( 'NONE', *, *, #30757, .F. ) ;
#22987=CARTESIAN_POINT ( 'NONE',  ( -48.47912675150883643, -193.5000000000000000, -125.0000000000000000 ) ) ;
#22991=CARTESIAN_POINT ( 'NONE',  ( -48.47912675150885065, -175.3837268820161057, 6.938893903907228378E-15 ) ) ;
#22992=ORIENTED_EDGE ( 'NONE', *, *, #42562, .T. ) ;
#22993=EDGE_CURVE ( 'NONE', #27852, #20294, #45087, .T. ) ;
#22995=AXIS2_PLACEMENT_3D ( 'NONE', #43830, #41446, #25684 ) ;
#22996=EDGE_CURVE ( 'NONE', #23360, #50065, #5393, .T. ) ;
#22997=EDGE_LOOP ( 'NONE', ( #27254, #8497, #49997, #44719 ) ) ;
#22998=DIRECTION ( 'NONE',  ( 0.000000000000000000, 0.000000000000000000, -1.000000000000000000 ) ) ;
#23002=PLANE ( 'NONE',  #48349 ) ;
#23005=CARTESIAN_POINT ( 'NONE',  ( -156.6671849566220089, -175.3837268820161057, 60.59166255800404599 ) ) ;
#23007=ORIENTED_EDGE ( 'NONE', *, *, #50236, .T. ) ;
#23008=DIRECTION ( 'NONE',  ( -0.000000000000000000, -1.000000000000000000, 0.000000000000000000 ) ) ;
#23010=ORIENTED_EDGE ( 'NONE', *, *, #36343, .F. ) ;
#23011=AXIS2_PLACEMENT_3D ( 'NONE', #49058, #41160, #29332 ) ;
#23012=CIRCLE ( 'NONE', #43150, 125.0000000000000000 ) ;
#23013=ORIENTED_EDGE ( 'NONE', *, *, #46798, .F. ) ;
#23014=CARTESIAN_POINT ( 'NONE',  ( -128.2395503755045638, -183.6283474603465606, -96.24590808611419845 ) ) ;
#23016=LINE ( 'NONE', #6992, #49514 ) ;
#23017=ORIENTED_EDGE ( 'NONE', *, *, #44106, .F. ) ;
#23018=CARTESIAN_POINT ( 'NONE',  ( 12.12533326292403935, -193.5000000000000000, 109.3256576763158847 ) ) ;
#23019=DIRECTION ( 'NONE',  ( 0.000000000000000000, 1.000000000000000000, -0.000000000000000000 ) ) ;
#23020=ORIENTED_EDGE ( 'NONE', *, *, #48165, .T. ) ;
#23021=DIRECTION ( 'NONE',  ( 0.000000000000000000, 1.000000000000000000, 0.000000000000000000 ) ) ;
#23024=CARTESIAN_POINT ( 'NONE',  ( -48.53836737940255119, -183.6283474603465606, -0.9982437317643153563 ) ) ;
#23026=EDGE_LOOP ( 'NONE', ( #28009, #10107, #12543, #27995 ) ) ;
#23027=VERTEX_POINT ( 'NONE', #13274 ) ;
#23028=LINE ( 'NONE', #50637, #46070 ) ;
#23029=DIRECTION ( 'NONE',  ( -0.000000000000000000, 1.000000000000000000, -0.000000000000000000 ) ) ;
#23030=DIRECTION ( 'NONE',  ( -0.8294056854502090959, 0.000000000000000000, 0.5586467658036415873 ) ) ;
#23031=CARTESIAN_POINT ( 'NONE',  ( -37.08895481556041318, -177.1207230881787780, 124.4799742258550310 ) ) ;
#23033=ORIENTED_EDGE ( 'NONE', *, *, #33529, .T. ) ;
#23036=ADVANCED_FACE ( 'NONE', ( #41122 ), #45854, .F. ) ;
#23040=CARTESIAN_POINT ( 'NONE',  ( -108.5723883981723930, -193.5000000000000000, 109.6074810615846360 ) ) ;
#23041=ORIENTED_EDGE ( 'NONE', *, *, #15887, .F. ) ;
#23042=ORIENTED_EDGE ( 'NONE', *, *, #9952, .F. ) ;
#23043=EDGE_CURVE ( 'NONE', #12949, #37838, #33384, .T. ) ;
#23044=CARTESIAN_POINT ( 'NONE',  ( 69.99104047056320610, -175.3837268820161057, -39.87254040532513955 ) ) ;
#23045=ADVANCED_FACE ( 'NONE', ( #37702 ), #37178, .T. ) ;
#23046=FACE_OUTER_BOUND ( 'NONE', #3248, .T. ) ;
#23048=VECTOR ( 'NONE', #28426, 1000.000000000000000 ) ;
#23049=CARTESIAN_POINT ( 'NONE',  ( -48.18706998087188254, -177.1207230881787780, 0.9564009842765313074 ) ) ;
#23050=DIRECTION ( 'NONE',  ( -0.000000000000000000, 1.000000000000000000, -0.000000000000000000 ) ) ;
#23051=VERTEX_POINT ( 'NONE', #36924 ) ;
#23052=EDGE_CURVE ( 'NONE', #28153, #10381, #39259, .T. ) ;
#23053=DIRECTION ( 'NONE',  ( 0.000000000000000000, 0.000000000000000000, -1.000000000000000000 ) ) ;
#23056=ADVANCED_FACE ( 'NONE', ( #21680 ), #25354, .T. ) ;
#23057=EDGE_CURVE ( 'NONE', #30483, #16943, #28757, .T. ) ;
#23058=VERTEX_POINT ( 'NONE', #29295 ) ;
#23060=FACE_OUTER_BOUND ( 'NONE', #44490, .T. ) ;
#23062=DIRECTION ( 'NONE',  ( -0.000000000000000000, 1.000000000000000000, -0.000000000000000000 ) ) ;
#23063=FACE_OUTER_BOUND ( 'NONE', #16528, .T. ) ;
#23064=ORIENTED_EDGE ( 'NONE', *, *, #15775, .F. ) ;
#23065=DIRECTION ( 'NONE',  ( -0.9266896074318343723, 0.000000000000000000, 0.3758275821142357809 ) ) ;
#23066=CARTESIAN_POINT ( 'NONE',  ( -28.74596282265200387, -177.1207230881787780, 123.4325817657431372 ) ) ;
#23067=EDGE_CURVE ( 'NONE', #26646, #27341, #24833, .T. ) ;
#23068=DIRECTION ( 'NONE',  ( -0.9374196611341206742, 0.000000000000000000, -0.3482016354343996367 ) ) ;
#23069=CARTESIAN_POINT ( 'NONE',  ( -48.47912675150885065, -183.6283474603465606, 6.938893903907228378E-15 ) ) ;
#23071=VECTOR ( 'NONE', #26663, 1000.000000000000000 ) ;
#23072=LINE ( 'NONE', #42518, #42280 ) ;
#23076=FACE_OUTER_BOUND ( 'NONE', #40163, .T. ) ;
#23078=EDGE_LOOP ( 'NONE', ( #22245, #238, #10137, #36465 ) ) ;
#23083=VECTOR ( 'NONE', #32557, 1000.000000000000000 ) ;
#23084=FACE_BOUND ( 'NONE', #16481, .T. ) ;
#23085=CARTESIAN_POINT ( 'NONE',  ( -147.6585554144535024, -193.5000000000000000, 76.08180419845385245 ) ) ;
#23086=AXIS2_PLACEMENT_3D ( 'NONE', #24398, #16258, #32270 ) ;
#23087=VECTOR ( 'NONE', #26996, 1000.000000000000000 ) ;
#23089=EDGE_LOOP ( 'NONE', ( #46563, #2016, #40497, #33254 ) ) ;
#23090=CIRCLE ( 'NONE', #38159, 125.0000000000000000 ) ;
#23092=EDGE_CURVE ( 'NONE', #47750, #3706, #30862, .T. ) ;
#23094=ORIENTED_EDGE ( 'NONE', *, *, #19190, .F. ) ;
#23096=CARTESIAN_POINT ( 'NONE',  ( 50.70030191143631271, -177.1207230881787780, -76.08180419845318454 ) ) ;
#23098=EDGE_CURVE ( 'NONE', #467, #1035, #50568, .T. ) ;
#23100=EDGE_CURVE ( 'NONE', #12871, #49461, #25872, .T. ) ;
#23101=AXIS2_PLACEMENT_3D ( 'NONE', #38357, #18400, #34417 ) ;
#23104=DIRECTION ( 'NONE',  ( 0.000000000000000000, -0.000000000000000000, 1.000000000000000000 ) ) ;
#23105=CARTESIAN_POINT ( 'NONE',  ( 32.99469856375238663, -175.3837268820161057, 94.79987230212020677 ) ) ;
#23106=ORIENTED_EDGE ( 'NONE', *, *, #33025, .F. ) ;
#23108=DIRECTION ( 'NONE',  ( -0.000000000000000000, 1.000000000000000000, -0.000000000000000000 ) ) ;
#23109=VERTEX_POINT ( 'NONE', #34007 ) ;
#23111=LINE ( 'NONE', #39887, #430 ) ;
#23113=DIRECTION ( 'NONE',  ( -0.000000000000000000, 1.000000000000000000, -0.000000000000000000 ) ) ;
#23114=ORIENTED_EDGE ( 'NONE', *, *, #11307, .F. ) ;
#23116=VERTEX_POINT ( 'NONE', #6687 ) ;
#23120=ORIENTED_EDGE ( 'NONE', *, *, #45039, .T. ) ;
#23121=LINE ( 'NONE', #15235, #21540 ) ;
#23123=DIRECTION ( 'NONE',  ( 0.000000000000000000, -1.000000000000000000, -0.000000000000000000 ) ) ;
#23125=CARTESIAN_POINT ( 'NONE',  ( -172.9701362814535912, -189.7472609257535510, -11.26891947860197440 ) ) ;
#23126=EDGE_CURVE ( 'NONE', #20990, #672, #50199, .T. ) ;
#23127=ORIENTED_EDGE ( 'NONE', *, *, #6983, .F. ) ;
#23128=LINE ( 'NONE', #14997, #28888 ) ;
#23129=DIRECTION ( 'NONE',  ( 0.000000000000000000, -1.000000000000000000, 0.000000000000000000 ) ) ;
#23131=AXIS2_PLACEMENT_3D ( 'NONE', #621, #43728, #7731 ) ;
#23133=VECTOR ( 'NONE', #22428, 1000.000000000000114 ) ;
#23135=ORIENTED_EDGE ( 'NONE', *, *, #23676, .F. ) ;
#23137=FACE_OUTER_BOUND ( 'NONE', #29158, .T. ) ;
#23138=CARTESIAN_POINT ( 'NONE',  ( 62.86098202833237281, -183.6283474603465606, 56.81883646197908888 ) ) ;
#23140=CARTESIAN_POINT ( 'NONE',  ( 47.04848625005566021, -183.6283474603465606, 80.61932246194658092 ) ) ;
#23143=CARTESIAN_POINT ( 'NONE',  ( -47.70260288879081401, -177.1207230881787780, 0.6300878435817218737 ) ) ;
#23145=AXIS2_PLACEMENT_3D ( 'NONE', #45896, #951, #13310 ) ;
#23147=DIRECTION ( 'NONE',  ( -0.000000000000000000, 1.000000000000000000, -0.000000000000000000 ) ) ;
#23148=LINE ( 'NONE', #34700, #2307 ) ;
#23150=VECTOR ( 'NONE', #34918, 1000.000000000000000 ) ;
#23151=EDGE_CURVE ( 'NONE', #9685, #7739, #26381, .T. ) ;
#23152=CIRCLE ( 'NONE', #30666, 125.0000000000000000 ) ;
#23153=DIRECTION ( 'NONE',  ( 0.9646355819083556327, 0.000000000000000000, 0.2635871660690782825 ) ) ;
#23154=DIRECTION ( 'NONE',  ( 0.000000000000000000, -0.000000000000000000, -1.000000000000000000 ) ) ;
#23155=CARTESIAN_POINT ( 'NONE',  ( -152.8876895714563773, -175.3837268820161057, 66.89437584437912676 ) ) ;
#23156=CYLINDRICAL_SURFACE ( 'NONE', #38793, 125.0000000000000000 ) ;
#23158=ORIENTED_EDGE ( 'NONE', *, *, #6961, .T. ) ;
#23163=VERTEX_POINT ( 'NONE', #46631 ) ;
#23164=DIRECTION ( 'NONE',  ( -0.000000000000000000, 1.000000000000000000, -0.000000000000000000 ) ) ;
#23165=VECTOR ( 'NONE', #51501, 1000.000000000000000 ) ;
#23166=AXIS2_PLACEMENT_3D ( 'NONE', #50537, #35264, #14537 ) ;
#23167=EDGE_CURVE ( 'NONE', #6669, #48376, #37953, .T. ) ;
#23170=VERTEX_POINT ( 'NONE', #14310 ) ;
#23172=DIRECTION ( 'NONE',  ( 0.000000000000000000, 0.000000000000000000, 1.000000000000000000 ) ) ;
#23173=PLANE ( 'NONE',  #33357 ) ;
#23176=VECTOR ( 'NONE', #30087, 1000.000000000000227 ) ;
#23177=AXIS2_PLACEMENT_3D ( 'NONE', #8771, #21385, #44789 ) ;
#23179=ORIENTED_EDGE ( 'NONE', *, *, #13500, .T. ) ;
#23180=CARTESIAN_POINT ( 'NONE',  ( 72.95485052494852596, -177.1207230881787780, -29.64437826672757836 ) ) ;
#23181=ORIENTED_EDGE ( 'NONE', *, *, #5649, .F. ) ;
#23182=DIRECTION ( 'NONE',  ( -0.9027978299657446470, 0.000000000000000000, 0.4300652022765183435 ) ) ;
#23183=AXIS2_PLACEMENT_3D ( 'NONE', #41956, #38541, #46180 ) ;
#23186=CARTESIAN_POINT ( 'NONE',  ( 61.69163308845453031, -183.6283474603465606, -56.90809649257491998 ) ) ;
#23187=ORIENTED_EDGE ( 'NONE', *, *, #39174, .F. ) ;
#23188=VECTOR ( 'NONE', #13354, 1000.000000000000114 ) ;
#23190=ORIENTED_EDGE ( 'NONE', *, *, #14612, .T. ) ;
#23191=DIRECTION ( 'NONE',  ( -0.000000000000000000, 1.000000000000000000, -0.000000000000000000 ) ) ;
#23192=DIRECTION ( 'NONE',  ( 0.000000000000000000, 0.000000000000000000, 1.000000000000000000 ) ) ;
#23196=CARTESIAN_POINT ( 'NONE',  ( -18.31235070009513421, -193.5000000000000000, 121.3052580173829966 ) ) ;
#23200=EDGE_CURVE ( 'NONE', #25116, #16167, #10357, .T. ) ;
#23202=DIRECTION ( 'NONE',  ( -0.5085311186492216251, 0.000000000000000000, 0.8610436117673548884 ) ) ;
#23206=CARTESIAN_POINT ( 'NONE',  ( -173.0563034899574859, -193.5000000000000000, -10.27263529369817618 ) ) ;
#23207=CARTESIAN_POINT ( 'NONE',  ( -73.94077438226446475, -183.6283474603465606, 122.3793467049372481 ) ) ;
#23208=ORIENTED_EDGE ( 'NONE', *, *, #17404, .F. ) ;
#23209=VECTOR ( 'NONE', #29201, 1000.000000000000000 ) ;
#23211=DIRECTION ( 'NONE',  ( 0.000000000000000000, 0.000000000000000000, 1.000000000000000000 ) ) ;
#23212=PLANE ( 'NONE',  #32456 ) ;
#23213=DIRECTION ( 'NONE',  ( 0.000000000000000000, 0.000000000000000000, 1.000000000000000000 ) ) ;
#23215=VECTOR ( 'NONE', #16705, 1000.000000000000227 ) ;
#23217=CARTESIAN_POINT ( 'NONE',  ( -134.2540868116286674, -193.5000000000000000, 89.54698061029657197 ) ) ;
#23219=ORIENTED_EDGE ( 'NONE', *, *, #36269, .F. ) ;
#23221=VECTOR ( 'NONE', #44266, 999.9999999999998863 ) ;
#23223=DIRECTION ( 'NONE',  ( -0.9960498426152158968, 0.000000000000000000, -0.08879589532294571153 ) ) ;
#23225=AXIS2_PLACEMENT_3D ( 'NONE', #51301, #7422, #39447 ) ;
#23226=CARTESIAN_POINT ( 'NONE',  ( -101.9736325116273576, -183.6283474603465606, 112.9749434763330527 ) ) ;
#23229=DIRECTION ( 'NONE',  ( -0.9960498426152177842, 0.000000000000000000, 0.08879589532292482545 ) ) ;
#23230=ORIENTED_EDGE ( 'NONE', *, *, #26113, .T. ) ;
#23231=LINE ( 'NONE', #36074, #46853 ) ;
#23234=LINE ( 'NONE', #19527, #10988 ) ;
#23235=LINE ( 'NONE', #19295, #32479 ) ;
#23237=EDGE_LOOP ( 'NONE', ( #31422, #45016, #22598, #28283 ) ) ;
#23238=ORIENTED_EDGE ( 'NONE', *, *, #47832, .F. ) ;
#23240=LINE ( 'NONE', #51879, #47861 ) ;
#23242=PLANE ( 'NONE',  #29082 ) ;
#23243=VECTOR ( 'NONE', #30830, 1000.000000000000000 ) ;
#23244=CARTESIAN_POINT ( 'NONE',  ( -168.9345475356665531, -177.1207230881787780, 29.43839964798725362 ) ) ;
#23247=VECTOR ( 'NONE', #22448, 999.9999999999998863 ) ;
#23248=ADVANCED_FACE ( 'NONE', ( #14837 ), #46897, .T. ) ;
#23249=CARTESIAN_POINT ( 'NONE',  ( -122.3978016498073202, -177.1207230881787780, -100.8019320314827212 ) ) ;
#23250=DIRECTION ( 'NONE',  ( 0.000000000000000000, -1.000000000000000000, 0.000000000000000000 ) ) ;
#23252=EDGE_LOOP ( 'NONE', ( #42732, #5012, #15117, #13602 ) ) ;
#23253=VECTOR ( 'NONE', #9086, 1000.000000000000114 ) ;
#23254=FACE_OUTER_BOUND ( 'NONE', #10465, .T. ) ;
#23256=AXIS2_PLACEMENT_3D ( 'NONE', #7368, #19187, #14221 ) ;
#23257=VERTEX_POINT ( 'NONE', #38972 ) ;
#23261=AXIS2_PLACEMENT_3D ( 'NONE', #27121, #19754, #3469 ) ;
#23263=FACE_OUTER_BOUND ( 'NONE', #16675, .T. ) ;
#23265=FACE_OUTER_BOUND ( 'NONE', #40295, .T. ) ;
#23266=VECTOR ( 'NONE', #35552, 1000.000000000000000 ) ;
#23269=FACE_OUTER_BOUND ( 'NONE', #2132, .T. ) ;
#23270=FACE_OUTER_BOUND ( 'NONE', #18151, .T. ) ;
#23271=ORIENTED_EDGE ( 'NONE', *, *, #21553, .T. ) ;
#23272=CARTESIAN_POINT ( 'NONE',  ( -169.0855799822425922, -193.5000000000000000, -28.81338593823970839 ) ) ;
#23273=CARTESIAN_POINT ( 'NONE',  ( -48.47912675150885065, -193.5000000000000000, 6.938893903907228378E-15 ) ) ;
#23274=LINE ( 'NONE', #31393, #14792 ) ;
#23275=LINE ( 'NONE', #31917, #16524 ) ;
#23281=CARTESIAN_POINT ( 'NONE',  ( 72.82672500347334221, -193.5000000000000000, 25.70779184431858155 ) ) ;
#23283=VERTEX_POINT ( 'NONE', #47667 ) ;
#23287=EDGE_CURVE ( 'NONE', #3372, #41076, #27410, .T. ) ;
#23288=CARTESIAN_POINT ( 'NONE',  ( -40.96347969518280507, -193.5000000000000000, -123.7720294769268889 ) ) ;
#23290=VERTEX_POINT ( 'NONE', #11122 ) ;
#23291=LINE ( 'NONE', #7252, #1255 ) ;
#23292=CIRCLE ( 'NONE', #21607, 125.0000000000000000 ) ;
#23294=ORIENTED_EDGE ( 'NONE', *, *, #40633, .T. ) ;
#23295=PLANE ( 'NONE',  #15757 ) ;
#23296=CIRCLE ( 'NONE', #628, 125.0000000000000000 ) ;
#23297=EDGE_CURVE ( 'NONE', #32383, #50178, #15339, .T. ) ;
#23298=AXIS2_PLACEMENT_3D ( 'NONE', #41811, #13690, #37611 ) ;
#23300=DIRECTION ( 'NONE',  ( -0.000000000000000000, 1.000000000000000000, -0.000000000000000000 ) ) ;
#23302=ORIENTED_EDGE ( 'NONE', *, *, #27187, .F. ) ;
#23303=EDGE_CURVE ( 'NONE', #9591, #28684, #26696, .T. ) ;
#23305=VECTOR ( 'NONE', #14517, 1000.000000000000000 ) ;
#23306=LINE ( 'NONE', #51174, #9980 ) ;
#23308=ADVANCED_FACE ( 'NONE', ( #39735 ), #23484, .T. ) ;
#23309=DIRECTION ( 'NONE',  ( 0.000000000000000000, 1.000000000000000000, 0.000000000000000000 ) ) ;
#23310=DIRECTION ( 'NONE',  ( -0.9646355819083594074, 0.000000000000000000, 0.2635871660690647933 ) ) ;
#23311=CARTESIAN_POINT ( 'NONE',  ( 73.66680038934278230, -189.7472609257535510, -26.55884942729568721 ) ) ;
#23312=EDGE_LOOP ( 'NONE', ( #42769, #36671, #11972, #223 ) ) ;
#23313=FACE_OUTER_BOUND ( 'NONE', #40274, .T. ) ;
#23316=DIRECTION ( 'NONE',  ( 0.4566292373937140270, 0.000000000000000000, -0.8896570909947467687 ) ) ;
#23318=VECTOR ( 'NONE', #1720, 1000.000000000000000 ) ;
#23319=ORIENTED_EDGE ( 'NONE', *, *, #50424, .F. ) ;
#23321=LINE ( 'NONE', #18837, #44237 ) ;
#23322=EDGE_CURVE ( 'NONE', #17812, #28521, #1524, .T. ) ;
#23323=CARTESIAN_POINT ( 'NONE',  ( 52.59568867645218404, -189.7472609257535510, -73.54509967498589162 ) ) ;
#23326=DIRECTION ( 'NONE',  ( -0.000000000000000000, 1.000000000000000000, -0.000000000000000000 ) ) ;
#23327=VERTEX_POINT ( 'NONE', #11649 ) ;
#23328=DIRECTION ( 'NONE',  ( -0.000000000000000000, 1.000000000000000000, -0.000000000000000000 ) ) ;
#23329=VERTEX_POINT ( 'NONE', #43181 ) ;
#23330=EDGE_LOOP ( 'NONE', ( #2957, #30384, #10622, #14427 ) ) ;
#23332=AXIS2_PLACEMENT_3D ( 'NONE', #8534, #3829, #31935 ) ;
#23333=CARTESIAN_POINT ( 'NONE',  ( -173.0003472773501301, -193.5000000000000000, 10.93003379476953363 ) ) ;
#23335=CARTESIAN_POINT ( 'NONE',  ( -124.4642912599203726, -175.3837268820161057, 99.25348746834863789 ) ) ;
#23336=DIRECTION ( 'NONE',  ( 0.2920567706369764371, 0.000000000000000000, -0.9564009842765223146 ) ) ;
#23339=LINE ( 'NONE', #51455, #12912 ) ;
#23340=CARTESIAN_POINT ( 'NONE',  ( 17.15229921100055321, -183.6283474603465606, -106.3838142112212779 ) ) ;
#23341=VECTOR ( 'NONE', #15484, 1000.000000000000000 ) ;
#23342=DIRECTION ( 'NONE',  ( 0.000000000000000000, 0.000000000000000000, 1.000000000000000000 ) ) ;
#23343=ORIENTED_EDGE ( 'NONE', *, *, #14094, .F. ) ;
#23344=DIRECTION ( 'NONE',  ( -0.000000000000000000, 1.000000000000000000, -0.000000000000000000 ) ) ;
#23345=EDGE_CURVE ( 'NONE', #16540, #50918, #12874, .T. ) ;
#23346=ORIENTED_EDGE ( 'NONE', *, *, #33016, .F. ) ;
#23348=DIRECTION ( 'NONE',  ( -0.6965510290630033685, 0.000000000000000000, 0.7175072570443249420 ) ) ;
#23350=CIRCLE ( 'NONE', #9920, 125.0000000000000000 ) ;
#23351=PLANE ( 'NONE',  #51133 ) ;
#23352=CIRCLE ( 'NONE', #48535, 125.0000000000000000 ) ;
#23353=FACE_BOUND ( 'NONE', #18550, .T. ) ;
#23354=DIRECTION ( 'NONE',  ( 0.000000000000000000, 0.000000000000000000, 1.000000000000000000 ) ) ;
#23355=CIRCLE ( 'NONE', #30066, 125.0000000000000000 ) ;
#23357=CARTESIAN_POINT ( 'NONE',  ( -53.47502265695602119, -193.5000000000000000, -123.9001241957025883 ) ) ;
#23359=EDGE_CURVE ( 'NONE', #21393, #11641, #23362, .T. ) ;
#23360=VERTEX_POINT ( 'NONE', #8941 ) ;
#23361=DIRECTION ( 'NONE',  ( 0.000000000000000000, 1.000000000000000000, 0.000000000000000000 ) ) ;
#23362=CIRCLE ( 'NONE', #14968, 125.0000000000000000 ) ;
#23363=EDGE_CURVE ( 'NONE', #8278, #14662, #5744, .T. ) ;
#23364=EDGE_LOOP ( 'NONE', ( #23475, #8146, #6196, #33935 ) ) ;
#23366=EDGE_CURVE ( 'NONE', #9485, #3068, #23231, .T. ) ;
#23367=AXIS2_PLACEMENT_3D ( 'NONE', #50214, #46781, #17638 ) ;
#23371=LINE ( 'NONE', #47027, #15525 ) ;
#23372=VERTEX_POINT ( 'NONE', #7705 ) ;
#23374=ORIENTED_EDGE ( 'NONE', *, *, #28548, .F. ) ;
#23375=CARTESIAN_POINT ( 'NONE',  ( -171.9838957966129840, -175.3837268820161057, 19.27620354518724355 ) ) ;
#23376=VERTEX_POINT ( 'NONE', #71 ) ;
#23378=ORIENTED_EDGE ( 'NONE', *, *, #7066, .T. ) ;
#23380=CARTESIAN_POINT ( 'NONE',  ( -48.47912675150885065, -189.7472609257535510, 6.938893903907228378E-15 ) ) ;
#23382=LINE ( 'NONE', #19425, #10611 ) ;
#23385=DIRECTION ( 'NONE',  ( -0.000000000000000000, 1.000000000000000000, 0.000000000000000000 ) ) ;
#23390=DIRECTION ( 'NONE',  ( -0.000000000000000000, 1.000000000000000000, -0.000000000000000000 ) ) ;
#23391=PLANE ( 'NONE',  #38152 ) ;
#23392=VERTEX_POINT ( 'NONE', #24979 ) ;
#23394=DIRECTION ( 'NONE',  ( -0.000000000000000000, 1.000000000000000000, -0.000000000000000000 ) ) ;
#23396=ADVANCED_FACE ( 'NONE', ( #40993 ), #19522, .T. ) ;
#23397=DIRECTION ( 'NONE',  ( -0.000000000000000000, 1.000000000000000000, -0.000000000000000000 ) ) ;
#23398=VERTEX_POINT ( 'NONE', #51593 ) ;
#23399=VECTOR ( 'NONE', #27215, 1000.000000000000000 ) ;
#23400=PLANE ( 'NONE',  #37448 ) ;
#23401=DIRECTION ( 'NONE',  ( 0.000000000000000000, -0.000000000000000000, -1.000000000000000000 ) ) ;
#23402=EDGE_CURVE ( 'NONE', #33538, #45739, #31614, .T. ) ;
#23403=CYLINDRICAL_SURFACE ( 'NONE', #19385, 124.9999999999999858 ) ;
#23404=CARTESIAN_POINT ( 'NONE',  ( 74.13662511985246795, -175.3837268820161057, 18.47640724094593168 ) ) ;
#23407=ADVANCED_FACE ( 'NONE', ( #5270 ), #13142, .T. ) ;
#23408=ORIENTED_EDGE ( 'NONE', *, *, #14324, .F. ) ;
#23409=ORIENTED_EDGE ( 'NONE', *, *, #28211, .F. ) ;
#23410=EDGE_CURVE ( 'NONE', #48020, #38286, #12426, .T. ) ;
#23412=ADVANCED_FACE ( 'NONE', ( #9460 ), #33629, .T. ) ;
#23413=CARTESIAN_POINT ( 'NONE',  ( 72.05536924052414349, -193.5000000000000000, 33.11246405730899056 ) ) ;
#23415=DIRECTION ( 'NONE',  ( 0.000000000000000000, 1.000000000000000000, 0.000000000000000000 ) ) ;
#23417=EDGE_CURVE ( 'NONE', #787, #32651, #47716, .T. ) ;
#23420=ORIENTED_EDGE ( 'NONE', *, *, #16533, .T. ) ;
#23421=ORIENTED_EDGE ( 'NONE', *, *, #39424, .T. ) ;
#23423=VECTOR ( 'NONE', #34138, 1000.000000000000000 ) ;
#23424=ORIENTED_EDGE ( 'NONE', *, *, #41368, .T. ) ;
#23425=DIRECTION ( 'NONE',  ( 0.000000000000000000, 0.000000000000000000, -1.000000000000000000 ) ) ;
#23427=EDGE_CURVE ( 'NONE', #18925, #11600, #49426, .T. ) ;
#23430=ADVANCED_FACE ( 'NONE', ( #29941 ), #26001, .T. ) ;
#23431=CARTESIAN_POINT ( 'NONE',  ( -48.47912675150885065, -183.6283474603465606, 6.938893903907228378E-15 ) ) ;
#23436=ORIENTED_EDGE ( 'NONE', *, *, #1460, .T. ) ;
#23438=VERTEX_POINT ( 'NONE', #1825 ) ;
#23441=CARTESIAN_POINT ( 'NONE',  ( 20.66186849114819069, -189.7472609257535510, -104.1370384486464928 ) ) ;
#23442=DIRECTION ( 'NONE',  ( -0.5586467658036415873, 0.000000000000000000, -0.8294056854502090959 ) ) ;
#23444=FACE_OUTER_BOUND ( 'NONE', #16017, .T. ) ;
#23445=ADVANCED_FACE ( 'NONE', ( #41782 ), #5533, .T. ) ;
#23446=EDGE_LOOP ( 'NONE', ( #26356, #19714, #24759, #16834 ) ) ;
#23450=DIRECTION ( 'NONE',  ( -0.000000000000000000, 1.000000000000000000, -0.000000000000000000 ) ) ;
#23451=VERTEX_POINT ( 'NONE', #21812 ) ;
#23453=DIRECTION ( 'NONE',  ( -0.000000000000000000, 1.000000000000000000, -0.000000000000000000 ) ) ;
#23454=ORIENTED_EDGE ( 'NONE', *, *, #41047, .T. ) ;
#23456=PLANE ( 'NONE',  #2138 ) ;
#23457=ORIENTED_EDGE ( 'NONE', *, *, #31260, .T. ) ;
#23458=CARTESIAN_POINT ( 'NONE',  ( -91.84482189527193441, -175.3837268820161057, -117.2365833888816695 ) ) ;
#23460=VECTOR ( 'NONE', #49342, 1000.000000000000227 ) ;
#23461=DIRECTION ( 'NONE',  ( -0.6068001458186002006, 0.000000000000000000, 0.7948544414133481562 ) ) ;
#23462=CARTESIAN_POINT ( 'NONE',  ( -40.90423906728908321, -193.5000000000000000, -124.7702732086912221 ) ) ;
#23463=VECTOR ( 'NONE', #32073, 1000.000000000000000 ) ;
#23464=EDGE_CURVE ( 'NONE', #24906, #41605, #45726, .T. ) ;
#23466=CARTESIAN_POINT ( 'NONE',  ( -151.5051191635538146, -183.6283474603465606, -69.00559874123518966 ) ) ;
#23467=LINE ( 'NONE', #15080, #23243 ) ;
#23468=EDGE_CURVE ( 'NONE', #3230, #48106, #17864, .T. ) ;
#23470=LINE ( 'NONE', #15319, #12863 ) ;
#23471=ADVANCED_FACE ( 'NONE', ( #33107 ), #30209, .T. ) ;
#23472=DIRECTION ( 'NONE',  ( -0.9995608365087944591, 0.000000000000000000, 0.02963332782255633305 ) ) ;
#23473=DIRECTION ( 'NONE',  ( -0.000000000000000000, 1.000000000000000000, -0.000000000000000000 ) ) ;
#23475=ORIENTED_EDGE ( 'NONE', *, *, #2209, .F. ) ;
#23477=LINE ( 'NONE', #43450, #28291 ) ;
#23478=VECTOR ( 'NONE', #21746, 999.9999999999998863 ) ;
#23479=CARTESIAN_POINT ( 'NONE',  ( 8.448131207122532516, -193.5000000000000000, 111.2847127925100352 ) ) ;
#23480=ORIENTED_EDGE ( 'NONE', *, *, #28276, .F. ) ;
#23482=FACE_OUTER_BOUND ( 'NONE', #17083, .T. ) ;
#23483=EDGE_LOOP ( 'NONE', ( #36228, #11293, #4462, #38281 ) ) ;
#23484=CYLINDRICAL_SURFACE ( 'NONE', #21676, 125.0000000000000000 ) ;
#23486=CARTESIAN_POINT ( 'NONE',  ( 13.86276369408137477, -189.7472609257535510, -107.1890582354654526 ) ) ;
#23488=ORIENTED_EDGE ( 'NONE', *, *, #18487, .T. ) ;
#23489=VERTEX_POINT ( 'NONE', #46250 ) ;
#23491=EDGE_LOOP ( 'NONE', ( #3205, #23703, #23436, #24760 ) ) ;
#23492=DIRECTION ( 'NONE',  ( -0.7765238627180482966, 0.000000000000000000, 0.6300878435817038881 ) ) ;
#23493=DIRECTION ( 'NONE',  ( 0.000000000000000000, -0.000000000000000000, -1.000000000000000000 ) ) ;
#23494=CARTESIAN_POINT ( 'NONE',  ( -148.0127667507368585, -193.5000000000000000, -75.61781872352626976 ) ) ;
#23497=LINE ( 'NONE', #32144, #44906 ) ;
#23499=CARTESIAN_POINT ( 'NONE',  ( 58.95724912996274725, -177.1207230881787780, 61.91627321685103169 ) ) ;
#23500=CARTESIAN_POINT ( 'NONE',  ( 33.75048693540709621, -175.3837268820161057, 94.14505102712816154 ) ) ;
#23501=VERTEX_POINT ( 'NONE', #51224 ) ;
#23502=ORIENTED_EDGE ( 'NONE', *, *, #311, .T. ) ;
#23505=CARTESIAN_POINT ( 'NONE',  ( -138.3705904895685421, -183.6283474603465606, -86.85922373029301014 ) ) ;
#23506=EDGE_LOOP ( 'NONE', ( #709, #15444, #91, #28185 ) ) ;
#23509=DIRECTION ( 'NONE',  ( 0.000000000000000000, 0.000000000000000000, -1.000000000000000000 ) ) ;
#23510=ORIENTED_EDGE ( 'NONE', *, *, #11587, .F. ) ;
#23511=LINE ( 'NONE', #34304, #41840 ) ;
#23512=CIRCLE ( 'NONE', #41959, 125.0000000000000000 ) ;
#23515=DIRECTION ( 'NONE',  ( -0.000000000000000000, 1.000000000000000000, -0.000000000000000000 ) ) ;
#23516=FACE_OUTER_BOUND ( 'NONE', #45433, .T. ) ;
#23517=VERTEX_POINT ( 'NONE', #34652 ) ;
#23518=DIRECTION ( 'NONE',  ( 0.3758275821142422202, 0.000000000000000000, -0.9266896074318318188 ) ) ;
#23519=LINE ( 'NONE', #27970, #46550 ) ;
#23520=LINE ( 'NONE', #15383, #30707 ) ;
#23521=ADVANCED_FACE ( 'NONE', ( #26774 ), #50698, .T. ) ;
#23522=DIRECTION ( 'NONE',  ( -0.6068001458186002006, 0.000000000000000000, 0.7948544414133481562 ) ) ;
#23525=ORIENTED_EDGE ( 'NONE', *, *, #23092, .T. ) ;
#23526=AXIS2_PLACEMENT_3D ( 'NONE', #10992, #7576, #23596 ) ;
#23528=DIRECTION ( 'NONE',  ( 0.6528221181905174975, 0.000000000000000000, 0.7575112421616236880 ) ) ;
#23531=CARTESIAN_POINT ( 'NONE',  ( -26.53529504715430676, -175.3837268820161057, 123.0587999703026867 ) ) ;
#23532=DIRECTION ( 'NONE',  ( 0.000000000000000000, 0.000000000000000000, -1.000000000000000000 ) ) ;
#23533=EDGE_LOOP ( 'NONE', ( #6964, #23010, #2826, #41303 ) ) ;
#23537=ORIENTED_EDGE ( 'NONE', *, *, #32654, .F. ) ;
#23538=LINE ( 'NONE', #32195, #17450 ) ;
#23540=DIRECTION ( 'NONE',  ( -0.9027978299657477557, 0.000000000000000000, 0.4300652022765115712 ) ) ;
#23541=CARTESIAN_POINT ( 'NONE',  ( -85.77912150413021664, -175.3837268820161057, -119.3051146910911768 ) ) ;
#23546=ORIENTED_EDGE ( 'NONE', *, *, #18905, .T. ) ;
#23547=DIRECTION ( 'NONE',  ( 0.000000000000000000, -1.000000000000000000, -0.000000000000000000 ) ) ;
#23549=FACE_OUTER_BOUND ( 'NONE', #33192, .T. ) ;
#23552=EDGE_LOOP ( 'NONE', ( #1362, #30044, #30307, #33053 ) ) ;
#23554=CARTESIAN_POINT ( 'NONE',  ( -170.7635349987907034, -189.7472609257535510, -25.91377046305883169 ) ) ;
#23556=FACE_OUTER_BOUND ( 'NONE', #20904, .T. ) ;
#23557=ORIENTED_EDGE ( 'NONE', *, *, #23812, .F. ) ;
#23558=VERTEX_POINT ( 'NONE', #43062 ) ;
#23560=EDGE_CURVE ( 'NONE', #47778, #27224, #26510, .T. ) ;
#23561=DIRECTION ( 'NONE',  ( -0.2059786187410953262, 0.000000000000000000, -0.9785564922995046988 ) ) ;
#23563=DIRECTION ( 'NONE',  ( -0.000000000000000000, 1.000000000000000000, -0.000000000000000000 ) ) ;
#23566=DIRECTION ( 'NONE',  ( 0.000000000000000000, 0.000000000000000000, -1.000000000000000000 ) ) ;
#23567=ORIENTED_EDGE ( 'NONE', *, *, #26227, .F. ) ;
#23568=ADVANCED_FACE ( 'NONE', ( #30973 ), #27548, .F. ) ;
#23570=CARTESIAN_POINT ( 'NONE',  ( -91.22542124915045747, -193.5000000000000000, 117.4638425504669783 ) ) ;
#23574=DIRECTION ( 'NONE',  ( 0.000000000000000000, 0.000000000000000000, 1.000000000000000000 ) ) ;
#23577=ORIENTED_EDGE ( 'NONE', *, *, #14163, .F. ) ;
#23581=AXIS2_PLACEMENT_3D ( 'NONE', #50435, #1804, #17847 ) ;
#23582=CARTESIAN_POINT ( 'NONE',  ( -166.6807411098556031, -177.1207230881787780, 37.47770156625504256 ) ) ;
#23583=ORIENTED_EDGE ( 'NONE', *, *, #49530, .F. ) ;
#23584=EDGE_CURVE ( 'NONE', #23845, #38723, #3216, .T. ) ;
#23585=DIRECTION ( 'NONE',  ( 0.9785564922995032555, 0.000000000000000000, 0.2059786187411021818 ) ) ;
#23586=CARTESIAN_POINT ( 'NONE',  ( -95.72791768350688812, -193.5000000000000000, -115.7261930397105232 ) ) ;
#23587=EDGE_LOOP ( 'NONE', ( #49536, #11693, #16139, #19416 ) ) ;
#23590=DIRECTION ( 'NONE',  ( -0.000000000000000000, 1.000000000000000000, -0.000000000000000000 ) ) ;
#23592=FACE_BOUND ( 'NONE', #17563, .T. ) ;
#23594=ORIENTED_EDGE ( 'NONE', *, *, #36455, .T. ) ;
#23595=EDGE_CURVE ( 'NONE', #13008, #47040, #47017, .T. ) ;
#23596=DIRECTION ( 'NONE',  ( 0.000000000000000000, 0.000000000000000000, 1.000000000000000000 ) ) ;
#23597=EDGE_CURVE ( 'NONE', #33930, #46522, #32579, .T. ) ;
#23599=ORIENTED_EDGE ( 'NONE', *, *, #23410, .T. ) ;
#23600=CARTESIAN_POINT ( 'NONE',  ( -47.63353074800703268, -189.7472609257535510, 0.5338233779648018373 ) ) ;
#23602=CARTESIAN_POINT ( 'NONE',  ( -48.02249751411514467, -177.1207230881787780, 0.8896570909947569827 ) ) ;
#23603=AXIS2_PLACEMENT_3D ( 'NONE', #34321, #44277, #51922 ) ;
#23604=CARTESIAN_POINT ( 'NONE',  ( 64.01121016852529522, -175.3837268820161057, -54.50618404930953176 ) ) ;
#23605=DIRECTION ( 'NONE',  ( -0.000000000000000000, 1.000000000000000000, -0.000000000000000000 ) ) ;
#23607=DIRECTION ( 'NONE',  ( 0.8124868780056783146, 0.000000000000000000, 0.5829794791144762289 ) ) ;
#23608=VERTEX_POINT ( 'NONE', #10995 ) ;
#23610=DIRECTION ( 'NONE',  ( -0.2059786187410953262, 0.000000000000000000, -0.9785564922995046988 ) ) ;
#23611=ORIENTED_EDGE ( 'NONE', *, *, #10235, .F. ) ;
#23612=PLANE ( 'NONE',  #31476 ) ;
#23616=CYLINDRICAL_SURFACE ( 'NONE', #31764, 125.0000000000000000 ) ;
#23617=EDGE_LOOP ( 'NONE', ( #14269, #35984, #43533, #17603 ) ) ;
#23618=CARTESIAN_POINT ( 'NONE',  ( 29.90148147319962035, -193.5000000000000000, 96.08646119224012239 ) ) ;
#23620=ORIENTED_EDGE ( 'NONE', *, *, #19214, .F. ) ;
#23621=AXIS2_PLACEMENT_3D ( 'NONE', #1805, #29926, #9975 ) ;
#23623=ORIENTED_EDGE ( 'NONE', *, *, #17666, .F. ) ;
#23624=CARTESIAN_POINT ( 'NONE',  ( -124.3803110981236273, -175.3837268820161057, -98.05618656931940791 ) ) ;
#23627=DIRECTION ( 'NONE',  ( 0.7765238627180482966, 0.000000000000000000, -0.6300878435817038881 ) ) ;
#23628=LINE ( 'NONE', #34434, #51731 ) ;
#23629=DIRECTION ( 'NONE',  ( 0.000000000000000000, 1.000000000000000000, 0.000000000000000000 ) ) ;
#23631=ORIENTED_EDGE ( 'NONE', *, *, #29692, .T. ) ;
#23634=DIRECTION ( 'NONE',  ( 0.1476465640024710868, 0.000000000000000000, 0.9890401873221654760 ) ) ;
#23635=CARTESIAN_POINT ( 'NONE',  ( -48.24424070572787571, -193.5000000000000000, 0.9720229140804191870 ) ) ;
#23636=EDGE_CURVE ( 'NONE', #25951, #38237, #15212, .T. ) ;
#23637=CARTESIAN_POINT ( 'NONE',  ( -49.40581635894069024, -175.3837268820161057, 0.3758275821142362250 ) ) ;
#23639=EDGE_CURVE ( 'NONE', #32593, #2592, #50451, .T. ) ;
#23642=EDGE_CURVE ( 'NONE', #34175, #8967, #4913, .T. ) ;
#23643=CARTESIAN_POINT ( 'NONE',  ( 30.50828161901820224, -177.1207230881787780, 96.88131563365348597 ) ) ;
#23644=DIRECTION ( 'NONE',  ( 0.000000000000000000, 0.000000000000000000, 1.000000000000000000 ) ) ;
#23645=EDGE_LOOP ( 'NONE', ( #37978, #34907, #40318, #36223 ) ) ;
#23646=VERTEX_POINT ( 'NONE', #31998 ) ;
#23647=VECTOR ( 'NONE', #48008, 1000.000000000000000 ) ;
#23648=ORIENTED_EDGE ( 'NONE', *, *, #48139, .F. ) ;
#23649=AXIS2_PLACEMENT_3D ( 'NONE', #31279, #27602, #11299 ) ;
#23651=DIRECTION ( 'NONE',  ( -0.4566292373937077542, 0.000000000000000000, -0.8896570909947499883 ) ) ;
#23652=CARTESIAN_POINT ( 'NONE',  ( -49.30901192927175458, -175.3837268820161057, -124.9972451320097093 ) ) ;
#23654=ORIENTED_EDGE ( 'NONE', *, *, #31519, .F. ) ;
#23657=ORIENTED_EDGE ( 'NONE', *, *, #34498, .F. ) ;
#23659=ORIENTED_EDGE ( 'NONE', *, *, #24362, .T. ) ;
#23661=ORIENTED_EDGE ( 'NONE', *, *, #17963, .F. ) ;
#23665=DIRECTION ( 'NONE',  ( 0.2920567706369694982, 0.000000000000000000, 0.9564009842765243130 ) ) ;
#23666=DIRECTION ( 'NONE',  ( -0.000000000000000000, 1.000000000000000000, -0.000000000000000000 ) ) ;
#23667=LINE ( 'NONE', #31042, #14896 ) ;
#23669=EDGE_CURVE ( 'NONE', #18052, #34792, #49410, .T. ) ;
#23670=CARTESIAN_POINT ( 'NONE',  ( -38.66762320617017679, -193.5000000000000000, -124.6143426664033740 ) ) ;
#23671=ORIENTED_EDGE ( 'NONE', *, *, #51586, .F. ) ;
#23672=FACE_OUTER_BOUND ( 'NONE', #46120, .T. ) ;
#23673=AXIS2_PLACEMENT_3D ( 'NONE', #39899, #24167, #36480 ) ;
#23674=ORIENTED_EDGE ( 'NONE', *, *, #42679, .T. ) ;
#23676=EDGE_CURVE ( 'NONE', #32651, #46212, #19924, .T. ) ;
#23677=EDGE_CURVE ( 'NONE', #41991, #43010, #24910, .T. ) ;
#23679=DIRECTION ( 'NONE',  ( 0.000000000000000000, 0.000000000000000000, 1.000000000000000000 ) ) ;
#23680=CARTESIAN_POINT ( 'NONE',  ( -170.7635349987907603, -175.3837268820161057, -25.91377046305877130 ) ) ;
#23681=LINE ( 'NONE', #43663, #13070 ) ;
#23682=VERTEX_POINT ( 'NONE', #48041 ) ;
#23686=CARTESIAN_POINT ( 'NONE',  ( -172.5669052183642407, -177.1207230881787780, 15.07392567185553744 ) ) ;
#23688=ORIENTED_EDGE ( 'NONE', *, *, #20786, .T. ) ;
#23689=EDGE_CURVE ( 'NONE', #34695, #48626, #42673, .T. ) ;
#23692=EDGE_CURVE ( 'NONE', #21919, #38136, #12021, .T. ) ;
#23693=CARTESIAN_POINT ( 'NONE',  ( 73.80528149577284580, -189.7472609257535510, 25.91377046305970211 ) ) ;
#23694=VERTEX_POINT ( 'NONE', #35957 ) ;
#23695=DIRECTION ( 'NONE',  ( 0.000000000000000000, 0.000000000000000000, 1.000000000000000000 ) ) ;
#23696=EDGE_CURVE ( 'NONE', #1758, #2274, #39871, .T. ) ;
#23697=VECTOR ( 'NONE', #51276, 999.9999999999998863 ) ;
#23698=DIRECTION ( 'NONE',  ( 0.000000000000000000, -1.000000000000000000, 0.000000000000000000 ) ) ;
#23699=AXIS2_PLACEMENT_3D ( 'NONE', #9040, #16678, #20077 ) ;
#23703=ORIENTED_EDGE ( 'NONE', *, *, #13331, .F. ) ;
#23706=EDGE_CURVE ( 'NONE', #5333, #42630, #44370, .T. ) ;
#23708=DIRECTION ( 'NONE',  ( 0.000000000000000000, -1.000000000000000000, 0.000000000000000000 ) ) ;
#23711=LINE ( 'NONE', #19760, #7958 ) ;
#23712=CARTESIAN_POINT ( 'NONE',  ( 45.36094686508022988, -183.6283474603465606, -82.57748230379236531 ) ) ;
#23713=EDGE_CURVE ( 'NONE', #46918, #48966, #15991, .T. ) ;
#23714=CARTESIAN_POINT ( 'NONE',  ( -50.89116676070551648, -193.5000000000000000, 124.9767260852757147 ) ) ;
#23715=DIRECTION ( 'NONE',  ( -0.000000000000000000, 1.000000000000000000, -0.000000000000000000 ) ) ;
#23716=CARTESIAN_POINT ( 'NONE',  ( -127.0132498732366457, -183.6283474603465606, 97.24912084693259828 ) ) ;
#23717=CARTESIAN_POINT ( 'NONE',  ( -48.98765787015808115, -193.5000000000000000, 0.8610436117673582190 ) ) ;
#23720=EDGE_LOOP ( 'NONE', ( #2041, #1654, #29418, #46674 ) ) ;
#23722=ADVANCED_FACE ( 'NONE', ( #8098 ), #8360, .T. ) ;
#23723=VECTOR ( 'NONE', #16295, 1000.000000000000000 ) ;
#23724=FACE_OUTER_BOUND ( 'NONE', #23078, .T. ) ;
#23725=ORIENTED_EDGE ( 'NONE', *, *, #15648, .T. ) ;
#23726=VERTEX_POINT ( 'NONE', #40648 ) ;
#23728=EDGE_LOOP ( 'NONE', ( #36581, #51443, #4250, #20720 ) ) ;
#23729=DIRECTION ( 'NONE',  ( -0.000000000000000000, 1.000000000000000000, 0.000000000000000000 ) ) ;
#23731=CARTESIAN_POINT ( 'NONE',  ( -111.8989814360438828, -175.3837268820161057, -107.7168604805787027 ) ) ;
#23732=CARTESIAN_POINT ( 'NONE',  ( -124.4642912599203726, -193.5000000000000000, 99.25348746834863789 ) ) ;
#23734=VERTEX_POINT ( 'NONE', #4410 ) ;
#23735=AXIS2_PLACEMENT_3D ( 'NONE', #15982, #36448, #44609 ) ;
#23736=VERTEX_POINT ( 'NONE', #16510 ) ;
#23737=VERTEX_POINT ( 'NONE', #8603 ) ;
#23738=ADVANCED_FACE ( 'NONE', ( #32526 ), #48578, .T. ) ;
#23741=AXIS2_PLACEMENT_3D ( 'NONE', #46945, #39021, #39791 ) ;
#23743=AXIS2_PLACEMENT_3D ( 'NONE', #6347, #2404, #22367 ) ;
#23744=CARTESIAN_POINT ( 'NONE',  ( 76.09804998693969935, -189.7472609257535510, 10.27263529369908746 ) ) ;
#23745=FACE_OUTER_BOUND ( 'NONE', #51053, .T. ) ;
#23746=EDGE_LOOP ( 'NONE', ( #10254, #24876, #28851, #11007 ) ) ;
#23747=PLANE ( 'NONE',  #23831 ) ;
#23748=EDGE_CURVE ( 'NONE', #32802, #16247, #4671, .T. ) ;
#23750=EDGE_CURVE ( 'NONE', #33090, #41579, #28402, .T. ) ;
#23752=DIRECTION ( 'NONE',  ( 0.000000000000000000, 1.000000000000000000, -0.000000000000000000 ) ) ;
#23753=FACE_OUTER_BOUND ( 'NONE', #24334, .T. ) ;
#23756=ORIENTED_EDGE ( 'NONE', *, *, #18392, .T. ) ;
#23758=CARTESIAN_POINT ( 'NONE',  ( -115.4536696835167930, -183.6283474603465606, -105.5434062319793895 ) ) ;
#23759=DIRECTION ( 'NONE',  ( 0.4031234292879665171, 0.000000000000000000, 0.9151456172430210145 ) ) ;
#23760=ORIENTED_EDGE ( 'NONE', *, *, #45533, .F. ) ;
#23761=CARTESIAN_POINT ( 'NONE',  ( -155.0851258170080484, -193.5000000000000000, 63.33473559879990233 ) ) ;
#23762=VECTOR ( 'NONE', #51261, 1000.000000000000000 ) ;
#23765=VERTEX_POINT ( 'NONE', #45157 ) ;
#23766=DIRECTION ( 'NONE',  ( -0.000000000000000000, 1.000000000000000000, -0.000000000000000000 ) ) ;
#23767=AXIS2_PLACEMENT_3D ( 'NONE', #11885, #28434, #16637 ) ;
#23768=VERTEX_POINT ( 'NONE', #5726 ) ;
#23770=FACE_BOUND ( 'NONE', #22542, .T. ) ;
#23772=LINE ( 'NONE', #19819, #42107 ) ;
#23773=ORIENTED_EDGE ( 'NONE', *, *, #29380, .F. ) ;
#23774=EDGE_CURVE ( 'NONE', #25657, #39370, #36000, .T. ) ;
#23775=LINE ( 'NONE', #44002, #49185 ) ;
#23776=FACE_OUTER_BOUND ( 'NONE', #4997, .T. ) ;
#23777=DIRECTION ( 'NONE',  ( -0.05924062789370748011, 0.000000000000000000, -0.9982437317643217956 ) ) ;
#23778=VECTOR ( 'NONE', #38431, 1000.000000000000000 ) ;
#23780=EDGE_CURVE ( 'NONE', #30279, #27547, #29612, .T. ) ;
#23781=ORIENTED_EDGE ( 'NONE', *, *, #30508, .F. ) ;
#23783=ORIENTED_EDGE ( 'NONE', *, *, #2739, .T. ) ;
#23784=ORIENTED_EDGE ( 'NONE', *, *, #36933, .F. ) ;
#23786=DIRECTION ( 'NONE',  ( 0.000000000000000000, -1.000000000000000000, 0.000000000000000000 ) ) ;
#23788=ORIENTED_EDGE ( 'NONE', *, *, #46082, .F. ) ;
#23791=LINE ( 'NONE', #382, #21813 ) ;
#23793=CARTESIAN_POINT ( 'NONE',  ( -1.771278280434274155, -183.6283474603465606, -115.9455772817710226 ) ) ;
#23795=ORIENTED_EDGE ( 'NONE', *, *, #47074, .F. ) ;
#23796=DIRECTION ( 'NONE',  ( -0.000000000000000000, 1.000000000000000000, -0.000000000000000000 ) ) ;
#23797=DIRECTION ( 'NONE',  ( 0.000000000000000000, 0.000000000000000000, -1.000000000000000000 ) ) ;
#23798=VECTOR ( 'NONE', #11490, 1000.000000000000114 ) ;
#23799=DIRECTION ( 'NONE',  ( -0.000000000000000000, 1.000000000000000000, -0.000000000000000000 ) ) ;
#23800=CARTESIAN_POINT ( 'NONE',  ( -48.47912675150885065, -189.7472609257535510, 6.938893903907228378E-15 ) ) ;
#23801=ORIENTED_EDGE ( 'NONE', *, *, #11751, .T. ) ;
#23802=ORIENTED_EDGE ( 'NONE', *, *, #12406, .T. ) ;
#23803=CIRCLE ( 'NONE', #32202, 125.0000000000000000 ) ;
#23804=ORIENTED_EDGE ( 'NONE', *, *, #12799, .T. ) ;
#23805=CARTESIAN_POINT ( 'NONE',  ( 64.01121016852529522, -175.3837268820161057, -54.50618404930953176 ) ) ;
#23806=CARTESIAN_POINT ( 'NONE',  ( -135.4258661347518853, -193.5000000000000000, -89.80681772907007598 ) ) ;
#23807=CARTESIAN_POINT ( 'NONE',  ( -23.99795575808071035, -183.6283474603465606, -122.5792489240757703 ) ) ;
#23811=ADVANCED_FACE ( 'NONE', ( #41961 ), #1761, .T. ) ;
#23812=EDGE_CURVE ( 'NONE', #38465, #2804, #25096, .T. ) ;
#23813=AXIS2_PLACEMENT_3D ( 'NONE', #9352, #36687, #5415 ) ;
#23814=LINE ( 'NONE', #11461, #14889 ) ;
#23815=ORIENTED_EDGE ( 'NONE', *, *, #20182, .F. ) ;
#23816=DIRECTION ( 'NONE',  ( -0.000000000000000000, 1.000000000000000000, -0.000000000000000000 ) ) ;
#23817=EDGE_LOOP ( 'NONE', ( #1180, #25735, #43379, #38615 ) ) ;
#23818=ORIENTED_EDGE ( 'NONE', *, *, #22420, .T. ) ;
#23819=DIRECTION ( 'NONE',  ( 0.000000000000000000, -1.000000000000000000, 0.000000000000000000 ) ) ;
#23821=DIRECTION ( 'NONE',  ( 0.7378332790417285736, 0.000000000000000000, -0.6749830015182091136 ) ) ;
#23822=CARTESIAN_POINT ( 'NONE',  ( 74.68865188374466868, -183.6283474603465606, 14.34663989163627740 ) ) ;
#23824=DIRECTION ( 'NONE',  ( 0.000000000000000000, 0.000000000000000000, -1.000000000000000000 ) ) ;
#23825=ORIENTED_EDGE ( 'NONE', *, *, #24240, .T. ) ;
#23826=ORIENTED_EDGE ( 'NONE', *, *, #20141, .T. ) ;
#23827=DIRECTION ( 'NONE',  ( -0.000000000000000000, 1.000000000000000000, -0.000000000000000000 ) ) ;
#23829=FACE_OUTER_BOUND ( 'NONE', #48465, .T. ) ;
#23831=AXIS2_PLACEMENT_3D ( 'NONE', #7970, #20313, #31628 ) ;
#23833=AXIS2_PLACEMENT_3D ( 'NONE', #2107, #34433, #46281 ) ;
#23834=CARTESIAN_POINT ( 'NONE',  ( -47.57632892154310866, -193.5000000000000000, -0.4300652022765113491 ) ) ;
#23835=CARTESIAN_POINT ( 'NONE',  ( -153.7332855749581881, -175.3837268820161057, 67.42819922234392038 ) ) ;
#23836=ORIENTED_EDGE ( 'NONE', *, *, #37247, .T. ) ;
#23838=DIRECTION ( 'NONE',  ( -0.000000000000000000, 1.000000000000000000, -0.000000000000000000 ) ) ;
#23839=AXIS2_PLACEMENT_3D ( 'NONE', #13829, #5176, #25397 ) ;
#23841=FACE_BOUND ( 'NONE', #35041, .T. ) ;
#23842=EDGE_LOOP ( 'NONE', ( #18118, #51336, #41735, #48002 ) ) ;
#23843=DIRECTION ( 'NONE',  ( 0.000000000000000000, -0.000000000000000000, 1.000000000000000000 ) ) ;
#23844=CARTESIAN_POINT ( 'NONE',  ( -49.47517659412406488, -193.5000000000000000, -0.08879589532293878651 ) ) ;
#23845=VERTEX_POINT ( 'NONE', #29094 ) ;
#23846=CARTESIAN_POINT ( 'NONE',  ( -148.0127667507368585, -183.6283474603465606, -75.61781872352626976 ) ) ;
#23847=AXIS2_PLACEMENT_3D ( 'NONE', #14377, #46190, #35120 ) ;
#23848=ORIENTED_EDGE ( 'NONE', *, *, #4359, .T. ) ;
#23849=CARTESIAN_POINT ( 'NONE',  ( -46.06708674231130374, -177.1207230881787780, -124.9767260852756863 ) ) ;
#23850=FACE_BOUND ( 'NONE', #22037, .T. ) ;
#23851=FACE_OUTER_BOUND ( 'NONE', #45912, .T. ) ;
#23852=LINE ( 'NONE', #19398, #50397 ) ;
#23853=EDGE_LOOP ( 'NONE', ( #23855, #32607, #40968, #4425 ) ) ;
#23854=EDGE_CURVE ( 'NONE', #15236, #46340, #13856, .T. ) ;
#23855=ORIENTED_EDGE ( 'NONE', *, *, #33675, .F. ) ;
#23856=DIRECTION ( 'NONE',  ( 0.000000000000000000, 0.000000000000000000, 1.000000000000000000 ) ) ;
#23857=ORIENTED_EDGE ( 'NONE', *, *, #51350, .F. ) ;
#23858=CARTESIAN_POINT ( 'NONE',  ( -132.6364218684650211, -193.5000000000000000, 92.42591454022807795 ) ) ;
#23859=FACE_OUTER_BOUND ( 'NONE', #46867, .T. ) ;
#23860=AXIS2_PLACEMENT_3D ( 'NONE', #18669, #11022, #18919 ) ;
#23861=EDGE_CURVE ( 'NONE', #14309, #3034, #37650, .T. ) ;
#23863=CARTESIAN_POINT ( 'NONE',  ( 41.00573479224733120, -177.1207230881787780, -87.27805883780175122 ) ) ;
#23865=ORIENTED_EDGE ( 'NONE', *, *, #40338, .F. ) ;
#23869=ADVANCED_FACE ( 'NONE', ( #17287 ), #10164, .F. ) ;
#23870=ORIENTED_EDGE ( 'NONE', *, *, #52008, .F. ) ;
#23873=CARTESIAN_POINT ( 'NONE',  ( -167.9436818089035057, -193.5000000000000000, 36.78613984830044359 ) ) ;
#23874=VERTEX_POINT ( 'NONE', #29356 ) ;
#23875=CARTESIAN_POINT ( 'NONE',  ( -56.05401443572774411, -175.3837268820161057, 124.7702732086912931 ) ) ;
#23878=CARTESIAN_POINT ( 'NONE',  ( -140.1460956102404509, -189.7472609257535510, 84.98333260264821831 ) ) ;
#23879=AXIS2_PLACEMENT_3D ( 'NONE', #50139, #6236, #6760 ) ;
#23880=VERTEX_POINT ( 'NONE', #45407 ) ;
#23883=DIRECTION ( 'NONE',  ( 0.05924062789370006937, 0.000000000000000000, 0.9982437317643222396 ) ) ;
#23884=DIRECTION ( 'NONE',  ( 0.8294056854502049880, 0.000000000000000000, -0.5586467658036476935 ) ) ;
#23885=EDGE_CURVE ( 'NONE', #5747, #25612, #45246, .T. ) ;
#23886=PLANE ( 'NONE',  #11253 ) ;
#23888=CARTESIAN_POINT ( 'NONE',  ( 5.015379008610418410, -177.1207230881787780, -112.9749434763326690 ) ) ;
#23889=CARTESIAN_POINT ( 'NONE',  ( 17.15229921100054611, -183.6283474603465606, -106.3838142112212921 ) ) ;
#23890=ORIENTED_EDGE ( 'NONE', *, *, #48225, .T. ) ;
#23892=LINE ( 'NONE', #24422, #13933 ) ;
#23893=DIRECTION ( 'NONE',  ( 0.2348860457809911206, 0.000000000000000000, -0.9720229140804089729 ) ) ;
#23894=VERTEX_POINT ( 'NONE', #14127 ) ;
#23895=VECTOR ( 'NONE', #40423, 1000.000000000000000 ) ;
#23904=AXIS2_PLACEMENT_3D ( 'NONE', #40765, #38061, #20818 ) ;
#23906=DIRECTION ( 'NONE',  ( 0.000000000000000000, 0.000000000000000000, -1.000000000000000000 ) ) ;
#23907=CIRCLE ( 'NONE', #20538, 125.0000000000000000 ) ;
#23908=LINE ( 'NONE', #11819, #17852 ) ;
#23910=VECTOR ( 'NONE', #17214, 1000.000000000000000 ) ;
#23912=EDGE_CURVE ( 'NONE', #20769, #11672, #32617, .T. ) ;
#23913=AXIS2_PLACEMENT_3D ( 'NONE', #8742, #24783, #17161 ) ;
#23916=ORIENTED_EDGE ( 'NONE', *, *, #48458, .F. ) ;
#23917=AXIS2_PLACEMENT_3D ( 'NONE', #11256, #47803, #3908 ) ;
#23918=ORIENTED_EDGE ( 'NONE', *, *, #41487, .F. ) ;
#23919=EDGE_LOOP ( 'NONE', ( #11573, #24301, #20172, #1369 ) ) ;
#23922=ORIENTED_EDGE ( 'NONE', *, *, #18309, .T. ) ;
#23923=ADVANCED_FACE ( 'NONE', ( #18572 ), #3054, .T. ) ;
#23924=EDGE_CURVE ( 'NONE', #39444, #1712, #34346, .T. ) ;
#23925=CARTESIAN_POINT ( 'NONE',  ( 58.12687231399075927, -193.5000000000000000, -63.33473559879914916 ) ) ;
#23926=LINE ( 'NONE', #42871, #51247 ) ;
#23931=AXIS2_PLACEMENT_3D ( 'NONE', #13440, #8708, #37081 ) ;
#23932=EDGE_CURVE ( 'NONE', #31839, #34695, #43000, .T. ) ;
#23933=CARTESIAN_POINT ( 'NONE',  ( -150.5215542367829471, -193.5000000000000000, -72.19655804061974891 ) ) ;
#23934=AXIS2_PLACEMENT_3D ( 'NONE', #52024, #8113, #8375 ) ;
#23935=ORIENTED_EDGE ( 'NONE', *, *, #14484, .F. ) ;
#23936=CARTESIAN_POINT ( 'NONE',  ( -38.78589637709156790, -177.1207230881787780, -123.6213615703898654 ) ) ;
#23937=ORIENTED_EDGE ( 'NONE', *, *, #32344, .T. ) ;
#23938=VECTOR ( 'NONE', #25973, 1000.000000000000000 ) ;
#23939=CARTESIAN_POINT ( 'NONE',  ( -91.81555821786918159, -189.7472609257535510, 116.1806952091180563 ) ) ;
#23942=DIRECTION ( 'NONE',  ( -0.9646355819083576311, 0.000000000000000000, -0.2635871660690715101 ) ) ;
#23943=VECTOR ( 'NONE', #180, 1000.000000000000000 ) ;
#23945=CARTESIAN_POINT ( 'NONE',  ( -138.3705904895685990, -177.1207230881787780, -86.85922373029299592 ) ) ;
#23948=ORIENTED_EDGE ( 'NONE', *, *, #16880, .F. ) ;
#23949=CARTESIAN_POINT ( 'NONE',  ( -47.51449116960048968, -177.1207230881787780, -0.2635871660690578544 ) ) ;
#23950=CARTESIAN_POINT ( 'NONE',  ( -109.9568094315246327, -183.6283474603465606, -108.8370090194290611 ) ) ;
#23952=LINE ( 'NONE', #39705, #27387 ) ;
#23953=ORIENTED_EDGE ( 'NONE', *, *, #25077, .F. ) ;
#23954=PLANE ( 'NONE',  #37675 ) ;
#23958=ORIENTED_EDGE ( 'NONE', *, *, #38240, .F. ) ;
#23959=CARTESIAN_POINT ( 'NONE',  ( -48.47912675150885065, -175.3837268820161057, 6.938893903907228378E-15 ) ) ;
#23961=CARTESIAN_POINT ( 'NONE',  ( -166.6265240196292439, -175.3837268820161057, 40.81902153125349741 ) ) ;
#23962=LINE ( 'NONE', #27385, #51312 ) ;
#23963=CARTESIAN_POINT ( 'NONE',  ( -48.47912675150885065, -175.3837268820161057, 6.938893903907228378E-15 ) ) ;
#23964=CARTESIAN_POINT ( 'NONE',  ( -121.8391548840036762, -193.5000000000000000, -99.97252634603249533 ) ) ;
#23966=DIRECTION ( 'NONE',  ( 0.3482016354343995812, 0.000000000000000000, -0.9374196611341205632 ) ) ;
#23968=DIRECTION ( 'NONE',  ( -0.9785564922995017012, 0.000000000000000000, -0.2059786187411094538 ) ) ;
#23971=ORIENTED_EDGE ( 'NONE', *, *, #18374, .F. ) ;
#23972=VECTOR ( 'NONE', #38680, 1000.000000000000000 ) ;
#23973=VECTOR ( 'NONE', #26621, 1000.000000000000000 ) ;
#23975=ORIENTED_EDGE ( 'NONE', *, *, #21815, .F. ) ;
#23977=EDGE_CURVE ( 'NONE', #36397, #17068, #46964, .T. ) ;
#23978=DIRECTION ( 'NONE',  ( 0.000000000000000000, -1.000000000000000000, 0.000000000000000000 ) ) ;
#23979=CARTESIAN_POINT ( 'NONE',  ( -48.47912675150885065, -189.7472609257535510, 6.938893903907228378E-15 ) ) ;
#23981=ORIENTED_EDGE ( 'NONE', *, *, #9296, .T. ) ;
#23982=VECTOR ( 'NONE', #41013, 1000.000000000000114 ) ;
#23984=DIRECTION ( 'NONE',  ( 0.000000000000000000, 0.000000000000000000, -1.000000000000000000 ) ) ;
#23985=CARTESIAN_POINT ( 'NONE',  ( -167.1580984288390823, -175.3837268820161057, -39.24667733211878584 ) ) ;
#23986=EDGE_CURVE ( 'NONE', #49319, #15063, #34841, .T. ) ;
#23988=EDGE_CURVE ( 'NONE', #2175, #5608, #35365, .T. ) ;
#23989=DIRECTION ( 'NONE',  ( -0.000000000000000000, 1.000000000000000000, -0.000000000000000000 ) ) ;
#23992=ORIENTED_EDGE ( 'NONE', *, *, #14535, .F. ) ;
#23993=ORIENTED_EDGE ( 'NONE', *, *, #4710, .T. ) ;
#23994=EDGE_CURVE ( 'NONE', #20319, #12264, #23306, .T. ) ;
#23998=CARTESIAN_POINT ( 'NONE',  ( 76.09804998693969935, -193.5000000000000000, 10.27263529369908746 ) ) ;
#23999=DIRECTION ( 'NONE',  ( -0.000000000000000000, 1.000000000000000000, -0.000000000000000000 ) ) ;
#24003=ORIENTED_EDGE ( 'NONE', *, *, #22979, .F. ) ;
#24005=EDGE_CURVE ( 'NONE', #1407, #2868, #23028, .T. ) ;
#24006=CARTESIAN_POINT ( 'NONE',  ( -5.113431607746569796, -189.7472609257535510, 117.2365833888819537 ) ) ;
#24007=CARTESIAN_POINT ( 'NONE',  ( 49.88781503343063406, -183.6283474603465606, -75.49882471933871386 ) ) ;
#24008=CARTESIAN_POINT ( 'NONE',  ( 57.12946453413545100, -189.7472609257535510, 66.87170886601998632 ) ) ;
#24009=ORIENTED_EDGE ( 'NONE', *, *, #5037, .T. ) ;
#24013=DIRECTION ( 'NONE',  ( -0.8455960035018311727, 0.000000000000000000, 0.5338233779647826305 ) ) ;
#24014=VECTOR ( 'NONE', #31278, 1000.000000000000227 ) ;
#24017=CARTESIAN_POINT ( 'NONE',  ( 33.09766481721658238, -175.3837268820161057, 93.38753978496653474 ) ) ;
#24019=AXIS2_PLACEMENT_3D ( 'NONE', #28663, #40490, #36045 ) ;
#24020=CARTESIAN_POINT ( 'NONE',  ( -55.05561436132770581, -193.5000000000000000, 124.8268793598474105 ) ) ;
#24022=ORIENTED_EDGE ( 'NONE', *, *, #47554, .F. ) ;
#24024=EDGE_CURVE ( 'NONE', #775, #10747, #14371, .T. ) ;
#24025=EDGE_LOOP ( 'NONE', ( #52019, #42608, #39810, #33640 ) ) ;
#24028=CARTESIAN_POINT ( 'NONE',  ( -75.48985759771373694, -183.6283474603465606, -122.0467960216648606 ) ) ;
#24029=VECTOR ( 'NONE', #41083, 1000.000000000000114 ) ;
#24031=DIRECTION ( 'NONE',  ( 0.000000000000000000, 0.000000000000000000, 1.000000000000000000 ) ) ;
#24032=ORIENTED_EDGE ( 'NONE', *, *, #29380, .T. ) ;
#24033=AXIS2_PLACEMENT_3D ( 'NONE', #49647, #13635, #6011 ) ;
#24034=VECTOR ( 'NONE', #49521, 1000.000000000000227 ) ;
#24036=CARTESIAN_POINT ( 'NONE',  ( -48.65601702663143868, -193.5000000000000000, 0.9842305779476024918 ) ) ;
#24037=LINE ( 'NONE', #40050, #5578 ) ;
#24038=VECTOR ( 'NONE', #10415, 1000.000000000000000 ) ;
#24042=VECTOR ( 'NONE', #25063, 1000.000000000000000 ) ;
#24043=ORIENTED_EDGE ( 'NONE', *, *, #33662, .F. ) ;
#24045=ORIENTED_EDGE ( 'NONE', *, *, #12598, .F. ) ;
#24047=DIRECTION ( 'NONE',  ( 0.000000000000000000, 0.000000000000000000, 1.000000000000000000 ) ) ;
#24048=EDGE_LOOP ( 'NONE', ( #1644, #14545, #43794, #37294 ) ) ;
#24050=EDGE_CURVE ( 'NONE', #11314, #34044, #50267, .T. ) ;
#24051=ORIENTED_EDGE ( 'NONE', *, *, #7054, .F. ) ;
#24053=DIRECTION ( 'NONE',  ( -0.000000000000000000, 0.000000000000000000, -1.000000000000000000 ) ) ;
#24054=EDGE_CURVE ( 'NONE', #42459, #35361, #14635, .T. ) ;
#24057=AXIS2_PLACEMENT_3D ( 'NONE', #3026, #43499, #16160 ) ;
#24058=AXIS2_PLACEMENT_3D ( 'NONE', #25090, #27971, #12709 ) ;
#24059=ORIENTED_EDGE ( 'NONE', *, *, #39204, .T. ) ;
#24060=CARTESIAN_POINT ( 'NONE',  ( -38.78589637709156790, -183.6283474603465606, -123.6213615703898654 ) ) ;
#24062=CARTESIAN_POINT ( 'NONE',  ( 11.66870402553031560, -183.6283474603465606, 108.4360005853211391 ) ) ;
#24063=EDGE_LOOP ( 'NONE', ( #43592, #48621, #6279, #21301 ) ) ;
#24064=CARTESIAN_POINT ( 'NONE',  ( 67.42090074966655777, -175.3837268820161057, -46.82076062204441769 ) ) ;
#24066=CIRCLE ( 'NONE', #48369, 125.0000000000000000 ) ;
#24067=ADVANCED_FACE ( 'NONE', ( #886, #20877, #44269, #40821, #16928, #48990, #28988, #4315, #45056, #32169, #4067, #106, #20335, #8255, #36368, #361, #16414, #32427, #48484, #47428, #43738, #51629, #23770, #3793, #15902, #10989, #8087, #7821, #15467, #2847, #18871, #15737, #27536, #19916, #31473, #44082, #19396, #30967, #47272, #39364, #51467, #47524, #3109, #31216, #11243, #19150, #7061, #31990, #38845, #15206, #43309, #23592, #51727, #7574, #34893, #35675, #35164, #47011, #27271, #50962, #51997, #23084, #14959, #23850, #11507, #27013, #43054, #39094, #3619, #51218, #7319, #23353, #3367, #35414, #43819, #48033, #43573, #39605, #31746, #19648, #35950, #47783, #39861, #3890, #11759, #27786, #15981, #12013, #28041, #49343, #13333, #20690, #44608, #444, #40141, #36447, #4398, #24897, #20424, #24625, #48293, #45150, #726, #4158, #20168, #17024 ), #36188, .T. ) ;
#24070=ORIENTED_EDGE ( 'NONE', *, *, #25077, .T. ) ;
#24071=ORIENTED_EDGE ( 'NONE', *, *, #16342, .T. ) ;
#24074=LINE ( 'NONE', #35625, #3928 ) ;
#24075=PLANE ( 'NONE',  #6718 ) ;
#24078=VECTOR ( 'NONE', #3660, 1000.000000000000000 ) ;
#24079=LINE ( 'NONE', #3842, #5852 ) ;
#24081=AXIS2_PLACEMENT_3D ( 'NONE', #51298, #27099, #22916 ) ;
#24084=DIRECTION ( 'NONE',  ( 0.5586467658036594619, 0.000000000000000000, -0.8294056854501971054 ) ) ;
#24085=VERTEX_POINT ( 'NONE', #16498 ) ;
#24087=VECTOR ( 'NONE', #28255, 1000.000000000000114 ) ;
#24089=AXIS2_PLACEMENT_3D ( 'NONE', #28595, #47557, #11542 ) ;
#24092=CARTESIAN_POINT ( 'NONE',  ( 72.05536924052414349, -175.3837268820161057, 33.11246405730899056 ) ) ;
#24093=EDGE_LOOP ( 'NONE', ( #12438, #1136, #34383, #10362 ) ) ;
#24098=DIRECTION ( 'NONE',  ( 0.9266896074318370369, 0.000000000000000000, -0.3758275821142292306 ) ) ;
#24101=ORIENTED_EDGE ( 'NONE', *, *, #35262, .F. ) ;
#24104=ORIENTED_EDGE ( 'NONE', *, *, #1230, .F. ) ;
#24106=AXIS2_PLACEMENT_3D ( 'NONE', #34857, #3070, #39332 ) ;
#24108=CARTESIAN_POINT ( 'NONE',  ( -49.46816693883101834, -193.5000000000000000, 0.1476465640024780257 ) ) ;
#24109=DIRECTION ( 'NONE',  ( 0.000000000000000000, 1.000000000000000000, -0.000000000000000000 ) ) ;
#24110=PLANE ( 'NONE',  #8821 ) ;
#24111=VECTOR ( 'NONE', #12662, 1000.000000000000000 ) ;
#24112=DIRECTION ( 'NONE',  ( 0.000000000000000000, 0.000000000000000000, -1.000000000000000000 ) ) ;
#24113=CARTESIAN_POINT ( 'NONE',  ( -172.0839188101924719, -189.7472609257535510, -18.62405380494754681 ) ) ;
#24116=DIRECTION ( 'NONE',  ( 0.000000000000000000, 0.000000000000000000, 1.000000000000000000 ) ) ;
#24117=FACE_BOUND ( 'NONE', #32547, .T. ) ;
#24118=ORIENTED_EDGE ( 'NONE', *, *, #9529, .F. ) ;
#24119=CIRCLE ( 'NONE', #13195, 125.0000000000000000 ) ;
#24120=VECTOR ( 'NONE', #16903, 1000.000000000000000 ) ;
#24121=DIRECTION ( 'NONE',  ( 0.000000000000000000, -1.000000000000000000, -0.000000000000000000 ) ) ;
#24122=AXIS2_PLACEMENT_3D ( 'NONE', #14649, #2812, #34859 ) ;
#24123=DIRECTION ( 'NONE',  ( 0.000000000000000000, -1.000000000000000000, 0.000000000000000000 ) ) ;
#24124=EDGE_CURVE ( 'NONE', #48059, #49114, #29081, .T. ) ;
#24125=EDGE_LOOP ( 'NONE', ( #21391, #37501, #45279, #25809 ) ) ;
#24126=ADVANCED_FACE ( 'NONE', ( #32520 ), #48569, .T. ) ;
#24127=CARTESIAN_POINT ( 'NONE',  ( 75.67769207106684348, -177.1207230881787780, 14.49428645563876650 ) ) ;
#24130=AXIS2_PLACEMENT_3D ( 'NONE', #6878, #18710, #34724 ) ;
#24132=DIRECTION ( 'NONE',  ( 0.000000000000000000, 0.000000000000000000, 1.000000000000000000 ) ) ;
#24136=VERTEX_POINT ( 'NONE', #16771 ) ;
#24137=ORIENTED_EDGE ( 'NONE', *, *, #39398, .T. ) ;
#24138=DIRECTION ( 'NONE',  ( 0.000000000000000000, 1.000000000000000000, 0.000000000000000000 ) ) ;
#24139=AXIS2_PLACEMENT_3D ( 'NONE', #19311, #35324, #50338 ) ;
#24140=CIRCLE ( 'NONE', #1478, 125.0000000000000000 ) ;
#24144=CARTESIAN_POINT ( 'NONE',  ( 14.37129481273060172, -175.3837268820161057, -108.0501018472328099 ) ) ;
#24147=CARTESIAN_POINT ( 'NONE',  ( -110.8210171970983566, -189.7472609257535510, 107.1890582354659074 ) ) ;
#24148=ORIENTED_EDGE ( 'NONE', *, *, #14324, .T. ) ;
#24151=ORIENTED_EDGE ( 'NONE', *, *, #38996, .T. ) ;
#24155=VECTOR ( 'NONE', #13752, 1000.000000000000000 ) ;
#24156=PLANE ( 'NONE',  #43279 ) ;
#24158=CARTESIAN_POINT ( 'NONE',  ( 66.49421114223471818, -193.5000000000000000, -46.44493303993018429 ) ) ;
#24160=LINE ( 'NONE', #32274, #39303 ) ;
#24161=EDGE_LOOP ( 'NONE', ( #5745, #22757, #42888, #38340 ) ) ;
#24163=CARTESIAN_POINT ( 'NONE',  ( -47.78257572244586271, -183.6283474603465606, 0.7175072570443418174 ) ) ;
#24166=EDGE_LOOP ( 'NONE', ( #11833, #2487, #9986, #40100 ) ) ;
#24167=DIRECTION ( 'NONE',  ( -0.000000000000000000, 1.000000000000000000, -0.000000000000000000 ) ) ;
#24168=DIRECTION ( 'NONE',  ( 0.6300878435817148793, 0.000000000000000000, -0.7765238627180394149 ) ) ;
#24170=CARTESIAN_POINT ( 'NONE',  ( 31.84037011350117297, -175.3837268820161057, -94.47107458416900272 ) ) ;
#24172=DIRECTION ( 'NONE',  ( -0.4031234292879665171, 0.000000000000000000, -0.9151456172430210145 ) ) ;
#24173=ORIENTED_EDGE ( 'NONE', *, *, #24184, .F. ) ;
#24176=CARTESIAN_POINT ( 'NONE',  ( -134.9734323446613473, -189.7472609257535510, 88.85232316304889366 ) ) ;
#24180=VECTOR ( 'NONE', #9334, 1000.000000000000000 ) ;
#24184=EDGE_CURVE ( 'NONE', #49764, #23726, #30375, .T. ) ;
#24185=ORIENTED_EDGE ( 'NONE', *, *, #39151, .F. ) ;
#24186=VERTEX_POINT ( 'NONE', #17546 ) ;
#24188=DIRECTION ( 'NONE',  ( 0.000000000000000000, -1.000000000000000000, 0.000000000000000000 ) ) ;
#24189=CARTESIAN_POINT ( 'NONE',  ( -69.77312546433407192, -175.3837268820161057, 123.1729094355500109 ) ) ;
#24191=PLANE ( 'NONE',  #42152 ) ;
#24197=ORIENTED_EDGE ( 'NONE', *, *, #9939, .T. ) ;
#24198=EDGE_CURVE ( 'NONE', #32264, #49114, #33561, .T. ) ;
#24199=DIRECTION ( 'NONE',  ( -0.5586467658036535777, 0.000000000000000000, 0.8294056854502011022 ) ) ;
#24200=ORIENTED_EDGE ( 'NONE', *, *, #29496, .T. ) ;
#24201=LINE ( 'NONE', #16309, #31745 ) ;
#24202=CARTESIAN_POINT ( 'NONE',  ( -90.87721961371605062, -193.5000000000000000, 116.5264228893328635 ) ) ;
#24203=CARTESIAN_POINT ( 'NONE',  ( -142.3192003680973130, -193.5000000000000000, 82.57748230379306165 ) ) ;
#24208=EDGE_CURVE ( 'NONE', #23027, #51264, #1497, .T. ) ;
#24210=ORIENTED_EDGE ( 'NONE', *, *, #37557, .T. ) ;
#24211=CARTESIAN_POINT ( 'NONE',  ( -117.6201219941651601, -175.3837268820161057, 104.1370384486469902 ) ) ;
#24212=AXIS2_PLACEMENT_3D ( 'NONE', #5275, #28897, #797 ) ;
#24214=DIRECTION ( 'NONE',  ( -0.000000000000000000, 1.000000000000000000, -0.000000000000000000 ) ) ;
#24218=DIRECTION ( 'NONE',  ( 0.000000000000000000, 0.000000000000000000, 1.000000000000000000 ) ) ;
#24220=DIRECTION ( 'NONE',  ( -0.000000000000000000, 1.000000000000000000, -0.000000000000000000 ) ) ;
#24222=ORIENTED_EDGE ( 'NONE', *, *, #28561, .F. ) ;
#24223=DIRECTION ( 'NONE',  ( -0.000000000000000000, -1.000000000000000000, 0.000000000000000000 ) ) ;
#24224=FACE_OUTER_BOUND ( 'NONE', #27612, .T. ) ;
#24227=DIRECTION ( 'NONE',  ( 0.7948544414133481562, 0.000000000000000000, 0.6068001458186002006 ) ) ;
#24229=AXIS2_PLACEMENT_3D ( 'NONE', #4127, #40880, #32488 ) ;
#24230=EDGE_CURVE ( 'NONE', #41086, #45277, #12509, .T. ) ;
#24231=ORIENTED_EDGE ( 'NONE', *, *, #14748, .T. ) ;
#24232=CARTESIAN_POINT ( 'NONE',  ( 1.663811650136604481, -193.5000000000000000, -113.4093733337827672 ) ) ;
#24234=DIRECTION ( 'NONE',  ( 0.8757349421956379665, 0.000000000000000000, -0.4827922027307427477 ) ) ;
#24235=DIRECTION ( 'NONE',  ( 0.000000000000000000, 0.000000000000000000, 1.000000000000000000 ) ) ;
#24236=FACE_OUTER_BOUND ( 'NONE', #26487, .T. ) ;
#24237=LINE ( 'NONE', #3476, #24743 ) ;
#24240=EDGE_CURVE ( 'NONE', #29344, #20898, #18046, .T. ) ;
#24242=VECTOR ( 'NONE', #7433, 1000.000000000000000 ) ;
#24243=EDGE_CURVE ( 'NONE', #24900, #39679, #47781, .T. ) ;
#24244=VECTOR ( 'NONE', #3378, 1000.000000000000000 ) ;
#24251=DIRECTION ( 'NONE',  ( -0.000000000000000000, 1.000000000000000000, -0.000000000000000000 ) ) ;
#24252=FACE_OUTER_BOUND ( 'NONE', #44225, .T. ) ;
#24253=ORIENTED_EDGE ( 'NONE', *, *, #33844, .T. ) ;
#24254=VECTOR ( 'NONE', #51934, 1000.000000000000000 ) ;
#24255=EDGE_LOOP ( 'NONE', ( #6063, #9592, #30554, #46024 ) ) ;
#24256=ORIENTED_EDGE ( 'NONE', *, *, #46239, .T. ) ;
#24259=DIRECTION ( 'NONE',  ( -0.000000000000000000, 1.000000000000000000, 0.000000000000000000 ) ) ;
#24262=ORIENTED_EDGE ( 'NONE', *, *, #17007, .F. ) ;
#24266=LINE ( 'NONE', #15610, #34426 ) ;
#24270=ORIENTED_EDGE ( 'NONE', *, *, #38250, .T. ) ;
#24271=DIRECTION ( 'NONE',  ( -0.000000000000000000, 1.000000000000000000, -0.000000000000000000 ) ) ;
#24272=LINE ( 'NONE', #40277, #50125 ) ;
#24273=DIRECTION ( 'NONE',  ( 0.000000000000000000, -1.000000000000000000, 0.000000000000000000 ) ) ;
#24275=EDGE_LOOP ( 'NONE', ( #21237, #18041, #9729, #16657 ) ) ;
#24276=ORIENTED_EDGE ( 'NONE', *, *, #16334, .F. ) ;
#24277=ORIENTED_EDGE ( 'NONE', *, *, #45496, .T. ) ;
#24278=CARTESIAN_POINT ( 'NONE',  ( -68.09401750944518028, -183.6283474603465606, -122.4396006697294581 ) ) ;
#24280=AXIS2_PLACEMENT_3D ( 'NONE', #51217, #2846, #11241 ) ;
#24282=DIRECTION ( 'NONE',  ( 0.000000000000000000, 1.000000000000000000, 0.000000000000000000 ) ) ;
#24283=CIRCLE ( 'NONE', #39382, 124.9999999999999858 ) ;
#24284=DIRECTION ( 'NONE',  ( -0.000000000000000000, 1.000000000000000000, -0.000000000000000000 ) ) ;
#24285=ADVANCED_FACE ( 'NONE', ( #2279 ), #38535, .T. ) ;
#24287=ORIENTED_EDGE ( 'NONE', *, *, #50302, .T. ) ;
#24289=CARTESIAN_POINT ( 'NONE',  ( -11.80936624585915418, -189.7472609257535510, -119.5003291395395877 ) ) ;
#24291=FACE_OUTER_BOUND ( 'NONE', #4617, .T. ) ;
#24292=DIRECTION ( 'NONE',  ( -0.8757349421956310831, 0.000000000000000000, -0.4827922027307550712 ) ) ;
#24293=VERTEX_POINT ( 'NONE', #21987 ) ;
#24296=CARTESIAN_POINT ( 'NONE',  ( -152.8713435144644563, -183.6283474603465606, -68.75510947788596638 ) ) ;
#24298=FACE_OUTER_BOUND ( 'NONE', #18357, .T. ) ;
#24299=ADVANCED_FACE ( 'NONE', ( #50374 ), #26433, .T. ) ;
#24300=VECTOR ( 'NONE', #25009, 1000.000000000000000 ) ;
#24301=ORIENTED_EDGE ( 'NONE', *, *, #31700, .F. ) ;
#24302=CARTESIAN_POINT ( 'NONE',  ( -23.99795575808071035, -177.1207230881787780, -122.5792489240757703 ) ) ;
#24304=ORIENTED_EDGE ( 'NONE', *, *, #14633, .F. ) ;
#24305=EDGE_CURVE ( 'NONE', #41471, #10047, #36856, .T. ) ;
#24306=CARTESIAN_POINT ( 'NONE',  ( 59.00260725618642965, -177.1207230881787780, -63.81752780152989857 ) ) ;
#24307=DIRECTION ( 'NONE',  ( 0.000000000000000000, -1.000000000000000000, 0.000000000000000000 ) ) ;
#24309=ADVANCED_FACE ( 'NONE', ( #18562 ), #21734, .F. ) ;
#24310=ORIENTED_EDGE ( 'NONE', *, *, #41519, .T. ) ;
#24312=CARTESIAN_POINT ( 'NONE',  ( -48.47912675150883643, -175.3837268820161057, -125.0000000000000000 ) ) ;
#24315=CARTESIAN_POINT ( 'NONE',  ( -48.64924157374594671, -193.5000000000000000, 123.9998842437354227 ) ) ;
#24318=FACE_OUTER_BOUND ( 'NONE', #13479, .T. ) ;
#24319=CARTESIAN_POINT ( 'NONE',  ( 12.54192669111252734, -177.1207230881787780, 107.9473519284347418 ) ) ;
#24320=CARTESIAN_POINT ( 'NONE',  ( -173.2419626162308646, -183.6283474603465606, 7.696413904698412800 ) ) ;
#24321=FACE_OUTER_BOUND ( 'NONE', #10686, .T. ) ;
#24322=ORIENTED_EDGE ( 'NONE', *, *, #35138, .T. ) ;
#24323=EDGE_LOOP ( 'NONE', ( #26795, #35922, #10950, #6186 ) ) ;
#24324=ORIENTED_EDGE ( 'NONE', *, *, #21289, .F. ) ;
#24325=CARTESIAN_POINT ( 'NONE',  ( -148.7414553014637590, -189.7472609257535510, 72.96212019587208886 ) ) ;
#24331=AXIS2_PLACEMENT_3D ( 'NONE', #25616, #28766, #41130 ) ;
#24332=VECTOR ( 'NONE', #25862, 1000.000000000000000 ) ;
#24333=EDGE_CURVE ( 'NONE', #32376, #39548, #33809, .T. ) ;
#24334=EDGE_LOOP ( 'NONE', ( #37710, #29119, #25239, #27574 ) ) ;
#24336=ORIENTED_EDGE ( 'NONE', *, *, #2756, .T. ) ;
#24338=DIRECTION ( 'NONE',  ( 0.8455960035018272869, 0.000000000000000000, -0.5338233779647886257 ) ) ;
#24339=FACE_OUTER_BOUND ( 'NONE', #17080, .T. ) ;
#24340=ADVANCED_FACE ( 'NONE', ( #14622 ), #9390, .T. ) ;
#24342=EDGE_CURVE ( 'NONE', #9658, #35836, #15148, .T. ) ;
#24346=LINE ( 'NONE', #4630, #5729 ) ;
#24348=EDGE_CURVE ( 'NONE', #10662, #23768, #14895, .T. ) ;
#24349=VERTEX_POINT ( 'NONE', #51665 ) ;
#24350=DIRECTION ( 'NONE',  ( -0.000000000000000000, 1.000000000000000000, -0.000000000000000000 ) ) ;
#24353=CARTESIAN_POINT ( 'NONE',  ( -94.78385179329468713, -193.5000000000000000, 115.0304316645283222 ) ) ;
#24355=PLANE ( 'NONE',  #18875 ) ;
#24356=DIRECTION ( 'NONE',  ( 0.000000000000000000, -0.000000000000000000, 1.000000000000000000 ) ) ;
#24357=DIRECTION ( 'NONE',  ( 0.000000000000000000, 1.000000000000000000, 0.000000000000000000 ) ) ;
#24358=EDGE_CURVE ( 'NONE', #37425, #7460, #15665, .T. ) ;
#24359=ORIENTED_EDGE ( 'NONE', *, *, #16489, .F. ) ;
#24360=DIRECTION ( 'NONE',  ( -0.000000000000000000, 1.000000000000000000, -0.000000000000000000 ) ) ;
#24362=EDGE_CURVE ( 'NONE', #40230, #37865, #19589, .T. ) ;
#24363=CARTESIAN_POINT ( 'NONE',  ( -28.74596282265200387, -183.6283474603465606, 123.4325817657431230 ) ) ;
#24364=FACE_BOUND ( 'NONE', #44575, .T. ) ;
#24365=ORIENTED_EDGE ( 'NONE', *, *, #35612, .F. ) ;
#24366=EDGE_CURVE ( 'NONE', #17543, #36353, #43242, .T. ) ;
#24367=CARTESIAN_POINT ( 'NONE',  ( -48.88225018079683082, -177.1207230881787780, 0.9151456172430223468 ) ) ;
#24368=LINE ( 'NONE', #5188, #2608 ) ;
#24372=ORIENTED_EDGE ( 'NONE', *, *, #9184, .T. ) ;
#24374=VECTOR ( 'NONE', #12425, 1000.000000000000000 ) ;
#24376=CARTESIAN_POINT ( 'NONE',  ( -48.47912675150885065, -189.7472609257535510, 6.938893903907228378E-15 ) ) ;
#24378=DIRECTION ( 'NONE',  ( 0.000000000000000000, -0.000000000000000000, -1.000000000000000000 ) ) ;
#24379=DIRECTION ( 'NONE',  ( 0.000000000000000000, 0.000000000000000000, 1.000000000000000000 ) ) ;
#24380=EDGE_CURVE ( 'NONE', #14956, #2833, #42739, .T. ) ;
#24381=ORIENTED_EDGE ( 'NONE', *, *, #13872, .F. ) ;
#24382=ORIENTED_EDGE ( 'NONE', *, *, #9116, .F. ) ;
#24383=DIRECTION ( 'NONE',  ( 0.000000000000000000, -1.000000000000000000, 0.000000000000000000 ) ) ;
#24384=VECTOR ( 'NONE', #8598, 1000.000000000000000 ) ;
#24385=VERTEX_POINT ( 'NONE', #51164 ) ;
#24386=CARTESIAN_POINT ( 'NONE',  ( -48.47912675150885065, -183.6283474603465606, 6.938893903907228378E-15 ) ) ;
#24387=FACE_OUTER_BOUND ( 'NONE', #999, .T. ) ;
#24388=PLANE ( 'NONE',  #31383 ) ;
#24391=ORIENTED_EDGE ( 'NONE', *, *, #14402, .T. ) ;
#24392=PLANE ( 'NONE',  #28344 ) ;
#24393=DIRECTION ( 'NONE',  ( -0.000000000000000000, 1.000000000000000000, -0.000000000000000000 ) ) ;
#24394=ORIENTED_EDGE ( 'NONE', *, *, #10533, .F. ) ;
#24395=ORIENTED_EDGE ( 'NONE', *, *, #37829, .F. ) ;
#24396=LINE ( 'NONE', #48849, #3863 ) ;
#24397=EDGE_LOOP ( 'NONE', ( #25421, #47181, #33909, #51690 ) ) ;
#24398=CARTESIAN_POINT ( 'NONE',  ( -48.77118352214583297, -189.7472609257535510, 0.9564009842765270886 ) ) ;
#24399=CIRCLE ( 'NONE', #31114, 125.0000000000000000 ) ;
#24401=EDGE_CURVE ( 'NONE', #50764, #18911, #23291, .T. ) ;
#24404=DIRECTION ( 'NONE',  ( -0.000000000000000000, 1.000000000000000000, -0.000000000000000000 ) ) ;
#24405=ORIENTED_EDGE ( 'NONE', *, *, #41361, .F. ) ;
#24406=DIRECTION ( 'NONE',  ( 0.5338233779647948429, 0.000000000000000000, -0.8455960035018234011 ) ) ;
#24407=DIRECTION ( 'NONE',  ( -0.8455960035018199594, 0.000000000000000000, -0.5338233779648003940 ) ) ;
#24408=VERTEX_POINT ( 'NONE', #27205 ) ;
#24409=EDGE_CURVE ( 'NONE', #21525, #24900, #39307, .T. ) ;
#24411=EDGE_CURVE ( 'NONE', #4174, #19776, #15405, .T. ) ;
#24412=ORIENTED_EDGE ( 'NONE', *, *, #11312, .F. ) ;
#24413=DIRECTION ( 'NONE',  ( 0.000000000000000000, 0.000000000000000000, 1.000000000000000000 ) ) ;
#24414=CARTESIAN_POINT ( 'NONE',  ( -85.77912150413021664, -193.5000000000000000, -119.3051146910911768 ) ) ;
#24415=CARTESIAN_POINT ( 'NONE',  ( -49.40581635894069024, -189.7472609257535510, 0.3758275821142362250 ) ) ;
#24417=DIRECTION ( 'NONE',  ( 0.000000000000000000, -1.000000000000000000, -0.000000000000000000 ) ) ;
#24418=ORIENTED_EDGE ( 'NONE', *, *, #10876, .F. ) ;
#24420=CARTESIAN_POINT ( 'NONE',  ( -51.83230197877468015, -177.1207230881787780, 123.9551692589637639 ) ) ;
#24422=CARTESIAN_POINT ( 'NONE',  ( 69.88207517204676833, -189.7472609257535510, 40.19484891390058579 ) ) ;
#24423=CARTESIAN_POINT ( 'NONE',  ( -19.92568551777507224, -193.5000000000000000, -121.6951149130962904 ) ) ;
#24424=ORIENTED_EDGE ( 'NONE', *, *, #39397, .T. ) ;
#24426=FACE_OUTER_BOUND ( 'NONE', #44169, .T. ) ;
#24427=ADVANCED_FACE ( 'NONE', ( #130 ), #9074, .T. ) ;
#24428=CARTESIAN_POINT ( 'NONE',  ( -48.47912675150885065, -183.6283474603465606, 6.938893903907228378E-15 ) ) ;
#24429=CARTESIAN_POINT ( 'NONE',  ( -170.0502155641509319, -177.1207230881787780, -29.07697310430878090 ) ) ;
#24430=VERTEX_POINT ( 'NONE', #16959 ) ;
#24431=ORIENTED_EDGE ( 'NONE', *, *, #23167, .F. ) ;
#24433=EDGE_CURVE ( 'NONE', #50666, #34406, #37351, .T. ) ;
#24434=CARTESIAN_POINT ( 'NONE',  ( -48.47912675150885065, -175.3837268820161057, 6.938893903907228378E-15 ) ) ;
#24436=DIRECTION ( 'NONE',  ( -0.000000000000000000, 1.000000000000000000, -0.000000000000000000 ) ) ;
#24437=DIRECTION ( 'NONE',  ( -0.000000000000000000, 1.000000000000000000, -0.000000000000000000 ) ) ;
#24438=AXIS2_PLACEMENT_3D ( 'NONE', #32879, #20028, #40243 ) ;
#24441=CARTESIAN_POINT ( 'NONE',  ( 52.36832552120770146, -193.5000000000000000, -72.15117186584490128 ) ) ;
#24442=ORIENTED_EDGE ( 'NONE', *, *, #39677, .F. ) ;
#24443=CIRCLE ( 'NONE', #4298, 125.0000000000000000 ) ;
#24444=ORIENTED_EDGE ( 'NONE', *, *, #12717, .T. ) ;
#24448=FACE_OUTER_BOUND ( 'NONE', #10927, .T. ) ;
#24449=LINE ( 'NONE', #8950, #49977 ) ;
#24450=CARTESIAN_POINT ( 'NONE',  ( -166.0019676197264005, -189.7472609257535510, 39.55227055146323067 ) ) ;
#24452=AXIS2_PLACEMENT_3D ( 'NONE', #28441, #24259, #44747 ) ;
#24453=FACE_OUTER_BOUND ( 'NONE', #21478, .T. ) ;
#24454=ORIENTED_EDGE ( 'NONE', *, *, #23297, .F. ) ;
#24455=CARTESIAN_POINT ( 'NONE',  ( 36.84288420123323249, -177.1207230881787780, 91.35181687837503262 ) ) ;
#24457=ORIENTED_EDGE ( 'NONE', *, *, #25097, .F. ) ;
#24459=DIRECTION ( 'NONE',  ( 0.000000000000000000, -1.000000000000000000, -0.000000000000000000 ) ) ;
#24460=ADVANCED_FACE ( 'NONE', ( #29018 ), #16710, .F. ) ;
#24461=DIRECTION ( 'NONE',  ( 0.000000000000000000, 0.000000000000000000, -1.000000000000000000 ) ) ;
#24462=DIRECTION ( 'NONE',  ( 0.000000000000000000, -1.000000000000000000, 0.000000000000000000 ) ) ;
#24464=ORIENTED_EDGE ( 'NONE', *, *, #48396, .T. ) ;
#24465=DIRECTION ( 'NONE',  ( -0.3482016354343866471, 0.000000000000000000, -0.9374196611341253371 ) ) ;
#24466=DIRECTION ( 'NONE',  ( -0.9646355819083576311, 0.000000000000000000, -0.2635871660690715101 ) ) ;
#24467=ORIENTED_EDGE ( 'NONE', *, *, #26000, .T. ) ;
#24468=CARTESIAN_POINT ( 'NONE',  ( -173.4291566779743050, -193.5000000000000000, 3.534122433558352760 ) ) ;
#24470=VECTOR ( 'NONE', #37223, 1000.000000000000000 ) ;
#24471=CARTESIAN_POINT ( 'NONE',  ( -156.2577088867455473, -177.1207230881787780, -63.31490529818420754 ) ) ;
#24473=CARTESIAN_POINT ( 'NONE',  ( -135.6699833737243353, -175.3837268820161057, 89.56983042009326823 ) ) ;
#24475=LINE ( 'NONE', #20530, #39860 ) ;
#24476=VERTEX_POINT ( 'NONE', #12215 ) ;
#24477=CARTESIAN_POINT ( 'NONE',  ( 8.448131207122532516, -193.5000000000000000, 111.2847127925100352 ) ) ;
#24478=ORIENTED_EDGE ( 'NONE', *, *, #2923, .T. ) ;
#24479=LINE ( 'NONE', #43936, #25628 ) ;
#24480=DIRECTION ( 'NONE',  ( -0.000000000000000000, 1.000000000000000000, -0.000000000000000000 ) ) ;
#24481=EDGE_CURVE ( 'NONE', #13211, #17151, #28965, .T. ) ;
#24482=CARTESIAN_POINT ( 'NONE',  ( -162.7543581613524282, -193.5000000000000000, 50.65739320402010293 ) ) ;
#24483=PLANE ( 'NONE',  #14690 ) ;
#24486=ADVANCED_FACE ( 'NONE', ( #25108 ), #47973, .T. ) ;
#24489=CARTESIAN_POINT ( 'NONE',  ( 31.28129687248616619, -193.5000000000000000, 96.24590808611479531 ) ) ;
#24491=DIRECTION ( 'NONE',  ( -0.000000000000000000, 1.000000000000000000, -0.000000000000000000 ) ) ;
#24492=ORIENTED_EDGE ( 'NONE', *, *, #8294, .F. ) ;
#24495=EDGE_CURVE ( 'NONE', #20143, #50250, #24567, .T. ) ;
#24496=CARTESIAN_POINT ( 'NONE',  ( -98.71382891444399377, -175.3837268820161057, -114.4616734920523555 ) ) ;
#24497=ORIENTED_EDGE ( 'NONE', *, *, #10184, .T. ) ;
#24499=VERTEX_POINT ( 'NONE', #24060 ) ;
#24500=DIRECTION ( 'NONE',  ( -0.000000000000000000, 1.000000000000000000, -0.000000000000000000 ) ) ;
#24501=VECTOR ( 'NONE', #17199, 1000.000000000000114 ) ;
#24505=ORIENTED_EDGE ( 'NONE', *, *, #42848, .T. ) ;
#24510=LINE ( 'NONE', #51604, #4834 ) ;
#24511=CARTESIAN_POINT ( 'NONE',  ( -139.4082623311987277, -189.7472609257535510, 84.30834960113001841 ) ) ;
#24512=DIRECTION ( 'NONE',  ( -0.6965510290629932655, 0.000000000000000000, -0.7175072570443347120 ) ) ;
#24520=EDGE_CURVE ( 'NONE', #51281, #19239, #384, .T. ) ;
#24521=CARTESIAN_POINT ( 'NONE',  ( -48.13092511607445090, -193.5000000000000000, -0.9374196611341135688 ) ) ;
#24522=DIRECTION ( 'NONE',  ( -0.6068001458185945385, 0.000000000000000000, 0.7948544414133523750 ) ) ;
#24524=VECTOR ( 'NONE', #22793, 1000.000000000000114 ) ;
#24526=AXIS2_PLACEMENT_3D ( 'NONE', #20364, #43761, #19590 ) ;
#24529=VECTOR ( 'NONE', #5928, 1000.000000000000114 ) ;
#24530=LINE ( 'NONE', #48466, #44049 ) ;
#24531=PLANE ( 'NONE',  #6552 ) ;
#24532=ORIENTED_EDGE ( 'NONE', *, *, #23098, .T. ) ;
#24534=CARTESIAN_POINT ( 'NONE',  ( -13.05859477122062806, -193.5000000000000000, -118.8334608768479654 ) ) ;
#24536=ORIENTED_EDGE ( 'NONE', *, *, #3377, .F. ) ;
#24537=CARTESIAN_POINT ( 'NONE',  ( 47.70255505652111339, -175.3837268820161057, 78.26291788638732783 ) ) ;
#24540=DIRECTION ( 'NONE',  ( 0.000000000000000000, 1.000000000000000000, -0.000000000000000000 ) ) ;
#24541=ORIENTED_EDGE ( 'NONE', *, *, #15090, .T. ) ;
#24544=VERTEX_POINT ( 'NONE', #20905 ) ;
#24548=CARTESIAN_POINT ( 'NONE',  ( 75.46126020185813843, -193.5000000000000000, 3.844569333773215192 ) ) ;
#24549=DIRECTION ( 'NONE',  ( 0.000000000000000000, 0.000000000000000000, -1.000000000000000000 ) ) ;
#24551=ORIENTED_EDGE ( 'NONE', *, *, #28832, .F. ) ;
#24552=FACE_OUTER_BOUND ( 'NONE', #29798, .T. ) ;
#24553=ORIENTED_EDGE ( 'NONE', *, *, #32052, .T. ) ;
#24554=ORIENTED_EDGE ( 'NONE', *, *, #29448, .F. ) ;
#24555=DIRECTION ( 'NONE',  ( -0.000000000000000000, 1.000000000000000000, -0.000000000000000000 ) ) ;
#24557=ORIENTED_EDGE ( 'NONE', *, *, #31286, .F. ) ;
#24561=VECTOR ( 'NONE', #28527, 999.9999999999998863 ) ;
#24562=DIRECTION ( 'NONE',  ( -0.000000000000000000, 1.000000000000000000, -0.000000000000000000 ) ) ;
#24563=CARTESIAN_POINT ( 'NONE',  ( 30.05499637021958392, -193.5000000000000000, -97.24912084693205827 ) ) ;
#24565=CIRCLE ( 'NONE', #35472, 125.0000000000000000 ) ;
#24567=LINE ( 'NONE', #40580, #13876 ) ;
#24568=ORIENTED_EDGE ( 'NONE', *, *, #37821, .F. ) ;
#24569=DIRECTION ( 'NONE',  ( 0.000000000000000000, -0.000000000000000000, -1.000000000000000000 ) ) ;
#24570=PLANE ( 'NONE',  #30853 ) ;
#24572=DIRECTION ( 'NONE',  ( 0.1768902751225666370, 0.000000000000000000, 0.9842305779475979399 ) ) ;
#24573=CARTESIAN_POINT ( 'NONE',  ( 10.73478887071927623, -177.1207230881787780, -110.0850225811106924 ) ) ;
#24576=ORIENTED_EDGE ( 'NONE', *, *, #20147, .T. ) ;
#24577=DIRECTION ( 'NONE',  ( 0.2635871660690581320, 0.000000000000000000, 0.9646355819083614058 ) ) ;
#24578=PLANE ( 'NONE',  #19 ) ;
#24581=DIRECTION ( 'NONE',  ( -0.000000000000000000, 1.000000000000000000, -0.000000000000000000 ) ) ;
#24586=CIRCLE ( 'NONE', #45581, 125.0000000000000000 ) ;
#24588=FACE_OUTER_BOUND ( 'NONE', #43595, .T. ) ;
#24589=VERTEX_POINT ( 'NONE', #45085 ) ;
#24591=EDGE_CURVE ( 'NONE', #12134, #2552, #38207, .T. ) ;
#24592=PLANE ( 'NONE',  #37522 ) ;
#24596=ORIENTED_EDGE ( 'NONE', *, *, #35799, .F. ) ;
#24602=DIRECTION ( 'NONE',  ( 0.000000000000000000, -0.000000000000000000, 1.000000000000000000 ) ) ;
#24605=DIRECTION ( 'NONE',  ( -0.000000000000000000, 1.000000000000000000, -0.000000000000000000 ) ) ;
#24607=DIRECTION ( 'NONE',  ( 0.8455960035018234011, 0.000000000000000000, 0.5338233779647948429 ) ) ;
#24609=VECTOR ( 'NONE', #31151, 1000.000000000000000 ) ;
#24610=EDGE_LOOP ( 'NONE', ( #29900, #21659, #33322, #47207 ) ) ;
#24614=FACE_BOUND ( 'NONE', #38704, .T. ) ;
#24615=ORIENTED_EDGE ( 'NONE', *, *, #20788, .F. ) ;
#24617=ORIENTED_EDGE ( 'NONE', *, *, #4779, .T. ) ;
#24618=AXIS2_PLACEMENT_3D ( 'NONE', #42314, #6331, #11800 ) ;
#24620=VERTEX_POINT ( 'NONE', #14055 ) ;
#24621=DIRECTION ( 'NONE',  ( 0.000000000000000000, 0.000000000000000000, -1.000000000000000000 ) ) ;
#24622=ORIENTED_EDGE ( 'NONE', *, *, #29520, .F. ) ;
#24623=AXIS2_PLACEMENT_3D ( 'NONE', #22124, #26057, #42086 ) ;
#24624=DIRECTION ( 'NONE',  ( -0.9890401873221654760, 0.000000000000000000, 0.1476465640024710868 ) ) ;
#24625=FACE_BOUND ( 'NONE', #25964, .T. ) ;
#24628=EDGE_CURVE ( 'NONE', #9774, #45236, #9581, .T. ) ;
#24630=EDGE_CURVE ( 'NONE', #33552, #34512, #26425, .T. ) ;
#24631=CARTESIAN_POINT ( 'NONE',  ( -49.40581635894068313, -183.6283474603465606, -0.3758275821142418316 ) ) ;
#24632=ORIENTED_EDGE ( 'NONE', *, *, #38831, .F. ) ;
#24634=ORIENTED_EDGE ( 'NONE', *, *, #46430, .T. ) ;
#24635=CARTESIAN_POINT ( 'NONE',  ( 41.00573479224733120, -177.1207230881787780, -87.27805883780175122 ) ) ;
#24636=VECTOR ( 'NONE', #16986, 1000.000000000000000 ) ;
#24638=ADVANCED_FACE ( 'NONE', ( #46370 ), #33752, .T. ) ;
#24639=DIRECTION ( 'NONE',  ( 0.000000000000000000, 0.000000000000000000, -1.000000000000000000 ) ) ;
#24643=EDGE_CURVE ( 'NONE', #42167, #45648, #39844, .T. ) ;
#24644=EDGE_CURVE ( 'NONE', #27476, #23880, #35656, .T. ) ;
#24645=CARTESIAN_POINT ( 'NONE',  ( 64.44365795514079309, -193.5000000000000000, -53.60452120946194299 ) ) ;
#24646=CARTESIAN_POINT ( 'NONE',  ( 41.41233698655026529, -177.1207230881787780, 86.85922373029362120 ) ) ;
#24647=ORIENTED_EDGE ( 'NONE', *, *, #31753, .T. ) ;
#24648=FACE_OUTER_BOUND ( 'NONE', #4511, .T. ) ;
#24649=CARTESIAN_POINT ( 'NONE',  ( 75.17589904515345722, -175.3837268820161057, -18.28755301364250485 ) ) ;
#24650=ORIENTED_EDGE ( 'NONE', *, *, #36657, .F. ) ;
#24651=VERTEX_POINT ( 'NONE', #46121 ) ;
#24652=EDGE_CURVE ( 'NONE', #32761, #26723, #3769, .T. ) ;
#24654=ORIENTED_EDGE ( 'NONE', *, *, #41015, .T. ) ;
#24655=CARTESIAN_POINT ( 'NONE',  ( -160.4991136281923616, -175.3837268820161057, 53.17445600718625798 ) ) ;
#24657=VERTEX_POINT ( 'NONE', #10100 ) ;
#24660=DIRECTION ( 'NONE',  ( -0.9473263538541923934, 0.000000000000000000, 0.3202698538628350744 ) ) ;
#24664=ORIENTED_EDGE ( 'NONE', *, *, #49091, .F. ) ;
#24665=AXIS2_PLACEMENT_3D ( 'NONE', #27766, #3602, #35658 ) ;
#24668=CARTESIAN_POINT ( 'NONE',  ( -48.24424070572786860, -193.5000000000000000, -0.9720229140804037549 ) ) ;
#24670=PLANE ( 'NONE',  #3138 ) ;
#24672=CARTESIAN_POINT ( 'NONE',  ( -48.47912675150885065, -177.1207230881787780, 6.938893903907228378E-15 ) ) ;
#24673=PRODUCT_CONTEXT ( 'NONE', #6200, 'mechanical' ) ;
#24674=DIRECTION ( 'NONE',  ( 0.000000000000000000, -1.000000000000000000, -0.000000000000000000 ) ) ;
#24675=AXIS2_PLACEMENT_3D ( 'NONE', #2147, #34219, #17688 ) ;
#24677=EDGE_CURVE ( 'NONE', #14215, #7533, #13272, .T. ) ;
#24679=PLANE ( 'NONE',  #15384 ) ;
#24680=VERTEX_POINT ( 'NONE', #45597 ) ;
#24681=ORIENTED_EDGE ( 'NONE', *, *, #18548, .F. ) ;
#24682=DIRECTION ( 'NONE',  ( -0.000000000000000000, 1.000000000000000000, -0.000000000000000000 ) ) ;
#24684=DIRECTION ( 'NONE',  ( -0.000000000000000000, 1.000000000000000000, 0.000000000000000000 ) ) ;
#24685=ORIENTED_EDGE ( 'NONE', *, *, #37879, .F. ) ;
#24686=ORIENTED_EDGE ( 'NONE', *, *, #14086, .F. ) ;
#24690=DIRECTION ( 'NONE',  ( 0.6965510290629982615, 0.000000000000000000, -0.7175072570443298270 ) ) ;
#24691=DIRECTION ( 'NONE',  ( -0.4031234292879730674, 0.000000000000000000, 0.9151456172430181280 ) ) ;
#24692=CARTESIAN_POINT ( 'NONE',  ( -48.47912675150885065, -189.7472609257535510, 6.938893903907228378E-15 ) ) ;
#24695=AXIS2_PLACEMENT_3D ( 'NONE', #13104, #21515, #16546 ) ;
#24697=EDGE_CURVE ( 'NONE', #27708, #23768, #45344, .T. ) ;
#24698=ADVANCED_FACE ( 'NONE', ( #22454 ), #17992, .F. ) ;
#24700=EDGE_CURVE ( 'NONE', #26506, #24824, #22185, .T. ) ;
#24701=CARTESIAN_POINT ( 'NONE',  ( -66.64622755927948106, -177.1207230881787780, 123.6727797384707372 ) ) ;
#24703=AXIS2_PLACEMENT_3D ( 'NONE', #24036, #12459, #28478 ) ;
#24705=DIRECTION ( 'NONE',  ( -0.000000000000000000, 1.000000000000000000, -0.000000000000000000 ) ) ;
#24708=EDGE_CURVE ( 'NONE', #26407, #47996, #18075, .T. ) ;
#24709=EDGE_CURVE ( 'NONE', #16046, #24680, #7155, .T. ) ;
#24710=DIRECTION ( 'NONE',  ( 0.2920567706369833760, 0.000000000000000000, -0.9564009842765202052 ) ) ;
#24712=CIRCLE ( 'NONE', #43993, 125.0000000000000000 ) ;
#24716=DIRECTION ( 'NONE',  ( -0.7175072570443395970, 0.000000000000000000, 0.6965510290629882695 ) ) ;
#24718=DIRECTION ( 'NONE',  ( 0.000000000000000000, -1.000000000000000000, -0.000000000000000000 ) ) ;
#24720=EDGE_CURVE ( 'NONE', #34028, #32675, #30849, .T. ) ;
#24723=FACE_OUTER_BOUND ( 'NONE', #15972, .T. ) ;
#24725=ORIENTED_EDGE ( 'NONE', *, *, #17657, .F. ) ;
#24726=EDGE_CURVE ( 'NONE', #21902, #50633, #18760, .T. ) ;
#24727=CARTESIAN_POINT ( 'NONE',  ( -170.9669310976187830, -175.3837268820161057, -24.93467037017130394 ) ) ;
#24729=CARTESIAN_POINT ( 'NONE',  ( 45.36094686508022988, -177.1207230881787780, -82.57748230379237953 ) ) ;
#24730=ORIENTED_EDGE ( 'NONE', *, *, #24628, .T. ) ;
#24731=EDGE_CURVE ( 'NONE', #8921, #8740, #3256, .T. ) ;
#24732=PLANE ( 'NONE',  #44142 ) ;
#24733=CARTESIAN_POINT ( 'NONE',  ( -48.47912675150885065, -175.3837268820161057, 6.938893903907228378E-15 ) ) ;
#24734=CARTESIAN_POINT ( 'NONE',  ( -47.49008656418669005, -177.1207230881787780, 0.1476465640024920423 ) ) ;
#24735=ORIENTED_EDGE ( 'NONE', *, *, #4474, .T. ) ;
#24736=CARTESIAN_POINT ( 'NONE',  ( -137.2624501260119985, -193.5000000000000000, 87.99159897727967916 ) ) ;
#24737=CARTESIAN_POINT ( 'NONE',  ( -37.14819544345410662, -193.5000000000000000, 123.4817304940907121 ) ) ;
#24738=VECTOR ( 'NONE', #48909, 1000.000000000000000 ) ;
#24739=CARTESIAN_POINT ( 'NONE',  ( 59.70893145360470555, -189.7472609257535510, -60.59166255800331413 ) ) ;
#24741=ORIENTED_EDGE ( 'NONE', *, *, #5725, .F. ) ;
#24743=VECTOR ( 'NONE', #35279, 1000.000000000000000 ) ;
#24744=EDGE_CURVE ( 'NONE', #41591, #11493, #2478, .T. ) ;
#24745=ORIENTED_EDGE ( 'NONE', *, *, #10877, .T. ) ;
#24746=DIRECTION ( 'NONE',  ( -0.1182731709213730997, 0.000000000000000000, 0.9929810960135161402 ) ) ;
#24747=ORIENTED_EDGE ( 'NONE', *, *, #28284, .F. ) ;
#24748=DIRECTION ( 'NONE',  ( -0.000000000000000000, -1.000000000000000000, 0.000000000000000000 ) ) ;
#24749=PLANE ( 'NONE',  #29461 ) ;
#24750=AXIS2_PLACEMENT_3D ( 'NONE', #18397, #33639, #2366 ) ;
#24751=CARTESIAN_POINT ( 'NONE',  ( -105.4063847101409408, -189.7472609257535510, -111.2847127925096515 ) ) ;
#24752=FACE_OUTER_BOUND ( 'NONE', #51056, .T. ) ;
#24753=DIRECTION ( 'NONE',  ( -0.000000000000000000, 1.000000000000000000, -0.000000000000000000 ) ) ;
#24755=DIRECTION ( 'NONE',  ( 0.000000000000000000, 0.000000000000000000, -1.000000000000000000 ) ) ;
#24757=CARTESIAN_POINT ( 'NONE',  ( 7.859956736328458149, -175.3837268820161057, -111.5836353223468649 ) ) ;
#24759=ORIENTED_EDGE ( 'NONE', *, *, #37307, .T. ) ;
#24760=ORIENTED_EDGE ( 'NONE', *, *, #22808, .T. ) ;
#24761=ADVANCED_FACE ( 'NONE', ( #23482 ), #19290, .F. ) ;
#24762=ADVANCED_FACE ( 'NONE', ( #35296 ), #27673, .F. ) ;
#24763=DIRECTION ( 'NONE',  ( 0.1768902751225666370, 0.000000000000000000, 0.9842305779475979399 ) ) ;
#24764=ORIENTED_EDGE ( 'NONE', *, *, #12038, .T. ) ;
#24765=ORIENTED_EDGE ( 'NONE', *, *, #41486, .T. ) ;
#24768=DIRECTION ( 'NONE',  ( 0.000000000000000000, 0.000000000000000000, -1.000000000000000000 ) ) ;
#24769=VECTOR ( 'NONE', #39516, 1000.000000000000000 ) ;
#24770=VECTOR ( 'NONE', #34624, 1000.000000000000114 ) ;
#24771=CARTESIAN_POINT ( 'NONE',  ( 50.70030191143630560, -183.6283474603465606, -76.08180419845319875 ) ) ;
#24772=LINE ( 'NONE', #4279, #20742 ) ;
#24774=ORIENTED_EDGE ( 'NONE', *, *, #5625, .T. ) ;
#24775=CARTESIAN_POINT ( 'NONE',  ( 75.12566530717464275, -175.3837268820161057, 18.62405380494841722 ) ) ;
#24776=CARTESIAN_POINT ( 'NONE',  ( -56.05401443572774411, -193.5000000000000000, 124.7702732086912931 ) ) ;
#24777=LINE ( 'NONE', #12154, #15723 ) ;
#24778=ORIENTED_EDGE ( 'NONE', *, *, #5529, .T. ) ;
#24779=CIRCLE ( 'NONE', #2122, 125.0000000000000000 ) ;
#24782=AXIS2_PLACEMENT_3D ( 'NONE', #49546, #14308, #29292 ) ;
#24783=DIRECTION ( 'NONE',  ( -0.000000000000000000, 1.000000000000000000, -0.000000000000000000 ) ) ;
#24784=VERTEX_POINT ( 'NONE', #26647 ) ;
#24785=DIRECTION ( 'NONE',  ( 0.5085311186492216251, 0.000000000000000000, -0.8610436117673548884 ) ) ;
#24787=DIRECTION ( 'NONE',  ( -0.000000000000000000, 1.000000000000000000, -0.000000000000000000 ) ) ;
#24790=CYLINDRICAL_SURFACE ( 'NONE', #33272, 125.0000000000000000 ) ;
#24791=EDGE_CURVE ( 'NONE', #50432, #5269, #27146, .T. ) ;
#24792=AXIS2_PLACEMENT_3D ( 'NONE', #38607, #50457, #2084 ) ;
#24793=EDGE_LOOP ( 'NONE', ( #19982, #18700, #43178, #27627 ) ) ;
#24795=CARTESIAN_POINT ( 'NONE',  ( -48.47912675150885065, -213.5000000000000000, 6.938893903907228378E-15 ) ) ;
#24796=LINE ( 'NONE', #42113, #45201 ) ;
#24797=ORIENTED_EDGE ( 'NONE', *, *, #19915, .T. ) ;
#24798=DIRECTION ( 'NONE',  ( -0.000000000000000000, 1.000000000000000000, -0.000000000000000000 ) ) ;
#24799=CARTESIAN_POINT ( 'NONE',  ( -121.5885020763900997, -177.1207230881787780, -101.3904297239421055 ) ) ;
#24802=DIRECTION ( 'NONE',  ( -0.000000000000000000, 1.000000000000000000, -0.000000000000000000 ) ) ;
#24804=LINE ( 'NONE', #41342, #3935 ) ;
#24807=AXIS2_PLACEMENT_3D ( 'NONE', #17905, #12906, #28929 ) ;
#24808=PLANE ( 'NONE',  #22720 ) ;
#24809=EDGE_LOOP ( 'NONE', ( #26848, #36079, #11454, #43298 ) ) ;
#24810=AXIS2_PLACEMENT_3D ( 'NONE', #50281, #34736, #7150 ) ;
#24811=VECTOR ( 'NONE', #43102, 1000.000000000000000 ) ;
#24813=DIRECTION ( 'NONE',  ( 0.000000000000000000, -0.000000000000000000, -1.000000000000000000 ) ) ;
#24814=FACE_OUTER_BOUND ( 'NONE', #22741, .T. ) ;
#24815=CARTESIAN_POINT ( 'NONE',  ( -49.46816693883101834, -175.3837268820161057, 0.1476465640024780257 ) ) ;
#24816=VERTEX_POINT ( 'NONE', #42675 ) ;
#24817=CARTESIAN_POINT ( 'NONE',  ( 26.52087324849106054, -198.5000000000000000, -60.00000000000003553 ) ) ;
#24818=VERTEX_POINT ( 'NONE', #19520 ) ;
#24819=ORIENTED_EDGE ( 'NONE', *, *, #31266, .T. ) ;
#24820=DIRECTION ( 'NONE',  ( -0.000000000000000000, -1.000000000000000000, 0.000000000000000000 ) ) ;
#24821=DIRECTION ( 'NONE',  ( -0.000000000000000000, -1.000000000000000000, 0.000000000000000000 ) ) ;
#24823=VECTOR ( 'NONE', #39733, 1000.000000000000000 ) ;
#24824=VERTEX_POINT ( 'NONE', #39247 ) ;
#24825=CARTESIAN_POINT ( 'NONE',  ( -127.6327502296859535, -177.1207230881787780, -95.45105364470086329 ) ) ;
#24826=ADVANCED_FACE ( 'NONE', ( #51342 ), #11372, .T. ) ;
#24827=CIRCLE ( 'NONE', #4680, 125.0000000000000000 ) ;
#24828=AXIS2_PLACEMENT_3D ( 'NONE', #51367, #11392, #27429 ) ;
#24831=DIRECTION ( 'NONE',  ( 0.000000000000000000, -0.000000000000000000, -1.000000000000000000 ) ) ;
#24832=ORIENTED_EDGE ( 'NONE', *, *, #40338, .T. ) ;
#24833=LINE ( 'NONE', #40852, #16623 ) ;
#24834=CARTESIAN_POINT ( 'NONE',  ( -104.8182102393454045, -193.5000000000000000, 111.5836353223472912 ) ) ;
#24839=ORIENTED_EDGE ( 'NONE', *, *, #12198, .T. ) ;
#24841=CARTESIAN_POINT ( 'NONE',  ( -1.771278280434267272, -193.5000000000000000, -115.9455772817710226 ) ) ;
#24842=VECTOR ( 'NONE', #44919, 1000.000000000000114 ) ;
#24843=VECTOR ( 'NONE', #29387, 1000.000000000000000 ) ;
#24844=EDGE_CURVE ( 'NONE', #37031, #2833, #43703, .T. ) ;
#24845=CARTESIAN_POINT ( 'NONE',  ( -48.88225018079683082, -183.6283474603465606, 0.9151456172430223468 ) ) ;
#24846=VECTOR ( 'NONE', #22343, 1000.000000000000000 ) ;
#24847=CARTESIAN_POINT ( 'NONE',  ( -48.24424070572787571, -177.1207230881787780, 0.9720229140804191870 ) ) ;
#24849=EDGE_LOOP ( 'NONE', ( #10088, #38298, #39526, #31533 ) ) ;
#24850=CIRCLE ( 'NONE', #36584, 125.0000000000000000 ) ;
#24853=VERTEX_POINT ( 'NONE', #50566 ) ;
#24857=DIRECTION ( 'NONE',  ( 0.000000000000000000, -0.000000000000000000, 1.000000000000000000 ) ) ;
#24858=AXIS2_PLACEMENT_3D ( 'NONE', #20886, #9052, #37411 ) ;
#24859=AXIS2_PLACEMENT_3D ( 'NONE', #1613, #33656, #37856 ) ;
#24861=DIRECTION ( 'NONE',  ( 0.3758275821142292861, 0.000000000000000000, 0.9266896074318371479 ) ) ;
#24862=VERTEX_POINT ( 'NONE', #14568 ) ;
#24865=ORIENTED_EDGE ( 'NONE', *, *, #19258, .T. ) ;
#24866=AXIS2_PLACEMENT_3D ( 'NONE', #31140, #35340, #2765 ) ;
#24867=ORIENTED_EDGE ( 'NONE', *, *, #8849, .F. ) ;
#24869=DIRECTION ( 'NONE',  ( 0.000000000000000000, 1.000000000000000000, 0.000000000000000000 ) ) ;
#24870=LINE ( 'NONE', #15964, #39120 ) ;
#24871=LINE ( 'NONE', #42386, #51635 ) ;
#24872=ADVANCED_FACE ( 'NONE', ( #30571 ), #41241, .F. ) ;
#24874=CARTESIAN_POINT ( 'NONE',  ( -129.4514457347087273, -193.5000000000000000, 95.22858582633115532 ) ) ;
#24875=DIRECTION ( 'NONE',  ( 0.4566292373937018145, 0.000000000000000000, 0.8896570909947529859 ) ) ;
#24876=ORIENTED_EDGE ( 'NONE', *, *, #28724, .F. ) ;
#24877=CARTESIAN_POINT ( 'NONE',  ( -48.47912675150885065, -177.1207230881787780, -0.9999999999999931166 ) ) ;
#24878=DIRECTION ( 'NONE',  ( 0.000000000000000000, 0.000000000000000000, -1.000000000000000000 ) ) ;
#24881=FACE_BOUND ( 'NONE', #6439, .T. ) ;
#24882=ORIENTED_EDGE ( 'NONE', *, *, #25578, .F. ) ;
#24885=CARTESIAN_POINT ( 'NONE',  ( -47.74129347246713451, -193.5000000000000000, 0.6749830015182212151 ) ) ;
#24886=ORIENTED_EDGE ( 'NONE', *, *, #9165, .F. ) ;
#24891=EDGE_CURVE ( 'NONE', #44141, #49533, #20619, .T. ) ;
#24893=EDGE_CURVE ( 'NONE', #29042, #22971, #41500, .T. ) ;
#24894=CARTESIAN_POINT ( 'NONE',  ( -55.71438232577009586, -175.3837268820161057, -124.7904286264580804 ) ) ;
#24897=FACE_BOUND ( 'NONE', #45243, .T. ) ;
#24899=CARTESIAN_POINT ( 'NONE',  ( 29.27398957514434130, -193.5000000000000000, -97.87467957287998388 ) ) ;
#24900=VERTEX_POINT ( 'NONE', #36521 ) ;
#24903=AXIS2_PLACEMENT_3D ( 'NONE', #40041, #11926, #38820 ) ;
#24904=AXIS2_PLACEMENT_3D ( 'NONE', #35109, #51940, #11711 ) ;
#24906=VERTEX_POINT ( 'NONE', #28634 ) ;
#24907=ORIENTED_EDGE ( 'NONE', *, *, #38092, .T. ) ;
#24910=LINE ( 'NONE', #4166, #51961 ) ;
#24911=DIRECTION ( 'NONE',  ( -0.000000000000000000, 1.000000000000000000, -0.000000000000000000 ) ) ;
#24913=EDGE_CURVE ( 'NONE', #43506, #49860, #37577, .T. ) ;
#24915=LINE ( 'NONE', #32792, #32212 ) ;
#24916=CARTESIAN_POINT ( 'NONE',  ( -172.2289551866394106, -193.5000000000000000, -17.63462396184707970 ) ) ;
#24918=ORIENTED_EDGE ( 'NONE', *, *, #31716, .F. ) ;
#24920=CARTESIAN_POINT ( 'NONE',  ( 73.66680038934278230, -175.3837268820161057, -26.55884942729568721 ) ) ;
#24923=ORIENTED_EDGE ( 'NONE', *, *, #39358, .F. ) ;
#24924=VECTOR ( 'NONE', #24753, 1000.000000000000000 ) ;
#24926=ORIENTED_EDGE ( 'NONE', *, *, #22631, .T. ) ;
#24929=VECTOR ( 'NONE', #34514, 1000.000000000000000 ) ;
#24931=DIRECTION ( 'NONE',  ( 0.000000000000000000, 0.000000000000000000, -1.000000000000000000 ) ) ;
#24932=VERTEX_POINT ( 'NONE', #32590 ) ;
#24936=DIRECTION ( 'NONE',  ( -0.3202698538628487301, 0.000000000000000000, 0.9473263538541877304 ) ) ;
#24937=AXIS2_PLACEMENT_3D ( 'NONE', #1966, #41385, #36935 ) ;
#24938=CYLINDRICAL_SURFACE ( 'NONE', #12140, 125.0000000000000000 ) ;
#24941=LINE ( 'NONE', #28862, #26667 ) ;
#24942=VERTEX_POINT ( 'NONE', #17361 ) ;
#24944=VECTOR ( 'NONE', #46601, 1000.000000000000000 ) ;
#24949=DIRECTION ( 'NONE',  ( 0.8455960035018199594, 0.000000000000000000, 0.5338233779648003940 ) ) ;
#24950=VECTOR ( 'NONE', #28660, 1000.000000000000000 ) ;
#24951=DIRECTION ( 'NONE',  ( -0.000000000000000000, 1.000000000000000000, -0.000000000000000000 ) ) ;
#24955=VERTEX_POINT ( 'NONE', #20768 ) ;
#24956=LINE ( 'NONE', #16822, #39087 ) ;
#24957=CARTESIAN_POINT ( 'NONE',  ( 14.94072793302542124, -175.3837268820161057, 107.7168604805791574 ) ) ;
#24960=ORIENTED_EDGE ( 'NONE', *, *, #6510, .F. ) ;
#24961=ADVANCED_FACE ( 'NONE', ( #28893 ), #48640, .T. ) ;
#24963=EDGE_CURVE ( 'NONE', #50756, #15492, #13655, .T. ) ;
#24964=AXIS2_PLACEMENT_3D ( 'NONE', #10126, #20929, #41652 ) ;
#24965=FACE_OUTER_BOUND ( 'NONE', #44405, .T. ) ;
#24967=EDGE_CURVE ( 'NONE', #8712, #2850, #29675, .T. ) ;
#24968=DIRECTION ( 'NONE',  ( 0.000000000000000000, -0.000000000000000000, -1.000000000000000000 ) ) ;
#24970=CARTESIAN_POINT ( 'NONE',  ( -92.16375985330356002, -175.3837268820161057, 117.1181148702521710 ) ) ;
#24971=VECTOR ( 'NONE', #7520, 1000.000000000000000 ) ;
#24972=ADVANCED_FACE ( 'NONE', ( #8939 ), #49424, .F. ) ;
#24975=PLANE ( 'NONE',  #36085 ) ;
#24976=VERTEX_POINT ( 'NONE', #13402 ) ;
#24978=ORIENTED_EDGE ( 'NONE', *, *, #29995, .F. ) ;
#24979=CARTESIAN_POINT ( 'NONE',  ( 49.88781503343063406, -177.1207230881787780, -75.49882471933871386 ) ) ;
#24981=VECTOR ( 'NONE', #2087, 1000.000000000000000 ) ;
#24983=CARTESIAN_POINT ( 'NONE',  ( -171.9740864388383557, -193.5000000000000000, -11.18012358327899314 ) ) ;
#24985=AXIS2_PLACEMENT_3D ( 'NONE', #6324, #49955, #2108 ) ;
#24986=AXIS2_PLACEMENT_3D ( 'NONE', #3972, #40469, #43653 ) ;
#24987=DIRECTION ( 'NONE',  ( -0.000000000000000000, -1.000000000000000000, 0.000000000000000000 ) ) ;
#24988=DIRECTION ( 'NONE',  ( 0.000000000000000000, 0.000000000000000000, 1.000000000000000000 ) ) ;
#24989=DIRECTION ( 'NONE',  ( 0.000000000000000000, -1.000000000000000000, 0.000000000000000000 ) ) ;
#24991=VERTEX_POINT ( 'NONE', #36799 ) ;
#24993=ORIENTED_EDGE ( 'NONE', *, *, #36269, .T. ) ;
#24994=DIRECTION ( 'NONE',  ( 0.000000000000000000, 0.000000000000000000, 1.000000000000000000 ) ) ;
#24995=DIRECTION ( 'NONE',  ( -0.000000000000000000, 1.000000000000000000, -0.000000000000000000 ) ) ;
#24999=DIRECTION ( 'NONE',  ( -0.000000000000000000, 1.000000000000000000, -0.000000000000000000 ) ) ;
#25001=EDGE_CURVE ( 'NONE', #43983, #30132, #25228, .T. ) ;
#25003=AXIS2_PLACEMENT_3D ( 'NONE', #22730, #15367, #35074 ) ;
#25005=VECTOR ( 'NONE', #757, 1000.000000000000000 ) ;
#25006=CARTESIAN_POINT ( 'NONE',  ( -106.2948367055609964, -189.7472609257535510, -110.8257356506552327 ) ) ;
#25007=ORIENTED_EDGE ( 'NONE', *, *, #20220, .F. ) ;
#25009=DIRECTION ( 'NONE',  ( -0.000000000000000000, 1.000000000000000000, -0.000000000000000000 ) ) ;
#25010=AXIS2_PLACEMENT_3D ( 'NONE', #30574, #19027, #15340 ) ;
#25012=EDGE_CURVE ( 'NONE', #45883, #37758, #8673, .T. ) ;
#25015=EDGE_CURVE ( 'NONE', #24991, #3996, #25482, .T. ) ;
#25017=EDGE_CURVE ( 'NONE', #33038, #23726, #46247, .T. ) ;
#25018=DIRECTION ( 'NONE',  ( 0.000000000000000000, -1.000000000000000000, 0.000000000000000000 ) ) ;
#25019=ORIENTED_EDGE ( 'NONE', *, *, #23676, .T. ) ;
#25020=VECTOR ( 'NONE', #5134, 1000.000000000000000 ) ;
#25023=PLANE ( 'NONE',  #24438 ) ;
#25024=LINE ( 'NONE', #12913, #15157 ) ;
#25025=DIRECTION ( 'NONE',  ( 0.000000000000000000, 1.000000000000000000, 0.000000000000000000 ) ) ;
#25031=ADVANCED_FACE ( 'NONE', ( #34405 ), #42801, .T. ) ;
#25032=DIRECTION ( 'NONE',  ( 0.000000000000000000, 0.000000000000000000, 1.000000000000000000 ) ) ;
#25033=DIRECTION ( 'NONE',  ( 0.000000000000000000, 0.000000000000000000, 1.000000000000000000 ) ) ;
#25037=ORIENTED_EDGE ( 'NONE', *, *, #35090, .T. ) ;
#25039=ADVANCED_FACE ( 'NONE', ( #1822 ), #30206, .T. ) ;
#25040=CARTESIAN_POINT ( 'NONE',  ( 73.32083127613157103, -177.1207230881787780, 28.10285082451656535 ) ) ;
#25042=AXIS2_PLACEMENT_3D ( 'NONE', #32490, #20142, #8563 ) ;
#25044=VECTOR ( 'NONE', #44434, 1000.000000000000000 ) ;
#25045=VERTEX_POINT ( 'NONE', #30450 ) ;
#25048=CARTESIAN_POINT ( 'NONE',  ( 47.04848625005566731, -193.5000000000000000, 80.61932246194658092 ) ) ;
#25049=DIRECTION ( 'NONE',  ( 0.000000000000000000, 0.000000000000000000, -1.000000000000000000 ) ) ;
#25050=ORIENTED_EDGE ( 'NONE', *, *, #35315, .F. ) ;
#25051=ORIENTED_EDGE ( 'NONE', *, *, #42064, .F. ) ;
#25052=ADVANCED_FACE ( 'NONE', ( #42023 ), #46758, .T. ) ;
#25053=DIRECTION ( 'NONE',  ( 0.000000000000000000, -1.000000000000000000, 0.000000000000000000 ) ) ;
#25054=AXIS2_PLACEMENT_3D ( 'NONE', #45469, #17621, #41502 ) ;
#25055=CARTESIAN_POINT ( 'NONE',  ( 59.80284513346456521, -193.5000000000000000, 62.45009659481583952 ) ) ;
#25056=ORIENTED_EDGE ( 'NONE', *, *, #28313, .F. ) ;
#25057=DIRECTION ( 'NONE',  ( 0.000000000000000000, 0.000000000000000000, 1.000000000000000000 ) ) ;
#25060=VERTEX_POINT ( 'NONE', #38075 ) ;
#25061=CARTESIAN_POINT ( 'NONE',  ( -171.5708553757489767, -177.1207230881787780, 14.98512977653257039 ) ) ;
#25062=CARTESIAN_POINT ( 'NONE',  ( -168.1386673294336163, -193.5000000000000000, 32.52067927015838933 ) ) ;
#25063=DIRECTION ( 'NONE',  ( -0.7378332790417189146, 0.000000000000000000, -0.6749830015182196608 ) ) ;
#25064=VECTOR ( 'NONE', #36757, 1000.000000000000000 ) ;
#25066=ORIENTED_EDGE ( 'NONE', *, *, #47130, .T. ) ;
#25068=CARTESIAN_POINT ( 'NONE',  ( 2.066935079424590871, -189.7472609257535510, -114.3245189510257660 ) ) ;
#25069=ORIENTED_EDGE ( 'NONE', *, *, #43111, .T. ) ;
#25070=DIRECTION ( 'NONE',  ( 0.000000000000000000, -1.000000000000000000, 0.000000000000000000 ) ) ;
#25071=DIRECTION ( 'NONE',  ( 0.1768902751225802927, 0.000000000000000000, -0.9842305779475953864 ) ) ;
#25074=EDGE_LOOP ( 'NONE', ( #5024, #28207, #1233, #30931 ) ) ;
#25076=DIRECTION ( 'NONE',  ( -0.000000000000000000, 1.000000000000000000, -0.000000000000000000 ) ) ;
#25077=EDGE_CURVE ( 'NONE', #18623, #43059, #18386, .T. ) ;
#25079=ORIENTED_EDGE ( 'NONE', *, *, #43283, .T. ) ;
#25080=CARTESIAN_POINT ( 'NONE',  ( -123.4791267515088435, -198.5000000000000000, 60.00000000000001421 ) ) ;
#25081=ORIENTED_EDGE ( 'NONE', *, *, #19149, .T. ) ;
#25083=CARTESIAN_POINT ( 'NONE',  ( -102.9981419485577590, -177.1207230881787780, -111.3726929437936377 ) ) ;
#25084=VECTOR ( 'NONE', #32794, 1000.000000000000000 ) ;
#25086=ORIENTED_EDGE ( 'NONE', *, *, #35871, .F. ) ;
#25087=AXIS2_PLACEMENT_3D ( 'NONE', #8100, #43829, #48306 ) ;
#25089=CARTESIAN_POINT ( 'NONE',  ( -48.47912675150885065, -177.1207230881787780, 6.938893903907228378E-15 ) ) ;
#25090=CARTESIAN_POINT ( 'NONE',  ( -49.35486169370449971, -193.5000000000000000, 0.4827922027307437469 ) ) ;
#25091=DIRECTION ( 'NONE',  ( -0.9960498426152165630, 0.000000000000000000, -0.08879589532293852283 ) ) ;
#25092=VERTEX_POINT ( 'NONE', #50696 ) ;
#25093=DIRECTION ( 'NONE',  ( 0.000000000000000000, -0.000000000000000000, -1.000000000000000000 ) ) ;
#25095=EDGE_LOOP ( 'NONE', ( #24359, #6540, #41501, #51012 ) ) ;
#25096=CIRCLE ( 'NONE', #26726, 125.0000000000000000 ) ;
#25097=EDGE_CURVE ( 'NONE', #42695, #45794, #25746, .T. ) ;
#25098=LINE ( 'NONE', #20896, #11004 ) ;
#25100=EDGE_LOOP ( 'NONE', ( #7671, #1480, #24210, #51475 ) ) ;
#25104=VECTOR ( 'NONE', #35133, 1000.000000000000000 ) ;
#25105=CARTESIAN_POINT ( 'NONE',  ( -172.1341525481709880, -193.5000000000000000, 18.28755301364337527 ) ) ;
#25107=ORIENTED_EDGE ( 'NONE', *, *, #36426, .T. ) ;
#25108=FACE_OUTER_BOUND ( 'NONE', #31243, .T. ) ;
#25109=EDGE_LOOP ( 'NONE', ( #6560, #30328, #16566, #48602 ) ) ;
#25111=CARTESIAN_POINT ( 'NONE',  ( -158.6498865914718408, -177.1207230881787780, 56.90809649257572289 ) ) ;
#25115=ORIENTED_EDGE ( 'NONE', *, *, #1594, .F. ) ;
#25116=VERTEX_POINT ( 'NONE', #20667 ) ;
#25117=LINE ( 'NONE', #1176, #45918 ) ;
#25118=DIRECTION ( 'NONE',  ( 0.9960498426152158968, 0.000000000000000000, 0.08879589532294571153 ) ) ;
#25122=CARTESIAN_POINT ( 'NONE',  ( -58.17235712592530206, -193.5000000000000000, 123.6213615703899649 ) ) ;
#25123=ORIENTED_EDGE ( 'NONE', *, *, #15077, .F. ) ;
#25124=AXIS2_PLACEMENT_3D ( 'NONE', #11968, #28001, #40092 ) ;
#25125=ORIENTED_EDGE ( 'NONE', *, *, #43507, .T. ) ;
#25126=CARTESIAN_POINT ( 'NONE',  ( -47.87232660569026166, -175.3837268820161057, 0.7948544414133635883 ) ) ;
#25127=VERTEX_POINT ( 'NONE', #33277 ) ;
#25128=EDGE_LOOP ( 'NONE', ( #12344, #25219, #25810, #35481 ) ) ;
#25129=CARTESIAN_POINT ( 'NONE',  ( -48.47912675150885065, -177.1207230881787780, 6.938893903907228378E-15 ) ) ;
#25131=CARTESIAN_POINT ( 'NONE',  ( -213.8817838414232426, -213.5000000000000000, -10.00000000000000000 ) ) ;
#25135=ORIENTED_EDGE ( 'NONE', *, *, #3906, .T. ) ;
#25136=CARTESIAN_POINT ( 'NONE',  ( -137.9639882952644143, -177.1207230881787780, 87.27805883780241913 ) ) ;
#25137=EDGE_LOOP ( 'NONE', ( #11434, #4021, #14140, #24101 ) ) ;
#25138=AXIS2_PLACEMENT_3D ( 'NONE', #1615, #29710, #45754 ) ;
#25141=CARTESIAN_POINT ( 'NONE',  ( -47.92047998570520662, -189.7472609257535510, 0.8294056854502119824 ) ) ;
#25144=LINE ( 'NONE', #41158, #50580 ) ;
#25145=ORIENTED_EDGE ( 'NONE', *, *, #21819, .F. ) ;
#25146=FACE_OUTER_BOUND ( 'NONE', #5303, .T. ) ;
#25147=DIRECTION ( 'NONE',  ( -0.7575112421616191360, 0.000000000000000000, -0.6528221181905227155 ) ) ;
#25150=FACE_BOUND ( 'NONE', #40873, .T. ) ;
#25152=CIRCLE ( 'NONE', #2490, 125.0000000000000000 ) ;
#25153=EDGE_CURVE ( 'NONE', #48128, #27213, #2158, .T. ) ;
#25155=VERTEX_POINT ( 'NONE', #28798 ) ;
#25156=AXIS2_PLACEMENT_3D ( 'NONE', #2667, #42351, #47086 ) ;
#25159=CARTESIAN_POINT ( 'NONE',  ( -33.52607327456454556, -193.5000000000000000, -124.1024020384603119 ) ) ;
#25160=EDGE_LOOP ( 'NONE', ( #40302, #37999, #47234, #39820 ) ) ;
#25161=CARTESIAN_POINT ( 'NONE',  ( 74.60098876342244978, -183.6283474603465606, 21.82395850507348811 ) ) ;
#25162=DIRECTION ( 'NONE',  ( 0.000000000000000000, -1.000000000000000000, 0.000000000000000000 ) ) ;
#25164=ORIENTED_EDGE ( 'NONE', *, *, #6396, .F. ) ;
#25165=EDGE_CURVE ( 'NONE', #26145, #38032, #41414, .T. ) ;
#25166=CARTESIAN_POINT ( 'NONE',  ( -48.47912675150885065, -189.7472609257535510, 6.938893903907228378E-15 ) ) ;
#25168=VERTEX_POINT ( 'NONE', #33789 ) ;
#25170=ORIENTED_EDGE ( 'NONE', *, *, #7891, .T. ) ;
#25172=CARTESIAN_POINT ( 'NONE',  ( -41.96187976958283627, -189.7472609257535510, -123.8286356280830205 ) ) ;
#25178=EDGE_CURVE ( 'NONE', #50890, #42195, #45639, .T. ) ;
#25179=CYLINDRICAL_SURFACE ( 'NONE', #45234, 125.0000000000000000 ) ;
#25180=LINE ( 'NONE', #32795, #17266 ) ;
#25182=DIRECTION ( 'NONE',  ( 0.9646355819083594074, 0.000000000000000000, -0.2635871660690647933 ) ) ;
#25183=CARTESIAN_POINT ( 'NONE',  ( -48.47912675150885065, -183.6283474603465606, 6.938893903907228378E-15 ) ) ;
#25185=VERTEX_POINT ( 'NONE', #48799 ) ;
#25186=VECTOR ( 'NONE', #44946, 1000.000000000000000 ) ;
#25190=VERTEX_POINT ( 'NONE', #49321 ) ;
#25192=EDGE_CURVE ( 'NONE', #42748, #16426, #37477, .T. ) ;
#25193=CARTESIAN_POINT ( 'NONE',  ( -48.47912675150885065, -177.1207230881787780, 6.938893903907228378E-15 ) ) ;
#25195=DIRECTION ( 'NONE',  ( 0.000000000000000000, -1.000000000000000000, 0.000000000000000000 ) ) ;
#25197=ORIENTED_EDGE ( 'NONE', *, *, #9938, .T. ) ;
#25198=CARTESIAN_POINT ( 'NONE',  ( -33.98218805075477178, -175.3837268820161057, 123.1496609813405314 ) ) ;
#25199=ADVANCED_FACE ( 'NONE', ( #33542 ), #13035, .T. ) ;
#25201=CARTESIAN_POINT ( 'NONE',  ( -36.15208382588832592, -193.5000000000000000, 123.3865623328509287 ) ) ;
#25212=DIRECTION ( 'NONE',  ( 0.000000000000000000, 0.000000000000000000, -1.000000000000000000 ) ) ;
#25213=ORIENTED_EDGE ( 'NONE', *, *, #33972, .F. ) ;
#25214=ADVANCED_FACE ( 'NONE', ( #8835 ), #37214, .T. ) ;
#25217=ORIENTED_EDGE ( 'NONE', *, *, #19261, .F. ) ;
#25219=ORIENTED_EDGE ( 'NONE', *, *, #5069, .F. ) ;
#25222=DIRECTION ( 'NONE',  ( 0.000000000000000000, 1.000000000000000000, 0.000000000000000000 ) ) ;
#25223=CARTESIAN_POINT ( 'NONE',  ( -95.18697522258266019, -177.1207230881787780, 115.9455772817713353 ) ) ;
#25224=CARTESIAN_POINT ( 'NONE',  ( -173.4291566779743050, -189.7472609257535510, 3.534122433558314125 ) ) ;
#25225=EDGE_LOOP ( 'NONE', ( #25654, #7889, #16376, #44639 ) ) ;
#25228=LINE ( 'NONE', #29415, #25640 ) ;
#25232=LINE ( 'NONE', #8676, #39287 ) ;
#25234=EDGE_CURVE ( 'NONE', #21107, #10986, #41675, .T. ) ;
#25235=VECTOR ( 'NONE', #42097, 1000.000000000000114 ) ;
#25236=CIRCLE ( 'NONE', #1751, 124.9999999999999858 ) ;
#25237=DIRECTION ( 'NONE',  ( -0.000000000000000000, 1.000000000000000000, -0.000000000000000000 ) ) ;
#25239=ORIENTED_EDGE ( 'NONE', *, *, #26626, .T. ) ;
#25241=DIRECTION ( 'NONE',  ( 0.000000000000000000, 0.000000000000000000, -1.000000000000000000 ) ) ;
#25244=ORIENTED_EDGE ( 'NONE', *, *, #30055, .T. ) ;
#25245=DIRECTION ( 'NONE',  ( 0.000000000000000000, 1.000000000000000000, -0.000000000000000000 ) ) ;
#25246=DIRECTION ( 'NONE',  ( -0.000000000000000000, -1.000000000000000000, 0.000000000000000000 ) ) ;
#25248=EDGE_CURVE ( 'NONE', #22157, #8359, #41935, .T. ) ;
#25249=CARTESIAN_POINT ( 'NONE',  ( -48.47912675150885065, -177.1207230881787780, 6.938893903907228378E-15 ) ) ;
#25252=ORIENTED_EDGE ( 'NONE', *, *, #26254, .T. ) ;
#25254=EDGE_CURVE ( 'NONE', #47106, #43249, #27327, .T. ) ;
#25255=CARTESIAN_POINT ( 'NONE',  ( -169.9131040279660283, -177.1207230881787780, 29.64437826672835996 ) ) ;
#25256=FACE_BOUND ( 'NONE', #47993, .T. ) ;
#25258=DIRECTION ( 'NONE',  ( -0.2920567706369628924, 0.000000000000000000, -0.9564009842765264224 ) ) ;
#25260=VERTEX_POINT ( 'NONE', #33008 ) ;
#25261=DIRECTION ( 'NONE',  ( 0.000000000000000000, 0.000000000000000000, 1.000000000000000000 ) ) ;
#25263=CARTESIAN_POINT ( 'NONE',  ( 21.21056010634072564, -193.5000000000000000, 103.7706487676302061 ) ) ;
#25264=CARTESIAN_POINT ( 'NONE',  ( -85.77912150413021664, -193.5000000000000000, -119.3051146910911768 ) ) ;
#25265=EDGE_CURVE ( 'NONE', #21281, #11883, #21718, .T. ) ;
#25266=EDGE_LOOP ( 'NONE', ( #31300, #48364, #17716, #25079 ) ) ;
#25267=PLANE ( 'NONE',  #19594 ) ;
#25269=DIRECTION ( 'NONE',  ( 0.000000000000000000, 0.000000000000000000, 1.000000000000000000 ) ) ;
#25270=ORIENTED_EDGE ( 'NONE', *, *, #30466, .T. ) ;
#25271=LINE ( 'NONE', #13189, #2142 ) ;
#25272=FACE_OUTER_BOUND ( 'NONE', #35685, .T. ) ;
#25274=DIRECTION ( 'NONE',  ( 0.000000000000000000, 1.000000000000000000, 0.000000000000000000 ) ) ;
#25276=AXIS2_PLACEMENT_3D ( 'NONE', #50680, #29401, #9442 ) ;
#25277=DIRECTION ( 'NONE',  ( -0.000000000000000000, -1.000000000000000000, 0.000000000000000000 ) ) ;
#25278=DIRECTION ( 'NONE',  ( 0.000000000000000000, 0.000000000000000000, 1.000000000000000000 ) ) ;
#25280=DIRECTION ( 'NONE',  ( -0.000000000000000000, 1.000000000000000000, 0.000000000000000000 ) ) ;
#25281=ORIENTED_EDGE ( 'NONE', *, *, #5444, .T. ) ;
#25282=ORIENTED_EDGE ( 'NONE', *, *, #29540, .F. ) ;
#25283=LINE ( 'NONE', #16888, #10668 ) ;
#25284=CARTESIAN_POINT ( 'NONE',  ( 141.7825277784304205, -193.5000000000000000, 41.45482488023466772 ) ) ;
#25285=DIRECTION ( 'NONE',  ( -0.000000000000000000, 1.000000000000000000, -0.000000000000000000 ) ) ;
#25286=VERTEX_POINT ( 'NONE', #1735 ) ;
#25288=VECTOR ( 'NONE', #42928, 999.9999999999998863 ) ;
#25290=DIRECTION ( 'NONE',  ( 0.000000000000000000, 0.000000000000000000, 1.000000000000000000 ) ) ;
#25291=ADVANCED_FACE ( 'NONE', ( #34809 ), #10390, .T. ) ;
#25292=EDGE_CURVE ( 'NONE', #49664, #3078, #6206, .T. ) ;
#25293=ADVANCED_FACE ( 'NONE', ( #26414 ), #1990, .T. ) ;
#25294=CARTESIAN_POINT ( 'NONE',  ( 38.71172987070723792, -189.7472609257535510, -89.56983042009264295 ) ) ;
#25296=ADVANCED_FACE ( 'NONE', ( #46664 ), #3022, .T. ) ;
#25297=PLANE ( 'NONE',  #7570 ) ;
#25298=DIRECTION ( 'NONE',  ( 0.4827922027307490205, 0.000000000000000000, -0.8757349421956345248 ) ) ;
#25299=ORIENTED_EDGE ( 'NONE', *, *, #24409, .F. ) ;
#25301=EDGE_CURVE ( 'NONE', #51223, #20567, #27184, .T. ) ;
#25303=VERTEX_POINT ( 'NONE', #19066 ) ;
#25304=DIRECTION ( 'NONE',  ( -0.000000000000000000, 1.000000000000000000, 0.000000000000000000 ) ) ;
#25306=ORIENTED_EDGE ( 'NONE', *, *, #34338, .T. ) ;
#25307=PLANE ( 'NONE',  #46744 ) ;
#25308=ADVANCED_FACE ( 'NONE', ( #2763 ), #42722, .T. ) ;
#25309=CARTESIAN_POINT ( 'NONE',  ( -135.4258661347518284, -189.7472609257535510, -89.80681772907011862 ) ) ;
#25312=EDGE_CURVE ( 'NONE', #24349, #17499, #6474, .T. ) ;
#25313=AXIS2_PLACEMENT_3D ( 'NONE', #29725, #33155, #49720 ) ;
#25314=ORIENTED_EDGE ( 'NONE', *, *, #5633, .F. ) ;
#25315=ORIENTED_EDGE ( 'NONE', *, *, #22993, .T. ) ;
#25316=PLANE ( 'NONE',  #9698 ) ;
#25317=ADVANCED_FACE ( 'NONE', ( #14877 ), #34313, .T. ) ;
#25322=ORIENTED_EDGE ( 'NONE', *, *, #23427, .T. ) ;
#25324=AXIS2_PLACEMENT_3D ( 'NONE', #47585, #43624, #23644 ) ;
#25327=CARTESIAN_POINT ( 'NONE',  ( -171.7300019102062265, -177.1207230881787780, -20.83798868929513759 ) ) ;
#25328=VERTEX_POINT ( 'NONE', #46159 ) ;
#25329=PLANE ( 'NONE',  #25407 ) ;
#25330=CARTESIAN_POINT ( 'NONE',  ( -127.0132498732365889, -177.1207230881787780, 97.24912084693261249 ) ) ;
#25332=FACE_OUTER_BOUND ( 'NONE', #13793, .T. ) ;
#25336=EDGE_CURVE ( 'NONE', #13870, #14725, #22222, .T. ) ;
#25337=VERTEX_POINT ( 'NONE', #14603 ) ;
#25338=CARTESIAN_POINT ( 'NONE',  ( -48.47912675150885065, -177.1207230881787780, 6.938893903907228378E-15 ) ) ;
#25339=ORIENTED_EDGE ( 'NONE', *, *, #28306, .T. ) ;
#25341=DIRECTION ( 'NONE',  ( -0.000000000000000000, 1.000000000000000000, 0.000000000000000000 ) ) ;
#25343=ORIENTED_EDGE ( 'NONE', *, *, #11810, .T. ) ;
#25344=VECTOR ( 'NONE', #5119, 1000.000000000000000 ) ;
#25345=ORIENTED_EDGE ( 'NONE', *, *, #18533, .T. ) ;
#25347=AXIS2_PLACEMENT_3D ( 'NONE', #42959, #31387, #51632 ) ;
#25348=VECTOR ( 'NONE', #5848, 1000.000000000000114 ) ;
#25349=EDGE_CURVE ( 'NONE', #29823, #25483, #14347, .T. ) ;
#25350=FACE_OUTER_BOUND ( 'NONE', #30433, .T. ) ;
#25351=VERTEX_POINT ( 'NONE', #30359 ) ;
#25352=DIRECTION ( 'NONE',  ( 0.000000000000000000, 0.000000000000000000, 1.000000000000000000 ) ) ;
#25354=PLANE ( 'NONE',  #43469 ) ;
#25355=DIRECTION ( 'NONE',  ( -0.000000000000000000, -1.000000000000000000, 0.000000000000000000 ) ) ;
#25356=EDGE_CURVE ( 'NONE', #22201, #50750, #38515, .T. ) ;
#25357=ADVANCED_FACE ( 'NONE', ( #15132 ), #26689, .T. ) ;
#25358=ADVANCED_FACE ( 'NONE', ( #47183 ), #23002, .F. ) ;
#25359=CARTESIAN_POINT ( 'NONE',  ( -118.9967449635792462, -193.5000000000000000, -103.2098131075562009 ) ) ;
#25362=VECTOR ( 'NONE', #35532, 1000.000000000000000 ) ;
#25363=ORIENTED_EDGE ( 'NONE', *, *, #50850, .T. ) ;
#25364=EDGE_CURVE ( 'NONE', #37475, #46340, #35587, .T. ) ;
#25365=EDGE_LOOP ( 'NONE', ( #46711, #968, #20130, #1438 ) ) ;
#25367=CARTESIAN_POINT ( 'NONE',  ( -89.73513343757494454, -177.1207230881787780, -117.9955164924467397 ) ) ;
#25368=AXIS2_PLACEMENT_3D ( 'NONE', #13379, #20740, #29390 ) ;
#25369=AXIS2_PLACEMENT_3D ( 'NONE', #7205, #14582, #31366 ) ;
#25371=LINE ( 'NONE', #41389, #13806 ) ;
#25373=PRODUCT_DEFINITION_CONTEXT ( 'detailed design', #2506, 'design' ) ;
#25376=CYLINDRICAL_SURFACE ( 'NONE', #41618, 125.0000000000000000 ) ;
#25377=ORIENTED_EDGE ( 'NONE', *, *, #39805, .T. ) ;
#25378=EDGE_LOOP ( 'NONE', ( #3486, #50684, #43817, #42840 ) ) ;
#25381=DIRECTION ( 'NONE',  ( 0.000000000000000000, 1.000000000000000000, -0.000000000000000000 ) ) ;
#25384=EDGE_CURVE ( 'NONE', #11395, #11764, #23775, .T. ) ;
#25386=LINE ( 'NONE', #37727, #51150 ) ;
#25387=VERTEX_POINT ( 'NONE', #16157 ) ;
#25388=LINE ( 'NONE', #29320, #40103 ) ;
#25389=ORIENTED_EDGE ( 'NONE', *, *, #35032, .T. ) ;
#25390=EDGE_CURVE ( 'NONE', #41176, #36336, #7232, .T. ) ;
#25391=ORIENTED_EDGE ( 'NONE', *, *, #23468, .T. ) ;
#25395=EDGE_LOOP ( 'NONE', ( #6828, #34283, #20365, #35422 ) ) ;
#25397=DIRECTION ( 'NONE',  ( 0.3482016354343866471, 0.000000000000000000, 0.9374196611341253371 ) ) ;
#25398=DIRECTION ( 'NONE',  ( 0.000000000000000000, 0.000000000000000000, 1.000000000000000000 ) ) ;
#25400=AXIS2_PLACEMENT_3D ( 'NONE', #16044, #44677, #40710 ) ;
#25401=AXIS2_PLACEMENT_3D ( 'NONE', #40550, #32683, #1129 ) ;
#25402=EDGE_CURVE ( 'NONE', #29823, #39129, #40047, .T. ) ;
#25404=FACE_BOUND ( 'NONE', #25551, .T. ) ;
#25405=ORIENTED_EDGE ( 'NONE', *, *, #30344, .F. ) ;
#25406=VECTOR ( 'NONE', #48013, 1000.000000000000114 ) ;
#25407=AXIS2_PLACEMENT_3D ( 'NONE', #21655, #37676, #41344 ) ;
#25408=DIRECTION ( 'NONE',  ( 0.000000000000000000, 1.000000000000000000, 0.000000000000000000 ) ) ;
#25409=VERTEX_POINT ( 'NONE', #39781 ) ;
#25410=VERTEX_POINT ( 'NONE', #3799 ) ;
#25411=CARTESIAN_POINT ( 'NONE',  ( -173.4787860028527007, -183.6283474603465606, 0.2918682030023308505 ) ) ;
#25412=ORIENTED_EDGE ( 'NONE', *, *, #6209, .F. ) ;
#25413=CARTESIAN_POINT ( 'NONE',  ( -26.20043062753592977, -175.3837268820161057, -122.9986166548863196 ) ) ;
#25417=ADVANCED_FACE ( 'NONE', ( #31659 ), #19570, .T. ) ;
#25419=DIRECTION ( 'NONE',  ( -0.6528221181905119463, 0.000000000000000000, -0.7575112421616284619 ) ) ;
#25420=ORIENTED_EDGE ( 'NONE', *, *, #17167, .F. ) ;
#25421=ORIENTED_EDGE ( 'NONE', *, *, #27608, .T. ) ;
#25422=CIRCLE ( 'NONE', #8600, 125.0000000000000000 ) ;
#25425=DIRECTION ( 'NONE',  ( -0.5586467658036415873, 0.000000000000000000, -0.8294056854502090959 ) ) ;
#25428=LINE ( 'NONE', #21487, #45482 ) ;
#25431=CIRCLE ( 'NONE', #32998, 125.0000000000000000 ) ;
#25432=VECTOR ( 'NONE', #15207, 1000.000000000000000 ) ;
#25436=DIRECTION ( 'NONE',  ( 0.000000000000000000, 1.000000000000000000, 0.000000000000000000 ) ) ;
#25437=VERTEX_POINT ( 'NONE', #39288 ) ;
#25440=EDGE_CURVE ( 'NONE', #40342, #41178, #8054, .T. ) ;
#25443=DIRECTION ( 'NONE',  ( 0.000000000000000000, 0.000000000000000000, -1.000000000000000000 ) ) ;
#25445=CARTESIAN_POINT ( 'NONE',  ( -47.63353074800703268, -193.5000000000000000, 0.5338233779648018373 ) ) ;
#25447=CYLINDRICAL_SURFACE ( 'NONE', #4955, 125.0000000000000000 ) ;
#25448=EDGE_LOOP ( 'NONE', ( #3675, #9447, #14284, #30327 ) ) ;
#25455=CARTESIAN_POINT ( 'NONE',  ( -49.13194886969936448, -189.7472609257535510, -0.7575112421616214675 ) ) ;
#25456=VERTEX_POINT ( 'NONE', #36371 ) ;
#25457=DIRECTION ( 'NONE',  ( 0.7765238627180349740, 0.000000000000000000, 0.6300878435817203194 ) ) ;
#25458=AXIS2_PLACEMENT_3D ( 'NONE', #2393, #27056, #42837 ) ;
#25459=CARTESIAN_POINT ( 'NONE',  ( 42.10477485469927927, -193.5000000000000000, 86.13684908212515268 ) ) ;
#25461=DIRECTION ( 'NONE',  ( 0.000000000000000000, 1.000000000000000000, 0.000000000000000000 ) ) ;
#25462=CARTESIAN_POINT ( 'NONE',  ( -167.9436818089035057, -177.1207230881787780, 36.78613984830045069 ) ) ;
#25464=VECTOR ( 'NONE', #51864, 1000.000000000000000 ) ;
#25465=CARTESIAN_POINT ( 'NONE',  ( 35.45604639379469347, -177.1207230881787780, 91.27439114664650788 ) ) ;
#25467=CARTESIAN_POINT ( 'NONE',  ( -99.62791064391781504, -189.7472609257535510, -114.0561348912352315 ) ) ;
#25469=ORIENTED_EDGE ( 'NONE', *, *, #27572, .F. ) ;
#25470=ORIENTED_EDGE ( 'NONE', *, *, #12598, .T. ) ;
#25471=VECTOR ( 'NONE', #1649, 1000.000000000000000 ) ;
#25472=ORIENTED_EDGE ( 'NONE', *, *, #3742, .F. ) ;
#25473=CARTESIAN_POINT ( 'NONE',  ( 75.67769207106684348, -177.1207230881787780, 14.49428645563876650 ) ) ;
#25474=CIRCLE ( 'NONE', #20434, 125.0000000000000000 ) ;
#25477=FACE_OUTER_BOUND ( 'NONE', #12043, .T. ) ;
#25478=LINE ( 'NONE', #33101, #608 ) ;
#25481=EDGE_LOOP ( 'NONE', ( #38256, #42199, #25831, #34031 ) ) ;
#25482=LINE ( 'NONE', #5530, #21451 ) ;
#25483=VERTEX_POINT ( 'NONE', #12193 ) ;
#25484=DIRECTION ( 'NONE',  ( 0.000000000000000000, 0.000000000000000000, 1.000000000000000000 ) ) ;
#25486=ORIENTED_EDGE ( 'NONE', *, *, #39814, .T. ) ;
#25487=DIRECTION ( 'NONE',  ( 0.9564009842765202052, 0.000000000000000000, 0.2920567706369833760 ) ) ;
#25490=AXIS2_PLACEMENT_3D ( 'NONE', #42515, #11487, #34381 ) ;
#25491=FACE_OUTER_BOUND ( 'NONE', #9818, .T. ) ;
#25493=ORIENTED_EDGE ( 'NONE', *, *, #2802, .F. ) ;
#25494=CARTESIAN_POINT ( 'NONE',  ( 8.448131207122518305, -175.3837268820161057, 111.2847127925100352 ) ) ;
#25500=LINE ( 'NONE', #17879, #19695 ) ;
#25501=ORIENTED_EDGE ( 'NONE', *, *, #47229, .F. ) ;
#25502=DIRECTION ( 'NONE',  ( -0.000000000000000000, 1.000000000000000000, -0.000000000000000000 ) ) ;
#25504=LINE ( 'NONE', #41522, #655 ) ;
#25506=VECTOR ( 'NONE', #37647, 1000.000000000000114 ) ;
#25507=ORIENTED_EDGE ( 'NONE', *, *, #42262, .T. ) ;
#25508=LINE ( 'NONE', #12375, #10568 ) ;
#25510=CARTESIAN_POINT ( 'NONE',  ( -168.1386673294336163, -189.7472609257535510, 32.52067927015837512 ) ) ;
#25511=ORIENTED_EDGE ( 'NONE', *, *, #7621, .T. ) ;
#25512=DIRECTION ( 'NONE',  ( 0.8124868780056742068, 0.000000000000000000, 0.5829794791144820021 ) ) ;
#25514=DIRECTION ( 'NONE',  ( 0.000000000000000000, 0.000000000000000000, -1.000000000000000000 ) ) ;
#25515=CARTESIAN_POINT ( 'NONE',  ( 55.35935253854127325, -177.1207230881787780, 69.58857822035042773 ) ) ;
#25517=DIRECTION ( 'NONE',  ( 0.000000000000000000, 0.000000000000000000, -1.000000000000000000 ) ) ;
#25518=CARTESIAN_POINT ( 'NONE',  ( 29.40217425202904167, -183.6283474603465606, -96.49160960477045990 ) ) ;
#25520=EDGE_LOOP ( 'NONE', ( #23654, #25217, #51544, #3948 ) ) ;
#25521=LINE ( 'NONE', #5572, #37410 ) ;
#25522=DIRECTION ( 'NONE',  ( 0.000000000000000000, 0.000000000000000000, 1.000000000000000000 ) ) ;
#25523=VECTOR ( 'NONE', #36876, 1000.000000000000114 ) ;
#25525=ADVANCED_FACE ( 'NONE', ( #16420 ), #32436, .F. ) ;
#25526=FACE_OUTER_BOUND ( 'NONE', #3914, .T. ) ;
#25533=VERTEX_POINT ( 'NONE', #48735 ) ;
#25535=LINE ( 'NONE', #40777, #24111 ) ;
#25536=EDGE_CURVE ( 'NONE', #33118, #7989, #16465, .T. ) ;
#25539=DIRECTION ( 'NONE',  ( -0.7378332790417285736, 0.000000000000000000, 0.6749830015182091136 ) ) ;
#25540=LINE ( 'NONE', #37365, #42123 ) ;
#25542=ORIENTED_EDGE ( 'NONE', *, *, #4735, .T. ) ;
#25543=ADVANCED_FACE ( 'NONE', ( #1681 ), #4857, .T. ) ;
#25544=ORIENTED_EDGE ( 'NONE', *, *, #30356, .T. ) ;
#25545=CARTESIAN_POINT ( 'NONE',  ( -48.47912675150885065, -183.6283474603465606, 6.938893903907228378E-15 ) ) ;
#25547=CARTESIAN_POINT ( 'NONE',  ( -48.47912675150885065, -177.1207230881787780, 6.938893903907228378E-15 ) ) ;
#25548=ORIENTED_EDGE ( 'NONE', *, *, #13327, .T. ) ;
#25550=FACE_OUTER_BOUND ( 'NONE', #34779, .T. ) ;
#25551=EDGE_LOOP ( 'NONE', ( #48770, #1523, #5981, #25639 ) ) ;
#25552=CARTESIAN_POINT ( 'NONE',  ( 63.31225588004632243, -177.1207230881787780, 55.92572546981597981 ) ) ;
#25553=CIRCLE ( 'NONE', #5429, 125.0000000000000000 ) ;
#25554=ORIENTED_EDGE ( 'NONE', *, *, #40415, .F. ) ;
#25558=CYLINDRICAL_SURFACE ( 'NONE', #22132, 125.0000000000000000 ) ;
#25559=DIRECTION ( 'NONE',  ( 0.9646355819083576311, 0.000000000000000000, 0.2635871660690715101 ) ) ;
#25560=AXIS2_PLACEMENT_3D ( 'NONE', #11102, #38451, #14290 ) ;
#25561=VERTEX_POINT ( 'NONE', #32941 ) ;
#25564=CARTESIAN_POINT ( 'NONE',  ( -148.6149069237406195, -183.6283474603465606, -74.81861753132353954 ) ) ;
#25566=CARTESIAN_POINT ( 'NONE',  ( 27.23560471289044571, -193.5000000000000000, 99.45993886622845537 ) ) ;
#25567=EDGE_LOOP ( 'NONE', ( #18028, #46191, #50131, #1281 ) ) ;
#25568=DIRECTION ( 'NONE',  ( -0.9564009842765223146, 0.000000000000000000, -0.2920567706369764371 ) ) ;
#25569=CIRCLE ( 'NONE', #16353, 125.0000000000000000 ) ;
#25571=ORIENTED_EDGE ( 'NONE', *, *, #4283, .T. ) ;
#25574=DIRECTION ( 'NONE',  ( 0.000000000000000000, -0.000000000000000000, -1.000000000000000000 ) ) ;
#25575=DIRECTION ( 'NONE',  ( 0.000000000000000000, 1.000000000000000000, -0.000000000000000000 ) ) ;
#25576=ORIENTED_EDGE ( 'NONE', *, *, #13621, .T. ) ;
#25577=DIRECTION ( 'NONE',  ( 0.000000000000000000, 0.000000000000000000, -1.000000000000000000 ) ) ;
#25578=EDGE_CURVE ( 'NONE', #4233, #30593, #44524, .T. ) ;
#25580=LINE ( 'NONE', #1420, #7295 ) ;
#25583=ORIENTED_EDGE ( 'NONE', *, *, #9224, .F. ) ;
#25584=DIRECTION ( 'NONE',  ( 0.000000000000000000, -1.000000000000000000, 0.000000000000000000 ) ) ;
#25586=VECTOR ( 'NONE', #6259, 1000.000000000000000 ) ;
#25587=CARTESIAN_POINT ( 'NONE',  ( -150.5816505765687623, -193.5000000000000000, 70.36529243996409377 ) ) ;
#25588=LINE ( 'NONE', #5651, #40419 ) ;
#25589=EDGE_LOOP ( 'NONE', ( #37174, #419, #31646, #21359 ) ) ;
#25590=EDGE_CURVE ( 'NONE', #48757, #26725, #45020, .T. ) ;
#25591=CIRCLE ( 'NONE', #45755, 125.0000000000000000 ) ;
#25592=VECTOR ( 'NONE', #21781, 1000.000000000000000 ) ;
#25593=ORIENTED_EDGE ( 'NONE', *, *, #30437, .F. ) ;
#25594=DIRECTION ( 'NONE',  ( -0.000000000000000000, 1.000000000000000000, -0.000000000000000000 ) ) ;
#25598=DIRECTION ( 'NONE',  ( -0.000000000000000000, 1.000000000000000000, -0.000000000000000000 ) ) ;
#25599=ORIENTED_EDGE ( 'NONE', *, *, #12541, .T. ) ;
#25600=ADVANCED_FACE ( 'NONE', ( #16933 ), #5113, .T. ) ;
#25601=CARTESIAN_POINT ( 'NONE',  ( -48.47912675150885065, -175.3837268820161057, 6.938893903907228378E-15 ) ) ;
#25604=CARTESIAN_POINT ( 'NONE',  ( -12.10142301649613827, -193.5000000000000000, -118.5439281552630604 ) ) ;
#25606=AXIS2_PLACEMENT_3D ( 'NONE', #910, #8532, #12482 ) ;
#25607=EDGE_CURVE ( 'NONE', #39414, #4155, #48994, .T. ) ;
#25612=VERTEX_POINT ( 'NONE', #49259 ) ;
#25613=EDGE_LOOP ( 'NONE', ( #46791, #6013, #27040, #20023 ) ) ;
#25614=VECTOR ( 'NONE', #26514, 1000.000000000000000 ) ;
#25616=CARTESIAN_POINT ( 'NONE',  ( -48.47912675150885065, -177.1207230881787780, 6.938893903907228378E-15 ) ) ;
#25617=DIRECTION ( 'NONE',  ( 0.000000000000000000, 0.000000000000000000, 1.000000000000000000 ) ) ;
#25618=LINE ( 'NONE', #1711, #16307 ) ;
#25619=VERTEX_POINT ( 'NONE', #21123 ) ;
#25620=ORIENTED_EDGE ( 'NONE', *, *, #22210, .F. ) ;
#25621=DIRECTION ( 'NONE',  ( 0.000000000000000000, 0.000000000000000000, 1.000000000000000000 ) ) ;
#25625=CARTESIAN_POINT ( 'NONE',  ( -89.44307666693794090, -177.1207230881787780, -117.0391155081702266 ) ) ;
#25627=VECTOR ( 'NONE', #38935, 1000.000000000000000 ) ;
#25628=VECTOR ( 'NONE', #32878, 1000.000000000000114 ) ;
#25629=CARTESIAN_POINT ( 'NONE',  ( -59.28786813212838069, -177.1207230881787780, 124.5318076226587323 ) ) ;
#25630=PLANE ( 'NONE',  #46904 ) ;
#25631=VERTEX_POINT ( 'NONE', #17470 ) ;
#25633=ORIENTED_EDGE ( 'NONE', *, *, #37390, .F. ) ;
#25634=EDGE_CURVE ( 'NONE', #39414, #35024, #34897, .T. ) ;
#25635=ORIENTED_EDGE ( 'NONE', *, *, #19626, .T. ) ;
#25636=CARTESIAN_POINT ( 'NONE',  ( -111.3904503173946381, -189.7472609257535510, -106.8558168688113454 ) ) ;
#25637=AXIS2_PLACEMENT_3D ( 'NONE', #31704, #8553, #151 ) ;
#25639=ORIENTED_EDGE ( 'NONE', *, *, #12198, .F. ) ;
#25640=VECTOR ( 'NONE', #24705, 1000.000000000000000 ) ;
#25641=ADVANCED_FACE ( 'NONE', ( #33489 ), #49526, .T. ) ;
#25643=CARTESIAN_POINT ( 'NONE',  ( -173.2419626162308646, -177.1207230881787780, 7.696413904698416353 ) ) ;
#25644=ADVANCED_FACE ( 'NONE', ( #25332 ), #4579, .T. ) ;
#25645=CARTESIAN_POINT ( 'NONE',  ( -129.4514457347087273, -175.3837268820161057, 95.22858582633115532 ) ) ;
#25646=DIRECTION ( 'NONE',  ( 0.000000000000000000, 0.000000000000000000, 1.000000000000000000 ) ) ;
#25650=EDGE_CURVE ( 'NONE', #47079, #32649, #11416, .T. ) ;
#25651=CARTESIAN_POINT ( 'NONE',  ( 74.95461934957533856, -189.7472609257535510, -11.83705339977243121 ) ) ;
#25652=VECTOR ( 'NONE', #2742, 1000.000000000000000 ) ;
#25654=ORIENTED_EDGE ( 'NONE', *, *, #5272, .F. ) ;
#25655=EDGE_CURVE ( 'NONE', #14417, #49807, #29777, .T. ) ;
#25656=CARTESIAN_POINT ( 'NONE',  ( -29.73468717939733352, -177.1207230881787780, 123.5865930638410930 ) ) ;
#25657=VERTEX_POINT ( 'NONE', #37935 ) ;
#25658=VERTEX_POINT ( 'NONE', #42128 ) ;
#25661=ORIENTED_EDGE ( 'NONE', *, *, #25745, .T. ) ;
#25662=EDGE_CURVE ( 'NONE', #6819, #39220, #42655, .T. ) ;
#25663=CARTESIAN_POINT ( 'NONE',  ( -48.93575598890257794, -193.5000000000000000, 0.8896570909947506545 ) ) ;
#25670=AXIS2_PLACEMENT_3D ( 'NONE', #36496, #32572, #776 ) ;
#25674=ORIENTED_EDGE ( 'NONE', *, *, #35426, .T. ) ;
#25675=EDGE_CURVE ( 'NONE', #48486, #50678, #8915, .T. ) ;
#25676=EDGE_LOOP ( 'NONE', ( #36503, #20835, #44817, #50326 ) ) ;
#25678=PLANE ( 'NONE',  #31870 ) ;
#25679=ORIENTED_EDGE ( 'NONE', *, *, #5091, .T. ) ;
#25680=AXIS2_PLACEMENT_3D ( 'NONE', #51060, #31838, #39448 ) ;
#25681=PLANE ( 'NONE',  #18403 ) ;
#25682=AXIS2_PLACEMENT_3D ( 'NONE', #46936, #37986, #31138 ) ;
#25684=DIRECTION ( 'NONE',  ( 0.000000000000000000, 0.000000000000000000, 1.000000000000000000 ) ) ;
#25685=ORIENTED_EDGE ( 'NONE', *, *, #43924, .F. ) ;
#25686=VECTOR ( 'NONE', #47043, 1000.000000000000000 ) ;
#25687=EDGE_CURVE ( 'NONE', #38237, #41833, #25853, .T. ) ;
#25689=AXIS2_PLACEMENT_3D ( 'NONE', #45171, #10372, #29106 ) ;
#25693=CARTESIAN_POINT ( 'NONE',  ( 76.21810084846656252, -193.5000000000000000, -8.694908215727984668 ) ) ;
#25694=EDGE_LOOP ( 'NONE', ( #12118, #3663, #22969, #49820 ) ) ;
#25695=ORIENTED_EDGE ( 'NONE', *, *, #39109, .T. ) ;
#25696=ORIENTED_EDGE ( 'NONE', *, *, #14835, .F. ) ;
#25699=ORIENTED_EDGE ( 'NONE', *, *, #41210, .T. ) ;
#25700=DIRECTION ( 'NONE',  ( -0.000000000000000000, 1.000000000000000000, -0.000000000000000000 ) ) ;
#25704=VERTEX_POINT ( 'NONE', #38182 ) ;
#25707=CIRCLE ( 'NONE', #34916, 125.0000000000000000 ) ;
#25709=AXIS2_PLACEMENT_3D ( 'NONE', #4637, #20403, #36702 ) ;
#25712=CARTESIAN_POINT ( 'NONE',  ( 46.40005841627163363, -183.6283474603465606, 81.38144888055276738 ) ) ;
#25713=LINE ( 'NONE', #25459, #6287 ) ;
#25717=CYLINDRICAL_SURFACE ( 'NONE', #27132, 124.9999999999999858 ) ;
#25718=CARTESIAN_POINT ( 'NONE',  ( -127.4665351220365892, -193.5000000000000000, -96.88131563365291754 ) ) ;
#25723=EDGE_CURVE ( 'NONE', #25303, #4861, #26056, .T. ) ;
#25724=LINE ( 'NONE', #37559, #34130 ) ;
#25725=ORIENTED_EDGE ( 'NONE', *, *, #20026, .F. ) ;
#25726=AXIS2_PLACEMENT_3D ( 'NONE', #17178, #21111, #49243 ) ;
#25727=AXIS2_PLACEMENT_3D ( 'NONE', #37336, #6071, #49458 ) ;
#25729=CIRCLE ( 'NONE', #3061, 125.0000000000000000 ) ;
#25731=LINE ( 'NONE', #17599, #28638 ) ;
#25733=CARTESIAN_POINT ( 'NONE',  ( -48.93575598890255662, -193.5000000000000000, -0.8896570909947461026 ) ) ;
#25734=AXIS2_PLACEMENT_3D ( 'NONE', #51672, #11190, #3565 ) ;
#25735=ORIENTED_EDGE ( 'NONE', *, *, #31115, .F. ) ;
#25739=DIRECTION ( 'NONE',  ( 0.000000000000000000, -1.000000000000000000, -0.000000000000000000 ) ) ;
#25742=PLANE ( 'NONE',  #45954 ) ;
#25743=DIRECTION ( 'NONE',  ( 0.2348860457809707758, 0.000000000000000000, 0.9720229140804138579 ) ) ;
#25745=EDGE_CURVE ( 'NONE', #33552, #16495, #50034, .T. ) ;
#25746=LINE ( 'NONE', #17529, #47485 ) ;
#25748=DIRECTION ( 'NONE',  ( 0.000000000000000000, 0.000000000000000000, 1.000000000000000000 ) ) ;
#25749=VECTOR ( 'NONE', #51019, 1000.000000000000000 ) ;
#25750=VECTOR ( 'NONE', #42657, 1000.000000000000227 ) ;
#25752=CARTESIAN_POINT ( 'NONE',  ( -70.75782287548091176, -193.5000000000000000, 122.9986166548864901 ) ) ;
#25753=VECTOR ( 'NONE', #9517, 1000.000000000000114 ) ;
#25754=ORIENTED_EDGE ( 'NONE', *, *, #31760, .T. ) ;
#25756=CARTESIAN_POINT ( 'NONE',  ( -95.72791768350683128, -183.6283474603465606, -115.7261930397105232 ) ) ;
#25757=ORIENTED_EDGE ( 'NONE', *, *, #25840, .T. ) ;
#25759=FACE_OUTER_BOUND ( 'NONE', #25395, .T. ) ;
#25761=AXIS2_PLACEMENT_3D ( 'NONE', #46794, #38377, #38630 ) ;
#25763=CARTESIAN_POINT ( 'NONE',  ( 45.36094686508022988, -183.6283474603465606, -82.57748230379237953 ) ) ;
#25764=AXIS2_PLACEMENT_3D ( 'NONE', #18736, #2182, #38445 ) ;
#25766=DIRECTION ( 'NONE',  ( -0.9890401873221654760, 0.000000000000000000, 0.1476465640024710868 ) ) ;
#25767=VERTEX_POINT ( 'NONE', #30051 ) ;
#25768=LINE ( 'NONE', #49686, #17533 ) ;
#25770=DIRECTION ( 'NONE',  ( 0.000000000000000000, 1.000000000000000000, 0.000000000000000000 ) ) ;
#25772=ORIENTED_EDGE ( 'NONE', *, *, #35486, .F. ) ;
#25773=AXIS2_PLACEMENT_3D ( 'NONE', #17639, #41264, #12892 ) ;
#25778=PLANE ( 'NONE',  #23298 ) ;
#25779=DIRECTION ( 'NONE',  ( -0.000000000000000000, 1.000000000000000000, -0.000000000000000000 ) ) ;
#25781=CARTESIAN_POINT ( 'NONE',  ( -37.08895481556041318, -193.5000000000000000, 124.4799742258550310 ) ) ;
#25783=EDGE_CURVE ( 'NONE', #7329, #22006, #10084, .T. ) ;
#25784=LINE ( 'NONE', #14226, #48979 ) ;
#25785=CARTESIAN_POINT ( 'NONE',  ( -172.2804936848317823, -183.6283474603465606, -7.024906801078577345 ) ) ;
#25787=EDGE_LOOP ( 'NONE', ( #21027, #33697, #46677, #5058 ) ) ;
#25788=VECTOR ( 'NONE', #5026, 1000.000000000000000 ) ;
#25789=VECTOR ( 'NONE', #16036, 1000.000000000000114 ) ;
#25790=DIRECTION ( 'NONE',  ( 0.000000000000000000, 1.000000000000000000, 0.000000000000000000 ) ) ;
#25791=LINE ( 'NONE', #2642, #30291 ) ;
#25793=DIRECTION ( 'NONE',  ( 0.000000000000000000, -1.000000000000000000, 0.000000000000000000 ) ) ;
#25797=AXIS2_PLACEMENT_3D ( 'NONE', #29746, #18456, #29486 ) ;
#25798=LINE ( 'NONE', #42076, #47153 ) ;
#25799=EDGE_CURVE ( 'NONE', #31054, #28133, #38698, .T. ) ;
#25800=DIRECTION ( 'NONE',  ( -0.6068001458186002006, 0.000000000000000000, 0.7948544414133481562 ) ) ;
#25801=DIRECTION ( 'NONE',  ( 0.7175072570443249420, 0.000000000000000000, 0.6965510290630033685 ) ) ;
#25802=ORIENTED_EDGE ( 'NONE', *, *, #31001, .F. ) ;
#25804=ORIENTED_EDGE ( 'NONE', *, *, #447, .F. ) ;
#25806=AXIS2_PLACEMENT_3D ( 'NONE', #24736, #40749, #293 ) ;
#25807=DIRECTION ( 'NONE',  ( -0.9564009842765223146, 0.000000000000000000, -0.2920567706369764371 ) ) ;
#25808=PLANE ( 'NONE',  #6052 ) ;
#25809=ORIENTED_EDGE ( 'NONE', *, *, #38153, .T. ) ;
#25810=ORIENTED_EDGE ( 'NONE', *, *, #11482, .T. ) ;
#25812=LINE ( 'NONE', #49991, #32573 ) ;
#25813=ADVANCED_FACE ( 'NONE', ( #34755 ), #50808, .T. ) ;
#25815=LINE ( 'NONE', #21623, #38098 ) ;
#25816=ORIENTED_EDGE ( 'NONE', *, *, #10936, .F. ) ;
#25817=DIRECTION ( 'NONE',  ( -0.000000000000000000, -1.000000000000000000, 0.000000000000000000 ) ) ;
#25818=AXIS2_PLACEMENT_3D ( 'NONE', #45876, #21429, #49038 ) ;
#25822=CARTESIAN_POINT ( 'NONE',  ( -43.48323084606168720, -193.5000000000000000, 123.9001241957026167 ) ) ;
#25823=ORIENTED_EDGE ( 'NONE', *, *, #3326, .T. ) ;
#25824=CARTESIAN_POINT ( 'NONE',  ( -173.3968853974275817, -189.7472609257535510, 4.533605064404221174 ) ) ;
#25825=VECTOR ( 'NONE', #24500, 1000.000000000000000 ) ;
#25826=ORIENTED_EDGE ( 'NONE', *, *, #32288, .F. ) ;
#25827=DIRECTION ( 'NONE',  ( 0.000000000000000000, -0.000000000000000000, 1.000000000000000000 ) ) ;
#25828=LINE ( 'NONE', #33959, #14563 ) ;
#25829=CARTESIAN_POINT ( 'NONE',  ( 15.80042947435468470, -189.7472609257535510, 107.2060569716377927 ) ) ;
#25830=EDGE_CURVE ( 'NONE', #47918, #16064, #35283, .T. ) ;
#25831=ORIENTED_EDGE ( 'NONE', *, *, #9165, .T. ) ;
#25834=DIRECTION ( 'NONE',  ( 0.000000000000000000, -0.000000000000000000, -1.000000000000000000 ) ) ;
#25836=ORIENTED_EDGE ( 'NONE', *, *, #37765, .T. ) ;
#25837=PLANE ( 'NONE',  #14938 ) ;
#25838=AXIS2_PLACEMENT_3D ( 'NONE', #8498, #21646, #9548 ) ;
#25839=ORIENTED_EDGE ( 'NONE', *, *, #11468, .F. ) ;
#25840=EDGE_CURVE ( 'NONE', #32508, #27501, #7600, .T. ) ;
#25841=LINE ( 'NONE', #14019, #41001 ) ;
#25845=ORIENTED_EDGE ( 'NONE', *, *, #16012, .T. ) ;
#25847=ORIENTED_EDGE ( 'NONE', *, *, #32040, .T. ) ;
#25848=ADVANCED_FACE ( 'NONE', ( #24236 ), #43684, .T. ) ;
#25849=PLANE ( 'NONE',  #1915 ) ;
#25853=LINE ( 'NONE', #41882, #6423 ) ;
#25854=DIRECTION ( 'NONE',  ( -0.000000000000000000, -1.000000000000000000, 0.000000000000000000 ) ) ;
#25855=DIRECTION ( 'NONE',  ( 0.000000000000000000, 0.000000000000000000, 1.000000000000000000 ) ) ;
#25856=CARTESIAN_POINT ( 'NONE',  ( -170.8336150310145172, -175.3837268820161057, 25.58083653558494674 ) ) ;
#25858=FACE_OUTER_BOUND ( 'NONE', #12579, .T. ) ;
#25859=VERTEX_POINT ( 'NONE', #39717 ) ;
#25860=VECTOR ( 'NONE', #23328, 1000.000000000000000 ) ;
#25861=ADVANCED_FACE ( 'NONE', ( #15316 ), #27127, .F. ) ;
#25862=DIRECTION ( 'NONE',  ( -0.000000000000000000, 1.000000000000000000, -0.000000000000000000 ) ) ;
#25864=ORIENTED_EDGE ( 'NONE', *, *, #31877, .F. ) ;
#25865=AXIS2_PLACEMENT_3D ( 'NONE', #38206, #51871, #72 ) ;
#25866=ORIENTED_EDGE ( 'NONE', *, *, #19784, .F. ) ;
#25867=CARTESIAN_POINT ( 'NONE',  ( 141.7825277784304205, -213.5000000000000000, -41.45482488023466061 ) ) ;
#25868=VECTOR ( 'NONE', #1044, 1000.000000000000227 ) ;
#25870=DIRECTION ( 'NONE',  ( -0.000000000000000000, 1.000000000000000000, -0.000000000000000000 ) ) ;
#25872=LINE ( 'NONE', #2480, #35880 ) ;
#25878=EDGE_LOOP ( 'NONE', ( #35461, #3103, #15309, #28443 ) ) ;
#25879=AXIS2_PLACEMENT_3D ( 'NONE', #4183, #41202, #28593 ) ;
#25881=CARTESIAN_POINT ( 'NONE',  ( -14.28570516517293676, -177.1207230881787780, 120.2323164553486663 ) ) ;
#25882=CARTESIAN_POINT ( 'NONE',  ( 36.10886851198521441, -193.5000000000000000, 92.03190238880813467 ) ) ;
#25883=CARTESIAN_POINT ( 'NONE',  ( -12.76653800058364574, -193.5000000000000000, -119.7898618611244927 ) ) ;
#25884=ORIENTED_EDGE ( 'NONE', *, *, #47801, .T. ) ;
#25885=EDGE_CURVE ( 'NONE', #40042, #34277, #40244, .T. ) ;
#25888=LINE ( 'NONE', #33255, #10527 ) ;
#25889=ORIENTED_EDGE ( 'NONE', *, *, #35313, .T. ) ;
#25891=EDGE_LOOP ( 'NONE', ( #48881, #7383, #27664, #34928 ) ) ;
#25894=VECTOR ( 'NONE', #45416, 1000.000000000000000 ) ;
#25896=VECTOR ( 'NONE', #40462, 1000.000000000000114 ) ;
#25899=ORIENTED_EDGE ( 'NONE', *, *, #52010, .F. ) ;
#25901=DIRECTION ( 'NONE',  ( 0.000000000000000000, 0.000000000000000000, -1.000000000000000000 ) ) ;
#25902=ORIENTED_EDGE ( 'NONE', *, *, #33047, .T. ) ;
#25903=ADVANCED_FACE ( 'NONE', ( #51572 ), #48153, .T. ) ;
#25905=PLANE ( 'NONE',  #16194 ) ;
#25906=AXIS2_PLACEMENT_3D ( 'NONE', #47794, #40150, #11767 ) ;
#25907=ADVANCED_FACE ( 'NONE', ( #35278 ), #15576, .T. ) ;
#25909=ORIENTED_EDGE ( 'NONE', *, *, #330, .T. ) ;
#25911=DIRECTION ( 'NONE',  ( 0.000000000000000000, 0.000000000000000000, -1.000000000000000000 ) ) ;
#25912=LINE ( 'NONE', #25645, #34747 ) ;
#25913=CARTESIAN_POINT ( 'NONE',  ( -48.18706998087188254, -189.7472609257535510, 0.9564009842765313074 ) ) ;
#25915=CARTESIAN_POINT ( 'NONE',  ( 70.68712318874649725, -183.6283474603465606, -37.74128873232327663 ) ) ;
#25916=CARTESIAN_POINT ( 'NONE',  ( -48.47912675150885065, -193.5000000000000000, 6.938893903907228378E-15 ) ) ;
#25917=VERTEX_POINT ( 'NONE', #19758 ) ;
#25921=CARTESIAN_POINT ( 'NONE',  ( -48.47912675150885065, -175.3837268820161057, 6.938893903907228378E-15 ) ) ;
#25923=DIRECTION ( 'NONE',  ( 0.000000000000000000, 0.000000000000000000, 1.000000000000000000 ) ) ;
#25924=AXIS2_PLACEMENT_3D ( 'NONE', #4467, #28622, #5001 ) ;
#25925=DIRECTION ( 'NONE',  ( -0.000000000000000000, 1.000000000000000000, -0.000000000000000000 ) ) ;
#25926=CARTESIAN_POINT ( 'NONE',  ( -162.7543581613524282, -177.1207230881787780, 50.65739320402010293 ) ) ;
#25927=VERTEX_POINT ( 'NONE', #39472 ) ;
#25928=VECTOR ( 'NONE', #20972, 1000.000000000000000 ) ;
#25929=CARTESIAN_POINT ( 'NONE',  ( 75.48400724637754422, -193.5000000000000000, -16.06677968424457248 ) ) ;
#25930=DIRECTION ( 'NONE',  ( 0.000000000000000000, 1.000000000000000000, -0.000000000000000000 ) ) ;
#25933=ORIENTED_EDGE ( 'NONE', *, *, #33376, .F. ) ;
#25934=DIRECTION ( 'NONE',  ( 0.000000000000000000, 1.000000000000000000, 0.000000000000000000 ) ) ;
#25937=ADVANCED_FACE ( 'NONE', ( #35792 ), #7683, .T. ) ;
#25939=DIRECTION ( 'NONE',  ( 0.000000000000000000, 1.000000000000000000, -0.000000000000000000 ) ) ;
#25941=EDGE_LOOP ( 'NONE', ( #22602, #8980, #23127, #17112 ) ) ;
#25943=EDGE_CURVE ( 'NONE', #37599, #21989, #47862, .T. ) ;
#25946=VECTOR ( 'NONE', #6714, 1000.000000000000000 ) ;
#25947=CARTESIAN_POINT ( 'NONE',  ( -91.81555821786916738, -175.3837268820161057, 116.1806952091180563 ) ) ;
#25950=ORIENTED_EDGE ( 'NONE', *, *, #4612, .F. ) ;
#25951=VERTEX_POINT ( 'NONE', #4260 ) ;
#25953=ORIENTED_EDGE ( 'NONE', *, *, #32127, .F. ) ;
#25954=LINE ( 'NONE', #10703, #36719 ) ;
#25955=CARTESIAN_POINT ( 'NONE',  ( -37.14819544345410662, -183.6283474603465606, 123.4817304940907263 ) ) ;
#25957=CYLINDRICAL_SURFACE ( 'NONE', #22961, 125.0000000000000000 ) ;
#25959=ORIENTED_EDGE ( 'NONE', *, *, #23584, .F. ) ;
#25960=EDGE_CURVE ( 'NONE', #3648, #17251, #37087, .T. ) ;
#25961=DIRECTION ( 'NONE',  ( 0.000000000000000000, 0.000000000000000000, -1.000000000000000000 ) ) ;
#25962=EDGE_LOOP ( 'NONE', ( #12236, #6693, #31388, #49648 ) ) ;
#25964=EDGE_LOOP ( 'NONE', ( #47451, #22936, #42383, #42419 ) ) ;
#25965=LINE ( 'NONE', #18849, #43823 ) ;
#25966=LINE ( 'NONE', #30417, #44922 ) ;
#25967=EDGE_CURVE ( 'NONE', #18737, #9242, #25024, .T. ) ;
#25968=VECTOR ( 'NONE', #50118, 1000.000000000000000 ) ;
#25969=CARTESIAN_POINT ( 'NONE',  ( -148.0127667507368585, -177.1207230881787780, -75.61781872352626976 ) ) ;
#25972=DIRECTION ( 'NONE',  ( -0.6300878435817203194, 0.000000000000000000, 0.7765238627180349740 ) ) ;
#25973=DIRECTION ( 'NONE',  ( -0.000000000000000000, 1.000000000000000000, -0.000000000000000000 ) ) ;
#25977=VERTEX_POINT ( 'NONE', #1087 ) ;
#25979=DIRECTION ( 'NONE',  ( 0.000000000000000000, 1.000000000000000000, 0.000000000000000000 ) ) ;
#25980=EDGE_CURVE ( 'NONE', #34528, #47296, #44998, .T. ) ;
#25981=DIRECTION ( 'NONE',  ( 0.9785564922995046988, 0.000000000000000000, -0.2059786187410953262 ) ) ;
#25982=EDGE_LOOP ( 'NONE', ( #8810, #31992, #24617, #10095 ) ) ;
#25983=FACE_OUTER_BOUND ( 'NONE', #45527, .T. ) ;
#25985=DIRECTION ( 'NONE',  ( 0.000000000000000000, 1.000000000000000000, 0.000000000000000000 ) ) ;
#25986=ORIENTED_EDGE ( 'NONE', *, *, #2663, .T. ) ;
#25987=DIRECTION ( 'NONE',  ( -0.000000000000000000, -1.000000000000000000, 0.000000000000000000 ) ) ;
#25989=ADVANCED_FACE ( 'NONE', ( #44468 ), #41287, .T. ) ;
#25990=VECTOR ( 'NONE', #44819, 1000.000000000000000 ) ;
#25993=PLANE ( 'NONE',  #32907 ) ;
#25994=CARTESIAN_POINT ( 'NONE',  ( -169.9131040279660283, -177.1207230881787780, 29.64437826672835996 ) ) ;
#25999=EDGE_LOOP ( 'NONE', ( #38219, #8120, #32700, #5276 ) ) ;
#26000=EDGE_CURVE ( 'NONE', #12871, #25410, #32880, .T. ) ;
#26001=PLANE ( 'NONE',  #25054 ) ;
#26002=AXIS2_PLACEMENT_3D ( 'NONE', #9713, #34402, #50446 ) ;
#26004=DIRECTION ( 'NONE',  ( -0.000000000000000000, 1.000000000000000000, -0.000000000000000000 ) ) ;
#26006=ADVANCED_FACE ( 'NONE', ( #21067 ), #17137, .T. ) ;
#26008=ADVANCED_FACE ( 'NONE', ( #9254 ), #16349, .T. ) ;
#26009=DIRECTION ( 'NONE',  ( 0.000000000000000000, -1.000000000000000000, 0.000000000000000000 ) ) ;
#26010=CARTESIAN_POINT ( 'NONE',  ( -48.47912675150885065, -183.6283474603465606, 6.938893903907228378E-15 ) ) ;
#26013=DIRECTION ( 'NONE',  ( -0.000000000000000000, 1.000000000000000000, -0.000000000000000000 ) ) ;
#26014=ORIENTED_EDGE ( 'NONE', *, *, #23924, .T. ) ;
#26015=PLANE ( 'NONE',  #15566 ) ;
#26017=DIRECTION ( 'NONE',  ( 0.9890401873221644768, 0.000000000000000000, -0.1476465640024779702 ) ) ;
#26019=LINE ( 'NONE', #2094, #713 ) ;
#26021=CARTESIAN_POINT ( 'NONE',  ( -22.44626007086656472, -183.6283474603465606, 122.2591094863196872 ) ) ;
#26023=ORIENTED_EDGE ( 'NONE', *, *, #21957, .T. ) ;
#26024=AXIS2_PLACEMENT_3D ( 'NONE', #35558, #80, #40268 ) ;
#26027=EDGE_LOOP ( 'NONE', ( #42021, #49572, #21765, #40036 ) ) ;
#26028=LINE ( 'NONE', #8970, #157 ) ;
#26029=LINE ( 'NONE', #38372, #36583 ) ;
#26031=ORIENTED_EDGE ( 'NONE', *, *, #48777, .F. ) ;
#26032=DIRECTION ( 'NONE',  ( 0.6068001458185945385, 0.000000000000000000, -0.7948544414133523750 ) ) ;
#26033=CARTESIAN_POINT ( 'NONE',  ( -154.6193097927903182, -189.7472609257535510, -66.02470404298124151 ) ) ;
#26034=DIRECTION ( 'NONE',  ( 0.000000000000000000, 0.000000000000000000, 1.000000000000000000 ) ) ;
#26037=EDGE_CURVE ( 'NONE', #14521, #3, #26874, .T. ) ;
#26039=LINE ( 'NONE', #49704, #46429 ) ;
#26045=DIRECTION ( 'NONE',  ( -0.9027978299657387629, 0.000000000000000000, -0.4300652022765304450 ) ) ;
#26046=DIRECTION ( 'NONE',  ( 0.000000000000000000, 0.000000000000000000, 1.000000000000000000 ) ) ;
#26047=DIRECTION ( 'NONE',  ( -0.000000000000000000, 1.000000000000000000, -0.000000000000000000 ) ) ;
#26048=LINE ( 'NONE', #1088, #19889 ) ;
#26049=CARTESIAN_POINT ( 'NONE',  ( -48.82732838694325750, -193.5000000000000000, 0.9374196611341252261 ) ) ;
#26050=CARTESIAN_POINT ( 'NONE',  ( -102.5006284722404502, -193.5000000000000000, -112.7238987608084386 ) ) ;
#26051=DIRECTION ( 'NONE',  ( 0.000000000000000000, 1.000000000000000000, 0.000000000000000000 ) ) ;
#26052=LINE ( 'NONE', #42078, #11089 ) ;
#26053=ORIENTED_EDGE ( 'NONE', *, *, #29452, .F. ) ;
#26055=CIRCLE ( 'NONE', #11789, 125.0000000000000000 ) ;
#26056=CIRCLE ( 'NONE', #45360, 125.0000000000000000 ) ;
#26057=DIRECTION ( 'NONE',  ( 0.000000000000000000, -1.000000000000000000, -0.000000000000000000 ) ) ;
#26060=ORIENTED_EDGE ( 'NONE', *, *, #43803, .T. ) ;
#26061=EDGE_LOOP ( 'NONE', ( #48596, #8531, #6106, #46946 ) ) ;
#26062=CARTESIAN_POINT ( 'NONE',  ( -171.5592422664403216, -193.5000000000000000, -21.82395850507255730 ) ) ;
#26063=ADVANCED_FACE ( 'NONE', ( #44727 ), #12395, .F. ) ;
#26064=ADVANCED_FACE ( 'NONE', ( #4788 ), #20817, .F. ) ;
#26065=CARTESIAN_POINT ( 'NONE',  ( 24.15597040328003331, -183.6283474603465606, -101.7307360698544159 ) ) ;
#26066=CARTESIAN_POINT ( 'NONE',  ( 59.80284513346456521, -193.5000000000000000, 62.45009659481583952 ) ) ;
#26069=LINE ( 'NONE', #26840, #25235 ) ;
#26070=DIRECTION ( 'NONE',  ( 0.000000000000000000, 1.000000000000000000, 0.000000000000000000 ) ) ;
#26073=CARTESIAN_POINT ( 'NONE',  ( -172.9701362814535912, -175.3837268820161057, -11.26891947860193177 ) ) ;
#26074=EDGE_LOOP ( 'NONE', ( #2205, #4549, #23725, #21551 ) ) ;
#26076=ORIENTED_EDGE ( 'NONE', *, *, #38827, .T. ) ;
#26078=CARTESIAN_POINT ( 'NONE',  ( 65.79610465833508215, -193.5000000000000000, -50.65739320401928580 ) ) ;
#26079=CARTESIAN_POINT ( 'NONE',  ( 70.19984492582109681, -175.3837268820161057, 39.24667733211968823 ) ) ;
#26080=EDGE_LOOP ( 'NONE', ( #27665, #4538, #36920, #18352 ) ) ;
#26081=VERTEX_POINT ( 'NONE', #2124 ) ;
#26082=CARTESIAN_POINT ( 'NONE',  ( -164.6246685127424882, -193.5000000000000000, -46.20836643930983456 ) ) ;
#26083=DIRECTION ( 'NONE',  ( -0.000000000000000000, 1.000000000000000000, 0.000000000000000000 ) ) ;
#26085=EDGE_CURVE ( 'NONE', #6100, #9931, #50748, .T. ) ;
#26086=CARTESIAN_POINT ( 'NONE',  ( 17.44316424268010124, -193.5000000000000000, -105.0256126866231625 ) ) ;
#26087=AXIS2_PLACEMENT_3D ( 'NONE', #9504, #14232, #26046 ) ;
#26091=ADVANCED_FACE ( 'NONE', ( #17914 ), #46297, .T. ) ;
#26092=VECTOR ( 'NONE', #21792, 1000.000000000000227 ) ;
#26093=EDGE_LOOP ( 'NONE', ( #19176, #35622, #27976, #39543 ) ) ;
#26094=LINE ( 'NONE', #18224, #17382 ) ;
#26095=ORIENTED_EDGE ( 'NONE', *, *, #51045, .T. ) ;
#26096=LINE ( 'NONE', #14026, #39011 ) ;
#26097=CARTESIAN_POINT ( 'NONE',  ( 21.21056010634070432, -189.7472609257535510, 103.7706487676302061 ) ) ;
#26099=CARTESIAN_POINT ( 'NONE',  ( 76.51419089073348800, -193.5000000000000000, -1.292495564988658030 ) ) ;
#26101=FACE_OUTER_BOUND ( 'NONE', #17328, .T. ) ;
#26102=EDGE_CURVE ( 'NONE', #27341, #7466, #9764, .T. ) ;
#26105=VERTEX_POINT ( 'NONE', #30499 ) ;
#26108=DIRECTION ( 'NONE',  ( 0.000000000000000000, 1.000000000000000000, 0.000000000000000000 ) ) ;
#26109=DIRECTION ( 'NONE',  ( 0.5085311186492216251, 0.000000000000000000, -0.8610436117673548884 ) ) ;
#26110=ORIENTED_EDGE ( 'NONE', *, *, #32534, .F. ) ;
#26111=VERTEX_POINT ( 'NONE', #14744 ) ;
#26113=EDGE_CURVE ( 'NONE', #39890, #8565, #4226, .T. ) ;
#26114=CARTESIAN_POINT ( 'NONE',  ( -48.47912675150885065, -189.7472609257535510, 1.000000000000006883 ) ) ;
#26115=ORIENTED_EDGE ( 'NONE', *, *, #13267, .F. ) ;
#26117=VERTEX_POINT ( 'NONE', #29993 ) ;
#26119=CARTESIAN_POINT ( 'NONE',  ( 76.52053249983501360, -183.6283474603465606, -0.2918682030015273265 ) ) ;
#26120=AXIS2_PLACEMENT_3D ( 'NONE', #26420, #9896, #37992 ) ;
#26121=EDGE_CURVE ( 'NONE', #32749, #5608, #14233, .T. ) ;
#26122=DIRECTION ( 'NONE',  ( 0.8294056854502049880, 0.000000000000000000, -0.5586467658036476935 ) ) ;
#26123=DIRECTION ( 'NONE',  ( 0.000000000000000000, 1.000000000000000000, -0.000000000000000000 ) ) ;
#26124=ORIENTED_EDGE ( 'NONE', *, *, #34547, .F. ) ;
#26125=EDGE_LOOP ( 'NONE', ( #30139, #10896, #1734, #51832 ) ) ;
#26128=CARTESIAN_POINT ( 'NONE',  ( 39.18328161278951427, -175.3837268820161057, 89.10837311819236106 ) ) ;
#26129=CARTESIAN_POINT ( 'NONE',  ( -47.70260288879080690, -189.7472609257535510, -0.6300878435817026668 ) ) ;
#26130=EDGE_CURVE ( 'NONE', #19079, #3016, #11757, .T. ) ;
#26131=CARTESIAN_POINT ( 'NONE',  ( -47.78257572244585560, -175.3837268820161057, -0.7175072570443230546 ) ) ;
#26133=EDGE_LOOP ( 'NONE', ( #25470, #6870, #25593, #51676 ) ) ;
#26134=DIRECTION ( 'NONE',  ( 0.5829794791144762289, 0.000000000000000000, -0.8124868780056783146 ) ) ;
#26135=CIRCLE ( 'NONE', #50506, 125.0000000000000000 ) ;
#26136=EDGE_LOOP ( 'NONE', ( #27414, #551, #50396, #15806 ) ) ;
#26137=DIRECTION ( 'NONE',  ( -0.000000000000000000, 1.000000000000000000, -0.000000000000000000 ) ) ;
#26138=ORIENTED_EDGE ( 'NONE', *, *, #47015, .F. ) ;
#26140=CARTESIAN_POINT ( 'NONE',  ( 58.48829670243886625, -193.5000000000000000, -64.67588669375805921 ) ) ;
#26141=ADVANCED_FACE ( 'NONE', ( #2644 ), #6086, .T. ) ;
#26145=VERTEX_POINT ( 'NONE', #30761 ) ;
#26146=PLANE ( 'NONE',  #51092 ) ;
#26148=ORIENTED_EDGE ( 'NONE', *, *, #11519, .F. ) ;
#26149=DIRECTION ( 'NONE',  ( 0.000000000000000000, -0.000000000000000000, 1.000000000000000000 ) ) ;
#26150=CARTESIAN_POINT ( 'NONE',  ( 32.99469856375239374, -189.7472609257535510, 94.79987230212019256 ) ) ;
#26151=ORIENTED_EDGE ( 'NONE', *, *, #10877, .F. ) ;
#26152=AXIS2_PLACEMENT_3D ( 'NONE', #25338, #13256, #29279 ) ;
#26154=PLANE ( 'NONE',  #47369 ) ;
#26155=DIRECTION ( 'NONE',  ( 0.000000000000000000, -1.000000000000000000, 0.000000000000000000 ) ) ;
#26158=VECTOR ( 'NONE', #46553, 1000.000000000000227 ) ;
#26159=DIRECTION ( 'NONE',  ( -0.000000000000000000, 1.000000000000000000, 0.000000000000000000 ) ) ;
#26160=ORIENTED_EDGE ( 'NONE', *, *, #19922, .T. ) ;
#26161=FACE_OUTER_BOUND ( 'NONE', #38909, .T. ) ;
#26163=ADVANCED_FACE ( 'NONE', ( #50494 ), #46545, .T. ) ;
#26165=LINE ( 'NONE', #38769, #24609 ) ;
#26170=VECTOR ( 'NONE', #29475, 1000.000000000000000 ) ;
#26171=CIRCLE ( 'NONE', #38737, 125.0000000000000000 ) ;
#26174=ORIENTED_EDGE ( 'NONE', *, *, #32846, .T. ) ;
#26176=EDGE_CURVE ( 'NONE', #50211, #6218, #21859, .T. ) ;
#26177=DIRECTION ( 'NONE',  ( 0.4566292373937200777, 0.000000000000000000, -0.8896570909947436601 ) ) ;
#26179=EDGE_LOOP ( 'NONE', ( #30735, #6885, #32467, #12083 ) ) ;
#26180=ORIENTED_EDGE ( 'NONE', *, *, #31105, .T. ) ;
#26183=CARTESIAN_POINT ( 'NONE',  ( 9.518239912201957864, -213.5000000000000000, 110.7307791902283043 ) ) ;
#26184=DIRECTION ( 'NONE',  ( -0.000000000000000000, 1.000000000000000000, -0.000000000000000000 ) ) ;
#26185=ADVANCED_FACE ( 'NONE', ( #30252 ), #10277, .T. ) ;
#26186=EDGE_CURVE ( 'NONE', #7641, #38149, #20206, .T. ) ;
#26188=DIRECTION ( 'NONE',  ( -0.3482016354344059095, 0.000000000000000000, 0.9374196611341183427 ) ) ;
#26190=AXIS2_PLACEMENT_3D ( 'NONE', #5760, #9173, #41467 ) ;
#26191=ORIENTED_EDGE ( 'NONE', *, *, #45245, .F. ) ;
#26193=CYLINDRICAL_SURFACE ( 'NONE', #19001, 125.0000000000000000 ) ;
#26195=DIRECTION ( 'NONE',  ( 0.000000000000000000, -1.000000000000000000, 0.000000000000000000 ) ) ;
#26196=ORIENTED_EDGE ( 'NONE', *, *, #24433, .T. ) ;
#26200=CARTESIAN_POINT ( 'NONE',  ( -19.92568551777506869, -189.7472609257535510, -121.6951149130962904 ) ) ;
#26201=ORIENTED_EDGE ( 'NONE', *, *, #4550, .F. ) ;
#26202=DIRECTION ( 'NONE',  ( -0.6068001458186002006, 0.000000000000000000, 0.7948544414133481562 ) ) ;
#26203=CARTESIAN_POINT ( 'NONE',  ( -47.50057025920934706, -175.3837268820161057, 0.2059786187411091207 ) ) ;
#26204=EDGE_LOOP ( 'NONE', ( #49611, #33862, #17746, #37945 ) ) ;
#26205=CARTESIAN_POINT ( 'NONE',  ( -168.1141659785444915, -193.5000000000000000, -36.22785377503943494 ) ) ;
#26206=ORIENTED_EDGE ( 'NONE', *, *, #45941, .F. ) ;
#26207=CIRCLE ( 'NONE', #7758, 125.0000000000000000 ) ;
#26208=CIRCLE ( 'NONE', #20357, 125.0000000000000000 ) ;
#26209=EDGE_LOOP ( 'NONE', ( #40162, #16119, #24741, #50542 ) ) ;
#26211=AXIS2_PLACEMENT_3D ( 'NONE', #48802, #24357, #953 ) ;
#26212=CARTESIAN_POINT ( 'NONE',  ( 73.32083127613157103, -183.6283474603465606, 28.10285082451656535 ) ) ;
#26215=EDGE_LOOP ( 'NONE', ( #23557, #36469, #11309, #24009 ) ) ;
#26217=CARTESIAN_POINT ( 'NONE',  ( -172.4422607493951318, -193.5000000000000000, 16.06677968424543579 ) ) ;
#26218=CARTESIAN_POINT ( 'NONE',  ( 24.15597040328006884, -177.1207230881787780, -101.7307360698544016 ) ) ;
#26219=DIRECTION ( 'NONE',  ( -0.000000000000000000, 1.000000000000000000, -0.000000000000000000 ) ) ;
#26220=ORIENTED_EDGE ( 'NONE', *, *, #37525, .T. ) ;
#26222=DIRECTION ( 'NONE',  ( 0.000000000000000000, 0.000000000000000000, 1.000000000000000000 ) ) ;
#26223=DIRECTION ( 'NONE',  ( 0.000000000000000000, 0.000000000000000000, -1.000000000000000000 ) ) ;
#26224=ORIENTED_EDGE ( 'NONE', *, *, #38374, .T. ) ;
#26225=FACE_OUTER_BOUND ( 'NONE', #5, .T. ) ;
#26227=EDGE_CURVE ( 'NONE', #24430, #12390, #38642, .T. ) ;
#26229=EDGE_CURVE ( 'NONE', #28974, #41796, #1627, .T. ) ;
#26234=EDGE_CURVE ( 'NONE', #34277, #50878, #47584, .T. ) ;
#26235=CIRCLE ( 'NONE', #35459, 125.0000000000000000 ) ;
#26237=CARTESIAN_POINT ( 'NONE',  ( -124.4642912599203726, -175.3837268820161057, 99.25348746834863789 ) ) ;
#26239=EDGE_CURVE ( 'NONE', #39687, #4324, #31017, .T. ) ;
#26241=EDGE_CURVE ( 'NONE', #6939, #10029, #11038, .T. ) ;
#26242=CARTESIAN_POINT ( 'NONE',  ( 55.91309001144630031, -177.1207230881787780, 68.75510947788670535 ) ) ;
#26244=ORIENTED_EDGE ( 'NONE', *, *, #34796, .F. ) ;
#26247=ORIENTED_EDGE ( 'NONE', *, *, #15342, .F. ) ;
#26249=VECTOR ( 'NONE', #5515, 1000.000000000000114 ) ;
#26252=VERTEX_POINT ( 'NONE', #3169 ) ;
#26253=CARTESIAN_POINT ( 'NONE',  ( 74.28166149629942083, -193.5000000000000000, 17.48697739784543614 ) ) ;
#26254=EDGE_CURVE ( 'NONE', #20806, #14667, #27064, .T. ) ;
#26258=ORIENTED_EDGE ( 'NONE', *, *, #15943, .F. ) ;
#26259=FACE_OUTER_BOUND ( 'NONE', #42211, .T. ) ;
#26262=DIRECTION ( 'NONE',  ( -0.9929810960135185827, 0.000000000000000000, 0.1182731709213523247 ) ) ;
#26265=AXIS2_PLACEMENT_3D ( 'NONE', #31196, #47247, #11218 ) ;
#26266=ORIENTED_EDGE ( 'NONE', *, *, #41475, .F. ) ;
#26268=CARTESIAN_POINT ( 'NONE',  ( -48.41988612361515010, -193.5000000000000000, 0.9982437317643287900 ) ) ;
#26271=ADVANCED_FACE ( 'NONE', ( #7622 ), #23403, .T. ) ;
#26272=ORIENTED_EDGE ( 'NONE', *, *, #34317, .T. ) ;
#26273=AXIS2_PLACEMENT_3D ( 'NONE', #36326, #36070, #28170 ) ;
#26274=PLANE ( 'NONE',  #3896 ) ;
#26275=EDGE_LOOP ( 'NONE', ( #8298, #45072, #21912, #33256 ) ) ;
#26276=CARTESIAN_POINT ( 'NONE',  ( -47.70260288879081401, -193.5000000000000000, 0.6300878435817218737 ) ) ;
#26277=DIRECTION ( 'NONE',  ( -0.7765238627180482966, 0.000000000000000000, 0.6300878435817038881 ) ) ;
#26278=EDGE_LOOP ( 'NONE', ( #49564, #45555, #38734, #35672 ) ) ;
#26279=LINE ( 'NONE', #34683, #39794 ) ;
#26285=VECTOR ( 'NONE', #8979, 1000.000000000000000 ) ;
#26288=EDGE_CURVE ( 'NONE', #716, #39966, #19444, .T. ) ;
#26289=FACE_OUTER_BOUND ( 'NONE', #47991, .T. ) ;
#26290=VERTEX_POINT ( 'NONE', #51269 ) ;
#26292=FACE_OUTER_BOUND ( 'NONE', #12570, .T. ) ;
#26294=EDGE_CURVE ( 'NONE', #246, #48253, #32041, .T. ) ;
#26295=DIRECTION ( 'NONE',  ( 0.000000000000000000, 0.000000000000000000, 1.000000000000000000 ) ) ;
#26297=FACE_OUTER_BOUND ( 'NONE', #50602, .T. ) ;
#26298=ADVANCED_FACE ( 'NONE', ( #47322 ), #2904, .T. ) ;
#26299=ADVANCED_FACE ( 'NONE', ( #31269 ), #11291, .T. ) ;
#26303=CYLINDRICAL_SURFACE ( 'NONE', #40533, 124.9999999999999858 ) ;
#26304=ADVANCED_FACE ( 'NONE', ( #31528 ), #11569, .T. ) ;
#26305=PLANE ( 'NONE',  #50531 ) ;
#26306=FACE_OUTER_BOUND ( 'NONE', #4128, .T. ) ;
#26308=VECTOR ( 'NONE', #8648, 1000.000000000000000 ) ;
#26311=CARTESIAN_POINT ( 'NONE',  ( 42.89728982752370001, -193.5000000000000000, 83.82333043185313670 ) ) ;
#26314=DIRECTION ( 'NONE',  ( -0.000000000000000000, 1.000000000000000000, -0.000000000000000000 ) ) ;
#26315=DIRECTION ( 'NONE',  ( 0.1182731709213730997, 0.000000000000000000, -0.9929810960135161402 ) ) ;
#26317=VERTEX_POINT ( 'NONE', #17345 ) ;
#26318=EDGE_CURVE ( 'NONE', #36451, #48105, #12853, .T. ) ;
#26319=VERTEX_POINT ( 'NONE', #36245 ) ;
#26321=ADVANCED_FACE ( 'NONE', ( #8918 ), #1286, .T. ) ;
#26323=DIRECTION ( 'NONE',  ( 0.000000000000000000, -1.000000000000000000, 0.000000000000000000 ) ) ;
#26325=ORIENTED_EDGE ( 'NONE', *, *, #16012, .F. ) ;
#26327=CARTESIAN_POINT ( 'NONE',  ( -48.77118352214581876, -175.3837268820161057, -0.9564009842765195391 ) ) ;
#26328=LINE ( 'NONE', #10558, #42859 ) ;
#26330=CARTESIAN_POINT ( 'NONE',  ( 25.43954814678888710, -183.6283474603465606, 100.8019320314832754 ) ) ;
#26331=EDGE_LOOP ( 'NONE', ( #17510, #26258, #31374, #20382 ) ) ;
#26333=FACE_OUTER_BOUND ( 'NONE', #44566, .T. ) ;
#26334=ORIENTED_EDGE ( 'NONE', *, *, #45334, .F. ) ;
#26335=CARTESIAN_POINT ( 'NONE',  ( -60.86541030502398542, -183.6283474603465606, -124.3848060646151623 ) ) ;
#26336=EDGE_LOOP ( 'NONE', ( #909, #37780, #29056, #48141 ) ) ;
#26337=CARTESIAN_POINT ( 'NONE',  ( -165.2002711502080672, -177.1207230881787780, 44.73448837594995098 ) ) ;
#26338=CARTESIAN_POINT ( 'NONE',  ( -52.47502265695599988, -183.6283474603465606, -124.9361149384469485 ) ) ;
#26340=EDGE_CURVE ( 'NONE', #22344, #24544, #11826, .T. ) ;
#26343=DIRECTION ( 'NONE',  ( -0.000000000000000000, 1.000000000000000000, -0.000000000000000000 ) ) ;
#26345=ORIENTED_EDGE ( 'NONE', *, *, #50042, .T. ) ;
#26346=DIRECTION ( 'NONE',  ( -0.7175072570443299380, 0.000000000000000000, -0.6965510290629983725 ) ) ;
#26348=FACE_OUTER_BOUND ( 'NONE', #28017, .T. ) ;
#26349=AXIS2_PLACEMENT_3D ( 'NONE', #50109, #37486, #1743 ) ;
#26352=DIRECTION ( 'NONE',  ( 0.000000000000000000, -1.000000000000000000, 0.000000000000000000 ) ) ;
#26353=AXIS2_PLACEMENT_3D ( 'NONE', #36174, #36427, #24112 ) ;
#26356=ORIENTED_EDGE ( 'NONE', *, *, #933, .F. ) ;
#26358=DIRECTION ( 'NONE',  ( 0.000000000000000000, -0.000000000000000000, 1.000000000000000000 ) ) ;
#26359=ORIENTED_EDGE ( 'NONE', *, *, #38055, .F. ) ;
#26363=CARTESIAN_POINT ( 'NONE',  ( -161.4019114581580823, -175.3837268820161057, 53.60452120946281696 ) ) ;
#26364=EDGE_CURVE ( 'NONE', #19097, #14965, #41206, .T. ) ;
#26367=DIRECTION ( 'NONE',  ( 0.000000000000000000, 1.000000000000000000, -0.000000000000000000 ) ) ;
#26371=CARTESIAN_POINT ( 'NONE',  ( -15.24927435600541692, -193.5000000000000000, 120.5021863277719234 ) ) ;
#26375=CARTESIAN_POINT ( 'NONE',  ( -73.94077438226446475, -183.6283474603465606, 122.3793467049372481 ) ) ;
#26378=DIRECTION ( 'NONE',  ( 0.3482016354343866471, 0.000000000000000000, 0.9374196611341253371 ) ) ;
#26380=ORIENTED_EDGE ( 'NONE', *, *, #51421, .F. ) ;
#26381=LINE ( 'NONE', #50321, #11575 ) ;
#26384=VECTOR ( 'NONE', #42578, 1000.000000000000000 ) ;
#26386=DIRECTION ( 'NONE',  ( -0.000000000000000000, 1.000000000000000000, -0.000000000000000000 ) ) ;
#26388=ORIENTED_EDGE ( 'NONE', *, *, #38951, .F. ) ;
#26389=AXIS2_PLACEMENT_3D ( 'NONE', #43742, #31392, #4580 ) ;
#26390=EDGE_CURVE ( 'NONE', #5817, #13416, #37028, .T. ) ;
#26391=EDGE_LOOP ( 'NONE', ( #22835, #50290, #21088, #22964 ) ) ;
#26392=DIRECTION ( 'NONE',  ( -1.000000000000000000, 0.000000000000000000, 4.884776371667510679E-16 ) ) ;
#26393=DIRECTION ( 'NONE',  ( -0.2348860457809707758, 0.000000000000000000, -0.9720229140804138579 ) ) ;
#26394=DIRECTION ( 'NONE',  ( 0.8124868780056783146, 0.000000000000000000, 0.5829794791144762289 ) ) ;
#26395=DIRECTION ( 'NONE',  ( 0.000000000000000000, 0.000000000000000000, 1.000000000000000000 ) ) ;
#26396=VERTEX_POINT ( 'NONE', #40440 ) ;
#26398=DIRECTION ( 'NONE',  ( 0.000000000000000000, 0.000000000000000000, 1.000000000000000000 ) ) ;
#26399=ORIENTED_EDGE ( 'NONE', *, *, #34059, .T. ) ;
#26402=DIRECTION ( 'NONE',  ( 0.2348860457809842095, 0.000000000000000000, -0.9720229140804107493 ) ) ;
#26404=CARTESIAN_POINT ( 'NONE',  ( -158.9435005891547803, -183.6283474603465606, -56.33604425924762182 ) ) ;
#26405=ORIENTED_EDGE ( 'NONE', *, *, #27279, .F. ) ;
#26407=VERTEX_POINT ( 'NONE', #13385 ) ;
#26409=VECTOR ( 'NONE', #42775, 1000.000000000000000 ) ;
#26410=CARTESIAN_POINT ( 'NONE',  ( 68.24201764719070695, -193.5000000000000000, -44.73448837594909833 ) ) ;
#26411=ORIENTED_EDGE ( 'NONE', *, *, #28260, .F. ) ;
#26412=AXIS2_PLACEMENT_3D ( 'NONE', #14263, #22402, #38426 ) ;
#26414=FACE_OUTER_BOUND ( 'NONE', #12748, .T. ) ;
#26415=DIRECTION ( 'NONE',  ( 0.000000000000000000, 0.000000000000000000, -1.000000000000000000 ) ) ;
#26416=DIRECTION ( 'NONE',  ( 0.9027978299657446470, 0.000000000000000000, -0.4300652022765183435 ) ) ;
#26417=EDGE_CURVE ( 'NONE', #22639, #1324, #18523, .T. ) ;
#26420=CARTESIAN_POINT ( 'NONE',  ( -48.47912675150885065, -189.7472609257535510, 6.938893903907228378E-15 ) ) ;
#26421=VERTEX_POINT ( 'NONE', #48350 ) ;
#26423=DIRECTION ( 'NONE',  ( -0.9473263538541899509, 0.000000000000000000, -0.3202698538628415692 ) ) ;
#26425=CIRCLE ( 'NONE', #32310, 125.0000000000000000 ) ;
#26428=CIRCLE ( 'NONE', #14668, 125.0000000000000000 ) ;
#26431=CARTESIAN_POINT ( 'NONE',  ( -170.7635349987907034, -189.7472609257535510, -25.91377046305883169 ) ) ;
#26432=ORIENTED_EDGE ( 'NONE', *, *, #41548, .T. ) ;
#26433=CYLINDRICAL_SURFACE ( 'NONE', #20045, 125.0000000000000000 ) ;
#26435=EDGE_CURVE ( 'NONE', #32675, #41833, #16019, .T. ) ;
#26437=CARTESIAN_POINT ( 'NONE',  ( -172.9701362814535912, -175.3837268820161057, -11.26891947860193177 ) ) ;
#26438=CARTESIAN_POINT ( 'NONE',  ( -48.47912675150885065, -175.3837268820161057, 6.938893903907228378E-15 ) ) ;
#26440=ORIENTED_EDGE ( 'NONE', *, *, #49031, .F. ) ;
#26442=VERTEX_POINT ( 'NONE', #4994 ) ;
#26444=CARTESIAN_POINT ( 'NONE',  ( 76.28370911321322012, -177.1207230881787780, -7.696413904697510411 ) ) ;
#26447=VECTOR ( 'NONE', #35323, 1000.000000000000000 ) ;
#26449=CARTESIAN_POINT ( 'NONE',  ( -49.35486169370448550, -193.5000000000000000, -0.4827922027307481878 ) ) ;
#26450=VERTEX_POINT ( 'NONE', #29142 ) ;
#26452=VECTOR ( 'NONE', #18801, 1000.000000000000000 ) ;
#26453=DIRECTION ( 'NONE',  ( -0.000000000000000000, 1.000000000000000000, 0.000000000000000000 ) ) ;
#26457=VERTEX_POINT ( 'NONE', #12595 ) ;
#26458=CARTESIAN_POINT ( 'NONE',  ( 36.84288420123323249, -183.6283474603465606, 91.35181687837503262 ) ) ;
#26459=AXIS2_PLACEMENT_3D ( 'NONE', #3852, #35637, #19876 ) ;
#26460=ORIENTED_EDGE ( 'NONE', *, *, #7952, .F. ) ;
#26462=AXIS2_PLACEMENT_3D ( 'NONE', #21190, #29584, #29328 ) ;
#26463=EDGE_CURVE ( 'NONE', #18846, #16398, #25236, .T. ) ;
#26464=LINE ( 'NONE', #21767, #51513 ) ;
#26465=LINE ( 'NONE', #1780, #20901 ) ;
#26467=CARTESIAN_POINT ( 'NONE',  ( 18.49541618049843095, -177.1207230881787780, 105.5434062319798159 ) ) ;
#26468=VECTOR ( 'NONE', #42814, 1000.000000000000000 ) ;
#26470=EDGE_CURVE ( 'NONE', #40253, #11142, #20225, .T. ) ;
#26472=ORIENTED_EDGE ( 'NONE', *, *, #36863, .T. ) ;
#26474=CARTESIAN_POINT ( 'NONE',  ( 71.44208735029287993, -183.6283474603465606, 35.26900067126700833 ) ) ;
#26475=PLANE ( 'NONE',  #36640 ) ;
#26476=EDGE_LOOP ( 'NONE', ( #26244, #14023, #15742, #43902 ) ) ;
#26478=DIRECTION ( 'NONE',  ( 0.000000000000000000, 0.000000000000000000, -1.000000000000000000 ) ) ;
#26479=PLANE ( 'NONE',  #17923 ) ;
#26480=CARTESIAN_POINT ( 'NONE',  ( -173.2419626162308361, -177.1207230881787780, 7.696413904698415465 ) ) ;
#26481=EDGE_CURVE ( 'NONE', #51204, #10929, #17081, .T. ) ;
#26483=LINE ( 'NONE', #34384, #10399 ) ;
#26484=CARTESIAN_POINT ( 'NONE',  ( 58.95724912996274725, -183.6283474603465606, 61.91627321685103169 ) ) ;
#26486=FACE_BOUND ( 'NONE', #24166, .T. ) ;
#26487=EDGE_LOOP ( 'NONE', ( #41947, #37323, #31894, #7938 ) ) ;
#26488=ADVANCED_FACE ( 'NONE', ( #241 ), #29659, .F. ) ;
#26489=AXIS2_PLACEMENT_3D ( 'NONE', #38054, #10457, #22567 ) ;
#26490=DIRECTION ( 'NONE',  ( -0.8124868780056742068, 0.000000000000000000, -0.5829794791144820021 ) ) ;
#26491=CIRCLE ( 'NONE', #17280, 125.0000000000000000 ) ;
#26492=VECTOR ( 'NONE', #18681, 1000.000000000000000 ) ;
#26493=CARTESIAN_POINT ( 'NONE',  ( 76.46082103836693022, -193.5000000000000000, 3.874202661595785191 ) ) ;
#26499=VECTOR ( 'NONE', #11330, 1000.000000000000000 ) ;
#26500=DIRECTION ( 'NONE',  ( 0.000000000000000000, -0.000000000000000000, 1.000000000000000000 ) ) ;
#26501=EDGE_CURVE ( 'NONE', #10308, #27859, #4264, .T. ) ;
#26505=DIRECTION ( 'NONE',  ( -0.000000000000000000, 0.000000000000000000, 1.000000000000000000 ) ) ;
#26506=VERTEX_POINT ( 'NONE', #25467 ) ;
#26509=AXIS2_PLACEMENT_3D ( 'NONE', #35589, #51640, #31661 ) ;
#26510=LINE ( 'NONE', #42541, #11609 ) ;
#26511=EDGE_LOOP ( 'NONE', ( #26224, #10491, #23916, #23488 ) ) ;
#26512=DIRECTION ( 'NONE',  ( -0.2348860457809707758, 0.000000000000000000, -0.9720229140804138579 ) ) ;
#26513=CARTESIAN_POINT ( 'NONE',  ( -133.1483155860611021, -193.5000000000000000, -90.59430563621275212 ) ) ;
#26514=DIRECTION ( 'NONE',  ( -0.000000000000000000, 1.000000000000000000, -0.000000000000000000 ) ) ;
#26515=ORIENTED_EDGE ( 'NONE', *, *, #47534, .F. ) ;
#26517=CYLINDRICAL_SURFACE ( 'NONE', #19706, 125.0000000000000000 ) ;
#26519=AXIS2_PLACEMENT_3D ( 'NONE', #13041, #25147, #432 ) ;
#26520=AXIS2_PLACEMENT_3D ( 'NONE', #30946, #22805, #23065 ) ;
#26521=CARTESIAN_POINT ( 'NONE',  ( -77.67449977936063021, -175.3837268820161057, -121.5427093402339267 ) ) ;
#26522=AXIS2_PLACEMENT_3D ( 'NONE', #19954, #7604, #226 ) ;
#26523=VERTEX_POINT ( 'NONE', #42527 ) ;
#26524=LINE ( 'NONE', #22850, #14650 ) ;
#26525=VERTEX_POINT ( 'NONE', #30432 ) ;
#26526=VECTOR ( 'NONE', #42319, 1000.000000000000000 ) ;
#26527=ADVANCED_FACE ( 'NONE', ( #1558 ), #34132, .T. ) ;
#26528=EDGE_CURVE ( 'NONE', #11646, #5101, #48769, .T. ) ;
#26529=DIRECTION ( 'NONE',  ( 0.000000000000000000, 0.000000000000000000, -1.000000000000000000 ) ) ;
#26530=PLANE ( 'NONE',  #28271 ) ;
#26531=DIRECTION ( 'NONE',  ( -0.000000000000000000, 1.000000000000000000, -0.000000000000000000 ) ) ;
#26532=ORIENTED_EDGE ( 'NONE', *, *, #31124, .T. ) ;
#26533=ORIENTED_EDGE ( 'NONE', *, *, #13134, .T. ) ;
#26534=CARTESIAN_POINT ( 'NONE',  ( 57.31108707223381771, -189.7472609257535510, -66.58401203837752291 ) ) ;
#26535=ORIENTED_EDGE ( 'NONE', *, *, #37206, .T. ) ;
#26537=DIRECTION ( 'NONE',  ( -0.000000000000000000, 1.000000000000000000, -0.000000000000000000 ) ) ;
#26538=ORIENTED_EDGE ( 'NONE', *, *, #51045, .F. ) ;
#26539=CIRCLE ( 'NONE', #32430, 125.0000000000000000 ) ;
#26540=DIRECTION ( 'NONE',  ( -0.05924062789371441901, 0.000000000000000000, 0.9982437317643214625 ) ) ;
#26542=CARTESIAN_POINT ( 'NONE',  ( -60.86541030502395699, -177.1207230881787780, -124.3848060646151481 ) ) ;
#26543=CARTESIAN_POINT ( 'NONE',  ( 34.98161733638499271, -177.1207230881787780, -91.70840728318313495 ) ) ;
#26544=VECTOR ( 'NONE', #30608, 1000.000000000000000 ) ;
#26546=DIRECTION ( 'NONE',  ( 0.000000000000000000, -0.000000000000000000, 1.000000000000000000 ) ) ;
#26547=ORIENTED_EDGE ( 'NONE', *, *, #42310, .F. ) ;
#26548=ADVANCED_FACE ( 'NONE', ( #29925 ), #22297, .F. ) ;
#26549=VECTOR ( 'NONE', #17121, 1000.000000000000000 ) ;
#26551=CARTESIAN_POINT ( 'NONE',  ( -150.1390659022305840, -189.7472609257535510, 72.73415134496008250 ) ) ;
#26552=ADVANCED_FACE ( 'NONE', ( #6547 ), #17598, .T. ) ;
#26553=VECTOR ( 'NONE', #7657, 1000.000000000000000 ) ;
#26554=DIRECTION ( 'NONE',  ( 0.7378332790417189146, 0.000000000000000000, 0.6749830015182196608 ) ) ;
#26555=ORIENTED_EDGE ( 'NONE', *, *, #23986, .F. ) ;
#26557=DIRECTION ( 'NONE',  ( 0.9995608365087944591, 0.000000000000000000, -0.02963332782255633305 ) ) ;
#26558=DIRECTION ( 'NONE',  ( 0.000000000000000000, -0.000000000000000000, 1.000000000000000000 ) ) ;
#26559=EDGE_CURVE ( 'NONE', #37732, #37490, #46235, .T. ) ;
#26560=DIRECTION ( 'NONE',  ( 0.000000000000000000, -0.000000000000000000, 1.000000000000000000 ) ) ;
#26561=CARTESIAN_POINT ( 'NONE',  ( -139.0630283577175987, -183.6283474603465606, -86.13684908212448477 ) ) ;
#26562=ORIENTED_EDGE ( 'NONE', *, *, #39768, .F. ) ;
#26563=VECTOR ( 'NONE', #43441, 1000.000000000000000 ) ;
#26564=DIRECTION ( 'NONE',  ( -0.000000000000000000, 1.000000000000000000, -0.000000000000000000 ) ) ;
#26565=CARTESIAN_POINT ( 'NONE',  ( -137.6740394605055826, -177.1207230881787780, -86.14171647324863557 ) ) ;
#26566=CARTESIAN_POINT ( 'NONE',  ( 40.26790151320558664, -177.1207230881787780, -86.60307583628353711 ) ) ;
#26567=VECTOR ( 'NONE', #11203, 1000.000000000000000 ) ;
#26568=ORIENTED_EDGE ( 'NONE', *, *, #37914, .T. ) ;
#26569=LINE ( 'NONE', #14760, #28535 ) ;
#26570=DIRECTION ( 'NONE',  ( 0.000000000000000000, 0.000000000000000000, -1.000000000000000000 ) ) ;
#26572=CIRCLE ( 'NONE', #29080, 125.0000000000000000 ) ;
#26573=ORIENTED_EDGE ( 'NONE', *, *, #47196, .F. ) ;
#26577=VECTOR ( 'NONE', #32915, 1000.000000000000000 ) ;
#26578=VECTOR ( 'NONE', #32935, 1000.000000000000114 ) ;
#26579=FACE_OUTER_BOUND ( 'NONE', #1104, .T. ) ;
#26580=CIRCLE ( 'NONE', #1421, 125.0000000000000000 ) ;
#26581=CARTESIAN_POINT ( 'NONE',  ( -63.09433862318517328, -175.3837268820161057, -124.1426420773539689 ) ) ;
#26583=VECTOR ( 'NONE', #48389, 1000.000000000000000 ) ;
#26586=DIRECTION ( 'NONE',  ( -0.000000000000000000, 1.000000000000000000, -0.000000000000000000 ) ) ;
#26590=DIRECTION ( 'NONE',  ( 0.000000000000000000, 0.000000000000000000, 1.000000000000000000 ) ) ;
#26591=ORIENTED_EDGE ( 'NONE', *, *, #44358, .T. ) ;
#26595=EDGE_CURVE ( 'NONE', #46596, #16650, #42032, .T. ) ;
#26598=CARTESIAN_POINT ( 'NONE',  ( 69.99104047056317768, -193.5000000000000000, -39.87254040532513244 ) ) ;
#26599=CARTESIAN_POINT ( 'NONE',  ( -158.0280232639029236, -189.7472609257535510, 60.19999396110247858 ) ) ;
#26600=ADVANCED_FACE ( 'NONE', ( #38062 ), #34635, .F. ) ;
#26603=DIRECTION ( 'NONE',  ( 0.000000000000000000, 1.000000000000000000, -0.000000000000000000 ) ) ;
#26604=VECTOR ( 'NONE', #18431, 1000.000000000000000 ) ;
#26605=PLANE ( 'NONE',  #51909 ) ;
#26606=VERTEX_POINT ( 'NONE', #30688 ) ;
#26608=DIRECTION ( 'NONE',  ( 0.000000000000000000, 1.000000000000000000, 0.000000000000000000 ) ) ;
#26610=DIRECTION ( 'NONE',  ( 0.000000000000000000, -1.000000000000000000, 0.000000000000000000 ) ) ;
#26613=EDGE_CURVE ( 'NONE', #45175, #3688, #43303, .T. ) ;
#26617=CARTESIAN_POINT ( 'NONE',  ( 33.25242634436024503, -193.5000000000000000, -94.57776286494160445 ) ) ;
#26618=ORIENTED_EDGE ( 'NONE', *, *, #17028, .T. ) ;
#26620=EDGE_CURVE ( 'NONE', #50992, #3704, #7312, .T. ) ;
#26621=DIRECTION ( 'NONE',  ( -0.000000000000000000, 1.000000000000000000, -0.000000000000000000 ) ) ;
#26623=DIRECTION ( 'NONE',  ( 0.000000000000000000, 0.000000000000000000, -1.000000000000000000 ) ) ;
#26625=AXIS2_PLACEMENT_3D ( 'NONE', #32612, #11846, #281 ) ;
#26626=EDGE_CURVE ( 'NONE', #1404, #8692, #2840, .T. ) ;
#26627=CARTESIAN_POINT ( 'NONE',  ( -48.47912675150885065, -177.1207230881787780, 6.938893903907228378E-15 ) ) ;
#26628=DIRECTION ( 'NONE',  ( -0.000000000000000000, 1.000000000000000000, -0.000000000000000000 ) ) ;
#26629=LINE ( 'NONE', #47123, #26563 ) ;
#26630=AXIS2_PLACEMENT_3D ( 'NONE', #553, #24223, #37073 ) ;
#26633=CARTESIAN_POINT ( 'NONE',  ( -23.99795575808070325, -177.1207230881787780, -122.5792489240757561 ) ) ;
#26634=AXIS2_PLACEMENT_3D ( 'NONE', #42621, #51048, #14778 ) ;
#26635=ADVANCED_FACE ( 'NONE', ( #47264 ), #35158, .F. ) ;
#26638=CARTESIAN_POINT ( 'NONE',  ( -164.6246685127424882, -189.7472609257535510, -46.20836643930983456 ) ) ;
#26640=VERTEX_POINT ( 'NONE', #43814 ) ;
#26642=ADVANCED_FACE ( 'NONE', ( #15727 ), #3360, .T. ) ;
#26643=DIRECTION ( 'NONE',  ( 0.000000000000000000, -1.000000000000000000, 0.000000000000000000 ) ) ;
#26645=CIRCLE ( 'NONE', #3988, 125.0000000000000000 ) ;
#26646=VERTEX_POINT ( 'NONE', #3101 ) ;
#26647=CARTESIAN_POINT ( 'NONE',  ( -169.3144491972411458, -183.6283474603465606, -27.83926365844663664 ) ) ;
#26650=CARTESIAN_POINT ( 'NONE',  ( -172.7479958471414250, -193.5000000000000000, -13.49993235881364129 ) ) ;
#26651=VECTOR ( 'NONE', #42272, 1000.000000000000000 ) ;
#26652=LINE ( 'NONE', #51351, #40379 ) ;
#26656=ORIENTED_EDGE ( 'NONE', *, *, #14951, .F. ) ;
#26657=PLANE ( 'NONE',  #35020 ) ;
#26658=CARTESIAN_POINT ( 'NONE',  ( 56.81546028627039391, -175.3837268820161057, 65.49088066501711580 ) ) ;
#26660=VECTOR ( 'NONE', #20251, 1000.000000000000000 ) ;
#26662=DIRECTION ( 'NONE',  ( 0.000000000000000000, 1.000000000000000000, 0.000000000000000000 ) ) ;
#26663=DIRECTION ( 'NONE',  ( -0.000000000000000000, 1.000000000000000000, -0.000000000000000000 ) ) ;
#26664=ORIENTED_EDGE ( 'NONE', *, *, #9108, .F. ) ;
#26665=EDGE_CURVE ( 'NONE', #15769, #3536, #24443, .T. ) ;
#26667=VECTOR ( 'NONE', #16810, 1000.000000000000000 ) ;
#26668=CARTESIAN_POINT ( 'NONE',  ( -48.30901192927175458, -175.3837268820161057, -124.9998842437354227 ) ) ;
#26669=LINE ( 'NONE', #22723, #2208 ) ;
#26670=ADVANCED_FACE ( 'NONE', ( #14953 ), #47003, .T. ) ;
#26671=CIRCLE ( 'NONE', #35934, 125.0000000000000000 ) ;
#26672=ADVANCED_FACE ( 'NONE', ( #7563 ), #43047, .F. ) ;
#26673=ORIENTED_EDGE ( 'NONE', *, *, #35426, .F. ) ;
#26676=LINE ( 'NONE', #18527, #4025 ) ;
#26677=CARTESIAN_POINT ( 'NONE',  ( -48.47912675150885065, -183.6283474603465606, 6.938893903907228378E-15 ) ) ;
#26679=PLANE ( 'NONE',  #45293 ) ;
#26680=ORIENTED_EDGE ( 'NONE', *, *, #27543, .F. ) ;
#26681=CARTESIAN_POINT ( 'NONE',  ( -48.47912675150885065, -177.1207230881787780, 6.938893903907228378E-15 ) ) ;
#26683=DIRECTION ( 'NONE',  ( 0.2348860457809911206, 0.000000000000000000, -0.9720229140804089729 ) ) ;
#26685=EDGE_CURVE ( 'NONE', #51763, #32514, #31153, .T. ) ;
#26687=ORIENTED_EDGE ( 'NONE', *, *, #42248, .T. ) ;
#26689=PLANE ( 'NONE',  #27358 ) ;
#26691=DIRECTION ( 'NONE',  ( 0.8124868780056742068, 0.000000000000000000, 0.5829794791144820021 ) ) ;
#26694=CYLINDRICAL_SURFACE ( 'NONE', #8524, 125.0000000000000000 ) ;
#26696=CIRCLE ( 'NONE', #19976, 125.0000000000000000 ) ;
#26697=DIRECTION ( 'NONE',  ( 0.000000000000000000, 0.000000000000000000, 1.000000000000000000 ) ) ;
#26699=ORIENTED_EDGE ( 'NONE', *, *, #5117, .T. ) ;
#26700=CARTESIAN_POINT ( 'NONE',  ( -164.3791542526839464, -189.7472609257535510, 46.82076062204520639 ) ) ;
#26701=VERTEX_POINT ( 'NONE', #10733 ) ;
#26703=CARTESIAN_POINT ( 'NONE',  ( -145.6517069852672535, -175.3837268820161057, 78.62880929222943394 ) ) ;
#26704=VERTEX_POINT ( 'NONE', #26758 ) ;
#26707=ORIENTED_EDGE ( 'NONE', *, *, #44293, .F. ) ;
#26708=CARTESIAN_POINT ( 'NONE',  ( -129.9529520667707914, -175.3837268820161057, -94.79987230211960991 ) ) ;
#26710=FACE_OUTER_BOUND ( 'NONE', #515, .T. ) ;
#26711=VERTEX_POINT ( 'NONE', #45140 ) ;
#26713=EDGE_LOOP ( 'NONE', ( #2999, #18662, #24148, #28802 ) ) ;
#26715=CIRCLE ( 'NONE', #32569, 125.0000000000000000 ) ;
#26716=DIRECTION ( 'NONE',  ( -0.1476465640024779702, 0.000000000000000000, -0.9890401873221644768 ) ) ;
#26718=FACE_OUTER_BOUND ( 'NONE', #17235, .T. ) ;
#26723=VERTEX_POINT ( 'NONE', #36438 ) ;
#26724=CYLINDRICAL_SURFACE ( 'NONE', #41576, 125.0000000000000000 ) ;
#26725=VERTEX_POINT ( 'NONE', #32769 ) ;
#26726=AXIS2_PLACEMENT_3D ( 'NONE', #9649, #980, #5974 ) ;
#26727=ORIENTED_EDGE ( 'NONE', *, *, #21803, .T. ) ;
#26728=DIRECTION ( 'NONE',  ( 0.08879589532293853671, 0.000000000000000000, -0.9960498426152166740 ) ) ;
#26730=CARTESIAN_POINT ( 'NONE',  ( -48.47912675150885065, -213.5000000000000000, 6.938893903907228378E-15 ) ) ;
#26734=ORIENTED_EDGE ( 'NONE', *, *, #20922, .T. ) ;
#26735=CIRCLE ( 'NONE', #23367, 125.0000000000000000 ) ;
#26736=ORIENTED_EDGE ( 'NONE', *, *, #17617, .T. ) ;
#26737=CARTESIAN_POINT ( 'NONE',  ( 20.93410174202488250, -193.5000000000000000, -102.7511748916624725 ) ) ;
#26738=CARTESIAN_POINT ( 'NONE',  ( 68.79964045138289919, -193.5000000000000000, 43.25148278810711133 ) ) ;
#26740=DIRECTION ( 'NONE',  ( -0.000000000000000000, 1.000000000000000000, 0.000000000000000000 ) ) ;
#26742=EDGE_LOOP ( 'NONE', ( #34432, #8010, #21497, #28975 ) ) ;
#26744=LINE ( 'NONE', #42780, #23087 ) ;
#26746=CARTESIAN_POINT ( 'NONE',  ( 68.59638248015002659, -183.6283474603465606, -43.79868877201407429 ) ) ;
#26747=ORIENTED_EDGE ( 'NONE', *, *, #19919, .F. ) ;
#26748=CARTESIAN_POINT ( 'NONE',  ( -114.9451385648676478, -193.5000000000000000, -104.6823626202119470 ) ) ;
#26750=EDGE_CURVE ( 'NONE', #17878, #36957, #36179, .T. ) ;
#26751=FACE_BOUND ( 'NONE', #31610, .T. ) ;
#26754=AXIS2_PLACEMENT_3D ( 'NONE', #20529, #3997, #23695 ) ;
#26756=LINE ( 'NONE', #7562, #18881 ) ;
#26757=AXIS2_PLACEMENT_3D ( 'NONE', #23096, #1827, #14445 ) ;
#26758=CARTESIAN_POINT ( 'NONE',  ( 75.10200014432449223, -175.3837268820161057, 10.18383939837613639 ) ) ;
#26760=CARTESIAN_POINT ( 'NONE',  ( 17.98688506184921465, -183.6283474603465606, 104.6823626202124444 ) ) ;
#26762=ORIENTED_EDGE ( 'NONE', *, *, #8310, .T. ) ;
#26763=VECTOR ( 'NONE', #13846, 1000.000000000000114 ) ;
#26766=DIRECTION ( 'NONE',  ( 0.000000000000000000, 0.000000000000000000, 1.000000000000000000 ) ) ;
#26768=PLANE ( 'NONE',  #10956 ) ;
#26769=ORIENTED_EDGE ( 'NONE', *, *, #6763, .F. ) ;
#26770=VECTOR ( 'NONE', #27238, 1000.000000000000000 ) ;
#26774=FACE_OUTER_BOUND ( 'NONE', #21316, .T. ) ;
#26775=EDGE_LOOP ( 'NONE', ( #42760, #41243, #32972, #9159 ) ) ;
#26778=CARTESIAN_POINT ( 'NONE',  ( -173.4190745413846457, -175.3837268820161057, -3.874202661594927211 ) ) ;
#26780=CARTESIAN_POINT ( 'NONE',  ( 36.84288420123323249, -183.6283474603465606, 91.35181687837503262 ) ) ;
#26781=DIRECTION ( 'NONE',  ( -0.000000000000000000, 1.000000000000000000, -0.000000000000000000 ) ) ;
#26782=ORIENTED_EDGE ( 'NONE', *, *, #40521, .F. ) ;
#26783=EDGE_CURVE ( 'NONE', #22586, #875, #42895, .T. ) ;
#26784=CIRCLE ( 'NONE', #33518, 125.0000000000000000 ) ;
#26785=LINE ( 'NONE', #11006, #22274 ) ;
#26786=EDGE_LOOP ( 'NONE', ( #46788, #44500, #48325, #1844 ) ) ;
#26787=DIRECTION ( 'NONE',  ( 0.000000000000000000, 0.000000000000000000, 1.000000000000000000 ) ) ;
#26788=ORIENTED_EDGE ( 'NONE', *, *, #13377, .T. ) ;
#26792=ORIENTED_EDGE ( 'NONE', *, *, #25248, .F. ) ;
#26793=ORIENTED_EDGE ( 'NONE', *, *, #21336, .F. ) ;
#26794=DIRECTION ( 'NONE',  ( 0.000000000000000000, 1.000000000000000000, -0.000000000000000000 ) ) ;
#26795=ORIENTED_EDGE ( 'NONE', *, *, #16404, .F. ) ;
#26797=LINE ( 'NONE', #14724, #3009 ) ;
#26799=ADVANCED_FACE ( 'NONE', ( #9127 ), #16766, .T. ) ;
#26800=LINE ( 'NONE', #50479, #16300 ) ;
#26802=DIRECTION ( 'NONE',  ( 0.000000000000000000, -1.000000000000000000, 0.000000000000000000 ) ) ;
#26804=CARTESIAN_POINT ( 'NONE',  ( -34.63763967761165929, -193.5000000000000000, -123.2250735253142864 ) ) ;
#26806=CARTESIAN_POINT ( 'NONE',  ( -41.24387117724851493, -175.3837268820161057, 124.7904286264581231 ) ) ;
#26809=CARTESIAN_POINT ( 'NONE',  ( -48.02249751411514467, -175.3837268820161057, 0.8896570909947569827 ) ) ;
#26810=ORIENTED_EDGE ( 'NONE', *, *, #14448, .F. ) ;
#26811=CARTESIAN_POINT ( 'NONE',  ( 29.27398957514434130, -193.5000000000000000, -97.87467957287998388 ) ) ;
#26812=CARTESIAN_POINT ( 'NONE',  ( -48.47912675150885065, -177.1207230881787780, 6.938893903907228378E-15 ) ) ;
#26818=CARTESIAN_POINT ( 'NONE',  ( -48.47912675150885065, -175.3837268820161057, 6.938893903907228378E-15 ) ) ;
#26820=CARTESIAN_POINT ( 'NONE',  ( -80.17897391495031911, -183.6283474603465606, 120.9136869416132498 ) ) ;
#26821=PLANE ( 'NONE',  #39652 ) ;
#26822=FACE_OUTER_BOUND ( 'NONE', #24025, .T. ) ;
#26826=LINE ( 'NONE', #4875, #49545 ) ;
#26827=CARTESIAN_POINT ( 'NONE',  ( -47.53180039765466347, -189.7472609257535510, 0.3202698538628485636 ) ) ;
#26828=ORIENTED_EDGE ( 'NONE', *, *, #2209, .T. ) ;
#26830=ORIENTED_EDGE ( 'NONE', *, *, #6738, .T. ) ;
#26831=DIRECTION ( 'NONE',  ( -0.000000000000000000, 1.000000000000000000, -0.000000000000000000 ) ) ;
#26834=DIRECTION ( 'NONE',  ( 0.000000000000000000, -1.000000000000000000, -0.000000000000000000 ) ) ;
#26835=ORIENTED_EDGE ( 'NONE', *, *, #29172, .T. ) ;
#26836=EDGE_CURVE ( 'NONE', #6242, #20290, #24368, .T. ) ;
#26838=AXIS2_PLACEMENT_3D ( 'NONE', #40312, #39539, #28745 ) ;
#26839=LINE ( 'NONE', #38920, #40973 ) ;
#26840=CARTESIAN_POINT ( 'NONE',  ( 14.94072793302542124, -189.7472609257535510, 107.7168604805791574 ) ) ;
#26842=DIRECTION ( 'NONE',  ( 0.9960498426152177842, 0.000000000000000000, -0.08879589532292482545 ) ) ;
#26846=VERTEX_POINT ( 'NONE', #40632 ) ;
#26847=CARTESIAN_POINT ( 'NONE',  ( -173.3968853974275817, -189.7472609257535510, 4.533605064404221174 ) ) ;
#26848=ORIENTED_EDGE ( 'NONE', *, *, #25364, .F. ) ;
#26850=DIRECTION ( 'NONE',  ( 0.000000000000000000, 0.000000000000000000, 1.000000000000000000 ) ) ;
#26852=VERTEX_POINT ( 'NONE', #4654 ) ;
#26853=ORIENTED_EDGE ( 'NONE', *, *, #37505, .F. ) ;
#26854=DIRECTION ( 'NONE',  ( 0.000000000000000000, 0.000000000000000000, 1.000000000000000000 ) ) ;
#26857=ORIENTED_EDGE ( 'NONE', *, *, #35305, .F. ) ;
#26864=DIRECTION ( 'NONE',  ( -0.000000000000000000, 1.000000000000000000, -0.000000000000000000 ) ) ;
#26867=LINE ( 'NONE', #46872, #11075 ) ;
#26868=ORIENTED_EDGE ( 'NONE', *, *, #44217, .F. ) ;
#26872=VECTOR ( 'NONE', #36605, 1000.000000000000227 ) ;
#26873=ORIENTED_EDGE ( 'NONE', *, *, #27148, .T. ) ;
#26874=CIRCLE ( 'NONE', #37800, 125.0000000000000000 ) ;
#26876=CARTESIAN_POINT ( 'NONE',  ( 68.24201764719070695, -193.5000000000000000, -44.73448837594909833 ) ) ;
#26879=EDGE_LOOP ( 'NONE', ( #29327, #50636, #5915, #46533 ) ) ;
#26880=EDGE_CURVE ( 'NONE', #13363, #40758, #36720, .T. ) ;
#26881=EDGE_LOOP ( 'NONE', ( #12092, #3762, #35815, #45291 ) ) ;
#26882=EDGE_CURVE ( 'NONE', #26711, #23372, #47113, .T. ) ;
#26883=ADVANCED_FACE ( 'NONE', ( #10344 ), #34761, .T. ) ;
#26884=FACE_OUTER_BOUND ( 'NONE', #30857, .T. ) ;
#26885=EDGE_CURVE ( 'NONE', #42243, #29510, #38190, .T. ) ;
#26886=FACE_OUTER_BOUND ( 'NONE', #29355, .T. ) ;
#26887=ORIENTED_EDGE ( 'NONE', *, *, #14930, .F. ) ;
#26888=ORIENTED_EDGE ( 'NONE', *, *, #37550, .F. ) ;
#26891=EDGE_CURVE ( 'NONE', #39890, #21288, #42397, .T. ) ;
#26892=ORIENTED_EDGE ( 'NONE', *, *, #42569, .F. ) ;
#26893=DIRECTION ( 'NONE',  ( 0.6749830015182038956, 0.000000000000000000, 0.7378332790417333475 ) ) ;
#26894=DIRECTION ( 'NONE',  ( 0.000000000000000000, 0.000000000000000000, -1.000000000000000000 ) ) ;
#26896=EDGE_CURVE ( 'NONE', #27207, #33001, #49334, .T. ) ;
#26898=CARTESIAN_POINT ( 'NONE',  ( 19.33815737959698566, -183.6283474603465606, 105.0038855142078233 ) ) ;
#26899=ORIENTED_EDGE ( 'NONE', *, *, #40119, .F. ) ;
#26900=EDGE_LOOP ( 'NONE', ( #1989, #29728, #29569, #28364 ) ) ;
#26901=ADVANCED_FACE ( 'NONE', ( #22175 ), #22951, .T. ) ;
#26902=EDGE_LOOP ( 'NONE', ( #6525, #12923, #17616, #46576 ) ) ;
#26904=FACE_OUTER_BOUND ( 'NONE', #44707, .T. ) ;
#26905=DIRECTION ( 'NONE',  ( -0.000000000000000000, -1.000000000000000000, 0.000000000000000000 ) ) ;
#26906=DIRECTION ( 'NONE',  ( -0.8124868780056742068, 0.000000000000000000, -0.5829794791144820021 ) ) ;
#26907=EDGE_CURVE ( 'NONE', #27896, #15221, #38708, .T. ) ;
#26908=CARTESIAN_POINT ( 'NONE',  ( 72.68824389704326450, -189.7472609257535510, -26.35287080855459863 ) ) ;
#26909=CARTESIAN_POINT ( 'NONE',  ( -87.28630321566649286, -183.6283474603465606, 118.8234112238818341 ) ) ;
#26910=ORIENTED_EDGE ( 'NONE', *, *, #43159, .F. ) ;
#26911=AXIS2_PLACEMENT_3D ( 'NONE', #39779, #3290, #19324 ) ;
#26912=EDGE_CURVE ( 'NONE', #51763, #27930, #30311, .T. ) ;
#26913=DIRECTION ( 'NONE',  ( -0.000000000000000000, 1.000000000000000000, 0.000000000000000000 ) ) ;
#26914=DIRECTION ( 'NONE',  ( 0.000000000000000000, 1.000000000000000000, 0.000000000000000000 ) ) ;
#26916=ORIENTED_EDGE ( 'NONE', *, *, #25885, .T. ) ;
#26918=LINE ( 'NONE', #42947, #17299 ) ;
#26919=CARTESIAN_POINT ( 'NONE',  ( -48.47912675150885065, -175.3837268820161057, 6.938893903907228378E-15 ) ) ;
#26922=CARTESIAN_POINT ( 'NONE',  ( 38.71172987070728055, -193.5000000000000000, -89.56983042009262874 ) ) ;
#26925=DIRECTION ( 'NONE',  ( 0.000000000000000000, -1.000000000000000000, -0.000000000000000000 ) ) ;
#26926=EDGE_CURVE ( 'NONE', #29344, #28119, #46884, .T. ) ;
#26927=ORIENTED_EDGE ( 'NONE', *, *, #16997, .F. ) ;
#26928=LINE ( 'NONE', #9882, #36320 ) ;
#26929=AXIS2_PLACEMENT_3D ( 'NONE', #2483, #22710, #50571 ) ;
#26930=CARTESIAN_POINT ( 'NONE',  ( 38.01517884164424999, -175.3837268820161057, -88.85232316304831102 ) ) ;
#26931=VERTEX_POINT ( 'NONE', #7175 ) ;
#26932=CARTESIAN_POINT ( 'NONE',  ( -49.42645310536303782, -193.5000000000000000, -0.3202698538628417357 ) ) ;
#26933=DIRECTION ( 'NONE',  ( -0.7175072570443395970, 0.000000000000000000, 0.6965510290629882695 ) ) ;
#26935=LINE ( 'NONE', #9057, #6481 ) ;
#26938=ORIENTED_EDGE ( 'NONE', *, *, #5649, .T. ) ;
#26942=CIRCLE ( 'NONE', #35312, 125.0000000000000000 ) ;
#26944=EDGE_LOOP ( 'NONE', ( #32060, #50715, #37632, #35725 ) ) ;
#26947=EDGE_CURVE ( 'NONE', #1492, #40253, #14403, .T. ) ;
#26948=ORIENTED_EDGE ( 'NONE', *, *, #19209, .F. ) ;
#26950=AXIS2_PLACEMENT_3D ( 'NONE', #11236, #42788, #46746 ) ;
#26951=DIRECTION ( 'NONE',  ( -0.000000000000000000, -1.000000000000000000, 0.000000000000000000 ) ) ;
#26952=EDGE_LOOP ( 'NONE', ( #47459, #7978, #24324, #1336, #28106, #17703, #28842, #32266, #31036, #35943, #32194, #10955, #21240, #21595, #35321, #13472 ) ) ;
#26953=AXIS2_PLACEMENT_3D ( 'NONE', #119, #51651, #32703 ) ;
#26956=VERTEX_POINT ( 'NONE', #27135 ) ;
#26957=DIRECTION ( 'NONE',  ( -0.9646355819083614058, 0.000000000000000000, 0.2635871660690581320 ) ) ;
#26958=ADVANCED_FACE ( 'NONE', ( #14557 ), #30562, .F. ) ;
#26960=DIRECTION ( 'NONE',  ( 0.000000000000000000, 0.000000000000000000, 1.000000000000000000 ) ) ;
#26961=ORIENTED_EDGE ( 'NONE', *, *, #8460, .T. ) ;
#26963=VERTEX_POINT ( 'NONE', #13322 ) ;
#26967=ADVANCED_FACE ( 'NONE', ( #29341 ), #45391, .T. ) ;
#26968=DIRECTION ( 'NONE',  ( -0.2059786187411094538, 0.000000000000000000, 0.9785564922995017012 ) ) ;
#26973=ADVANCED_FACE ( 'NONE', ( #31597 ), #43445, .T. ) ;
#26974=DIRECTION ( 'NONE',  ( 0.000000000000000000, 1.000000000000000000, 0.000000000000000000 ) ) ;
#26975=ORIENTED_EDGE ( 'NONE', *, *, #44287, .F. ) ;
#26981=FACE_OUTER_BOUND ( 'NONE', #47269, .T. ) ;
#26982=AXIS2_PLACEMENT_3D ( 'NONE', #48557, #958, #12532 ) ;
#26983=PLANE ( 'NONE',  #1874 ) ;
#26984=LINE ( 'NONE', #38807, #25104 ) ;
#26988=CIRCLE ( 'NONE', #51357, 125.0000000000000000 ) ;
#26989=EDGE_CURVE ( 'NONE', #38808, #51354, #11879, .T. ) ;
#26990=ORIENTED_EDGE ( 'NONE', *, *, #4011, .F. ) ;
#26992=FACE_OUTER_BOUND ( 'NONE', #51315, .T. ) ;
#26993=LINE ( 'NONE', #43029, #50087 ) ;
#26994=ORIENTED_EDGE ( 'NONE', *, *, #1872, .F. ) ;
#26995=DIRECTION ( 'NONE',  ( 0.9646355819083576311, 0.000000000000000000, 0.2635871660690715101 ) ) ;
#26996=DIRECTION ( 'NONE',  ( -0.8455960035018199594, 0.000000000000000000, -0.5338233779648003940 ) ) ;
#26997=CARTESIAN_POINT ( 'NONE',  ( -74.33510315702939408, -183.6283474603465606, -121.2748789083719032 ) ) ;
#26998=CARTESIAN_POINT ( 'NONE',  ( -77.67449977936063021, -175.3837268820161057, -121.5427093402339267 ) ) ;
#26999=ORIENTED_EDGE ( 'NONE', *, *, #16335, .T. ) ;
#27002=VECTOR ( 'NONE', #19511, 1000.000000000000000 ) ;
#27004=EDGE_LOOP ( 'NONE', ( #29169, #41623, #34574, #50200 ) ) ;
#27005=AXIS2_PLACEMENT_3D ( 'NONE', #33573, #45668, #2550 ) ;
#27006=CARTESIAN_POINT ( 'NONE',  ( -59.86929868745820471, -177.1207230881787780, -124.4799742258549458 ) ) ;
#27007=DIRECTION ( 'NONE',  ( 0.000000000000000000, 0.000000000000000000, 1.000000000000000000 ) ) ;
#27011=VERTEX_POINT ( 'NONE', #31338 ) ;
#27012=PLANE ( 'NONE',  #24280 ) ;
#27013=FACE_BOUND ( 'NONE', #25878, .T. ) ;
#27016=AXIS2_PLACEMENT_3D ( 'NONE', #43937, #15575, #31589 ) ;
#27017=DIRECTION ( 'NONE',  ( -0.05924062789371441901, 0.000000000000000000, 0.9982437317643214625 ) ) ;
#27019=VECTOR ( 'NONE', #12864, 1000.000000000000000 ) ;
#27020=ORIENTED_EDGE ( 'NONE', *, *, #30115, .T. ) ;
#27023=EDGE_CURVE ( 'NONE', #4313, #46169, #15320, .T. ) ;
#27027=DIRECTION ( 'NONE',  ( 0.000000000000000000, -0.000000000000000000, 1.000000000000000000 ) ) ;
#27031=DIRECTION ( 'NONE',  ( -0.000000000000000000, 1.000000000000000000, 0.000000000000000000 ) ) ;
#27032=ORIENTED_EDGE ( 'NONE', *, *, #946, .T. ) ;
#27034=VECTOR ( 'NONE', #43195, 1000.000000000000000 ) ;
#27035=DIRECTION ( 'NONE',  ( -0.000000000000000000, 1.000000000000000000, -0.000000000000000000 ) ) ;
#27036=ORIENTED_EDGE ( 'NONE', *, *, #35633, .F. ) ;
#27038=ORIENTED_EDGE ( 'NONE', *, *, #3742, .T. ) ;
#27039=DIRECTION ( 'NONE',  ( -0.000000000000000000, 1.000000000000000000, -0.000000000000000000 ) ) ;
#27040=ORIENTED_EDGE ( 'NONE', *, *, #19825, .T. ) ;
#27041=CARTESIAN_POINT ( 'NONE',  ( 67.42090074966655777, -189.7472609257535510, -46.82076062204440348 ) ) ;
#27043=ORIENTED_EDGE ( 'NONE', *, *, #43033, .T. ) ;
#27044=DIRECTION ( 'NONE',  ( 0.7378332790417239107, 0.000000000000000000, 0.6749830015182142207 ) ) ;
#27046=CARTESIAN_POINT ( 'NONE',  ( 71.44208735029287993, -177.1207230881787780, 35.26900067126700833 ) ) ;
#27047=CARTESIAN_POINT ( 'NONE',  ( -105.8382074681672975, -189.7472609257535510, -109.9360785596604728 ) ) ;
#27050=LINE ( 'NONE', #47050, #45021 ) ;
#27051=FACE_OUTER_BOUND ( 'NONE', #22788, .T. ) ;
#27052=VECTOR ( 'NONE', #18601, 999.9999999999998863 ) ;
#27056=DIRECTION ( 'NONE',  ( -0.000000000000000000, 1.000000000000000000, -0.000000000000000000 ) ) ;
#27059=DIRECTION ( 'NONE',  ( 0.000000000000000000, 1.000000000000000000, 0.000000000000000000 ) ) ;
#27061=DIRECTION ( 'NONE',  ( 0.000000000000000000, -1.000000000000000000, 0.000000000000000000 ) ) ;
#27063=CARTESIAN_POINT ( 'NONE',  ( -164.0008810331606810, -189.7472609257535510, 47.74645837849822527 ) ) ;
#27064=LINE ( 'NONE', #3417, #36145 ) ;
#27066=ADVANCED_FACE ( 'NONE', ( #3245 ), #16102, .F. ) ;
#27067=ORIENTED_EDGE ( 'NONE', *, *, #31193, .F. ) ;
#27069=VECTOR ( 'NONE', #22490, 1000.000000000000000 ) ;
#27070=AXIS2_PLACEMENT_3D ( 'NONE', #23069, #43556, #39078 ) ;
#27071=FACE_OUTER_BOUND ( 'NONE', #23312, .T. ) ;
#27073=PLANE ( 'NONE',  #13971 ) ;
#27075=LINE ( 'NONE', #30002, #14514 ) ;
#27076=FACE_OUTER_BOUND ( 'NONE', #6981, .T. ) ;
#27080=PLANE ( 'NONE',  #21293 ) ;
#27081=ORIENTED_EDGE ( 'NONE', *, *, #41028, .F. ) ;
#27082=ORIENTED_EDGE ( 'NONE', *, *, #34887, .F. ) ;
#27083=EDGE_LOOP ( 'NONE', ( #50722, #2872, #19419, #3051 ) ) ;
#27084=EDGE_CURVE ( 'NONE', #23558, #21890, #39481, .T. ) ;
#27085=CARTESIAN_POINT ( 'NONE',  ( -77.67449977936063021, -193.5000000000000000, -121.5427093402339267 ) ) ;
#27086=AXIS2_PLACEMENT_3D ( 'NONE', #4912, #44580, #33274 ) ;
#27088=ORIENTED_EDGE ( 'NONE', *, *, #25799, .F. ) ;
#27089=VECTOR ( 'NONE', #24562, 1000.000000000000000 ) ;
#27091=CARTESIAN_POINT ( 'NONE',  ( -48.02249751411514467, -189.7472609257535510, 0.8896570909947569827 ) ) ;
#27092=CARTESIAN_POINT ( 'NONE',  ( -48.47912675150885065, -175.3837268820161057, 6.938893903907228378E-15 ) ) ;
#27093=LINE ( 'NONE', #43130, #45098 ) ;
#27095=FACE_OUTER_BOUND ( 'NONE', #46199, .T. ) ;
#27096=EDGE_LOOP ( 'NONE', ( #606, #8729, #24541, #25322 ) ) ;
#27099=DIRECTION ( 'NONE',  ( 0.000000000000000000, 1.000000000000000000, 0.000000000000000000 ) ) ;
#27101=DIRECTION ( 'NONE',  ( -0.000000000000000000, 1.000000000000000000, -0.000000000000000000 ) ) ;
#27103=AXIS2_PLACEMENT_3D ( 'NONE', #16281, #9131, #48082 ) ;
#27105=ORIENTED_EDGE ( 'NONE', *, *, #8992, .T. ) ;
#27106=CARTESIAN_POINT ( 'NONE',  ( -49.47868758801764955, -193.5000000000000000, 0.02963332782255607284 ) ) ;
#27109=DIRECTION ( 'NONE',  ( 0.000000000000000000, 0.000000000000000000, -1.000000000000000000 ) ) ;
#27110=CARTESIAN_POINT ( 'NONE',  ( -49.47517659412406488, -183.6283474603465606, -0.08879589532293878651 ) ) ;
#27111=ORIENTED_EDGE ( 'NONE', *, *, #4493, .F. ) ;
#27112=CARTESIAN_POINT ( 'NONE',  ( 1.755575411425451593, -189.7472609257535510, 114.4616734920527108 ) ) ;
#27113=FACE_OUTER_BOUND ( 'NONE', #37194, .T. ) ;
#27114=EDGE_CURVE ( 'NONE', #12713, #14995, #51332, .T. ) ;
#27116=CARTESIAN_POINT ( 'NONE',  ( -159.3947744408687868, -193.5000000000000000, -55.44293326708444880 ) ) ;
#27117=AXIS2_PLACEMENT_3D ( 'NONE', #17786, #33027, #9906 ) ;
#27119=ADVANCED_FACE ( 'NONE', ( #31864 ), #4017, .T. ) ;
#27121=CARTESIAN_POINT ( 'NONE',  ( -48.47912675150885065, -189.7472609257535510, 6.938893903907228378E-15 ) ) ;
#27122=ORIENTED_EDGE ( 'NONE', *, *, #50685, .F. ) ;
#27124=DIRECTION ( 'NONE',  ( 0.9982437317643210184, 0.000000000000000000, 0.05924062789372143423 ) ) ;
#27127=PLANE ( 'NONE',  #34427 ) ;
#27129=CARTESIAN_POINT ( 'NONE',  ( 66.42899531795131907, -193.5000000000000000, 49.20491319441622124 ) ) ;
#27130=EDGE_CURVE ( 'NONE', #16977, #9440, #4266, .T. ) ;
#27132=AXIS2_PLACEMENT_3D ( 'NONE', #9182, #41476, #45196 ) ;
#27134=ADVANCED_FACE ( 'NONE', ( #28161 ), #44210, .T. ) ;
#27135=CARTESIAN_POINT ( 'NONE',  ( -102.5006284722403507, -183.6283474603465606, -112.7238987608084955 ) ) ;
#27136=DIRECTION ( 'NONE',  ( 0.000000000000000000, -1.000000000000000000, 0.000000000000000000 ) ) ;
#27138=EDGE_LOOP ( 'NONE', ( #47347, #28631, #44858, #11516 ) ) ;
#27142=DIRECTION ( 'NONE',  ( -0.1476465640024918202, 0.000000000000000000, 0.9890401873221624784 ) ) ;
#27144=CIRCLE ( 'NONE', #16246, 125.0000000000000000 ) ;
#27145=EDGE_LOOP ( 'NONE', ( #18256, #43072, #34462, #17570 ) ) ;
#27146=LINE ( 'NONE', #43179, #44095 ) ;
#27148=EDGE_CURVE ( 'NONE', #34929, #18995, #16357, .T. ) ;
#27152=CARTESIAN_POINT ( 'NONE',  ( -49.44376233341721161, -175.3837268820161057, 0.2635871660690650709 ) ) ;
#27153=ORIENTED_EDGE ( 'NONE', *, *, #19960, .F. ) ;
#27157=DIRECTION ( 'NONE',  ( -0.000000000000000000, 1.000000000000000000, -0.000000000000000000 ) ) ;
#27158=LINE ( 'NONE', #51881, #40864 ) ;
#27159=CARTESIAN_POINT ( 'NONE',  ( 69.04371411670898340, -175.3837268820161057, -39.55227055146230697 ) ) ;
#27163=CARTESIAN_POINT ( 'NONE',  ( -48.47912675150885065, -189.7472609257535510, 6.938893903907228378E-15 ) ) ;
#27164=DIRECTION ( 'NONE',  ( 0.3758275821142422202, 0.000000000000000000, -0.9266896074318318188 ) ) ;
#27165=CIRCLE ( 'NONE', #33885, 125.0000000000000000 ) ;
#27166=VERTEX_POINT ( 'NONE', #12400 ) ;
#27167=ORIENTED_EDGE ( 'NONE', *, *, #45282, .F. ) ;
#27169=LINE ( 'NONE', #41978, #24769 ) ;
#27170=LINE ( 'NONE', #10377, #2345 ) ;
#27176=DIRECTION ( 'NONE',  ( -0.9995608365087942371, 0.000000000000000000, -0.02963332782256331357 ) ) ;
#27177=VERTEX_POINT ( 'NONE', #5055 ) ;
#27179=VECTOR ( 'NONE', #48308, 1000.000000000000114 ) ;
#27180=ORIENTED_EDGE ( 'NONE', *, *, #20019, .F. ) ;
#27181=DIRECTION ( 'NONE',  ( 0.000000000000000000, 0.000000000000000000, 1.000000000000000000 ) ) ;
#27182=CARTESIAN_POINT ( 'NONE',  ( 61.69163308845453031, -193.5000000000000000, -56.90809649257490577 ) ) ;
#27184=LINE ( 'NONE', #2262, #15640 ) ;
#27186=PLANE ( 'NONE',  #13960 ) ;
#27187=EDGE_CURVE ( 'NONE', #17378, #39607, #19450, .T. ) ;
#27190=CARTESIAN_POINT ( 'NONE',  ( 72.14504940832446778, -175.3837268820161057, -32.78426643622660208 ) ) ;
#27192=EDGE_CURVE ( 'NONE', #7467, #39853, #40771, .T. ) ;
#27193=DIRECTION ( 'NONE',  ( -0.000000000000000000, 1.000000000000000000, -0.000000000000000000 ) ) ;
#27194=CYLINDRICAL_SURFACE ( 'NONE', #23741, 125.0000000000000000 ) ;
#27196=VECTOR ( 'NONE', #20849, 1000.000000000000000 ) ;
#27197=ADVANCED_FACE ( 'NONE', ( #16631 ), #32639, .T. ) ;
#27200=CARTESIAN_POINT ( 'NONE',  ( -132.4142998968130769, -177.1207230881787780, -91.27439114664585418 ) ) ;
#27201=VERTEX_POINT ( 'NONE', #37629 ) ;
#27202=VECTOR ( 'NONE', #646, 1000.000000000000000 ) ;
#27203=DIRECTION ( 'NONE',  ( 0.000000000000000000, -1.000000000000000000, 0.000000000000000000 ) ) ;
#27205=CARTESIAN_POINT ( 'NONE',  ( 46.31065297101394407, -177.1207230881787780, 79.94433946042836681 ) ) ;
#27207=VERTEX_POINT ( 'NONE', #48939 ) ;
#27208=CARTESIAN_POINT ( 'NONE',  ( -7.223120065443615623, -183.6283474603465606, 117.9955164924470523 ) ) ;
#27209=DIRECTION ( 'NONE',  ( 0.1182731709213592358, 0.000000000000000000, 0.9929810960135178055 ) ) ;
#27210=VECTOR ( 'NONE', #18827, 1000.000000000000000 ) ;
#27211=CARTESIAN_POINT ( 'NONE',  ( -172.9089226952081617, -189.7472609257535510, 11.92584929509620117 ) ) ;
#27213=VERTEX_POINT ( 'NONE', #37357 ) ;
#27214=ORIENTED_EDGE ( 'NONE', *, *, #25097, .T. ) ;
#27215=DIRECTION ( 'NONE',  ( -0.000000000000000000, 1.000000000000000000, -0.000000000000000000 ) ) ;
#27216=ADVANCED_FACE ( 'NONE', ( #12919 ), #45004, .F. ) ;
#27218=DIRECTION ( 'NONE',  ( -0.000000000000000000, 1.000000000000000000, -0.000000000000000000 ) ) ;
#27219=PLANE ( 'NONE',  #48899 ) ;
#27222=LINE ( 'NONE', #43534, #31629 ) ;
#27223=EDGE_CURVE ( 'NONE', #32514, #51763, #27845, .T. ) ;
#27224=VERTEX_POINT ( 'NONE', #41040 ) ;
#27225=DIRECTION ( 'NONE',  ( -0.000000000000000000, 1.000000000000000000, -0.000000000000000000 ) ) ;
#27226=ORIENTED_EDGE ( 'NONE', *, *, #27553, .T. ) ;
#27228=VERTEX_POINT ( 'NONE', #33680 ) ;
#27229=DIRECTION ( 'NONE',  ( 0.000000000000000000, 0.000000000000000000, -1.000000000000000000 ) ) ;
#27231=VECTOR ( 'NONE', #23113, 1000.000000000000000 ) ;
#27233=EDGE_CURVE ( 'NONE', #3300, #8154, #30363, .T. ) ;
#27236=EDGE_CURVE ( 'NONE', #26646, #23894, #8459, .T. ) ;
#27238=DIRECTION ( 'NONE',  ( 0.9785564922995032555, 0.000000000000000000, 0.2059786187411021818 ) ) ;
#27242=AXIS2_PLACEMENT_3D ( 'NONE', #42004, #25025, #10208 ) ;
#27243=EDGE_CURVE ( 'NONE', #14667, #11081, #42933, .T. ) ;
#27244=ORIENTED_EDGE ( 'NONE', *, *, #45720, .F. ) ;
#27245=FACE_OUTER_BOUND ( 'NONE', #42101, .T. ) ;
#27248=CIRCLE ( 'NONE', #40665, 125.0000000000000000 ) ;
#27249=LINE ( 'NONE', #27762, #50889 ) ;
#27251=PLANE ( 'NONE',  #8718 ) ;
#27253=EDGE_CURVE ( 'NONE', #20455, #9382, #49478, .T. ) ;
#27254=ORIENTED_EDGE ( 'NONE', *, *, #11751, .F. ) ;
#27255=AXIS2_PLACEMENT_3D ( 'NONE', #42877, #15042, #27868 ) ;
#27256=CARTESIAN_POINT ( 'NONE',  ( -9.070200226166589275, -177.1207230881787780, -117.5715283571803980 ) ) ;
#27257=LINE ( 'NONE', #31205, #46679 ) ;
#27259=DIRECTION ( 'NONE',  ( 0.9995608365087944591, 0.000000000000000000, -0.02963332782255633305 ) ) ;
#27261=ADVANCED_FACE ( 'NONE', ( #17670 ), #18174, .T. ) ;
#27263=DIRECTION ( 'NONE',  ( 0.000000000000000000, 0.000000000000000000, 1.000000000000000000 ) ) ;
#27264=ADVANCED_FACE ( 'NONE', ( #34201 ), #26305, .T. ) ;
#27265=ORIENTED_EDGE ( 'NONE', *, *, #28367, .F. ) ;
#27267=VERTEX_POINT ( 'NONE', #21862 ) ;
#27268=ADVANCED_FACE ( 'NONE', ( #18944 ), #38647, .T. ) ;
#27270=VECTOR ( 'NONE', #43551, 1000.000000000000000 ) ;
#27271=FACE_BOUND ( 'NONE', #51084, .T. ) ;
#27274=VECTOR ( 'NONE', #42246, 999.9999999999998863 ) ;
#27275=DIRECTION ( 'NONE',  ( 0.000000000000000000, 0.000000000000000000, -1.000000000000000000 ) ) ;
#27276=EDGE_CURVE ( 'NONE', #9666, #31844, #10538, .T. ) ;
#27278=AXIS2_PLACEMENT_3D ( 'NONE', #1490, #29854, #45647 ) ;
#27279=EDGE_CURVE ( 'NONE', #50350, #22576, #14498, .T. ) ;
#27281=DIRECTION ( 'NONE',  ( -0.000000000000000000, 1.000000000000000000, -0.000000000000000000 ) ) ;
#27282=ORIENTED_EDGE ( 'NONE', *, *, #3815, .T. ) ;
#27283=AXIS2_PLACEMENT_3D ( 'NONE', #46709, #31179, #42761 ) ;
#27284=CARTESIAN_POINT ( 'NONE',  ( -48.47912675150885065, -177.1207230881787780, 6.938893903907228378E-15 ) ) ;
#27285=VECTOR ( 'NONE', #19343, 1000.000000000000000 ) ;
#27286=CIRCLE ( 'NONE', #35691, 125.0000000000000000 ) ;
#27290=ORIENTED_EDGE ( 'NONE', *, *, #24409, .T. ) ;
#27292=CARTESIAN_POINT ( 'NONE',  ( 41.41233698655024398, -183.6283474603465606, 86.85922373029363541 ) ) ;
#27293=VERTEX_POINT ( 'NONE', #9770 ) ;
#27294=FACE_OUTER_BOUND ( 'NONE', #12172, .T. ) ;
#27295=EDGE_LOOP ( 'NONE', ( #32269, #36131, #42360, #15471 ) ) ;
#27296=DIRECTION ( 'NONE',  ( -0.9890401873221623674, 0.000000000000000000, -0.1476465640024917925 ) ) ;
#27297=VERTEX_POINT ( 'NONE', #6612 ) ;
#27298=EDGE_CURVE ( 'NONE', #34044, #31341, #10038, .T. ) ;
#27299=EDGE_CURVE ( 'NONE', #26956, #2085, #34704, .T. ) ;
#27301=ORIENTED_EDGE ( 'NONE', *, *, #27192, .F. ) ;
#27302=CARTESIAN_POINT ( 'NONE',  ( 76.31829002442924548, -193.5000000000000000, 7.113702696402420145 ) ) ;
#27304=VERTEX_POINT ( 'NONE', #6096 ) ;
#27305=EDGE_CURVE ( 'NONE', #8359, #8140, #26988, .T. ) ;
#27308=ORIENTED_EDGE ( 'NONE', *, *, #42716, .F. ) ;
#27312=ORIENTED_EDGE ( 'NONE', *, *, #4125, .T. ) ;
#27314=CARTESIAN_POINT ( 'NONE',  ( -26.20043062753592977, -193.5000000000000000, -122.9986166548863196 ) ) ;
#27316=AXIS2_PLACEMENT_3D ( 'NONE', #21369, #9545, #33193 ) ;
#27318=VECTOR ( 'NONE', #17409, 1000.000000000000000 ) ;
#27319=ORIENTED_EDGE ( 'NONE', *, *, #37247, .F. ) ;
#27320=FACE_OUTER_BOUND ( 'NONE', #45492, .T. ) ;
#27322=DIRECTION ( 'NONE',  ( 0.000000000000000000, -1.000000000000000000, 0.000000000000000000 ) ) ;
#27323=ORIENTED_EDGE ( 'NONE', *, *, #48895, .F. ) ;
#27324=CARTESIAN_POINT ( 'NONE',  ( -173.4291566779743050, -175.3837268820161057, 3.534122433558352760 ) ) ;
#27325=DIRECTION ( 'NONE',  ( 0.000000000000000000, 1.000000000000000000, 0.000000000000000000 ) ) ;
#27327=CIRCLE ( 'NONE', #4677, 125.0000000000000000 ) ;
#27328=CARTESIAN_POINT ( 'NONE',  ( -45.06671089634843952, -177.1207230881787780, -124.9534129907280402 ) ) ;
#27330=ORIENTED_EDGE ( 'NONE', *, *, #19922, .F. ) ;
#27331=EDGE_LOOP ( 'NONE', ( #46838, #11003, #11811, #34046 ) ) ;
#27334=EDGE_CURVE ( 'NONE', #32642, #28039, #25798, .T. ) ;
#27335=VECTOR ( 'NONE', #27945, 1000.000000000000000 ) ;
#27339=PLANE ( 'NONE',  #49737 ) ;
#27340=CARTESIAN_POINT ( 'NONE',  ( 55.03325008324586065, -177.1207230881787780, -70.07273251429356264 ) ) ;
#27341=VERTEX_POINT ( 'NONE', #38126 ) ;
#27346=EDGE_LOOP ( 'NONE', ( #22719, #16635, #6352, #34003 ) ) ;
#27349=AXIS2_PLACEMENT_3D ( 'NONE', #20526, #36296, #27885 ) ;
#27352=DIRECTION ( 'NONE',  ( 0.000000000000000000, 0.000000000000000000, -1.000000000000000000 ) ) ;
#27357=VECTOR ( 'NONE', #48390, 1000.000000000000000 ) ;
#27358=AXIS2_PLACEMENT_3D ( 'NONE', #10915, #42963, #6972 ) ;
#27362=ORIENTED_EDGE ( 'NONE', *, *, #28843, .T. ) ;
#27366=DIRECTION ( 'NONE',  ( -0.000000000000000000, -1.000000000000000000, 0.000000000000000000 ) ) ;
#27367=CARTESIAN_POINT ( 'NONE',  ( -169.0136227435421006, -193.5000000000000000, -33.11246405730811659 ) ) ;
#27369=AXIS2_PLACEMENT_3D ( 'NONE', #30869, #27164, #34790 ) ;
#27370=DIRECTION ( 'NONE',  ( 0.000000000000000000, 0.000000000000000000, -1.000000000000000000 ) ) ;
#27372=DIRECTION ( 'NONE',  ( 0.000000000000000000, 0.000000000000000000, 1.000000000000000000 ) ) ;
#27376=ORIENTED_EDGE ( 'NONE', *, *, #33318, .F. ) ;
#27377=CARTESIAN_POINT ( 'NONE',  ( 75.02564229359539638, -193.5000000000000000, -19.27620354518634826 ) ) ;
#27383=VECTOR ( 'NONE', #35223, 999.9999999999998863 ) ;
#27384=CARTESIAN_POINT ( 'NONE',  ( -114.1105527140175440, -177.1207230881787780, 106.3838142112217326 ) ) ;
#27385=CARTESIAN_POINT ( 'NONE',  ( -173.3294908491238004, -183.6283474603465606, -6.114457023560960991 ) ) ;
#27387=VECTOR ( 'NONE', #44715, 1000.000000000000227 ) ;
#27389=CARTESIAN_POINT ( 'NONE',  ( 7.859956736328458149, -189.7472609257535510, -111.5836353223468649 ) ) ;
#27390=DIRECTION ( 'NONE',  ( 0.000000000000000000, 1.000000000000000000, 0.000000000000000000 ) ) ;
#27391=DIRECTION ( 'NONE',  ( 0.000000000000000000, -0.000000000000000000, -1.000000000000000000 ) ) ;
#27392=AXIS2_PLACEMENT_3D ( 'NONE', #16402, #40287, #352 ) ;
#27396=ORIENTED_EDGE ( 'NONE', *, *, #9893, .T. ) ;
#27397=CIRCLE ( 'NONE', #42525, 125.0000000000000000 ) ;
#27398=CIRCLE ( 'NONE', #13161, 125.0000000000000000 ) ;
#27399=ORIENTED_EDGE ( 'NONE', *, *, #25248, .T. ) ;
#27400=LINE ( 'NONE', #39995, #50972 ) ;
#27401=EDGE_CURVE ( 'NONE', #28959, #3470, #1880, .T. ) ;
#27403=AXIS2_PLACEMENT_3D ( 'NONE', #12947, #89, #40279 ) ;
#27404=PLANE ( 'NONE',  #4455 ) ;
#27405=EDGE_LOOP ( 'NONE', ( #42302, #28182, #43920, #12285 ) ) ;
#27406=ORIENTED_EDGE ( 'NONE', *, *, #19844, .T. ) ;
#27408=CARTESIAN_POINT ( 'NONE',  ( -165.2002711502080672, -193.5000000000000000, 44.73448837594998651 ) ) ;
#27409=VERTEX_POINT ( 'NONE', #50501 ) ;
#27410=LINE ( 'NONE', #37048, #40981 ) ;
#27411=DIRECTION ( 'NONE',  ( 0.000000000000000000, 0.000000000000000000, 1.000000000000000000 ) ) ;
#27413=CARTESIAN_POINT ( 'NONE',  ( 141.7825277784304205, -213.5000000000000000, 10.00000000000000178 ) ) ;
#27414=ORIENTED_EDGE ( 'NONE', *, *, #17541, .F. ) ;
#27417=EDGE_CURVE ( 'NONE', #49057, #4116, #10226, .T. ) ;
#27418=CARTESIAN_POINT ( 'NONE',  ( -49.21696003055057389, -193.5000000000000000, -0.6749830015182127774 ) ) ;
#27419=DIRECTION ( 'NONE',  ( 0.000000000000000000, 0.000000000000000000, -1.000000000000000000 ) ) ;
#27420=AXIS2_PLACEMENT_3D ( 'NONE', #4323, #48740, #24549 ) ;
#27421=FACE_OUTER_BOUND ( 'NONE', #11843, .T. ) ;
#27422=VECTOR ( 'NONE', #43686, 1000.000000000000000 ) ;
#27424=CARTESIAN_POINT ( 'NONE',  ( -21.46839590530488096, -177.1207230881787780, 122.0467960216650880 ) ) ;
#27426=AXIS2_PLACEMENT_3D ( 'NONE', #7535, #3580, #35635 ) ;
#27428=EDGE_CURVE ( 'NONE', #37383, #6661, #32006, .T. ) ;
#27429=DIRECTION ( 'NONE',  ( 0.000000000000000000, 0.000000000000000000, 1.000000000000000000 ) ) ;
#27430=DIRECTION ( 'NONE',  ( 0.000000000000000000, -0.000000000000000000, 1.000000000000000000 ) ) ;
#27432=ORIENTED_EDGE ( 'NONE', *, *, #50685, .T. ) ;
#27435=EDGE_CURVE ( 'NONE', #16290, #6723, #8151, .T. ) ;
#27437=CARTESIAN_POINT ( 'NONE',  ( 75.21854001195777073, -193.5000000000000000, -8.665274887905434653 ) ) ;
#27438=LINE ( 'NONE', #50856, #46835 ) ;
#27440=DIRECTION ( 'NONE',  ( 0.000000000000000000, -1.000000000000000000, 0.000000000000000000 ) ) ;
#27442=AXIS2_PLACEMENT_3D ( 'NONE', #28932, #44720, #564 ) ;
#27443=CARTESIAN_POINT ( 'NONE',  ( 37.77106160267054236, -175.3837268820161057, 89.08931047202636933 ) ) ;
#27446=CARTESIAN_POINT ( 'NONE',  ( 29.90148147319962391, -177.1207230881787780, 96.08646119224012239 ) ) ;
#27448=VECTOR ( 'NONE', #4502, 1000.000000000000114 ) ;
#27450=CARTESIAN_POINT ( 'NONE',  ( -33.98218805075477178, -193.5000000000000000, 123.1496609813405314 ) ) ;
#27451=CARTESIAN_POINT ( 'NONE',  ( -48.47912675150885065, -183.6283474603465606, 6.938893903907228378E-15 ) ) ;
#27452=EDGE_CURVE ( 'NONE', #26525, #47039, #38725, .T. ) ;
#27455=CARTESIAN_POINT ( 'NONE',  ( -48.59739992243022755, -189.7472609257535510, 0.9929810960135230236 ) ) ;
#27456=CARTESIAN_POINT ( 'NONE',  ( 57.12946453413545100, -175.3837268820161057, 66.87170886602000053 ) ) ;
#27459=CARTESIAN_POINT ( 'NONE',  ( -48.47912675150885065, -177.1207230881787780, 6.938893903907228378E-15 ) ) ;
#27460=ORIENTED_EDGE ( 'NONE', *, *, #50424, .T. ) ;
#27462=VECTOR ( 'NONE', #6243, 1000.000000000000000 ) ;
#27464=FACE_OUTER_BOUND ( 'NONE', #26742, .T. ) ;
#27466=ORIENTED_EDGE ( 'NONE', *, *, #9296, .F. ) ;
#27468=ORIENTED_EDGE ( 'NONE', *, *, #40386, .F. ) ;
#27469=DIRECTION ( 'NONE',  ( -0.7575112421616284619, 0.000000000000000000, 0.6528221181905119463 ) ) ;
#27471=AXIS2_PLACEMENT_3D ( 'NONE', #43191, #34022, #332 ) ;
#27472=ORIENTED_EDGE ( 'NONE', *, *, #50183, .T. ) ;
#27473=CARTESIAN_POINT ( 'NONE',  ( -49.47868758801764955, -193.5000000000000000, 0.02963332782255607284 ) ) ;
#27474=CIRCLE ( 'NONE', #4838, 125.0000000000000000 ) ;
#27476=VERTEX_POINT ( 'NONE', #47328 ) ;
#27477=DIRECTION ( 'NONE',  ( 0.000000000000000000, 0.000000000000000000, 1.000000000000000000 ) ) ;
#27478=VECTOR ( 'NONE', #409, 1000.000000000000000 ) ;
#27480=EDGE_CURVE ( 'NONE', #21906, #5412, #31536, .T. ) ;
#27483=LINE ( 'NONE', #48243, #50956 ) ;
#27484=ORIENTED_EDGE ( 'NONE', *, *, #21809, .F. ) ;
#27485=ORIENTED_EDGE ( 'NONE', *, *, #41022, .T. ) ;
#27487=AXIS2_PLACEMENT_3D ( 'NONE', #7407, #31555, #44167 ) ;
#27488=CARTESIAN_POINT ( 'NONE',  ( -107.6930423737362190, -177.1207230881787780, 110.0850225811110761 ) ) ;
#27492=DIRECTION ( 'NONE',  ( 0.000000000000000000, 0.000000000000000000, -1.000000000000000000 ) ) ;
#27493=ORIENTED_EDGE ( 'NONE', *, *, #49783, .F. ) ;
#27495=ADVANCED_FACE ( 'NONE', ( #16042 ), #3179, .F. ) ;
#27496=CARTESIAN_POINT ( 'NONE',  ( -8.169009709621407822, -177.1207230881787780, 118.3219948448695504 ) ) ;
#27499=ORIENTED_EDGE ( 'NONE', *, *, #2462, .T. ) ;
#27500=VECTOR ( 'NONE', #33474, 1000.000000000000000 ) ;
#27501=VERTEX_POINT ( 'NONE', #11577 ) ;
#27502=VECTOR ( 'NONE', #16264, 1000.000000000000000 ) ;
#27503=EDGE_CURVE ( 'NONE', #4690, #19065, #47593, .T. ) ;
#27504=LINE ( 'NONE', #30932, #50147 ) ;
#27506=AXIS2_PLACEMENT_3D ( 'NONE', #8731, #20836, #29234 ) ;
#27507=EDGE_CURVE ( 'NONE', #19466, #19179, #51274, .T. ) ;
#27508=CARTESIAN_POINT ( 'NONE',  ( -154.2693405752510500, -193.5000000000000000, 66.58401203837830451 ) ) ;
#27509=CARTESIAN_POINT ( 'NONE',  ( -91.22542124915045747, -189.7472609257535510, 117.4638425504669783 ) ) ;
#27511=CARTESIAN_POINT ( 'NONE',  ( 75.52097166332625022, -193.5000000000000000, -0.3215015308241103709 ) ) ;
#27512=VERTEX_POINT ( 'NONE', #4214 ) ;
#27514=PLANE ( 'NONE',  #37147 ) ;
#27516=CARTESIAN_POINT ( 'NONE',  ( 25.43954814678887644, -177.1207230881787780, 100.8019320314832754 ) ) ;
#27517=CARTESIAN_POINT ( 'NONE',  ( -48.41988612361515010, -177.1207230881787780, 0.9982437317643287900 ) ) ;
#27518=CARTESIAN_POINT ( 'NONE',  ( 72.95485052494852596, -183.6283474603465606, -29.64437826672758192 ) ) ;
#27519=DIRECTION ( 'NONE',  ( -0.9151456172430237901, 0.000000000000000000, 0.4031234292879600778 ) ) ;
#27520=DIRECTION ( 'NONE',  ( -0.3482016354343866471, 0.000000000000000000, -0.9374196611341253371 ) ) ;
#27521=ORIENTED_EDGE ( 'NONE', *, *, #16992, .F. ) ;
#27524=AXIS2_PLACEMENT_3D ( 'NONE', #33124, #25502, #28913 ) ;
#27526=VERTEX_POINT ( 'NONE', #23155 ) ;
#27527=LINE ( 'NONE', #40130, #16378 ) ;
#27528=CARTESIAN_POINT ( 'NONE',  ( -49.44376233341721161, -193.5000000000000000, 0.2635871660690650709 ) ) ;
#27529=EDGE_LOOP ( 'NONE', ( #49631, #7240, #3510, #19353 ) ) ;
#27532=VECTOR ( 'NONE', #21370, 1000.000000000000000 ) ;
#27533=DIRECTION ( 'NONE',  ( 0.000000000000000000, 0.000000000000000000, 1.000000000000000000 ) ) ;
#27535=AXIS2_PLACEMENT_3D ( 'NONE', #23431, #39436, #18198 ) ;
#27536=FACE_BOUND ( 'NONE', #2886, .T. ) ;
#27537=ADVANCED_FACE ( 'NONE', ( #43110 ), #19452, .T. ) ;
#27538=LINE ( 'NONE', #7822, #28750 ) ;
#27540=VECTOR ( 'NONE', #29170, 1000.000000000000000 ) ;
#27541=EDGE_CURVE ( 'NONE', #31431, #40613, #12069, .T. ) ;
#27543=EDGE_CURVE ( 'NONE', #2344, #28891, #32306, .T. ) ;
#27544=DIRECTION ( 'NONE',  ( 0.000000000000000000, 0.000000000000000000, 1.000000000000000000 ) ) ;
#27547=VERTEX_POINT ( 'NONE', #40983 ) ;
#27548=PLANE ( 'NONE',  #38471 ) ;
#27549=VECTOR ( 'NONE', #7330, 1000.000000000000114 ) ;
#27550=ORIENTED_EDGE ( 'NONE', *, *, #28475, .F. ) ;
#27552=CARTESIAN_POINT ( 'NONE',  ( -48.53836737940257251, -183.6283474603465606, 0.9982437317643279018 ) ) ;
#27553=EDGE_CURVE ( 'NONE', #12201, #6494, #29408, .T. ) ;
#27554=EDGE_CURVE ( 'NONE', #14631, #18737, #1032, .T. ) ;
#27555=VECTOR ( 'NONE', #27810, 1000.000000000000114 ) ;
#27557=DIRECTION ( 'NONE',  ( 0.000000000000000000, 1.000000000000000000, -0.000000000000000000 ) ) ;
#27558=ORIENTED_EDGE ( 'NONE', *, *, #22709, .T. ) ;
#27562=CARTESIAN_POINT ( 'NONE',  ( -48.47912675150885065, -183.6283474603465606, 6.938893903907228378E-15 ) ) ;
#27563=EDGE_LOOP ( 'NONE', ( #12214, #17796, #37464, #5957 ) ) ;
#27566=EDGE_CURVE ( 'NONE', #653, #16210, #11079, .T. ) ;
#27567=FACE_OUTER_BOUND ( 'NONE', #1409, .T. ) ;
#27568=ORIENTED_EDGE ( 'NONE', *, *, #13135, .F. ) ;
#27570=DIRECTION ( 'NONE',  ( 0.2920567706369764371, 0.000000000000000000, -0.9564009842765223146 ) ) ;
#27571=EDGE_LOOP ( 'NONE', ( #13430, #51841, #46472, #48025 ) ) ;
#27572=EDGE_CURVE ( 'NONE', #2420, #37889, #32089, .T. ) ;
#27573=LINE ( 'NONE', #35709, #12282 ) ;
#27574=ORIENTED_EDGE ( 'NONE', *, *, #28184, .T. ) ;
#27575=CARTESIAN_POINT ( 'NONE',  ( -173.2419626162308646, -193.5000000000000000, 7.696413904698416353 ) ) ;
#27576=AXIS2_PLACEMENT_3D ( 'NONE', #18536, #11151, #42441 ) ;
#27577=CARTESIAN_POINT ( 'NONE',  ( -49.38192458147459973, -183.6283474603465606, 0.4300652022765185656 ) ) ;
#27578=AXIS2_PLACEMENT_3D ( 'NONE', #35176, #50973, #27027 ) ;
#27581=CARTESIAN_POINT ( 'NONE',  ( -172.4295958414655274, -189.7472609257535510, 3.504489105735757892 ) ) ;
#27582=VECTOR ( 'NONE', #42545, 1000.000000000000000 ) ;
#27583=LINE ( 'NONE', #43362, #29755 ) ;
#27584=ORIENTED_EDGE ( 'NONE', *, *, #14614, .T. ) ;
#27586=DIRECTION ( 'NONE',  ( -0.000000000000000000, 1.000000000000000000, -0.000000000000000000 ) ) ;
#27587=ADVANCED_FACE ( 'NONE', ( #45215 ), #49413, .T. ) ;
#27589=DIRECTION ( 'NONE',  ( -0.000000000000000000, -1.000000000000000000, 0.000000000000000000 ) ) ;
#27590=ORIENTED_EDGE ( 'NONE', *, *, #1500, .T. ) ;
#27593=LINE ( 'NONE', #18682, #40360 ) ;
#27594=CARTESIAN_POINT ( 'NONE',  ( 32.49319223169170812, -193.5000000000000000, -95.22858582633060109 ) ) ;
#27598=ORIENTED_EDGE ( 'NONE', *, *, #37635, .F. ) ;
#27599=AXIS2_PLACEMENT_3D ( 'NONE', #16468, #24861, #24098 ) ;
#27600=EDGE_CURVE ( 'NONE', #13819, #3616, #9450, .T. ) ;
#27602=DIRECTION ( 'NONE',  ( 0.000000000000000000, -1.000000000000000000, -0.000000000000000000 ) ) ;
#27603=DIRECTION ( 'NONE',  ( -0.000000000000000000, 1.000000000000000000, -0.000000000000000000 ) ) ;
#27604=DIRECTION ( 'NONE',  ( 0.000000000000000000, 0.000000000000000000, 1.000000000000000000 ) ) ;
#27605=ORIENTED_EDGE ( 'NONE', *, *, #17231, .F. ) ;
#27606=EDGE_CURVE ( 'NONE', #33402, #3342, #6891, .T. ) ;
#27608=EDGE_CURVE ( 'NONE', #48860, #17312, #40707, .T. ) ;
#27611=ORIENTED_EDGE ( 'NONE', *, *, #42612, .F. ) ;
#27612=EDGE_LOOP ( 'NONE', ( #36399, #45250, #36378, #9647 ) ) ;
#27614=ORIENTED_EDGE ( 'NONE', *, *, #8758, .F. ) ;
#27615=LINE ( 'NONE', #39938, #35952 ) ;
#27616=AXIS2_PLACEMENT_3D ( 'NONE', #10947, #26968, #8807 ) ;
#27618=VERTEX_POINT ( 'NONE', #16831 ) ;
#27625=ADVANCED_FACE ( 'NONE', ( #48886 ), #8930, .T. ) ;
#27627=ORIENTED_EDGE ( 'NONE', *, *, #39058, .F. ) ;
#27629=EDGE_LOOP ( 'NONE', ( #21131, #19681, #31502, #19903 ) ) ;
#27630=ADVANCED_FACE ( 'NONE', ( #21017 ), #37035, .T. ) ;
#27631=CIRCLE ( 'NONE', #4996, 125.0000000000000000 ) ;
#27632=DIRECTION ( 'NONE',  ( -0.4300652022765183435, 0.000000000000000000, -0.9027978299657446470 ) ) ;
#27636=EDGE_LOOP ( 'NONE', ( #13069, #51735, #849, #2818 ) ) ;
#27640=DIRECTION ( 'NONE',  ( -1.000000000000000000, 0.000000000000000000, -0.000000000000000000 ) ) ;
#27642=ORIENTED_EDGE ( 'NONE', *, *, #28276, .T. ) ;
#27643=CARTESIAN_POINT ( 'NONE',  ( -48.47912675150885065, -183.6283474603465606, 6.938893903907228378E-15 ) ) ;
#27646=VERTEX_POINT ( 'NONE', #26237 ) ;
#27647=PLANE ( 'NONE',  #28423 ) ;
#27652=ORIENTED_EDGE ( 'NONE', *, *, #24230, .T. ) ;
#27653=AXIS2_PLACEMENT_3D ( 'NONE', #31930, #12213, #8790 ) ;
#27654=DIRECTION ( 'NONE',  ( 0.2920567706369694982, 0.000000000000000000, 0.9564009842765243130 ) ) ;
#27655=DIRECTION ( 'NONE',  ( 0.8455960035018272869, 0.000000000000000000, -0.5338233779647886257 ) ) ;
#27656=AXIS2_PLACEMENT_3D ( 'NONE', #48372, #32597, #8683 ) ;
#27658=DIRECTION ( 'NONE',  ( 0.1182731709213592358, 0.000000000000000000, 0.9929810960135178055 ) ) ;
#27659=CARTESIAN_POINT ( 'NONE',  ( 75.78974234412359579, -177.1207230881787780, 13.49993235881449394 ) ) ;
#27662=CARTESIAN_POINT ( 'NONE',  ( -48.18706998087187543, -193.5000000000000000, -0.9564009842765152092 ) ) ;
#27663=CARTESIAN_POINT ( 'NONE',  ( 42.45000882818163035, -189.7472609257535510, -84.30834960112932208 ) ) ;
#27664=ORIENTED_EDGE ( 'NONE', *, *, #15996, .T. ) ;
#27665=ORIENTED_EDGE ( 'NONE', *, *, #21925, .F. ) ;
#27666=EDGE_CURVE ( 'NONE', #45739, #45186, #18678, .T. ) ;
#27667=ADVANCED_FACE ( 'NONE', ( #42269 ), #50190, .T. ) ;
#27669=AXIS2_PLACEMENT_3D ( 'NONE', #11197, #18056, #34084 ) ;
#27670=PLANE ( 'NONE',  #26273 ) ;
#27672=ORIENTED_EDGE ( 'NONE', *, *, #51153, .T. ) ;
#27673=PLANE ( 'NONE',  #13073 ) ;
#27675=DIRECTION ( 'NONE',  ( 0.000000000000000000, 0.000000000000000000, -1.000000000000000000 ) ) ;
#27677=DIRECTION ( 'NONE',  ( 0.000000000000000000, 1.000000000000000000, -0.000000000000000000 ) ) ;
#27680=ORIENTED_EDGE ( 'NONE', *, *, #202, .F. ) ;
#27682=CARTESIAN_POINT ( 'NONE',  ( -161.2555905272864436, -193.5000000000000000, -53.91167979418489864 ) ) ;
#27683=CARTESIAN_POINT ( 'NONE',  ( -172.0042974347349229, -175.3837268820161057, 10.84123789944660388 ) ) ;
#27686=CARTESIAN_POINT ( 'NONE',  ( -170.8336150310145172, -189.7472609257535510, 25.58083653558488280 ) ) ;
#27687=VERTEX_POINT ( 'NONE', #1566 ) ;
#27688=CARTESIAN_POINT ( 'NONE',  ( 72.35619569422321717, -183.6283474603465606, 27.83926365844748574 ) ) ;
#27692=EDGE_LOOP ( 'NONE', ( #35304, #33655, #13001, #27499 ) ) ;
#27693=ORIENTED_EDGE ( 'NONE', *, *, #49509, .F. ) ;
#27694=VERTEX_POINT ( 'NONE', #14185 ) ;
#27695=DIRECTION ( 'NONE',  ( 0.000000000000000000, 0.000000000000000000, -1.000000000000000000 ) ) ;
#27696=CARTESIAN_POINT ( 'NONE',  ( -78.64590280292340196, -175.3837268820161057, -121.3052580173827266 ) ) ;
#27697=VERTEX_POINT ( 'NONE', #2066 ) ;
#27698=DIRECTION ( 'NONE',  ( -0.000000000000000000, 1.000000000000000000, -0.000000000000000000 ) ) ;
#27699=LINE ( 'NONE', #3012, #22019 ) ;
#27700=DIRECTION ( 'NONE',  ( 0.000000000000000000, -1.000000000000000000, 0.000000000000000000 ) ) ;
#27701=EDGE_LOOP ( 'NONE', ( #22057, #48875, #5253, #31182 ) ) ;
#27703=VECTOR ( 'NONE', #20915, 1000.000000000000114 ) ;
#27704=VECTOR ( 'NONE', #29533, 1000.000000000000000 ) ;
#27706=CARTESIAN_POINT ( 'NONE',  ( -14.28570516517293854, -177.1207230881787780, 120.2323164553486521 ) ) ;
#27707=DIRECTION ( 'NONE',  ( -0.3482016354343866471, 0.000000000000000000, -0.9374196611341253371 ) ) ;
#27708=VERTEX_POINT ( 'NONE', #18111 ) ;
#27710=PLANE ( 'NONE',  #26389 ) ;
#27711=FACE_OUTER_BOUND ( 'NONE', #25225, .T. ) ;
#27712=FACE_OUTER_BOUND ( 'NONE', #2541, .T. ) ;
#27714=ORIENTED_EDGE ( 'NONE', *, *, #8646, .T. ) ;
#27717=ORIENTED_EDGE ( 'NONE', *, *, #7024, .F. ) ;
#27719=LINE ( 'NONE', #43750, #15126 ) ;
#27722=ORIENTED_EDGE ( 'NONE', *, *, #30836, .F. ) ;
#27723=CARTESIAN_POINT ( 'NONE',  ( -147.2362428880188077, -183.6283474603465606, -74.98773087994455011 ) ) ;
#27728=CARTESIAN_POINT ( 'NONE',  ( -16.77927958806651887, -177.1207230881787780, -120.9136869416130082 ) ) ;
#27729=PLANE ( 'NONE',  #17904 ) ;
#27730=EDGE_LOOP ( 'NONE', ( #14107, #26562, #45691, #43809 ) ) ;
#27731=CARTESIAN_POINT ( 'NONE',  ( -104.9497554727472703, -193.5000000000000000, -110.3950557015148632 ) ) ;
#27732=LINE ( 'NONE', #4603, #48456 ) ;
#27733=CARTESIAN_POINT ( 'NONE',  ( 116.9235303384055840, -193.5000000000000000, 10.00000000000000000 ) ) ;
#27734=FACE_OUTER_BOUND ( 'NONE', #47690, .T. ) ;
#27737=CIRCLE ( 'NONE', #48726, 125.0000000000000000 ) ;
#27740=CYLINDRICAL_SURFACE ( 'NONE', #50119, 125.0000000000000000 ) ;
#27745=LINE ( 'NONE', #19609, #19678 ) ;
#27747=CARTESIAN_POINT ( 'NONE',  ( 65.12862465015751923, -177.1207230881787780, 49.69312418816387833 ) ) ;
#27748=EDGE_LOOP ( 'NONE', ( #3593, #31604, #3978, #4973 ) ) ;
#27749=LINE ( 'NONE', #43782, #4635 ) ;
#27750=VERTEX_POINT ( 'NONE', #34642 ) ;
#27753=DIRECTION ( 'NONE',  ( -0.000000000000000000, 1.000000000000000000, -0.000000000000000000 ) ) ;
#27754=CARTESIAN_POINT ( 'NONE',  ( -37.08895481556041318, -177.1207230881787780, 124.4799742258550310 ) ) ;
#27755=DIRECTION ( 'NONE',  ( 0.000000000000000000, 0.000000000000000000, -1.000000000000000000 ) ) ;
#27760=ORIENTED_EDGE ( 'NONE', *, *, #24005, .T. ) ;
#27761=CARTESIAN_POINT ( 'NONE',  ( -84.19171550243319757, -189.7472609257535510, 119.7898618611247628 ) ) ;
#27762=CARTESIAN_POINT ( 'NONE',  ( -55.71438232577009586, -175.3837268820161057, -124.7904286264580804 ) ) ;
#27763=DIRECTION ( 'NONE',  ( 0.000000000000000000, 0.000000000000000000, -1.000000000000000000 ) ) ;
#27764=VECTOR ( 'NONE', #18739, 1000.000000000000000 ) ;
#27765=EDGE_CURVE ( 'NONE', #17878, #21936, #10215, .T. ) ;
#27766=CARTESIAN_POINT ( 'NONE',  ( -48.47912675150885065, -183.6283474603465606, 6.938893903907228378E-15 ) ) ;
#27771=VECTOR ( 'NONE', #4206, 1000.000000000000114 ) ;
#27772=ADVANCED_FACE ( 'NONE', ( #29934 ), #25993, .F. ) ;
#27773=FACE_BOUND ( 'NONE', #14538, .T. ) ;
#27775=PLANE ( 'NONE',  #34851 ) ;
#27777=ORIENTED_EDGE ( 'NONE', *, *, #51576, .T. ) ;
#27780=VERTEX_POINT ( 'NONE', #14432 ) ;
#27781=EDGE_CURVE ( 'NONE', #28621, #2310, #10740, .T. ) ;
#27782=EDGE_CURVE ( 'NONE', #35294, #23517, #38069, .T. ) ;
#27783=FACE_OUTER_BOUND ( 'NONE', #23446, .T. ) ;
#27785=AXIS2_PLACEMENT_3D ( 'NONE', #22388, #38411, #34218 ) ;
#27786=FACE_BOUND ( 'NONE', #48224, .T. ) ;
#27787=ADVANCED_FACE ( 'NONE', ( #22827 ), #29726, .T. ) ;
#27789=DIRECTION ( 'NONE',  ( 0.8124868780056863082, 0.000000000000000000, -0.5829794791144649047 ) ) ;
#27790=ORIENTED_EDGE ( 'NONE', *, *, #38650, .F. ) ;
#27795=DIRECTION ( 'NONE',  ( 0.000000000000000000, -1.000000000000000000, 0.000000000000000000 ) ) ;
#27797=AXIS2_PLACEMENT_3D ( 'NONE', #25141, #24869, #49578 ) ;
#27800=FACE_OUTER_BOUND ( 'NONE', #1832, .T. ) ;
#27803=PLANE ( 'NONE',  #3767 ) ;
#27804=EDGE_LOOP ( 'NONE', ( #34266, #32829, #45675, #6082 ) ) ;
#27806=CARTESIAN_POINT ( 'NONE',  ( -1.230335819511603423, -183.6283474603465606, 115.7261930397108216 ) ) ;
#27807=ORIENTED_EDGE ( 'NONE', *, *, #37450, .F. ) ;
#27808=DIRECTION ( 'NONE',  ( -0.6965510290629982615, 0.000000000000000000, 0.7175072570443298270 ) ) ;
#27809=ORIENTED_EDGE ( 'NONE', *, *, #37589, .T. ) ;
#27810=DIRECTION ( 'NONE',  ( -0.9027978299657387629, 0.000000000000000000, -0.4300652022765304450 ) ) ;
#27811=ORIENTED_EDGE ( 'NONE', *, *, #4474, .F. ) ;
#27812=CARTESIAN_POINT ( 'NONE',  ( -48.47912675150885065, -175.3837268820161057, 6.938893903907228378E-15 ) ) ;
#27815=AXIS2_PLACEMENT_3D ( 'NONE', #41484, #38765, #5785 ) ;
#27816=DIRECTION ( 'NONE',  ( -0.000000000000000000, 1.000000000000000000, -0.000000000000000000 ) ) ;
#27818=CARTESIAN_POINT ( 'NONE',  ( -82.67254833784559764, -193.5000000000000000, -120.2323164553483963 ) ) ;
#27819=CARTESIAN_POINT ( 'NONE',  ( -145.0195698084541505, -189.7472609257535510, 79.40367028273128369 ) ) ;
#27821=FACE_OUTER_BOUND ( 'NONE', #28275, .T. ) ;
#27822=DIRECTION ( 'NONE',  ( -0.7948544414133608127, 0.000000000000000000, 0.6068001458185834363 ) ) ;
#27823=DIRECTION ( 'NONE',  ( 0.9473263538541899509, 0.000000000000000000, 0.3202698538628415692 ) ) ;
#27824=PLANE ( 'NONE',  #7919 ) ;
#27825=EDGE_CURVE ( 'NONE', #20039, #50250, #20823, .T. ) ;
#27826=ADVANCED_FACE ( 'NONE', ( #4798 ), #41294, .T. ) ;
#27827=ORIENTED_EDGE ( 'NONE', *, *, #41730, .F. ) ;
#27828=EDGE_CURVE ( 'NONE', #39416, #14560, #5849, .T. ) ;
#27831=DIRECTION ( 'NONE',  ( -0.000000000000000000, 1.000000000000000000, -0.000000000000000000 ) ) ;
#27833=ORIENTED_EDGE ( 'NONE', *, *, #10118, .F. ) ;
#27834=CARTESIAN_POINT ( 'NONE',  ( -48.47912675150885065, -175.3837268820161057, 6.938893903907228378E-15 ) ) ;
#27835=EDGE_CURVE ( 'NONE', #18649, #46522, #9771, .T. ) ;
#27836=AXIS2_PLACEMENT_3D ( 'NONE', #45070, #48743, #25093 ) ;
#27839=ORIENTED_EDGE ( 'NONE', *, *, #25662, .T. ) ;
#27840=VERTEX_POINT ( 'NONE', #1632 ) ;
#27841=ADVANCED_FACE ( 'NONE', ( #45775 ), #45005, .T. ) ;
#27842=AXIS2_PLACEMENT_3D ( 'NONE', #3535, #19568, #15637 ) ;
#27845=CIRCLE ( 'NONE', #4335, 10.00000000000000178 ) ;
#27847=ADVANCED_FACE ( 'NONE', ( #21338 ), #16632, .T. ) ;
#27849=CARTESIAN_POINT ( 'NONE',  ( -137.9639882952644712, -183.6283474603465606, 87.27805883780237650 ) ) ;
#27851=EDGE_CURVE ( 'NONE', #10865, #10929, #33156, .T. ) ;
#27852=VERTEX_POINT ( 'NONE', #1093 ) ;
#27858=AXIS2_PLACEMENT_3D ( 'NONE', #30083, #21421, #17505 ) ;
#27859=VERTEX_POINT ( 'NONE', #17418 ) ;
#27860=FACE_OUTER_BOUND ( 'NONE', #46388, .T. ) ;
#27861=ORIENTED_EDGE ( 'NONE', *, *, #3104, .T. ) ;
#27864=CARTESIAN_POINT ( 'NONE',  ( 24.63024857337166296, -193.5000000000000000, 101.3904297239426597 ) ) ;
#27865=PLANE ( 'NONE',  #34210 ) ;
#27866=DIRECTION ( 'NONE',  ( 0.000000000000000000, 0.000000000000000000, -1.000000000000000000 ) ) ;
#27867=ORIENTED_EDGE ( 'NONE', *, *, #21853, .F. ) ;
#27868=DIRECTION ( 'NONE',  ( 0.9473263538541946138, 0.000000000000000000, -0.3202698538628279690 ) ) ;
#27869=ORIENTED_EDGE ( 'NONE', *, *, #34592, .T. ) ;
#27870=CARTESIAN_POINT ( 'NONE',  ( -136.1415351158078693, -193.5000000000000000, -89.10837311819173578 ) ) ;
#27873=LINE ( 'NONE', #9669, #47605 ) ;
#27874=CARTESIAN_POINT ( 'NONE',  ( 17.98688506184921820, -177.1207230881787780, 104.6823626202124444 ) ) ;
#27876=DIRECTION ( 'NONE',  ( 0.2635871660690715101, 0.000000000000000000, -0.9646355819083576311 ) ) ;
#27878=VECTOR ( 'NONE', #13709, 1000.000000000000114 ) ;
#27879=EDGE_CURVE ( 'NONE', #40321, #14309, #13198, .T. ) ;
#27881=LINE ( 'NONE', #31842, #11892 ) ;
#27882=ORIENTED_EDGE ( 'NONE', *, *, #21094, .F. ) ;
#27885=DIRECTION ( 'NONE',  ( 0.000000000000000000, 0.000000000000000000, -1.000000000000000000 ) ) ;
#27890=EDGE_CURVE ( 'NONE', #3230, #45161, #26235, .T. ) ;
#27891=CARTESIAN_POINT ( 'NONE',  ( -127.0132498732366173, -177.1207230881787780, 97.24912084693264092 ) ) ;
#27892=AXIS2_PLACEMENT_3D ( 'NONE', #24692, #16833, #32836 ) ;
#27894=VECTOR ( 'NONE', #46655, 1000.000000000000114 ) ;
#27895=ADVANCED_FACE ( 'NONE', ( #42077 ), #6098, .T. ) ;
#27896=VERTEX_POINT ( 'NONE', #30257 ) ;
#27900=VECTOR ( 'NONE', #17242, 1000.000000000000000 ) ;
#27902=EDGE_CURVE ( 'NONE', #25533, #8754, #50502, .T. ) ;
#27903=DIRECTION ( 'NONE',  ( -0.000000000000000000, 1.000000000000000000, 0.000000000000000000 ) ) ;
#27904=DIRECTION ( 'NONE',  ( 0.000000000000000000, -1.000000000000000000, 0.000000000000000000 ) ) ;
#27905=FACE_OUTER_BOUND ( 'NONE', #18445, .T. ) ;
#27906=CARTESIAN_POINT ( 'NONE',  ( -162.0868781531755758, -193.5000000000000000, -49.69312418816308963 ) ) ;
#27907=EDGE_CURVE ( 'NONE', #40028, #51485, #34705, .T. ) ;
#27908=EDGE_CURVE ( 'NONE', #17428, #1315, #22116, .T. ) ;
#27909=LINE ( 'NONE', #7444, #10353 ) ;
#27910=EDGE_CURVE ( 'NONE', #11425, #11764, #38127, .T. ) ;
#27913=PLANE ( 'NONE',  #39593 ) ;
#27915=VECTOR ( 'NONE', #5945, 1000.000000000000000 ) ;
#27916=ADVANCED_FACE ( 'NONE', ( #10039 ), #34454, .T. ) ;
#27917=ORIENTED_EDGE ( 'NONE', *, *, #27554, .F. ) ;
#27918=CARTESIAN_POINT ( 'NONE',  ( -19.18792875895802652, -175.3837268820161057, -120.4907712303050715 ) ) ;
#27921=CYLINDRICAL_SURFACE ( 'NONE', #45618, 125.0000000000000000 ) ;
#27923=VERTEX_POINT ( 'NONE', #34202 ) ;
#27925=DIRECTION ( 'NONE',  ( 0.000000000000000000, 0.000000000000000000, 1.000000000000000000 ) ) ;
#27926=CARTESIAN_POINT ( 'NONE',  ( 73.32544842769510751, -193.5000000000000000, -23.23456943914041517 ) ) ;
#27927=DIRECTION ( 'NONE',  ( 0.000000000000000000, -1.000000000000000000, 0.000000000000000000 ) ) ;
#27928=DIRECTION ( 'NONE',  ( 0.000000000000000000, 0.000000000000000000, 1.000000000000000000 ) ) ;
#27929=AXIS2_PLACEMENT_3D ( 'NONE', #23637, #43371, #30754 ) ;
#27930=VERTEX_POINT ( 'NONE', #50248 ) ;
#27933=VERTEX_POINT ( 'NONE', #42600 ) ;
#27934=EDGE_CURVE ( 'NONE', #49365, #43643, #27075, .T. ) ;
#27936=FACE_OUTER_BOUND ( 'NONE', #10884, .T. ) ;
#27938=CIRCLE ( 'NONE', #45595, 125.0000000000000000 ) ;
#27941=ORIENTED_EDGE ( 'NONE', *, *, #11193, .T. ) ;
#27942=CARTESIAN_POINT ( 'NONE',  ( 64.72501964220592185, -189.7472609257535510, 53.00774697410174952 ) ) ;
#27943=AXIS2_PLACEMENT_3D ( 'NONE', #4333, #8526, #19585 ) ;
#27945=DIRECTION ( 'NONE',  ( -0.1768902751225592818, 0.000000000000000000, -0.9842305779475992722 ) ) ;
#27946=DIRECTION ( 'NONE',  ( 0.000000000000000000, 0.000000000000000000, 1.000000000000000000 ) ) ;
#27949=EDGE_LOOP ( 'NONE', ( #28730, #44140, #1697, #8297 ) ) ;
#27950=DIRECTION ( 'NONE',  ( -0.000000000000000000, 1.000000000000000000, -0.000000000000000000 ) ) ;
#27951=DIRECTION ( 'NONE',  ( 0.000000000000000000, -1.000000000000000000, 0.000000000000000000 ) ) ;
#27952=EDGE_LOOP ( 'NONE', ( #33472, #1047, #12413, #38679 ) ) ;
#27954=AXIS2_PLACEMENT_3D ( 'NONE', #49962, #13958, #46038 ) ;
#27955=FACE_OUTER_BOUND ( 'NONE', #39455, .T. ) ;
#27956=ADVANCED_FACE ( 'NONE', ( #26306 ), #31024, .T. ) ;
#27957=DIRECTION ( 'NONE',  ( 0.000000000000000000, 0.000000000000000000, 1.000000000000000000 ) ) ;
#27958=EDGE_CURVE ( 'NONE', #30593, #12246, #51431, .T. ) ;
#27959=ORIENTED_EDGE ( 'NONE', *, *, #41242, .F. ) ;
#27960=DIRECTION ( 'NONE',  ( -0.000000000000000000, 1.000000000000000000, 0.000000000000000000 ) ) ;
#27961=AXIS2_PLACEMENT_3D ( 'NONE', #20554, #45525, #25539 ) ;
#27963=ORIENTED_EDGE ( 'NONE', *, *, #16190, .F. ) ;
#27964=CARTESIAN_POINT ( 'NONE',  ( -48.47912675150885065, -189.7472609257535510, 6.938893903907228378E-15 ) ) ;
#27965=EDGE_LOOP ( 'NONE', ( #4687, #3725, #27265, #30856 ) ) ;
#27967=DIRECTION ( 'NONE',  ( -0.000000000000000000, 1.000000000000000000, -0.000000000000000000 ) ) ;
#27968=ORIENTED_EDGE ( 'NONE', *, *, #22106, .F. ) ;
#27969=CARTESIAN_POINT ( 'NONE',  ( -48.18706998087187543, -183.6283474603465606, -0.9564009842765152092 ) ) ;
#27970=CARTESIAN_POINT ( 'NONE',  ( -170.7635349987907603, -175.3837268820161057, -25.91377046305877130 ) ) ;
#27971=DIRECTION ( 'NONE',  ( -0.000000000000000000, 1.000000000000000000, -0.000000000000000000 ) ) ;
#27973=CYLINDRICAL_SURFACE ( 'NONE', #2269, 125.0000000000000000 ) ;
#27974=ORIENTED_EDGE ( 'NONE', *, *, #23977, .F. ) ;
#27975=CARTESIAN_POINT ( 'NONE',  ( -158.1873290247468447, -193.5000000000000000, 57.79541595648305474 ) ) ;
#27976=ORIENTED_EDGE ( 'NONE', *, *, #43523, .T. ) ;
#27978=EDGE_CURVE ( 'NONE', #4174, #33649, #9486, .T. ) ;
#27980=CARTESIAN_POINT ( 'NONE',  ( -48.88225018079680950, -183.6283474603465606, -0.9151456172430169067 ) ) ;
#27981=ORIENTED_EDGE ( 'NONE', *, *, #26318, .F. ) ;
#27983=FACE_OUTER_BOUND ( 'NONE', #4877, .T. ) ;
#27986=VERTEX_POINT ( 'NONE', #26565 ) ;
#27987=DIRECTION ( 'NONE',  ( 0.000000000000000000, -0.000000000000000000, 1.000000000000000000 ) ) ;
#27989=VERTEX_POINT ( 'NONE', #50754 ) ;
#27990=DIRECTION ( 'NONE',  ( -0.000000000000000000, 1.000000000000000000, -0.000000000000000000 ) ) ;
#27991=DIRECTION ( 'NONE',  ( 0.000000000000000000, 0.000000000000000000, -1.000000000000000000 ) ) ;
#27992=AXIS2_PLACEMENT_3D ( 'NONE', #46473, #10456, #34629 ) ;
#27995=ORIENTED_EDGE ( 'NONE', *, *, #46733, .T. ) ;
#27997=VECTOR ( 'NONE', #46470, 1000.000000000000000 ) ;
#27998=EDGE_LOOP ( 'NONE', ( #42676, #34554, #31180, #29553 ) ) ;
#28001=DIRECTION ( 'NONE',  ( 0.000000000000000000, 1.000000000000000000, -0.000000000000000000 ) ) ;
#28007=PLANE ( 'NONE',  #26459 ) ;
#28008=VERTEX_POINT ( 'NONE', #46819 ) ;
#28009=ORIENTED_EDGE ( 'NONE', *, *, #20431, .T. ) ;
#28010=CYLINDRICAL_SURFACE ( 'NONE', #12337, 125.0000000000000000 ) ;
#28011=DIRECTION ( 'NONE',  ( 0.000000000000000000, 1.000000000000000000, 0.000000000000000000 ) ) ;
#28012=CARTESIAN_POINT ( 'NONE',  ( 73.32544842769512172, -183.6283474603465606, -23.23456943914042228 ) ) ;
#28013=ADVANCED_FACE ( 'NONE', ( #10801 ), #26821, .F. ) ;
#28015=ORIENTED_EDGE ( 'NONE', *, *, #45603, .F. ) ;
#28017=EDGE_LOOP ( 'NONE', ( #1680, #29636, #43180, #23993 ) ) ;
#28018=VERTEX_POINT ( 'NONE', #15021 ) ;
#28020=CARTESIAN_POINT ( 'NONE',  ( -137.2261550162227195, -177.1207230881787780, 86.60307583628417660 ) ) ;
#28021=CARTESIAN_POINT ( 'NONE',  ( 21.47984469475713354, -175.3837268820161057, 102.3804074221065292 ) ) ;
#28022=AXIS2_PLACEMENT_3D ( 'NONE', #9373, #32762, #48805 ) ;
#28023=FACE_OUTER_BOUND ( 'NONE', #6937, .T. ) ;
#28024=AXIS2_PLACEMENT_3D ( 'NONE', #19185, #3151, #34935 ) ;
#28031=FACE_BOUND ( 'NONE', #15257, .T. ) ;
#28032=ORIENTED_EDGE ( 'NONE', *, *, #6632, .F. ) ;
#28034=DIRECTION ( 'NONE',  ( 0.000000000000000000, 0.000000000000000000, 1.000000000000000000 ) ) ;
#28036=ORIENTED_EDGE ( 'NONE', *, *, #13136, .F. ) ;
#28038=VECTOR ( 'NONE', #18773, 1000.000000000000227 ) ;
#28039=VERTEX_POINT ( 'NONE', #51795 ) ;
#28040=DIRECTION ( 'NONE',  ( -0.9027978299657387629, 0.000000000000000000, -0.4300652022765304450 ) ) ;
#28041=FACE_BOUND ( 'NONE', #36449, .T. ) ;
#28042=FACE_OUTER_BOUND ( 'NONE', #50221, .T. ) ;
#28044=EDGE_CURVE ( 'NONE', #47044, #19921, #20345, .T. ) ;
#28048=CARTESIAN_POINT ( 'NONE',  ( -152.8713435144644848, -193.5000000000000000, -68.75510947788595217 ) ) ;
#28049=EDGE_LOOP ( 'NONE', ( #6261, #5423, #31085, #37423 ) ) ;
#28050=FACE_OUTER_BOUND ( 'NONE', #37098, .T. ) ;
#28051=VECTOR ( 'NONE', #13417, 999.9999999999998863 ) ;
#28052=CARTESIAN_POINT ( 'NONE',  ( -164.2512865680372727, -189.7472609257535510, -47.13604789772048775 ) ) ;
#28053=AXIS2_PLACEMENT_3D ( 'NONE', #31515, #36485, #8132 ) ;
#28056=DIRECTION ( 'NONE',  ( 0.000000000000000000, 0.000000000000000000, 1.000000000000000000 ) ) ;
#28057=ORIENTED_EDGE ( 'NONE', *, *, #22640, .T. ) ;
#28059=DIRECTION ( 'NONE',  ( -0.8858462335218260097, 0.000000000000000000, -0.4639789333096864810 ) ) ;
#28061=ORIENTED_EDGE ( 'NONE', *, *, #19261, .T. ) ;
#28062=DIRECTION ( 'NONE',  ( 0.1768902751225802927, 0.000000000000000000, -0.9842305779475953864 ) ) ;
#28064=DIRECTION ( 'NONE',  ( -0.9785564922995046988, 0.000000000000000000, 0.2059786187410953262 ) ) ;
#28066=EDGE_CURVE ( 'NONE', #7899, #9774, #23908, .T. ) ;
#28068=ORIENTED_EDGE ( 'NONE', *, *, #30813, .F. ) ;
#28069=DIRECTION ( 'NONE',  ( 0.000000000000000000, -1.000000000000000000, -0.000000000000000000 ) ) ;
#28070=DIRECTION ( 'NONE',  ( 0.000000000000000000, 1.000000000000000000, -0.000000000000000000 ) ) ;
#28074=ORIENTED_EDGE ( 'NONE', *, *, #2756, .F. ) ;
#28075=CARTESIAN_POINT ( 'NONE',  ( -114.9451385648676336, -177.1207230881787780, -104.6823626202119613 ) ) ;
#28076=ADVANCED_FACE ( 'NONE', ( #11302 ), #27339, .F. ) ;
#28084=LINE ( 'NONE', #40187, #8677 ) ;
#28085=CARTESIAN_POINT ( 'NONE',  ( 76.21810084846656252, -177.1207230881787780, -8.694908215727984668 ) ) ;
#28086=CARTESIAN_POINT ( 'NONE',  ( -157.1522883217072604, -189.7472609257535510, 59.71720175837172917 ) ) ;
#28087=ORIENTED_EDGE ( 'NONE', *, *, #9928, .F. ) ;
#28088=VECTOR ( 'NONE', #8764, 1000.000000000000000 ) ;
#28089=CARTESIAN_POINT ( 'NONE',  ( -48.47912675150885065, -177.1207230881787780, 6.938893903907228378E-15 ) ) ;
#28090=EDGE_CURVE ( 'NONE', #31327, #4741, #20234, .T. ) ;
#28092=VECTOR ( 'NONE', #6536, 1000.000000000000000 ) ;
#28093=DIRECTION ( 'NONE',  ( 0.000000000000000000, -0.000000000000000000, -1.000000000000000000 ) ) ;
#28094=LINE ( 'NONE', #20477, #2655 ) ;
#28095=ORIENTED_EDGE ( 'NONE', *, *, #19315, .F. ) ;
#28097=EDGE_LOOP ( 'NONE', ( #12773, #32239, #31547, #9934 ) ) ;
#28098=DIRECTION ( 'NONE',  ( 0.000000000000000000, -1.000000000000000000, 0.000000000000000000 ) ) ;
#28100=CARTESIAN_POINT ( 'NONE',  ( 20.65191334053707095, -175.3837268820161057, 102.9412430821799802 ) ) ;
#28101=CARTESIAN_POINT ( 'NONE',  ( -48.47912675150885065, -177.1207230881787780, 6.938893903907228378E-15 ) ) ;
#28102=AXIS2_PLACEMENT_3D ( 'NONE', #36922, #32458, #24831 ) ;
#28106=ORIENTED_EDGE ( 'NONE', *, *, #25943, .F. ) ;
#28107=VERTEX_POINT ( 'NONE', #255 ) ;
#28108=VECTOR ( 'NONE', #38349, 1000.000000000000000 ) ;
#28109=ORIENTED_EDGE ( 'NONE', *, *, #28713, .F. ) ;
#28110=ORIENTED_EDGE ( 'NONE', *, *, #46492, .T. ) ;
#28111=DIRECTION ( 'NONE',  ( -0.7378332790417189146, 0.000000000000000000, -0.6749830015182196608 ) ) ;
#28113=EDGE_CURVE ( 'NONE', #41296, #35254, #31813, .T. ) ;
#28114=VERTEX_POINT ( 'NONE', #27849 ) ;
#28115=DIRECTION ( 'NONE',  ( -0.3202698538628487301, 0.000000000000000000, 0.9473263538541877304 ) ) ;
#28119=VERTEX_POINT ( 'NONE', #7880 ) ;
#28120=VECTOR ( 'NONE', #31010, 1000.000000000000114 ) ;
#28121=CARTESIAN_POINT ( 'NONE',  ( -49.25565061422688728, -177.1207230881787780, -0.6300878435817132139 ) ) ;
#28125=ORIENTED_EDGE ( 'NONE', *, *, #27299, .T. ) ;
#28126=VECTOR ( 'NONE', #39469, 1000.000000000000000 ) ;
#28127=CARTESIAN_POINT ( 'NONE',  ( -49.25565061422688728, -189.7472609257535510, -0.6300878435817132139 ) ) ;
#28128=EDGE_CURVE ( 'NONE', #30637, #48961, #39169, .T. ) ;
#28131=CARTESIAN_POINT ( 'NONE',  ( 64.46023522152408702, -193.5000000000000000, -51.19472891551279048 ) ) ;
#28132=VECTOR ( 'NONE', #27193, 1000.000000000000000 ) ;
#28133=VERTEX_POINT ( 'NONE', #36254 ) ;
#28135=DIRECTION ( 'NONE',  ( 0.000000000000000000, 0.000000000000000000, -1.000000000000000000 ) ) ;
#28136=DIRECTION ( 'NONE',  ( 0.000000000000000000, 1.000000000000000000, 0.000000000000000000 ) ) ;
#28138=DIRECTION ( 'NONE',  ( 0.000000000000000000, -1.000000000000000000, -0.000000000000000000 ) ) ;
#28139=ORIENTED_EDGE ( 'NONE', *, *, #37297, .F. ) ;
#28142=DIRECTION ( 'NONE',  ( 0.000000000000000000, 0.000000000000000000, -1.000000000000000000 ) ) ;
#28144=LINE ( 'NONE', #43673, #6448 ) ;
#28145=ADVANCED_FACE ( 'NONE', ( #51524 ), #16043, .F. ) ;
#28146=ORIENTED_EDGE ( 'NONE', *, *, #32946, .F. ) ;
#28147=DIRECTION ( 'NONE',  ( -1.000000000000000000, 0.000000000000000000, -0.000000000000000000 ) ) ;
#28148=VECTOR ( 'NONE', #35772, 1000.000000000000000 ) ;
#28151=VERTEX_POINT ( 'NONE', #48099 ) ;
#28152=CARTESIAN_POINT ( 'NONE',  ( -48.47912675150885065, -175.3837268820161057, -0.9999999999999931166 ) ) ;
#28153=VERTEX_POINT ( 'NONE', #31538 ) ;
#28154=DIRECTION ( 'NONE',  ( 0.9473263538541923934, 0.000000000000000000, -0.3202698538628350744 ) ) ;
#28155=FACE_OUTER_BOUND ( 'NONE', #27563, .T. ) ;
#28159=CARTESIAN_POINT ( 'NONE',  ( -85.14888725715768203, -175.3837268820161057, 119.5003291395398577 ) ) ;
#28160=VECTOR ( 'NONE', #6602, 1000.000000000000000 ) ;
#28161=FACE_OUTER_BOUND ( 'NONE', #29944, .T. ) ;
#28163=CARTESIAN_POINT ( 'NONE',  ( -132.4142998968131053, -193.5000000000000000, -91.27439114664585418 ) ) ;
#28164=ORIENTED_EDGE ( 'NONE', *, *, #22703, .T. ) ;
#28165=CIRCLE ( 'NONE', #8902, 124.9999999999999858 ) ;
#28166=AXIS2_PLACEMENT_3D ( 'NONE', #39968, #16084, #11617 ) ;
#28167=VERTEX_POINT ( 'NONE', #28100 ) ;
#28168=DIRECTION ( 'NONE',  ( -0.000000000000000000, 1.000000000000000000, -0.000000000000000000 ) ) ;
#28170=DIRECTION ( 'NONE',  ( -0.3482016354343928088, 0.000000000000000000, -0.9374196611341231167 ) ) ;
#28171=ORIENTED_EDGE ( 'NONE', *, *, #323, .T. ) ;
#28172=ORIENTED_EDGE ( 'NONE', *, *, #37810, .T. ) ;
#28176=VECTOR ( 'NONE', #645, 1000.000000000000227 ) ;
#28177=EDGE_CURVE ( 'NONE', #21402, #2898, #40202, .T. ) ;
#28178=ADVANCED_FACE ( 'NONE', ( #28371 ), #23156, .T. ) ;
#28179=EDGE_CURVE ( 'NONE', #9404, #14211, #38843, .T. ) ;
#28180=DIRECTION ( 'NONE',  ( 0.000000000000000000, 0.000000000000000000, 1.000000000000000000 ) ) ;
#28181=CARTESIAN_POINT ( 'NONE',  ( -48.47912675150885065, -175.3837268820161057, 6.938893903907228378E-15 ) ) ;
#28182=ORIENTED_EDGE ( 'NONE', *, *, #49485, .F. ) ;
#28184=EDGE_CURVE ( 'NONE', #8692, #27526, #40709, .T. ) ;
#28185=ORIENTED_EDGE ( 'NONE', *, *, #34387, .T. ) ;
#28186=VECTOR ( 'NONE', #15134, 1000.000000000000000 ) ;
#28187=DIRECTION ( 'NONE',  ( 0.000000000000000000, 0.000000000000000000, -1.000000000000000000 ) ) ;
#28188=CARTESIAN_POINT ( 'NONE',  ( -48.41988612361515010, -193.5000000000000000, 0.9982437317643287900 ) ) ;
#28190=ADVANCED_FACE ( 'NONE', ( #12865 ), #28884, .T. ) ;
#28191=DIRECTION ( 'NONE',  ( 0.9982437317643217956, 0.000000000000000000, -0.05924062789370748011 ) ) ;
#28193=ORIENTED_EDGE ( 'NONE', *, *, #47218, .F. ) ;
#28194=CYLINDRICAL_SURFACE ( 'NONE', #29719, 125.0000000000000000 ) ;
#28201=ORIENTED_EDGE ( 'NONE', *, *, #3807, .T. ) ;
#28204=AXIS2_PLACEMENT_3D ( 'NONE', #8003, #48489, #28479 ) ;
#28205=ADVANCED_FACE ( 'NONE', ( #5003 ), #33621, .F. ) ;
#28207=ORIENTED_EDGE ( 'NONE', *, *, #42635, .F. ) ;
#28211=EDGE_CURVE ( 'NONE', #44616, #6723, #37036, .T. ) ;
#28212=FACE_OUTER_BOUND ( 'NONE', #29115, .T. ) ;
#28216=ORIENTED_EDGE ( 'NONE', *, *, #29877, .T. ) ;
#28217=CARTESIAN_POINT ( 'NONE',  ( 65.12862465015753344, -183.6283474603465606, 49.69312418816388544 ) ) ;
#28219=PLANE ( 'NONE',  #12006 ) ;
#28222=CARTESIAN_POINT ( 'NONE',  ( -104.8182102393454045, -175.3837268820161057, 111.5836353223472770 ) ) ;
#28223=ORIENTED_EDGE ( 'NONE', *, *, #16336, .T. ) ;
#28224=VECTOR ( 'NONE', #34631, 1000.000000000000114 ) ;
#28225=AXIS2_PLACEMENT_3D ( 'NONE', #21380, #40296, #32689 ) ;
#28230=DIRECTION ( 'NONE',  ( 0.9890401873221644768, 0.000000000000000000, -0.1476465640024779702 ) ) ;
#28231=EDGE_CURVE ( 'NONE', #41178, #50666, #9201, .T. ) ;
#28232=ORIENTED_EDGE ( 'NONE', *, *, #27765, .F. ) ;
#28234=VECTOR ( 'NONE', #1121, 1000.000000000000000 ) ;
#28235=EDGE_LOOP ( 'NONE', ( #9220, #21698, #19550, #44321 ) ) ;
#28237=DIRECTION ( 'NONE',  ( -0.000000000000000000, 1.000000000000000000, -0.000000000000000000 ) ) ;
#28239=VERTEX_POINT ( 'NONE', #40451 ) ;
#28241=DIRECTION ( 'NONE',  ( 0.000000000000000000, -0.000000000000000000, -1.000000000000000000 ) ) ;
#28242=CARTESIAN_POINT ( 'NONE',  ( -48.47912675150885065, -189.7472609257535510, 6.938893903907228378E-15 ) ) ;
#28244=VECTOR ( 'NONE', #1938, 1000.000000000000000 ) ;
#28248=VERTEX_POINT ( 'NONE', #49144 ) ;
#28249=DIRECTION ( 'NONE',  ( -0.7378332790417189146, 0.000000000000000000, -0.6749830015182196608 ) ) ;
#28253=ADVANCED_FACE ( 'NONE', ( #5524 ), #29154, .T. ) ;
#28254=DIRECTION ( 'NONE',  ( -0.000000000000000000, 1.000000000000000000, 0.000000000000000000 ) ) ;
#28255=DIRECTION ( 'NONE',  ( 0.9890401873221644768, 0.000000000000000000, -0.1476465640024779702 ) ) ;
#28256=ORIENTED_EDGE ( 'NONE', *, *, #45533, .T. ) ;
#28260=EDGE_CURVE ( 'NONE', #52027, #31544, #45538, .T. ) ;
#28261=DIRECTION ( 'NONE',  ( 0.000000000000000000, -1.000000000000000000, 0.000000000000000000 ) ) ;
#28262=DIRECTION ( 'NONE',  ( -0.6965510290629932655, 0.000000000000000000, -0.7175072570443347120 ) ) ;
#28263=VECTOR ( 'NONE', #7430, 1000.000000000000114 ) ;
#28264=CIRCLE ( 'NONE', #41698, 125.0000000000000000 ) ;
#28265=DIRECTION ( 'NONE',  ( 0.000000000000000000, 0.000000000000000000, 1.000000000000000000 ) ) ;
#28266=AXIS2_PLACEMENT_3D ( 'NONE', #47621, #14524, #6886 ) ;
#28271=AXIS2_PLACEMENT_3D ( 'NONE', #42565, #14715, #14986 ) ;
#28275=EDGE_LOOP ( 'NONE', ( #35681, #15704, #47154, #31130 ) ) ;
#28276=EDGE_CURVE ( 'NONE', #43984, #43356, #49659, .T. ) ;
#28277=DIRECTION ( 'NONE',  ( 0.000000000000000000, 0.000000000000000000, 1.000000000000000000 ) ) ;
#28279=CARTESIAN_POINT ( 'NONE',  ( -167.1580984288391107, -189.7472609257535510, -39.24667733211878584 ) ) ;
#28281=ORIENTED_EDGE ( 'NONE', *, *, #50367, .F. ) ;
#28282=CARTESIAN_POINT ( 'NONE',  ( -11.80936624585915418, -189.7472609257535510, -119.5003291395395877 ) ) ;
#28283=ORIENTED_EDGE ( 'NONE', *, *, #5967, .T. ) ;
#28284=EDGE_CURVE ( 'NONE', #29227, #41086, #13396, .T. ) ;
#28285=VERTEX_POINT ( 'NONE', #36792 ) ;
#28286=CARTESIAN_POINT ( 'NONE',  ( -147.0463339291295881, -177.1207230881787780, 76.87330921200150158 ) ) ;
#28287=VECTOR ( 'NONE', #28648, 1000.000000000000000 ) ;
#28290=DIRECTION ( 'NONE',  ( -0.8124868780056863082, 0.000000000000000000, 0.5829794791144649047 ) ) ;
#28291=VECTOR ( 'NONE', #24251, 1000.000000000000000 ) ;
#28292=DIRECTION ( 'NONE',  ( 0.000000000000000000, -1.000000000000000000, 0.000000000000000000 ) ) ;
#28293=PLANE ( 'NONE',  #26211 ) ;
#28294=VERTEX_POINT ( 'NONE', #16832 ) ;
#28295=LINE ( 'NONE', #16221, #8714 ) ;
#28296=LINE ( 'NONE', #47771, #37442 ) ;
#28297=FACE_BOUND ( 'NONE', #18008, .T. ) ;
#28298=ORIENTED_EDGE ( 'NONE', *, *, #16616, .T. ) ;
#28300=AXIS2_PLACEMENT_3D ( 'NONE', #35756, #11595, #27866 ) ;
#28301=DIRECTION ( 'NONE',  ( -0.000000000000000000, 1.000000000000000000, -0.000000000000000000 ) ) ;
#28302=AXIS2_PLACEMENT_3D ( 'NONE', #44329, #17239, #40878 ) ;
#28304=ORIENTED_EDGE ( 'NONE', *, *, #27279, .T. ) ;
#28305=DIRECTION ( 'NONE',  ( 0.8124868780056825335, 0.000000000000000000, -0.5829794791144703447 ) ) ;
#28306=EDGE_CURVE ( 'NONE', #17420, #36143, #25422, .T. ) ;
#28308=ORIENTED_EDGE ( 'NONE', *, *, #33557, .T. ) ;
#28309=VECTOR ( 'NONE', #2152, 1000.000000000000000 ) ;
#28310=CARTESIAN_POINT ( 'NONE',  ( -26.37732090265850005, -175.3837268820161057, -122.0143860769387061 ) ) ;
#28313=EDGE_CURVE ( 'NONE', #37656, #41503, #44542, .T. ) ;
#28315=DIRECTION ( 'NONE',  ( 0.000000000000000000, 0.000000000000000000, 1.000000000000000000 ) ) ;
#28317=EDGE_LOOP ( 'NONE', ( #4629, #18038, #49822, #45226 ) ) ;
#28319=CIRCLE ( 'NONE', #16608, 125.0000000000000000 ) ;
#28320=ORIENTED_EDGE ( 'NONE', *, *, #51375, .F. ) ;
#28321=CARTESIAN_POINT ( 'NONE',  ( 51.05451324771860300, -193.5000000000000000, 75.61781872352698031 ) ) ;
#28322=CARTESIAN_POINT ( 'NONE',  ( -126.2322430781613889, -177.1207230881787780, 97.87467957288052389 ) ) ;
#28324=CARTESIAN_POINT ( 'NONE',  ( -48.47912675150885065, -177.1207230881787780, 6.938893903907228378E-15 ) ) ;
#28325=DIRECTION ( 'NONE',  ( -0.000000000000000000, 1.000000000000000000, -0.000000000000000000 ) ) ;
#28326=ORIENTED_EDGE ( 'NONE', *, *, #8789, .F. ) ;
#28327=DIRECTION ( 'NONE',  ( -0.6965510290629882695, 0.000000000000000000, -0.7175072570443395970 ) ) ;
#28333=VECTOR ( 'NONE', #22488, 1000.000000000000114 ) ;
#28334=CARTESIAN_POINT ( 'NONE',  ( -47.82630463331832971, -189.7472609257535510, -0.7575112421616121416 ) ) ;
#28335=EDGE_LOOP ( 'NONE', ( #18323, #18541, #24464, #34934 ) ) ;
#28336=DIRECTION ( 'NONE',  ( -0.2635871660690648488, 0.000000000000000000, -0.9646355819083595184 ) ) ;
#28337=ORIENTED_EDGE ( 'NONE', *, *, #28792, .F. ) ;
#28338=DIRECTION ( 'NONE',  ( 0.4031234292879792847, 0.000000000000000000, -0.9151456172430153524 ) ) ;
#28339=ORIENTED_EDGE ( 'NONE', *, *, #18626, .T. ) ;
#28344=AXIS2_PLACEMENT_3D ( 'NONE', #37326, #1062, #44704 ) ;
#28345=ORIENTED_EDGE ( 'NONE', *, *, #18769, .T. ) ;
#28346=DIRECTION ( 'NONE',  ( -0.9995608365087944591, 0.000000000000000000, 0.02963332782255633305 ) ) ;
#28347=CARTESIAN_POINT ( 'NONE',  ( 68.93474881819257405, -189.7472609257535510, 39.87457906003773900 ) ) ;
#28349=DIRECTION ( 'NONE',  ( 0.000000000000000000, -0.000000000000000000, -1.000000000000000000 ) ) ;
#28350=CARTESIAN_POINT ( 'NONE',  ( -124.9871112439422092, -175.3837268820161057, -98.85104101073277150 ) ) ;
#28351=CARTESIAN_POINT ( 'NONE',  ( 65.38692482895591240, -183.6283474603465606, -51.57055649762701677 ) ) ;
#28354=EDGE_CURVE ( 'NONE', #51222, #29810, #42212, .T. ) ;
#28355=DIRECTION ( 'NONE',  ( 0.6068001458185890984, 0.000000000000000000, 0.7948544414133565938 ) ) ;
#28356=CARTESIAN_POINT ( 'NONE',  ( -171.4462109067799247, -177.1207230881787780, 15.97798378892250426 ) ) ;
#28358=ORIENTED_EDGE ( 'NONE', *, *, #16231, .T. ) ;
#28359=VECTOR ( 'NONE', #41078, 1000.000000000000114 ) ;
#28360=DIRECTION ( 'NONE',  ( -0.8757349421956412971, 0.000000000000000000, 0.4827922027307366970 ) ) ;
#28361=AXIS2_PLACEMENT_3D ( 'NONE', #47143, #3259, #2984 ) ;
#28362=DIRECTION ( 'NONE',  ( 0.000000000000000000, 0.000000000000000000, 1.000000000000000000 ) ) ;
#28363=DIRECTION ( 'NONE',  ( -0.000000000000000000, 1.000000000000000000, -0.000000000000000000 ) ) ;
#28364=ORIENTED_EDGE ( 'NONE', *, *, #39701, .F. ) ;
#28365=ORIENTED_EDGE ( 'NONE', *, *, #34270, .F. ) ;
#28367=EDGE_CURVE ( 'NONE', #50110, #26396, #29543, .T. ) ;
#28368=VECTOR ( 'NONE', #39495, 1000.000000000000000 ) ;
#28370=DIRECTION ( 'NONE',  ( -0.000000000000000000, 1.000000000000000000, -0.000000000000000000 ) ) ;
#28371=FACE_OUTER_BOUND ( 'NONE', #28317, .T. ) ;
#28372=DIRECTION ( 'NONE',  ( 0.000000000000000000, 0.000000000000000000, -1.000000000000000000 ) ) ;
#28376=PLANE ( 'NONE',  #41942 ) ;
#28378=AXIS2_PLACEMENT_3D ( 'NONE', #4970, #474, #32549 ) ;
#28381=ORIENTED_EDGE ( 'NONE', *, *, #19825, .F. ) ;
#28382=DIRECTION ( 'NONE',  ( 0.7575112421616236880, 0.000000000000000000, -0.6528221181905174975 ) ) ;
#28383=CARTESIAN_POINT ( 'NONE',  ( -53.47502265695602119, -193.5000000000000000, -124.9001241957025883 ) ) ;
#28384=DIRECTION ( 'NONE',  ( 0.6965510290629882695, 0.000000000000000000, 0.7175072570443395970 ) ) ;
#28385=PLANE ( 'NONE',  #24986 ) ;
#28387=EDGE_LOOP ( 'NONE', ( #23958, #8034, #12374, #19251 ) ) ;
#28388=CIRCLE ( 'NONE', #12453, 125.0000000000000000 ) ;
#28389=CIRCLE ( 'NONE', #37641, 125.0000000000000000 ) ;
#28392=ORIENTED_EDGE ( 'NONE', *, *, #2575, .T. ) ;
#28393=CARTESIAN_POINT ( 'NONE',  ( -162.3451783319732442, -183.6283474603465606, 51.57055649762783389 ) ) ;
#28396=ORIENTED_EDGE ( 'NONE', *, *, #46811, .F. ) ;
#28397=DIRECTION ( 'NONE',  ( 0.2920567706369833760, 0.000000000000000000, -0.9564009842765202052 ) ) ;
#28398=PLANE ( 'NONE',  #4887 ) ;
#28399=CARTESIAN_POINT ( 'NONE',  ( 3.652658254809377336, -177.1207230881787780, -112.5098962032389522 ) ) ;
#28400=CARTESIAN_POINT ( 'NONE',  ( -48.47912675150885065, -175.3837268820161057, 6.938893903907228378E-15 ) ) ;
#28401=VERTEX_POINT ( 'NONE', #9329 ) ;
#28402=CIRCLE ( 'NONE', #38512, 125.0000000000000000 ) ;
#28408=CARTESIAN_POINT ( 'NONE',  ( -48.36085358058748795, -183.6283474603465606, 0.9929810960135245779 ) ) ;
#28409=ORIENTED_EDGE ( 'NONE', *, *, #29494, .T. ) ;
#28410=CARTESIAN_POINT ( 'NONE',  ( -48.47912675150885065, -177.1207230881787780, 6.938893903907228378E-15 ) ) ;
#28411=DIRECTION ( 'NONE',  ( -0.9960498426152171181, 0.000000000000000000, 0.08879589532293157006 ) ) ;
#28412=VECTOR ( 'NONE', #23326, 1000.000000000000000 ) ;
#28414=DIRECTION ( 'NONE',  ( 0.000000000000000000, 1.000000000000000000, -0.000000000000000000 ) ) ;
#28416=DIRECTION ( 'NONE',  ( 0.000000000000000000, 0.000000000000000000, 1.000000000000000000 ) ) ;
#28417=CARTESIAN_POINT ( 'NONE',  ( 67.04262753014327814, -189.7472609257535510, -47.74645837849745078 ) ) ;
#28418=CARTESIAN_POINT ( 'NONE',  ( -51.89154260666836649, -193.5000000000000000, 124.9534129907280828 ) ) ;
#28421=LINE ( 'NONE', #4790, #14885 ) ;
#28422=CARTESIAN_POINT ( 'NONE',  ( -48.53836737940257251, -177.1207230881787780, 0.9982437317643279018 ) ) ;
#28423=AXIS2_PLACEMENT_3D ( 'NONE', #36560, #28147, #4251 ) ;
#28424=CIRCLE ( 'NONE', #41876, 125.0000000000000000 ) ;
#28426=DIRECTION ( 'NONE',  ( -0.000000000000000000, 1.000000000000000000, -0.000000000000000000 ) ) ;
#28427=LINE ( 'NONE', #12132, #7725 ) ;
#28429=VECTOR ( 'NONE', #10997, 1000.000000000000000 ) ;
#28430=EDGE_LOOP ( 'NONE', ( #51698, #50410, #7452, #11319 ) ) ;
#28431=DIRECTION ( 'NONE',  ( 0.000000000000000000, 0.000000000000000000, -1.000000000000000000 ) ) ;
#28433=EDGE_CURVE ( 'NONE', #471, #7989, #5655, .T. ) ;
#28434=DIRECTION ( 'NONE',  ( 0.7948544414133565938, 0.000000000000000000, -0.6068001458185890984 ) ) ;
#28435=ORIENTED_EDGE ( 'NONE', *, *, #47505, .F. ) ;
#28436=AXIS2_PLACEMENT_3D ( 'NONE', #45655, #9642, #6491 ) ;
#28437=EDGE_LOOP ( 'NONE', ( #29503, #6241, #15675, #22391 ) ) ;
#28438=ADVANCED_FACE ( 'NONE', ( #25350 ), #41369, .F. ) ;
#28439=ORIENTED_EDGE ( 'NONE', *, *, #41074, .F. ) ;
#28440=FACE_OUTER_BOUND ( 'NONE', #35556, .T. ) ;
#28441=CARTESIAN_POINT ( 'NONE',  ( -48.47912675150885065, -189.7472609257535510, 6.938893903907228378E-15 ) ) ;
#28443=ORIENTED_EDGE ( 'NONE', *, *, #22155, .F. ) ;
#28444=ORIENTED_EDGE ( 'NONE', *, *, #2800, .T. ) ;
#28445=ORIENTED_EDGE ( 'NONE', *, *, #34552, .F. ) ;
#28449=CARTESIAN_POINT ( 'NONE',  ( -138.3705904895685705, -193.5000000000000000, -86.85922373029296750 ) ) ;
#28450=ORIENTED_EDGE ( 'NONE', *, *, #3196, .F. ) ;
#28453=VERTEX_POINT ( 'NONE', #34002 ) ;
#28455=DIRECTION ( 'NONE',  ( -0.8455960035018272869, 0.000000000000000000, 0.5338233779647886257 ) ) ;
#28457=DIRECTION ( 'NONE',  ( 0.000000000000000000, 1.000000000000000000, 0.000000000000000000 ) ) ;
#28459=ORIENTED_EDGE ( 'NONE', *, *, #20358, .T. ) ;
#28460=DIRECTION ( 'NONE',  ( 0.000000000000000000, 0.000000000000000000, 1.000000000000000000 ) ) ;
#28461=CARTESIAN_POINT ( 'NONE',  ( -47.55243714407702527, -175.3837268820161057, 0.3758275821142491591 ) ) ;
#28462=AXIS2_PLACEMENT_3D ( 'NONE', #33294, #9909, #25923 ) ;
#28463=ORIENTED_EDGE ( 'NONE', *, *, #5396, .T. ) ;
#28467=ORIENTED_EDGE ( 'NONE', *, *, #49685, .T. ) ;
#28468=DIRECTION ( 'NONE',  ( 0.000000000000000000, 0.000000000000000000, -1.000000000000000000 ) ) ;
#28469=DIRECTION ( 'NONE',  ( 0.000000000000000000, 0.000000000000000000, 1.000000000000000000 ) ) ;
#28471=LINE ( 'NONE', #40556, #34938 ) ;
#28472=ORIENTED_EDGE ( 'NONE', *, *, #18530, .T. ) ;
#28473=DIRECTION ( 'NONE',  ( -0.000000000000000000, 1.000000000000000000, -0.000000000000000000 ) ) ;
#28474=EDGE_LOOP ( 'NONE', ( #25493, #40723, #5993, #31697 ) ) ;
#28475=EDGE_CURVE ( 'NONE', #51761, #24816, #1433, .T. ) ;
#28478=DIRECTION ( 'NONE',  ( 0.000000000000000000, 0.000000000000000000, 1.000000000000000000 ) ) ;
#28479=DIRECTION ( 'NONE',  ( 0.000000000000000000, 0.000000000000000000, 1.000000000000000000 ) ) ;
#28481=CARTESIAN_POINT ( 'NONE',  ( -148.7414553014637590, -175.3837268820161057, 72.96212019587208886 ) ) ;
#28482=ADVANCED_FACE ( 'NONE', ( #22450 ), #7456, .F. ) ;
#28483=VECTOR ( 'NONE', #26184, 1000.000000000000000 ) ;
#28484=EDGE_LOOP ( 'NONE', ( #871, #6988, #40330, #47464 ) ) ;
#28485=DIRECTION ( 'NONE',  ( 0.000000000000000000, 0.000000000000000000, -1.000000000000000000 ) ) ;
#28487=ORIENTED_EDGE ( 'NONE', *, *, #43998, .F. ) ;
#28488=EDGE_CURVE ( 'NONE', #33930, #9394, #6928, .T. ) ;
#28489=CARTESIAN_POINT ( 'NONE',  ( -63.31390705753094039, -189.7472609257535510, 123.1094209424469312 ) ) ;
#28490=DIRECTION ( 'NONE',  ( 0.000000000000000000, 1.000000000000000000, 0.000000000000000000 ) ) ;
#28491=ORIENTED_EDGE ( 'NONE', *, *, #6285, .F. ) ;
#28493=ORIENTED_EDGE ( 'NONE', *, *, #6409, .F. ) ;
#28494=CARTESIAN_POINT ( 'NONE',  ( -32.87124591993210743, -175.3837268820161057, 124.0217483183788261 ) ) ;
#28495=ADVANCED_FACE ( 'NONE', ( #18251 ), #27404, .F. ) ;
#28496=EDGE_CURVE ( 'NONE', #29784, #49553, #46368, .T. ) ;
#28497=EDGE_CURVE ( 'NONE', #31354, #24136, #41394, .T. ) ;
#28499=ORIENTED_EDGE ( 'NONE', *, *, #24411, .F. ) ;
#28500=EDGE_CURVE ( 'NONE', #30377, #8106, #46625, .T. ) ;
#28502=CARTESIAN_POINT ( 'NONE',  ( -27.18512803868276251, -189.7472609257535510, -123.1729094355498404 ) ) ;
#28504=CARTESIAN_POINT ( 'NONE',  ( -75.48985759771373694, -177.1207230881787780, -122.0467960216648606 ) ) ;
#28508=CARTESIAN_POINT ( 'NONE',  ( -144.0067397530739299, -177.1207230881787780, -80.61932246194588458 ) ) ;
#28509=ORIENTED_EDGE ( 'NONE', *, *, #41070, .T. ) ;
#28512=FACE_OUTER_BOUND ( 'NONE', #16136, .T. ) ;
#28514=CARTESIAN_POINT ( 'NONE',  ( 38.46761263173351608, -175.3837268820161057, 89.80681772907068705 ) ) ;
#28517=ORIENTED_EDGE ( 'NONE', *, *, #42015, .T. ) ;
#28518=ADVANCED_FACE ( 'NONE', ( #11369 ), #31089, .T. ) ;
#28519=AXIS2_PLACEMENT_3D ( 'NONE', #23998, #4039, #44494 ) ;
#28520=VECTOR ( 'NONE', #30838, 1000.000000000000000 ) ;
#28521=VERTEX_POINT ( 'NONE', #47389 ) ;
#28522=CARTESIAN_POINT ( 'NONE',  ( -49.35486169370449971, -177.1207230881787780, 0.4827922027307437469 ) ) ;
#28523=EDGE_LOOP ( 'NONE', ( #38425, #10, #13209, #43173 ) ) ;
#28524=ORIENTED_EDGE ( 'NONE', *, *, #35478, .F. ) ;
#28525=CARTESIAN_POINT ( 'NONE',  ( -133.0671220150036049, -183.6283474603465606, -92.03190238880748097 ) ) ;
#28526=CARTESIAN_POINT ( 'NONE',  ( -149.5539421794694306, -189.7472609257535510, 73.54509967498654532 ) ) ;
#28527=DIRECTION ( 'NONE',  ( 0.9785564922995046988, 0.000000000000000000, -0.2059786187410953262 ) ) ;
#28528=CARTESIAN_POINT ( 'NONE',  ( -48.47912675150885065, -175.3837268820161057, 6.938893903907228378E-15 ) ) ;
#28532=EDGE_CURVE ( 'NONE', #29008, #13637, #24586, .T. ) ;
#28534=DIRECTION ( 'NONE',  ( 0.000000000000000000, 1.000000000000000000, 0.000000000000000000 ) ) ;
#28535=VECTOR ( 'NONE', #29290, 1000.000000000000114 ) ;
#28537=CARTESIAN_POINT ( 'NONE',  ( -48.47912675150885065, -183.6283474603465606, 6.938893903907228378E-15 ) ) ;
#28538=DIRECTION ( 'NONE',  ( -0.000000000000000000, 1.000000000000000000, -0.000000000000000000 ) ) ;
#28539=ADVANCED_FACE ( 'NONE', ( #26886 ), #2977, .T. ) ;
#28541=EDGE_CURVE ( 'NONE', #43643, #11866, #29610, .T. ) ;
#28543=DIRECTION ( 'NONE',  ( 0.000000000000000000, -0.000000000000000000, 1.000000000000000000 ) ) ;
#28545=ORIENTED_EDGE ( 'NONE', *, *, #25254, .F. ) ;
#28546=DIRECTION ( 'NONE',  ( 0.000000000000000000, -1.000000000000000000, -0.000000000000000000 ) ) ;
#28548=EDGE_CURVE ( 'NONE', #4246, #43850, #30845, .T. ) ;
#28549=CARTESIAN_POINT ( 'NONE',  ( 75.28414827670442833, -193.5000000000000000, -7.666780576874961284 ) ) ;
#28550=FACE_BOUND ( 'NONE', #16993, .T. ) ;
#28551=ORIENTED_EDGE ( 'NONE', *, *, #15648, .F. ) ;
#28552=EDGE_CURVE ( 'NONE', #25351, #11371, #39242, .T. ) ;
#28553=CARTESIAN_POINT ( 'NONE',  ( -172.2804936848317823, -193.5000000000000000, -7.024906801078567575 ) ) ;
#28556=ORIENTED_EDGE ( 'NONE', *, *, #33535, .F. ) ;
#28558=EDGE_CURVE ( 'NONE', #39566, #28133, #31609, .T. ) ;
#28560=AXIS2_PLACEMENT_3D ( 'NONE', #27864, #47087, #22908 ) ;
#28561=EDGE_CURVE ( 'NONE', #19688, #38326, #37193, .T. ) ;
#28562=VECTOR ( 'NONE', #38391, 1000.000000000000000 ) ;
#28563=DIRECTION ( 'NONE',  ( 0.000000000000000000, 0.000000000000000000, 1.000000000000000000 ) ) ;
#28566=FACE_OUTER_BOUND ( 'NONE', #19738, .T. ) ;
#28567=ORIENTED_EDGE ( 'NONE', *, *, #41059, .T. ) ;
#28568=EDGE_CURVE ( 'NONE', #6875, #2378, #28773, .T. ) ;
#28569=CARTESIAN_POINT ( 'NONE',  ( 48.47907891923915713, -175.3837268820161057, 78.89300572996904748 ) ) ;
#28570=ORIENTED_EDGE ( 'NONE', *, *, #49778, .T. ) ;
#28571=ADVANCED_FACE ( 'NONE', ( #48431 ), #27921, .T. ) ;
#28572=ORIENTED_EDGE ( 'NONE', *, *, #9405, .T. ) ;
#28573=CARTESIAN_POINT ( 'NONE',  ( 9.336583202542589888, -189.7472609257535510, 110.8257356506556306 ) ) ;
#28574=AXIS2_PLACEMENT_3D ( 'NONE', #21476, #49600, #17282 ) ;
#28575=ORIENTED_EDGE ( 'NONE', *, *, #14112, .T. ) ;
#28577=CARTESIAN_POINT ( 'NONE',  ( 30.50828161901820224, -177.1207230881787780, 96.88131563365348597 ) ) ;
#28578=CYLINDRICAL_SURFACE ( 'NONE', #22995, 125.0000000000000000 ) ;
#28579=EDGE_CURVE ( 'NONE', #20140, #45478, #11643, .T. ) ;
#28582=ORIENTED_EDGE ( 'NONE', *, *, #42547, .F. ) ;
#28583=DIRECTION ( 'NONE',  ( -0.000000000000000000, 1.000000000000000000, -0.000000000000000000 ) ) ;
#28587=DIRECTION ( 'NONE',  ( 0.000000000000000000, 1.000000000000000000, -0.000000000000000000 ) ) ;
#28588=ORIENTED_EDGE ( 'NONE', *, *, #26417, .F. ) ;
#28590=AXIS2_PLACEMENT_3D ( 'NONE', #33431, #33670, #25522 ) ;
#28593=DIRECTION ( 'NONE',  ( 0.8455960035018311727, 0.000000000000000000, -0.5338233779647826305 ) ) ;
#28595=CARTESIAN_POINT ( 'NONE',  ( -48.07600332222088468, -193.5000000000000000, 0.9151456172430280089 ) ) ;
#28596=CARTESIAN_POINT ( 'NONE',  ( -48.82732838694323618, -177.1207230881787780, -0.9374196611341184537 ) ) ;
#28598=AXIS2_PLACEMENT_3D ( 'NONE', #24428, #12332, #40193 ) ;
#28599=ORIENTED_EDGE ( 'NONE', *, *, #31579, .F. ) ;
#28602=CARTESIAN_POINT ( 'NONE',  ( 64.01121016852529522, -189.7472609257535510, -54.50618404930953176 ) ) ;
#28603=DIRECTION ( 'NONE',  ( 0.000000000000000000, -1.000000000000000000, 0.000000000000000000 ) ) ;
#28605=CARTESIAN_POINT ( 'NONE',  ( -48.47912675150883643, -213.5000000000000000, -125.0000000000000568 ) ) ;
#28606=ADVANCED_FACE ( 'NONE', ( #24252 ), #27670, .F. ) ;
#28607=EDGE_CURVE ( 'NONE', #1605, #49769, #8218, .T. ) ;
#28609=DIRECTION ( 'NONE',  ( 0.8294056854501971054, 0.000000000000000000, 0.5586467658036594619 ) ) ;
#28610=CARTESIAN_POINT ( 'NONE',  ( 6.039888445539280504, -183.6283474603465606, 111.3726929437940498 ) ) ;
#28611=LINE ( 'NONE', #41757, #48333 ) ;
#28612=CARTESIAN_POINT ( 'NONE',  ( -238.7407812814481076, -213.5000000000000000, 41.45482488023466772 ) ) ;
#28613=ORIENTED_EDGE ( 'NONE', *, *, #28681, .T. ) ;
#28614=ORIENTED_EDGE ( 'NONE', *, *, #17023, .T. ) ;
#28615=VECTOR ( 'NONE', #5140, 1000.000000000000000 ) ;
#28617=CARTESIAN_POINT ( 'NONE',  ( -48.47912675150885065, -177.1207230881787780, 6.938893903907228378E-15 ) ) ;
#28618=DIRECTION ( 'NONE',  ( 0.000000000000000000, 0.000000000000000000, 1.000000000000000000 ) ) ;
#28620=ORIENTED_EDGE ( 'NONE', *, *, #17404, .T. ) ;
#28621=VERTEX_POINT ( 'NONE', #12663 ) ;
#28622=DIRECTION ( 'NONE',  ( -0.9720229140804139689, 0.000000000000000000, 0.2348860457809708036 ) ) ;
#28623=DIRECTION ( 'NONE',  ( 0.000000000000000000, 0.000000000000000000, 1.000000000000000000 ) ) ;
#28624=EDGE_CURVE ( 'NONE', #30907, #45145, #10340, .T. ) ;
#28625=CARTESIAN_POINT ( 'NONE',  ( -153.7332855749581881, -175.3837268820161057, 67.42819922234390617 ) ) ;
#28628=VERTEX_POINT ( 'NONE', #320 ) ;
#28631=ORIENTED_EDGE ( 'NONE', *, *, #26113, .F. ) ;
#28634=CARTESIAN_POINT ( 'NONE',  ( -78.00521078983979351, -175.3837268820161057, 121.4627941443857253 ) ) ;
#28635=ORIENTED_EDGE ( 'NONE', *, *, #31118, .F. ) ;
#28637=DIRECTION ( 'NONE',  ( -0.7765238627180437447, 0.000000000000000000, 0.6300878435817094392 ) ) ;
#28638=VECTOR ( 'NONE', #29660, 1000.000000000000000 ) ;
#28639=PLANE ( 'NONE',  #10780 ) ;
#28642=DIRECTION ( 'NONE',  ( -0.000000000000000000, 1.000000000000000000, -0.000000000000000000 ) ) ;
#28644=AXIS2_PLACEMENT_3D ( 'NONE', #35819, #12670, #16116 ) ;
#28645=CARTESIAN_POINT ( 'NONE',  ( -21.46839590530488451, -183.6283474603465606, 122.0467960216650738 ) ) ;
#28646=ORIENTED_EDGE ( 'NONE', *, *, #49903, .F. ) ;
#28648=DIRECTION ( 'NONE',  ( -0.000000000000000000, 1.000000000000000000, -0.000000000000000000 ) ) ;
#28649=ORIENTED_EDGE ( 'NONE', *, *, #11307, .T. ) ;
#28652=DIRECTION ( 'NONE',  ( 0.000000000000000000, 0.000000000000000000, -1.000000000000000000 ) ) ;
#28653=PLANE ( 'NONE',  #9747 ) ;
#28657=DIRECTION ( 'NONE',  ( -0.7378332790417189146, 0.000000000000000000, -0.6749830015182196608 ) ) ;
#28659=ORIENTED_EDGE ( 'NONE', *, *, #49650, .T. ) ;
#28660=DIRECTION ( 'NONE',  ( -0.000000000000000000, 1.000000000000000000, -0.000000000000000000 ) ) ;
#28663=CARTESIAN_POINT ( 'NONE',  ( 52.59568867645218404, -189.7472609257535510, -73.54509967498589162 ) ) ;
#28664=VERTEX_POINT ( 'NONE', #12408 ) ;
#28665=ADVANCED_FACE ( 'NONE', ( #32124 ), #48170, .F. ) ;
#28667=CARTESIAN_POINT ( 'NONE',  ( -105.4063847101409692, -175.3837268820161057, -111.2847127925096373 ) ) ;
#28669=DIRECTION ( 'NONE',  ( 0.000000000000000000, 0.000000000000000000, -1.000000000000000000 ) ) ;
#28671=LINE ( 'NONE', #23961, #7180 ) ;
#28672=DIRECTION ( 'NONE',  ( 0.05924062789370748011, 0.000000000000000000, 0.9982437317643217956 ) ) ;
#28674=LINE ( 'NONE', #50434, #45762 ) ;
#28675=DIRECTION ( 'NONE',  ( -0.2348860457809775482, 0.000000000000000000, -0.9720229140804121926 ) ) ;
#28676=VECTOR ( 'NONE', #14559, 1000.000000000000227 ) ;
#28678=VECTOR ( 'NONE', #12216, 1000.000000000000227 ) ;
#28679=VECTOR ( 'NONE', #14133, 1000.000000000000114 ) ;
#28680=CARTESIAN_POINT ( 'NONE',  ( -173.0563034899574859, -175.3837268820161057, -10.27263529369817618 ) ) ;
#28681=EDGE_CURVE ( 'NONE', #37834, #51354, #1099, .T. ) ;
#28683=PLANE ( 'NONE',  #5232 ) ;
#28684=VERTEX_POINT ( 'NONE', #15592 ) ;
#28686=DIRECTION ( 'NONE',  ( -0.000000000000000000, 1.000000000000000000, -0.000000000000000000 ) ) ;
#28687=DIRECTION ( 'NONE',  ( 0.000000000000000000, 0.000000000000000000, -1.000000000000000000 ) ) ;
#28690=ORIENTED_EDGE ( 'NONE', *, *, #48797, .F. ) ;
#28691=LINE ( 'NONE', #7706, #6557 ) ;
#28693=LINE ( 'NONE', #24771, #4316 ) ;
#28695=ORIENTED_EDGE ( 'NONE', *, *, #3369, .T. ) ;
#28697=AXIS2_PLACEMENT_3D ( 'NONE', #28883, #25222, #44934 ) ;
#28699=FACE_OUTER_BOUND ( 'NONE', #18832, .T. ) ;
#28700=DIRECTION ( 'NONE',  ( -0.000000000000000000, 1.000000000000000000, -0.000000000000000000 ) ) ;
#28701=EDGE_LOOP ( 'NONE', ( #24747, #37455, #6454, #33726 ) ) ;
#28702=CARTESIAN_POINT ( 'NONE',  ( 60.58466639580034041, -189.7472609257535510, -61.07445476073405644 ) ) ;
#28703=LINE ( 'NONE', #32667, #51613 ) ;
#28705=DIRECTION ( 'NONE',  ( 0.000000000000000000, 1.000000000000000000, 0.000000000000000000 ) ) ;
#28706=ORIENTED_EDGE ( 'NONE', *, *, #44831, .T. ) ;
#28708=CARTESIAN_POINT ( 'NONE',  ( 55.10060313344061456, -193.5000000000000000, 68.17212999877224888 ) ) ;
#28713=EDGE_CURVE ( 'NONE', #35017, #22103, #589, .T. ) ;
#28715=VECTOR ( 'NONE', #12528, 1000.000000000000114 ) ;
#28716=ORIENTED_EDGE ( 'NONE', *, *, #19275, .T. ) ;
#28717=AXIS2_PLACEMENT_3D ( 'NONE', #34785, #26662, #50845 ) ;
#28718=DIRECTION ( 'NONE',  ( 0.000000000000000000, -1.000000000000000000, 0.000000000000000000 ) ) ;
#28721=LINE ( 'NONE', #4840, #39262 ) ;
#28722=CARTESIAN_POINT ( 'NONE',  ( -95.72791768350688812, -177.1207230881787780, -115.7261930397105232 ) ) ;
#28724=EDGE_CURVE ( 'NONE', #10667, #27207, #2790, .T. ) ;
#28725=CARTESIAN_POINT ( 'NONE',  ( 71.09073365861578964, -189.7472609257535510, 32.84887689123991095 ) ) ;
#28726=ADVANCED_FACE ( 'NONE', ( #23724 ), #39730, .F. ) ;
#28729=DIRECTION ( 'NONE',  ( 0.000000000000000000, -0.000000000000000000, 1.000000000000000000 ) ) ;
#28730=ORIENTED_EDGE ( 'NONE', *, *, #11232, .F. ) ;
#28732=DIRECTION ( 'NONE',  ( 0.000000000000000000, 0.000000000000000000, -1.000000000000000000 ) ) ;
#28733=VERTEX_POINT ( 'NONE', #41048 ) ;
#28736=LINE ( 'NONE', #13508, #29759 ) ;
#28738=DIRECTION ( 'NONE',  ( 0.000000000000000000, 0.000000000000000000, 1.000000000000000000 ) ) ;
#28739=AXIS2_PLACEMENT_3D ( 'NONE', #22371, #14756, #22890 ) ;
#28740=ORIENTED_EDGE ( 'NONE', *, *, #16543, .F. ) ;
#28741=CARTESIAN_POINT ( 'NONE',  ( -48.47912675150885065, -189.7472609257535510, 6.938893903907228378E-15 ) ) ;
#28742=ORIENTED_EDGE ( 'NONE', *, *, #44512, .T. ) ;
#28745=DIRECTION ( 'NONE',  ( 0.000000000000000000, 0.000000000000000000, 1.000000000000000000 ) ) ;
#28746=DIRECTION ( 'NONE',  ( -0.000000000000000000, 1.000000000000000000, -0.000000000000000000 ) ) ;
#28747=EDGE_LOOP ( 'NONE', ( #4592, #31121, #9574, #20657 ) ) ;
#28749=FACE_OUTER_BOUND ( 'NONE', #34329, .T. ) ;
#28750=VECTOR ( 'NONE', #35676, 1000.000000000000000 ) ;
#28751=DIRECTION ( 'NONE',  ( 0.000000000000000000, 0.000000000000000000, 1.000000000000000000 ) ) ;
#28752=AXIS2_PLACEMENT_3D ( 'NONE', #36653, #657, #20101 ) ;
#28753=CIRCLE ( 'NONE', #41332, 125.0000000000000000 ) ;
#28754=EDGE_LOOP ( 'NONE', ( #47904, #16767, #41898, #1300 ) ) ;
#28756=ORIENTED_EDGE ( 'NONE', *, *, #23303, .T. ) ;
#28757=LINE ( 'NONE', #16712, #13232 ) ;
#28758=PLANE ( 'NONE',  #34193 ) ;
#28759=VECTOR ( 'NONE', #45455, 999.9999999999998863 ) ;
#28760=CARTESIAN_POINT ( 'NONE',  ( 69.25251857196690253, -193.5000000000000000, 38.92640747825684144 ) ) ;
#28762=ORIENTED_EDGE ( 'NONE', *, *, #19282, .T. ) ;
#28763=ORIENTED_EDGE ( 'NONE', *, *, #18108, .T. ) ;
#28766=DIRECTION ( 'NONE',  ( 0.000000000000000000, -1.000000000000000000, 0.000000000000000000 ) ) ;
#28769=DIRECTION ( 'NONE',  ( 0.5586467658036535777, 0.000000000000000000, -0.8294056854502011022 ) ) ;
#28770=ORIENTED_EDGE ( 'NONE', *, *, #46344, .T. ) ;
#28771=EDGE_CURVE ( 'NONE', #48639, #18266, #49210, .T. ) ;
#28773=CIRCLE ( 'NONE', #32164, 125.0000000000000000 ) ;
#28774=VERTEX_POINT ( 'NONE', #25284 ) ;
#28775=CARTESIAN_POINT ( 'NONE',  ( -8.721998590732194856, -193.5000000000000000, -118.5089480183145270 ) ) ;
#28776=VERTEX_POINT ( 'NONE', #16891 ) ;
#28777=VERTEX_POINT ( 'NONE', #25040 ) ;
#28778=CARTESIAN_POINT ( 'NONE',  ( 2.066935079424583765, -175.3837268820161057, -114.3245189510257802 ) ) ;
#28781=PLANE ( 'NONE',  #27599 ) ;
#28782=ORIENTED_EDGE ( 'NONE', *, *, #15658, .T. ) ;
#28785=AXIS2_PLACEMENT_3D ( 'NONE', #2897, #42839, #6846 ) ;
#28787=CIRCLE ( 'NONE', #6165, 125.0000000000000000 ) ;
#28788=EDGE_CURVE ( 'NONE', #4396, #44477, #48948, .T. ) ;
#28789=VERTEX_POINT ( 'NONE', #41559 ) ;
#28790=DIRECTION ( 'NONE',  ( 0.000000000000000000, -1.000000000000000000, 0.000000000000000000 ) ) ;
#28792=EDGE_CURVE ( 'NONE', #48639, #47918, #37887, .T. ) ;
#28794=PLANE ( 'NONE',  #46330 ) ;
#28795=DIRECTION ( 'NONE',  ( 0.000000000000000000, -0.000000000000000000, -1.000000000000000000 ) ) ;
#28798=CARTESIAN_POINT ( 'NONE',  ( 18.82962626094778003, -177.1207230881787780, 104.1428419024404377 ) ) ;
#28799=DIRECTION ( 'NONE',  ( 0.000000000000000000, -1.000000000000000000, 0.000000000000000000 ) ) ;
#28800=DIRECTION ( 'NONE',  ( -0.000000000000000000, 1.000000000000000000, -0.000000000000000000 ) ) ;
#28801=VECTOR ( 'NONE', #35671, 1000.000000000000114 ) ;
#28802=ORIENTED_EDGE ( 'NONE', *, *, #4358, .T. ) ;
#28803=CARTESIAN_POINT ( 'NONE',  ( -147.6585554144535024, -177.1207230881787780, 76.08180419845385245 ) ) ;
#28804=DIRECTION ( 'NONE',  ( 0.000000000000000000, -1.000000000000000000, -0.000000000000000000 ) ) ;
#28805=DIRECTION ( 'NONE',  ( -0.000000000000000000, 1.000000000000000000, -0.000000000000000000 ) ) ;
#28806=FACE_BOUND ( 'NONE', #14453, .T. ) ;
#28807=ORIENTED_EDGE ( 'NONE', *, *, #22338, .F. ) ;
#28808=PLANE ( 'NONE',  #8006 ) ;
#28809=ORIENTED_EDGE ( 'NONE', *, *, #19979, .F. ) ;
#28812=ORIENTED_EDGE ( 'NONE', *, *, #46940, .F. ) ;
#28813=LINE ( 'NONE', #51993, #28801 ) ;
#28814=ORIENTED_EDGE ( 'NONE', *, *, #20865, .F. ) ;
#28818=CARTESIAN_POINT ( 'NONE',  ( -40.96347969518279797, -175.3837268820161057, -123.7720294769269032 ) ) ;
#28823=ORIENTED_EDGE ( 'NONE', *, *, #33944, .F. ) ;
#28826=AXIS2_PLACEMENT_3D ( 'NONE', #15955, #3587, #27755 ) ;
#28827=DIRECTION ( 'NONE',  ( 0.000000000000000000, -1.000000000000000000, 0.000000000000000000 ) ) ;
#28830=CARTESIAN_POINT ( 'NONE',  ( -29.85296035031868911, -183.6283474603465606, 122.5936119678275986 ) ) ;
#28831=PLANE ( 'NONE',  #7865 ) ;
#28832=EDGE_CURVE ( 'NONE', #45987, #51254, #23803, .T. ) ;
#28833=EDGE_CURVE ( 'NONE', #43088, #17428, #12878, .T. ) ;
#28834=EDGE_CURVE ( 'NONE', #5601, #24900, #20829, .T. ) ;
#28835=ADVANCED_FACE ( 'NONE', ( #29474 ), #5330, .T. ) ;
#28836=CARTESIAN_POINT ( 'NONE',  ( -145.6517069852673103, -189.7472609257535510, 78.62880929222940551 ) ) ;
#28838=ORIENTED_EDGE ( 'NONE', *, *, #40126, .T. ) ;
#28839=FACE_OUTER_BOUND ( 'NONE', #15287, .T. ) ;
#28840=CARTESIAN_POINT ( 'NONE',  ( -49.21696003055058810, -193.5000000000000000, 0.6749830015182108900 ) ) ;
#28842=ORIENTED_EDGE ( 'NONE', *, *, #23359, .T. ) ;
#28843=EDGE_CURVE ( 'NONE', #29027, #12470, #7003, .T. ) ;
#28844=CARTESIAN_POINT ( 'NONE',  ( -70.42295845586424718, -189.7472609257535510, -123.0587999703025162 ) ) ;
#28847=VECTOR ( 'NONE', #33859, 1000.000000000000227 ) ;
#28848=ORIENTED_EDGE ( 'NONE', *, *, #32441, .T. ) ;
#28850=CARTESIAN_POINT ( 'NONE',  ( -47.66663987350317200, -175.3837268820161057, -0.5829794791144634614 ) ) ;
#28851=ORIENTED_EDGE ( 'NONE', *, *, #14687, .T. ) ;
#28852=EDGE_CURVE ( 'NONE', #38380, #42973, #42255, .T. ) ;
#28854=VERTEX_POINT ( 'NONE', #34460 ) ;
#28856=EDGE_CURVE ( 'NONE', #45319, #43465, #48157, .T. ) ;
#28857=ORIENTED_EDGE ( 'NONE', *, *, #11531, .F. ) ;
#28858=DIRECTION ( 'NONE',  ( 0.000000000000000000, 0.000000000000000000, 1.000000000000000000 ) ) ;
#28860=EDGE_CURVE ( 'NONE', #34735, #9360, #30511, .T. ) ;
#28861=CARTESIAN_POINT ( 'NONE',  ( 73.80528149577284580, -193.5000000000000000, 25.91377046305969145 ) ) ;
#28862=CARTESIAN_POINT ( 'NONE',  ( -123.4791267515088435, -198.5000000000000000, 80.00000000000000000 ) ) ;
#28863=VERTEX_POINT ( 'NONE', #22643 ) ;
#28865=EDGE_CURVE ( 'NONE', #23646, #44424, #30514, .T. ) ;
#28867=DIRECTION ( 'NONE',  ( 0.3202698538628416247, 0.000000000000000000, -0.9473263538541900619 ) ) ;
#28868=AXIS2_PLACEMENT_3D ( 'NONE', #39876, #3905, #12025 ) ;
#28871=EDGE_CURVE ( 'NONE', #17942, #6329, #15417, .T. ) ;
#28872=LINE ( 'NONE', #44659, #46699 ) ;
#28875=DIRECTION ( 'NONE',  ( 0.000000000000000000, -1.000000000000000000, 0.000000000000000000 ) ) ;
#28876=CARTESIAN_POINT ( 'NONE',  ( -140.8230258362169707, -175.3837268820161057, 84.24728067916045404 ) ) ;
#28877=FACE_OUTER_BOUND ( 'NONE', #26775, .T. ) ;
#28879=ORIENTED_EDGE ( 'NONE', *, *, #46344, .F. ) ;
#28880=ORIENTED_EDGE ( 'NONE', *, *, #24891, .T. ) ;
#28883=CARTESIAN_POINT ( 'NONE',  ( -47.55243714407702527, -189.7472609257535510, 0.3758275821142491591 ) ) ;
#28884=PLANE ( 'NONE',  #21222 ) ;
#28885=DIRECTION ( 'NONE',  ( 0.000000000000000000, -1.000000000000000000, -0.000000000000000000 ) ) ;
#28887=ORIENTED_EDGE ( 'NONE', *, *, #43712, .F. ) ;
#28888=VECTOR ( 'NONE', #39141, 1000.000000000000000 ) ;
#28889=CARTESIAN_POINT ( 'NONE',  ( -48.47912675150885065, -189.7472609257535510, 6.938893903907228378E-15 ) ) ;
#28890=CARTESIAN_POINT ( 'NONE',  ( -121.1142239062970560, -177.1207230881787780, 101.7307360698549132 ) ) ;
#28891=VERTEX_POINT ( 'NONE', #46824 ) ;
#28893=FACE_OUTER_BOUND ( 'NONE', #51245, .T. ) ;
#28894=VERTEX_POINT ( 'NONE', #50763 ) ;
#28897=DIRECTION ( 'NONE',  ( 0.6300878435817148793, 0.000000000000000000, -0.7765238627180394149 ) ) ;
#28898=ADVANCED_FACE ( 'NONE', ( #46561 ), #2917, .T. ) ;
#28899=EDGE_CURVE ( 'NONE', #51292, #43700, #10044, .T. ) ;
#28900=CIRCLE ( 'NONE', #8763, 125.0000000000000000 ) ;
#28901=EDGE_CURVE ( 'NONE', #18053, #38078, #18698, .T. ) ;
#28902=EDGE_CURVE ( 'NONE', #14774, #5680, #34710, .T. ) ;
#28903=CARTESIAN_POINT ( 'NONE',  ( 30.50828161901820224, -193.5000000000000000, 96.88131563365348597 ) ) ;
#28904=CARTESIAN_POINT ( 'NONE',  ( 42.10477485469927927, -193.5000000000000000, 86.13684908212515268 ) ) ;
#28905=DIRECTION ( 'NONE',  ( 0.000000000000000000, 1.000000000000000000, -0.000000000000000000 ) ) ;
#28907=ORIENTED_EDGE ( 'NONE', *, *, #23057, .T. ) ;
#28908=DIRECTION ( 'NONE',  ( 0.000000000000000000, 0.000000000000000000, 1.000000000000000000 ) ) ;
#28910=CARTESIAN_POINT ( 'NONE',  ( 75.17589904515342880, -175.3837268820161057, -18.28755301364250130 ) ) ;
#28913=DIRECTION ( 'NONE',  ( 0.000000000000000000, 0.000000000000000000, 1.000000000000000000 ) ) ;
#28914=CARTESIAN_POINT ( 'NONE',  ( -102.0975050429524487, -177.1207230881787780, -111.8087531435654256 ) ) ;
#28915=PLANE ( 'NONE',  #6372 ) ;
#28916=ORIENTED_EDGE ( 'NONE', *, *, #28843, .F. ) ;
#28917=FACE_OUTER_BOUND ( 'NONE', #9164, .T. ) ;
#28919=DIRECTION ( 'NONE',  ( 0.000000000000000000, 0.000000000000000000, -1.000000000000000000 ) ) ;
#28921=EDGE_LOOP ( 'NONE', ( #28095, #27082, #8031, #14825 ) ) ;
#28922=FACE_OUTER_BOUND ( 'NONE', #15841, .T. ) ;
#28924=CARTESIAN_POINT ( 'NONE',  ( -48.47912675150885065, -193.5000000000000000, -0.9999999999999931166 ) ) ;
#28925=AXIS2_PLACEMENT_3D ( 'NONE', #41004, #21043, #41260 ) ;
#28926=DIRECTION ( 'NONE',  ( 0.000000000000000000, 1.000000000000000000, 0.000000000000000000 ) ) ;
#28927=CIRCLE ( 'NONE', #32260, 125.0000000000000000 ) ;
#28928=VERTEX_POINT ( 'NONE', #31028 ) ;
#28929=DIRECTION ( 'NONE',  ( 0.000000000000000000, 0.000000000000000000, 1.000000000000000000 ) ) ;
#28931=EDGE_CURVE ( 'NONE', #35, #14481, #6354, .T. ) ;
#28932=CARTESIAN_POINT ( 'NONE',  ( -48.59739992243022755, -175.3837268820161057, 0.9929810960135230236 ) ) ;
#28933=ORIENTED_EDGE ( 'NONE', *, *, #28856, .F. ) ;
#28934=DIRECTION ( 'NONE',  ( 0.000000000000000000, 0.000000000000000000, 1.000000000000000000 ) ) ;
#28935=DIRECTION ( 'NONE',  ( 0.1476465640024710868, 0.000000000000000000, 0.9890401873221654760 ) ) ;
#28936=VECTOR ( 'NONE', #16004, 1000.000000000000114 ) ;
#28939=CARTESIAN_POINT ( 'NONE',  ( -161.8276685539205744, -193.5000000000000000, 50.28156562190586953 ) ) ;
#28940=VECTOR ( 'NONE', #10310, 1000.000000000000000 ) ;
#28941=DIRECTION ( 'NONE',  ( 0.000000000000000000, 0.000000000000000000, 1.000000000000000000 ) ) ;
#28942=CARTESIAN_POINT ( 'NONE',  ( 26.52087324849106054, -198.5000000000000000, -70.00000000000002842 ) ) ;
#28943=CARTESIAN_POINT ( 'NONE',  ( 24.15597040328003331, -183.6283474603465606, -101.7307360698544159 ) ) ;
#28944=DIRECTION ( 'NONE',  ( 0.000000000000000000, 0.000000000000000000, 1.000000000000000000 ) ) ;
#28947=DIRECTION ( 'NONE',  ( 0.9960498426152165630, 0.000000000000000000, 0.08879589532293852283 ) ) ;
#28948=ORIENTED_EDGE ( 'NONE', *, *, #10104, .F. ) ;
#28949=ORIENTED_EDGE ( 'NONE', *, *, #42562, .F. ) ;
#28950=CIRCLE ( 'NONE', #33130, 125.0000000000000000 ) ;
#28952=DIRECTION ( 'NONE',  ( -0.000000000000000000, -1.000000000000000000, 0.000000000000000000 ) ) ;
#28955=EDGE_CURVE ( 'NONE', #39789, #16540, #45653, .T. ) ;
#28956=DIRECTION ( 'NONE',  ( 0.000000000000000000, 1.000000000000000000, 0.000000000000000000 ) ) ;
#28957=FACE_OUTER_BOUND ( 'NONE', #42829, .T. ) ;
#28958=ORIENTED_EDGE ( 'NONE', *, *, #46279, .T. ) ;
#28959=VERTEX_POINT ( 'NONE', #15025 ) ;
#28960=VECTOR ( 'NONE', #4652, 999.9999999999998863 ) ;
#28962=DIRECTION ( 'NONE',  ( -0.4031234292879600778, 0.000000000000000000, -0.9151456172430237901 ) ) ;
#28965=CIRCLE ( 'NONE', #25606, 125.0000000000000000 ) ;
#28966=DIRECTION ( 'NONE',  ( 0.000000000000000000, -0.000000000000000000, 1.000000000000000000 ) ) ;
#28967=ORIENTED_EDGE ( 'NONE', *, *, #19405, .T. ) ;
#28968=FACE_OUTER_BOUND ( 'NONE', #7749, .T. ) ;
#28971=LINE ( 'NONE', #25309, #4681 ) ;
#28972=CARTESIAN_POINT ( 'NONE',  ( -173.1763543514842070, -177.1207230881787780, 8.694908215728872847 ) ) ;
#28973=AXIS2_PLACEMENT_3D ( 'NONE', #45037, #17700, #8488 ) ;
#28974=VERTEX_POINT ( 'NONE', #18443 ) ;
#28975=ORIENTED_EDGE ( 'NONE', *, *, #20026, .T. ) ;
#28978=VERTEX_POINT ( 'NONE', #10544 ) ;
#28979=ADVANCED_FACE ( 'NONE', ( #11053 ), #27080, .T. ) ;
#28980=DIRECTION ( 'NONE',  ( -0.000000000000000000, 1.000000000000000000, -0.000000000000000000 ) ) ;
#28981=CARTESIAN_POINT ( 'NONE',  ( 56.28386853063362594, -193.5000000000000000, 66.33788548805519270 ) ) ;
#28983=CARTESIAN_POINT ( 'NONE',  ( 38.46761263173351608, -193.5000000000000000, 89.80681772907068705 ) ) ;
#28985=EDGE_LOOP ( 'NONE', ( #17586, #51214, #4309, #43752 ) ) ;
#28988=FACE_BOUND ( 'NONE', #30808, .T. ) ;
#28989=AXIS2_PLACEMENT_3D ( 'NONE', #38944, #30295, #30547 ) ;
#28990=PLANE ( 'NONE',  #48054 ) ;
#28992=EDGE_LOOP ( 'NONE', ( #10700, #46083, #41692, #45035 ) ) ;
#28993=CIRCLE ( 'NONE', #33209, 125.0000000000000000 ) ;
#28995=DIRECTION ( 'NONE',  ( -0.6528221181905227155, 0.000000000000000000, 0.7575112421616191360 ) ) ;
#28996=FACE_OUTER_BOUND ( 'NONE', #26204, .T. ) ;
#28998=ADVANCED_FACE ( 'NONE', ( #30182 ), #25717, .T. ) ;
#28999=CARTESIAN_POINT ( 'NONE',  ( 31.84037011350117297, -189.7472609257535510, -94.47107458416900272 ) ) ;
#29001=DIRECTION ( 'NONE',  ( 0.000000000000000000, 0.000000000000000000, -1.000000000000000000 ) ) ;
#29002=ORIENTED_EDGE ( 'NONE', *, *, #33599, .T. ) ;
#29003=ORIENTED_EDGE ( 'NONE', *, *, #51644, .T. ) ;
#29007=CARTESIAN_POINT ( 'NONE',  ( -132.4142998968130769, -183.6283474603465606, -91.27439114664586839 ) ) ;
#29008=VERTEX_POINT ( 'NONE', #46224 ) ;
#29011=DIRECTION ( 'NONE',  ( -0.000000000000000000, -1.000000000000000000, 0.000000000000000000 ) ) ;
#29016=DIRECTION ( 'NONE',  ( -0.000000000000000000, 1.000000000000000000, -0.000000000000000000 ) ) ;
#29018=FACE_OUTER_BOUND ( 'NONE', #48577, .T. ) ;
#29019=ORIENTED_EDGE ( 'NONE', *, *, #8217, .T. ) ;
#29021=DIRECTION ( 'NONE',  ( -0.000000000000000000, 1.000000000000000000, -0.000000000000000000 ) ) ;
#29024=DIRECTION ( 'NONE',  ( -0.000000000000000000, 1.000000000000000000, -0.000000000000000000 ) ) ;
#29026=EDGE_LOOP ( 'NONE', ( #35364, #29629, #48382, #39270 ) ) ;
#29027=VERTEX_POINT ( 'NONE', #33601 ) ;
#29030=ADVANCED_FACE ( 'NONE', ( #21522 ), #1795, .T. ) ;
#29032=CIRCLE ( 'NONE', #8076, 125.0000000000000000 ) ;
#29033=FACE_OUTER_BOUND ( 'NONE', #23364, .T. ) ;
#29034=AXIS2_PLACEMENT_3D ( 'NONE', #27819, #43857, #11273 ) ;
#29036=LINE ( 'NONE', #41133, #1223 ) ;
#29037=EDGE_LOOP ( 'NONE', ( #42003, #22668, #2745, #42026 ) ) ;
#29038=AXIS2_PLACEMENT_3D ( 'NONE', #51514, #6338, #20751 ) ;
#29039=VERTEX_POINT ( 'NONE', #26218 ) ;
#29040=DIRECTION ( 'NONE',  ( -0.000000000000000000, 1.000000000000000000, -0.000000000000000000 ) ) ;
#29041=ORIENTED_EDGE ( 'NONE', *, *, #34498, .T. ) ;
#29042=VERTEX_POINT ( 'NONE', #17590 ) ;
#29043=CARTESIAN_POINT ( 'NONE',  ( -28.74596282265200387, -193.5000000000000000, 123.4325817657431230 ) ) ;
#29044=CIRCLE ( 'NONE', #21532, 125.0000000000000000 ) ;
#29045=EDGE_CURVE ( 'NONE', #44067, #42973, #50171, .T. ) ;
#29046=DIRECTION ( 'NONE',  ( 0.000000000000000000, 0.000000000000000000, 1.000000000000000000 ) ) ;
#29047=AXIS2_PLACEMENT_3D ( 'NONE', #37149, #16691, #17721 ) ;
#29048=CIRCLE ( 'NONE', #24985, 125.0000000000000000 ) ;
#29049=LINE ( 'NONE', #8822, #30496 ) ;
#29056=ORIENTED_EDGE ( 'NONE', *, *, #49931, .T. ) ;
#29057=CARTESIAN_POINT ( 'NONE',  ( -47.51449116960048968, -193.5000000000000000, -0.2635871660690578544 ) ) ;
#29059=DIRECTION ( 'NONE',  ( -0.000000000000000000, 1.000000000000000000, -0.000000000000000000 ) ) ;
#29060=CARTESIAN_POINT ( 'NONE',  ( -19.92568551777507224, -193.5000000000000000, -121.6951149130962904 ) ) ;
#29062=FACE_OUTER_BOUND ( 'NONE', #27405, .T. ) ;
#29063=ORIENTED_EDGE ( 'NONE', *, *, #44573, .F. ) ;
#29064=CARTESIAN_POINT ( 'NONE',  ( -48.47912675150885065, -177.1207230881787780, 6.938893903907228378E-15 ) ) ;
#29067=FACE_BOUND ( 'NONE', #47712, .T. ) ;
#29069=AXIS2_PLACEMENT_3D ( 'NONE', #6727, #21721, #38518 ) ;
#29070=AXIS2_PLACEMENT_3D ( 'NONE', #35280, #11357, #14552 ) ;
#29072=ORIENTED_EDGE ( 'NONE', *, *, #7953, .T. ) ;
#29073=AXIS2_PLACEMENT_3D ( 'NONE', #46446, #49869, #10426 ) ;
#29075=EDGE_CURVE ( 'NONE', #2077, #34754, #49895, .T. ) ;
#29076=ORIENTED_EDGE ( 'NONE', *, *, #8806, .F. ) ;
#29078=LINE ( 'NONE', #1747, #42234 ) ;
#29079=CARTESIAN_POINT ( 'NONE',  ( -68.21229068036655008, -177.1207230881787780, -123.4325817657429809 ) ) ;
#29080=AXIS2_PLACEMENT_3D ( 'NONE', #35513, #35776, #14797 ) ;
#29081=LINE ( 'NONE', #21215, #8314 ) ;
#29082=AXIS2_PLACEMENT_3D ( 'NONE', #30863, #2996, #51606 ) ;
#29083=DIRECTION ( 'NONE',  ( -0.000000000000000000, -1.000000000000000000, 0.000000000000000000 ) ) ;
#29084=ORIENTED_EDGE ( 'NONE', *, *, #47518, .F. ) ;
#29085=VECTOR ( 'NONE', #17340, 1000.000000000000000 ) ;
#29086=VECTOR ( 'NONE', #13371, 1000.000000000000000 ) ;
#29090=EDGE_LOOP ( 'NONE', ( #15777, #8753, #27301, #23190 ) ) ;
#29091=ORIENTED_EDGE ( 'NONE', *, *, #6256, .F. ) ;
#29092=EDGE_CURVE ( 'NONE', #12643, #19641, #29913, .T. ) ;
#29093=ORIENTED_EDGE ( 'NONE', *, *, #33000, .F. ) ;
#29094=CARTESIAN_POINT ( 'NONE',  ( 116.9235303384055840, -193.5000000000000000, -9.999999999999971578 ) ) ;
#29095=DIRECTION ( 'NONE',  ( 0.6965510290630033685, 0.000000000000000000, -0.7175072570443249420 ) ) ;
#29096=EDGE_CURVE ( 'NONE', #16039, #19239, #17836, .T. ) ;
#29098=DIRECTION ( 'NONE',  ( 0.000000000000000000, -0.000000000000000000, 1.000000000000000000 ) ) ;
#29100=CARTESIAN_POINT ( 'NONE',  ( -47.63353074800703268, -193.5000000000000000, 0.5338233779648018373 ) ) ;
#29101=VERTEX_POINT ( 'NONE', #6005 ) ;
#29102=EDGE_CURVE ( 'NONE', #19173, #33563, #4487, .T. ) ;
#29105=ORIENTED_EDGE ( 'NONE', *, *, #32930, .T. ) ;
#29106=DIRECTION ( 'NONE',  ( 0.000000000000000000, 0.000000000000000000, 1.000000000000000000 ) ) ;
#29107=CARTESIAN_POINT ( 'NONE',  ( -162.7543581613524282, -183.6283474603465606, 50.65739320402011003 ) ) ;
#29108=VERTEX_POINT ( 'NONE', #33078 ) ;
#29110=ORIENTED_EDGE ( 'NONE', *, *, #29211, .T. ) ;
#29111=VECTOR ( 'NONE', #39412, 1000.000000000000000 ) ;
#29112=DIRECTION ( 'NONE',  ( 0.5085311186492154079, 0.000000000000000000, 0.8610436117673585521 ) ) ;
#29113=EDGE_LOOP ( 'NONE', ( #50623, #9722, #16804, #280 ) ) ;
#29115=EDGE_LOOP ( 'NONE', ( #42757, #21193, #20413, #24576 ) ) ;
#29118=CARTESIAN_POINT ( 'NONE',  ( -16.77927958806651887, -183.6283474603465606, -120.9136869416130082 ) ) ;
#29119=ORIENTED_EDGE ( 'NONE', *, *, #32776, .F. ) ;
#29122=ORIENTED_EDGE ( 'NONE', *, *, #49749, .F. ) ;
#29124=VECTOR ( 'NONE', #26957, 999.9999999999998863 ) ;
#29129=ORIENTED_EDGE ( 'NONE', *, *, #37829, .T. ) ;
#29130=CIRCLE ( 'NONE', #6496, 125.0000000000000000 ) ;
#29131=CARTESIAN_POINT ( 'NONE',  ( -49.45768324380835423, -183.6283474603465606, -0.2059786187411025149 ) ) ;
#29135=CIRCLE ( 'NONE', #8165, 125.0000000000000000 ) ;
#29137=DIRECTION ( 'NONE',  ( 0.000000000000000000, -1.000000000000000000, 0.000000000000000000 ) ) ;
#29138=VECTOR ( 'NONE', #42820, 1000.000000000000227 ) ;
#29140=ORIENTED_EDGE ( 'NONE', *, *, #4293, .F. ) ;
#29142=CARTESIAN_POINT ( 'NONE',  ( -45.06671089634843952, -177.1207230881787780, -124.9534129907280544 ) ) ;
#29143=DIRECTION ( 'NONE',  ( -0.9960498426152158968, 0.000000000000000000, -0.08879589532294571153 ) ) ;
#29144=ADVANCED_FACE ( 'NONE', ( #43292 ), #26479, .T. ) ;
#29145=ORIENTED_EDGE ( 'NONE', *, *, #15954, .F. ) ;
#29146=ADVANCED_FACE ( 'NONE', ( #15450 ), #34626, .T. ) ;
#29148=EDGE_LOOP ( 'NONE', ( #22795, #19207, #23033, #39225 ) ) ;
#29149=EDGE_CURVE ( 'NONE', #51044, #32234, #37235, .T. ) ;
#29150=DIRECTION ( 'NONE',  ( 0.000000000000000000, -0.000000000000000000, 1.000000000000000000 ) ) ;
#29152=EDGE_CURVE ( 'NONE', #50966, #47996, #47503, .T. ) ;
#29154=PLANE ( 'NONE',  #34640 ) ;
#29157=VECTOR ( 'NONE', #40713, 1000.000000000000000 ) ;
#29158=EDGE_LOOP ( 'NONE', ( #12688, #34429, #26656, #46902 ) ) ;
#29160=EDGE_CURVE ( 'NONE', #17350, #44424, #14941, .T. ) ;
#29162=EDGE_CURVE ( 'NONE', #9912, #48105, #46994, .T. ) ;
#29163=DIRECTION ( 'NONE',  ( 0.000000000000000000, 1.000000000000000000, -0.000000000000000000 ) ) ;
#29165=CARTESIAN_POINT ( 'NONE',  ( -48.47912675150885065, -177.1207230881787780, 6.938893903907228378E-15 ) ) ;
#29167=EDGE_CURVE ( 'NONE', #51235, #51254, #47254, .T. ) ;
#29168=AXIS2_PLACEMENT_3D ( 'NONE', #16313, #24718, #48375 ) ;
#29169=ORIENTED_EDGE ( 'NONE', *, *, #39302, .F. ) ;
#29170=DIRECTION ( 'NONE',  ( -0.000000000000000000, 1.000000000000000000, -0.000000000000000000 ) ) ;
#29172=EDGE_CURVE ( 'NONE', #27213, #7756, #10974, .T. ) ;
#29173=VECTOR ( 'NONE', #39394, 1000.000000000000000 ) ;
#29175=LINE ( 'NONE', #9213, #19998 ) ;
#29176=CARTESIAN_POINT ( 'NONE',  ( -69.77312546433407192, -189.7472609257535510, 123.1729094355500109 ) ) ;
#29179=ORIENTED_EDGE ( 'NONE', *, *, #26318, .T. ) ;
#29182=CARTESIAN_POINT ( 'NONE',  ( -67.22356632362124174, -177.1207230881787780, -123.5865930638409509 ) ) ;
#29183=DIRECTION ( 'NONE',  ( -0.000000000000000000, 1.000000000000000000, 0.000000000000000000 ) ) ;
#29184=VERTEX_POINT ( 'NONE', #26997 ) ;
#29189=EDGE_CURVE ( 'NONE', #47995, #48520, #27165, .T. ) ;
#29190=ORIENTED_EDGE ( 'NONE', *, *, #48436, .F. ) ;
#29191=FACE_OUTER_BOUND ( 'NONE', #10976, .T. ) ;
#29192=AXIS2_PLACEMENT_3D ( 'NONE', #4304, #27951, #622 ) ;
#29193=DIRECTION ( 'NONE',  ( -0.000000000000000000, 1.000000000000000000, -0.000000000000000000 ) ) ;
#29194=AXIS2_PLACEMENT_3D ( 'NONE', #9169, #25195, #37271 ) ;
#29195=DIRECTION ( 'NONE',  ( 0.9266896074318317078, 0.000000000000000000, 0.3758275821142421647 ) ) ;
#29197=LINE ( 'NONE', #34180, #31561 ) ;
#29198=DIRECTION ( 'NONE',  ( 0.000000000000000000, -0.000000000000000000, 1.000000000000000000 ) ) ;
#29200=CIRCLE ( 'NONE', #35912, 9.999999999999994671 ) ;
#29201=DIRECTION ( 'NONE',  ( -0.1768902751225592818, 0.000000000000000000, -0.9842305779475992722 ) ) ;
#29203=CARTESIAN_POINT ( 'NONE',  ( 1.755575411425451593, -175.3837268820161057, 114.4616734920527392 ) ) ;
#29205=EDGE_CURVE ( 'NONE', #29027, #34600, #3349, .T. ) ;
#29206=LINE ( 'NONE', #12644, #14031 ) ;
#29207=ORIENTED_EDGE ( 'NONE', *, *, #25799, .T. ) ;
#29209=CARTESIAN_POINT ( 'NONE',  ( -161.4019114581580823, -175.3837268820161057, 53.60452120946281696 ) ) ;
#29210=DIRECTION ( 'NONE',  ( 0.9890401873221654760, 0.000000000000000000, -0.1476465640024710868 ) ) ;
#29211=EDGE_CURVE ( 'NONE', #25859, #12134, #14665, .T. ) ;
#29216=EDGE_CURVE ( 'NONE', #9326, #48404, #13758, .T. ) ;
#29218=AXIS2_PLACEMENT_3D ( 'NONE', #32265, #36212, #31234 ) ;
#29220=DIRECTION ( 'NONE',  ( 0.8455960035018234011, 0.000000000000000000, 0.5338233779647948429 ) ) ;
#29221=PLANE ( 'NONE',  #32059 ) ;
#29223=ORIENTED_EDGE ( 'NONE', *, *, #37589, .F. ) ;
#29224=FACE_OUTER_BOUND ( 'NONE', #42749, .T. ) ;
#29225=DIRECTION ( 'NONE',  ( 0.000000000000000000, 1.000000000000000000, -0.000000000000000000 ) ) ;
#29227=VERTEX_POINT ( 'NONE', #38577 ) ;
#29228=AXIS2_PLACEMENT_3D ( 'NONE', #39965, #12379, #19741 ) ;
#29229=VECTOR ( 'NONE', #33534, 1000.000000000000000 ) ;
#29230=ORIENTED_EDGE ( 'NONE', *, *, #1381, .F. ) ;
#29234=DIRECTION ( 'NONE',  ( 0.000000000000000000, -0.000000000000000000, 1.000000000000000000 ) ) ;
#29236=EDGE_CURVE ( 'NONE', #14954, #19312, #31201, .T. ) ;
#29237=DIRECTION ( 'NONE',  ( 0.000000000000000000, 0.000000000000000000, 1.000000000000000000 ) ) ;
#29238=EDGE_LOOP ( 'NONE', ( #45608, #41784, #17193, #25377 ) ) ;
#29239=ADVANCED_FACE ( 'NONE', ( #11225 ), #27251, .T. ) ;
#29240=CARTESIAN_POINT ( 'NONE',  ( 72.12732647922463514, -183.6283474603465606, 28.81338593824056460 ) ) ;
#29241=AXIS2_PLACEMENT_3D ( 'NONE', #50198, #5800, #21555 ) ;
#29244=CARTESIAN_POINT ( 'NONE',  ( 74.31448861501728231, -177.1207230881787780, -23.38221600314289361 ) ) ;
#29245=ORIENTED_EDGE ( 'NONE', *, *, #7610, .T. ) ;
#29246=FACE_OUTER_BOUND ( 'NONE', #1474, .T. ) ;
#29247=VERTEX_POINT ( 'NONE', #19895 ) ;
#29248=CARTESIAN_POINT ( 'NONE',  ( 75.67769207106684348, -183.6283474603465606, 14.49428645563876827 ) ) ;
#29250=CARTESIAN_POINT ( 'NONE',  ( -154.0877180371535360, -189.7472609257535510, -66.87170886601934683 ) ) ;
#29253=EDGE_LOOP ( 'NONE', ( #8811, #25696, #15364, #19345 ) ) ;
#29255=LINE ( 'NONE', #5354, #27500 ) ;
#29258=DIRECTION ( 'NONE',  ( 0.000000000000000000, -1.000000000000000000, 0.000000000000000000 ) ) ;
#29261=CARTESIAN_POINT ( 'NONE',  ( 73.09196206113300320, -183.6283474603465606, 29.07697310430964421 ) ) ;
#29263=CARTESIAN_POINT ( 'NONE',  ( 35.67816836544797354, -183.6283474603465606, -92.42591454022746689 ) ) ;
#29264=ORIENTED_EDGE ( 'NONE', *, *, #4640, .T. ) ;
#29266=CIRCLE ( 'NONE', #39319, 125.0000000000000000 ) ;
#29268=VECTOR ( 'NONE', #20976, 1000.000000000000114 ) ;
#29270=VERTEX_POINT ( 'NONE', #170 ) ;
#29271=VECTOR ( 'NONE', #34655, 1000.000000000000000 ) ;
#29273=LINE ( 'NONE', #45326, #17171 ) ;
#29274=CARTESIAN_POINT ( 'NONE',  ( -87.28630321566649286, -193.5000000000000000, 118.8234112238818341 ) ) ;
#29276=ADVANCED_FACE ( 'NONE', ( #16217 ), #44065, .T. ) ;
#29277=CARTESIAN_POINT ( 'NONE',  ( -53.47502265695599277, -183.6283474603465606, -124.9001241957025883 ) ) ;
#29279=DIRECTION ( 'NONE',  ( 0.000000000000000000, 0.000000000000000000, -1.000000000000000000 ) ) ;
#29280=ORIENTED_EDGE ( 'NONE', *, *, #49642, .T. ) ;
#29281=ORIENTED_EDGE ( 'NONE', *, *, #14250, .T. ) ;
#29283=CARTESIAN_POINT ( 'NONE',  ( 54.46899307705341187, -193.5000000000000000, -70.89911581792813422 ) ) ;
#29284=CARTESIAN_POINT ( 'NONE',  ( -145.2888470698896981, -175.3837268820161057, -77.48473115145237955 ) ) ;
#29285=ORIENTED_EDGE ( 'NONE', *, *, #11519, .T. ) ;
#29287=LINE ( 'NONE', #1432, #34128 ) ;
#29288=AXIS2_PLACEMENT_3D ( 'NONE', #37532, #34365, #37782 ) ;
#29290=DIRECTION ( 'NONE',  ( 0.6965510290629932655, 0.000000000000000000, 0.7175072570443347120 ) ) ;
#29291=ORIENTED_EDGE ( 'NONE', *, *, #38223, .F. ) ;
#29292=DIRECTION ( 'NONE',  ( 0.000000000000000000, 0.000000000000000000, 1.000000000000000000 ) ) ;
#29294=VERTEX_POINT ( 'NONE', #40362 ) ;
#29295=CARTESIAN_POINT ( 'NONE',  ( -44.48323084606168720, -183.6283474603465606, 123.9361149384469769 ) ) ;
#29297=CARTESIAN_POINT ( 'NONE',  ( -163.0741914257288272, -189.7472609257535510, 47.37063079638398477 ) ) ;
#29298=CARTESIAN_POINT ( 'NONE',  ( -24.23284180386169240, -183.6283474603465606, -121.6072260099953439 ) ) ;
#29299=EDGE_LOOP ( 'NONE', ( #50946, #18451, #26793, #47619 ) ) ;
#29301=EDGE_CURVE ( 'NONE', #35839, #42243, #39588, .T. ) ;
#29304=DIRECTION ( 'NONE',  ( -0.9995608365087946812, 0.000000000000000000, 0.02963332782254913048 ) ) ;
#29306=CARTESIAN_POINT ( 'NONE',  ( -33.86391487983340909, -189.7472609257535510, 124.1426420773540684 ) ) ;
#29307=DIRECTION ( 'NONE',  ( 0.000000000000000000, -0.000000000000000000, 1.000000000000000000 ) ) ;
#29313=ORIENTED_EDGE ( 'NONE', *, *, #26234, .T. ) ;
#29314=DIRECTION ( 'NONE',  ( 0.8757349421956412971, 0.000000000000000000, -0.4827922027307366970 ) ) ;
#29315=CYLINDRICAL_SURFACE ( 'NONE', #15760, 124.9999999999999858 ) ;
#29317=DIRECTION ( 'NONE',  ( -0.000000000000000000, 1.000000000000000000, -0.000000000000000000 ) ) ;
#29318=CYLINDRICAL_SURFACE ( 'NONE', #10837, 125.0000000000000000 ) ;
#29319=ORIENTED_EDGE ( 'NONE', *, *, #4969, .T. ) ;
#29320=CARTESIAN_POINT ( 'NONE',  ( 9.518239912201957864, -213.5000000000000000, 110.7307791902283043 ) ) ;
#29321=ORIENTED_EDGE ( 'NONE', *, *, #13441, .T. ) ;
#29323=ADVANCED_FACE ( 'NONE', ( #7804 ), #8575, .T. ) ;
#29324=ORIENTED_EDGE ( 'NONE', *, *, #18260, .F. ) ;
#29326=DIRECTION ( 'NONE',  ( -0.6528221181905280446, 0.000000000000000000, 0.7575112421616145841 ) ) ;
#29327=ORIENTED_EDGE ( 'NONE', *, *, #15065, .F. ) ;
#29328=DIRECTION ( 'NONE',  ( 0.000000000000000000, 0.000000000000000000, 1.000000000000000000 ) ) ;
#29329=DIRECTION ( 'NONE',  ( -0.5829794791144820021, 0.000000000000000000, 0.8124868780056742068 ) ) ;
#29330=CARTESIAN_POINT ( 'NONE',  ( -48.47912675150885065, -189.7472609257535510, 6.938893903907228378E-15 ) ) ;
#29331=EDGE_CURVE ( 'NONE', #30477, #26117, #31372, .T. ) ;
#29332=DIRECTION ( 'NONE',  ( -0.1182731709213592358, 0.000000000000000000, -0.9929810960135178055 ) ) ;
#29333=DIRECTION ( 'NONE',  ( -0.000000000000000000, 1.000000000000000000, -0.000000000000000000 ) ) ;
#29334=DIRECTION ( 'NONE',  ( 0.000000000000000000, -0.000000000000000000, -1.000000000000000000 ) ) ;
#29336=VERTEX_POINT ( 'NONE', #32500 ) ;
#29337=EDGE_CURVE ( 'NONE', #1331, #9353, #40620, .T. ) ;
#29338=VECTOR ( 'NONE', #35353, 1000.000000000000000 ) ;
#29339=DIRECTION ( 'NONE',  ( -0.000000000000000000, 1.000000000000000000, -0.000000000000000000 ) ) ;
#29341=FACE_OUTER_BOUND ( 'NONE', #731, .T. ) ;
#29342=ORIENTED_EDGE ( 'NONE', *, *, #47325, .T. ) ;
#29344=VERTEX_POINT ( 'NONE', #4641 ) ;
#29349=EDGE_CURVE ( 'NONE', #7460, #45794, #11230, .T. ) ;
#29352=ORIENTED_EDGE ( 'NONE', *, *, #9633, .T. ) ;
#29353=AXIS2_PLACEMENT_3D ( 'NONE', #51175, #10689, #2296 ) ;
#29355=EDGE_LOOP ( 'NONE', ( #29416, #16638, #6917, #44030 ) ) ;
#29356=CARTESIAN_POINT ( 'NONE',  ( -173.4291566779743050, -175.3837268820161057, 3.534122433558353205 ) ) ;
#29357=CARTESIAN_POINT ( 'NONE',  ( -149.7090673587773040, -175.3837268820161057, -71.61357856150524981 ) ) ;
#29358=ORIENTED_EDGE ( 'NONE', *, *, #42856, .T. ) ;
#29359=LINE ( 'NONE', #12806, #9179 ) ;
#29360=DIRECTION ( 'NONE',  ( 0.000000000000000000, 0.000000000000000000, -1.000000000000000000 ) ) ;
#29361=CARTESIAN_POINT ( 'NONE',  ( -4.794493649713349015, -189.7472609257535510, -117.1181148702518726 ) ) ;
#29362=ORIENTED_EDGE ( 'NONE', *, *, #29744, .T. ) ;
#29363=DIRECTION ( 'NONE',  ( 0.4300652022765115712, 0.000000000000000000, 0.9027978299657477557 ) ) ;
#29366=LINE ( 'NONE', #40936, #3028 ) ;
#29367=CARTESIAN_POINT ( 'NONE',  ( 38.71172987070723082, -189.7472609257535510, -89.56983042009264295 ) ) ;
#29368=VERTEX_POINT ( 'NONE', #3871 ) ;
#29369=ORIENTED_EDGE ( 'NONE', *, *, #18374, .T. ) ;
#29370=AXIS2_PLACEMENT_3D ( 'NONE', #15024, #31027, #43116 ) ;
#29372=DIRECTION ( 'NONE',  ( -0.000000000000000000, 1.000000000000000000, -0.000000000000000000 ) ) ;
#29373=ORIENTED_EDGE ( 'NONE', *, *, #17686, .T. ) ;
#29374=EDGE_CURVE ( 'NONE', #2592, #31707, #15455, .T. ) ;
#29375=FACE_OUTER_BOUND ( 'NONE', #16469, .T. ) ;
#29376=LINE ( 'NONE', #40413, #13315 ) ;
#29377=ORIENTED_EDGE ( 'NONE', *, *, #27298, .F. ) ;
#29380=EDGE_CURVE ( 'NONE', #16447, #25328, #38081, .T. ) ;
#29381=ORIENTED_EDGE ( 'NONE', *, *, #29448, .T. ) ;
#29383=DIRECTION ( 'NONE',  ( -0.3482016354344059095, 0.000000000000000000, 0.9374196611341183427 ) ) ;
#29385=CARTESIAN_POINT ( 'NONE',  ( -111.3904503173946381, -175.3837268820161057, -106.8558168688113454 ) ) ;
#29387=DIRECTION ( 'NONE',  ( -0.000000000000000000, 1.000000000000000000, -0.000000000000000000 ) ) ;
#29388=CARTESIAN_POINT ( 'NONE',  ( 43.63512310656540905, -189.7472609257535510, 84.49831343337136502 ) ) ;
#29390=DIRECTION ( 'NONE',  ( 0.000000000000000000, -0.000000000000000000, -1.000000000000000000 ) ) ;
#29391=ADVANCED_FACE ( 'NONE', ( #19634 ), #16479, .F. ) ;
#29392=CARTESIAN_POINT ( 'NONE',  ( -160.9694636715425702, -175.3837268820161057, 54.50618404931039862 ) ) ;
#29393=LINE ( 'NONE', #17594, #18135 ) ;
#29394=ADVANCED_FACE ( 'NONE', ( #11995 ), #12257, .T. ) ;
#29395=ADVANCED_FACE ( 'NONE', ( #707 ), #16754, .T. ) ;
#29399=ORIENTED_EDGE ( 'NONE', *, *, #16951, .F. ) ;
#29401=DIRECTION ( 'NONE',  ( -0.000000000000000000, 1.000000000000000000, -0.000000000000000000 ) ) ;
#29402=CARTESIAN_POINT ( 'NONE',  ( 16.59365244519689497, -183.6283474603465606, -105.5544085257710805 ) ) ;
#29403=EDGE_LOOP ( 'NONE', ( #7773, #2616, #20408, #36474 ) ) ;
#29405=ORIENTED_EDGE ( 'NONE', *, *, #15090, .F. ) ;
#29406=DIRECTION ( 'NONE',  ( 0.000000000000000000, 1.000000000000000000, -0.000000000000000000 ) ) ;
#29407=VECTOR ( 'NONE', #33035, 1000.000000000000000 ) ;
#29408=LINE ( 'NONE', #16571, #27019 ) ;
#29409=CARTESIAN_POINT ( 'NONE',  ( 53.62339707355158680, -193.5000000000000000, -70.36529243996335481 ) ) ;
#29411=ORIENTED_EDGE ( 'NONE', *, *, #4561, .T. ) ;
#29412=DIRECTION ( 'NONE',  ( 0.000000000000000000, 0.000000000000000000, -1.000000000000000000 ) ) ;
#29413=DIRECTION ( 'NONE',  ( 0.000000000000000000, 0.000000000000000000, -1.000000000000000000 ) ) ;
#29414=ORIENTED_EDGE ( 'NONE', *, *, #7183, .T. ) ;
#29415=CARTESIAN_POINT ( 'NONE',  ( 74.95461934957532435, -193.5000000000000000, -11.83705339977242410 ) ) ;
#29416=ORIENTED_EDGE ( 'NONE', *, *, #36282, .F. ) ;
#29417=CARTESIAN_POINT ( 'NONE',  ( -173.2765435274470178, -177.1207230881787780, -7.113702696401505321 ) ) ;
#29418=ORIENTED_EDGE ( 'NONE', *, *, #16293, .T. ) ;
#29420=VECTOR ( 'NONE', #24292, 1000.000000000000114 ) ;
#29421=ORIENTED_EDGE ( 'NONE', *, *, #11456, .F. ) ;
#29422=AXIS2_PLACEMENT_3D ( 'NONE', #27091, #31827, #15037 ) ;
#29423=AXIS2_PLACEMENT_3D ( 'NONE', #501, #48623, #777 ) ;
#29424=CARTESIAN_POINT ( 'NONE',  ( -172.4295958414655274, -193.5000000000000000, 3.504489105735796528 ) ) ;
#29425=CARTESIAN_POINT ( 'NONE',  ( -152.3176060415594861, -177.1207230881787780, -69.58857822034968876 ) ) ;
#29426=ORIENTED_EDGE ( 'NONE', *, *, #21349, .F. ) ;
#29427=CARTESIAN_POINT ( 'NONE',  ( -48.47912675150885065, -183.6283474603465606, 6.938893903907228378E-15 ) ) ;
#29429=ORIENTED_EDGE ( 'NONE', *, *, #45972, .T. ) ;
#29432=PLANE ( 'NONE',  #43183 ) ;
#29435=ADVANCED_FACE ( 'NONE', ( #45898 ), #45381, .T. ) ;
#29436=ADVANCED_FACE ( 'NONE', ( #13311 ), #9114, .T. ) ;
#29437=CYLINDRICAL_SURFACE ( 'NONE', #27524, 125.0000000000000000 ) ;
#29438=LINE ( 'NONE', #41012, #9005 ) ;
#29443=CARTESIAN_POINT ( 'NONE',  ( -48.47912675150885065, -173.5000000000000284, 6.938893903907228378E-15 ) ) ;
#29444=CARTESIAN_POINT ( 'NONE',  ( -165.2002711502080672, -183.6283474603465606, 44.73448837594998651 ) ) ;
#29446=ORIENTED_EDGE ( 'NONE', *, *, #51338, .F. ) ;
#29447=FACE_OUTER_BOUND ( 'NONE', #34126, .T. ) ;
#29448=EDGE_CURVE ( 'NONE', #2870, #45202, #33068, .T. ) ;
#29450=DIRECTION ( 'NONE',  ( -0.000000000000000000, 1.000000000000000000, -0.000000000000000000 ) ) ;
#29451=ORIENTED_EDGE ( 'NONE', *, *, #35030, .T. ) ;
#29452=EDGE_CURVE ( 'NONE', #12962, #32782, #4917, .T. ) ;
#29454=CARTESIAN_POINT ( 'NONE',  ( 56.28386853063362594, -189.7472609257535510, 66.33788548805517848 ) ) ;
#29455=EDGE_CURVE ( 'NONE', #37972, #23163, #1174, .T. ) ;
#29456=LINE ( 'NONE', #45509, #51472 ) ;
#29457=EDGE_LOOP ( 'NONE', ( #19005, #50419, #14301, #17961 ) ) ;
#29458=ADVANCED_FACE ( 'NONE', ( #45640 ), #41936, .T. ) ;
#29459=LINE ( 'NONE', #49711, #18924 ) ;
#29460=PLANE ( 'NONE',  #5958 ) ;
#29461=AXIS2_PLACEMENT_3D ( 'NONE', #40762, #4786, #36841 ) ;
#29464=FACE_OUTER_BOUND ( 'NONE', #37503, .T. ) ;
#29465=VECTOR ( 'NONE', #34886, 1000.000000000000000 ) ;
#29466=CARTESIAN_POINT ( 'NONE',  ( -3.104056038602969636, -183.6283474603465606, -115.4006183233321536 ) ) ;
#29469=CARTESIAN_POINT ( 'NONE',  ( -60.86541030502398542, -193.5000000000000000, -124.3848060646151623 ) ) ;
#29471=EDGE_LOOP ( 'NONE', ( #50484, #39248, #2090, #4898 ) ) ;
#29472=CARTESIAN_POINT ( 'NONE',  ( -93.85419746441394295, -177.1207230881787780, 115.4006183233324805 ) ) ;
#29474=FACE_OUTER_BOUND ( 'NONE', #5699, .T. ) ;
#29475=DIRECTION ( 'NONE',  ( -0.000000000000000000, 1.000000000000000000, -0.000000000000000000 ) ) ;
#29476=VERTEX_POINT ( 'NONE', #34055 ) ;
#29477=VERTEX_POINT ( 'NONE', #49055 ) ;
#29478=VECTOR ( 'NONE', #41846, 1000.000000000000000 ) ;
#29480=CARTESIAN_POINT ( 'NONE',  ( -160.2705093830644216, -177.1207230881787780, -55.92572546981520532 ) ) ;
#29482=FACE_OUTER_BOUND ( 'NONE', #44547, .T. ) ;
#29483=ORIENTED_EDGE ( 'NONE', *, *, #21324, .F. ) ;
#29484=ADVANCED_FACE ( 'NONE', ( #5950 ), #33790, .T. ) ;
#29486=DIRECTION ( 'NONE',  ( 0.3482016354344059095, 0.000000000000000000, -0.9374196611341183427 ) ) ;
#29487=ORIENTED_EDGE ( 'NONE', *, *, #50302, .F. ) ;
#29488=CARTESIAN_POINT ( 'NONE',  ( 141.7825277784304205, -193.5000000000000000, -41.45482488023466061 ) ) ;
#29489=ORIENTED_EDGE ( 'NONE', *, *, #49650, .F. ) ;
#29492=ORIENTED_EDGE ( 'NONE', *, *, #50142, .T. ) ;
#29493=EDGE_CURVE ( 'NONE', #34044, #1914, #1991, .T. ) ;
#29494=EDGE_CURVE ( 'NONE', #4854, #19952, #14618, .T. ) ;
#29496=EDGE_CURVE ( 'NONE', #1914, #6500, #25912, .T. ) ;
#29497=CARTESIAN_POINT ( 'NONE',  ( -164.2512865680372727, -175.3837268820161057, -47.13604789772046644 ) ) ;
#29498=CARTESIAN_POINT ( 'NONE',  ( -158.0280232639029236, -175.3837268820161057, 60.19999396110247147 ) ) ;
#29499=CIRCLE ( 'NONE', #16952, 125.0000000000000000 ) ;
#29501=ADVANCED_FACE ( 'NONE', ( #12770 ), #1736, .T. ) ;
#29502=VECTOR ( 'NONE', #15584, 1000.000000000000000 ) ;
#29503=ORIENTED_EDGE ( 'NONE', *, *, #25662, .F. ) ;
#29504=ORIENTED_EDGE ( 'NONE', *, *, #7964, .F. ) ;
#29506=PLANE ( 'NONE',  #18292 ) ;
#29507=ORIENTED_EDGE ( 'NONE', *, *, #16216, .F. ) ;
#29508=ADVANCED_FACE ( 'NONE', ( #18032 ), #18544, .T. ) ;
#29510=VERTEX_POINT ( 'NONE', #34558 ) ;
#29511=CARTESIAN_POINT ( 'NONE',  ( -48.77118352214581876, -193.5000000000000000, -0.9564009842765195391 ) ) ;
#29513=VECTOR ( 'NONE', #11637, 1000.000000000000000 ) ;
#29515=ADVANCED_FACE ( 'NONE', ( #51147 ), #14097, .T. ) ;
#29516=CARTESIAN_POINT ( 'NONE',  ( -171.2399149993172500, -175.3837268820161057, -17.48697739784461547 ) ) ;
#29517=VERTEX_POINT ( 'NONE', #10139 ) ;
#29518=AXIS2_PLACEMENT_3D ( 'NONE', #985, #16784, #29360 ) ;
#29520=EDGE_CURVE ( 'NONE', #48301, #34819, #32237, .T. ) ;
#29522=ORIENTED_EDGE ( 'NONE', *, *, #38198, .F. ) ;
#29525=CARTESIAN_POINT ( 'NONE',  ( 59.29945538372744096, -177.1207230881787780, 63.31490529818492519 ) ) ;
#29526=DIRECTION ( 'NONE',  ( -0.000000000000000000, 1.000000000000000000, -0.000000000000000000 ) ) ;
#29528=EDGE_CURVE ( 'NONE', #51044, #11425, #46665, .T. ) ;
#29529=ORIENTED_EDGE ( 'NONE', *, *, #30769, .T. ) ;
#29530=LINE ( 'NONE', #44794, #44620 ) ;
#29532=ORIENTED_EDGE ( 'NONE', *, *, #35206, .T. ) ;
#29533=DIRECTION ( 'NONE',  ( -0.000000000000000000, 1.000000000000000000, -0.000000000000000000 ) ) ;
#29534=CARTESIAN_POINT ( 'NONE',  ( -171.4462109067799247, -183.6283474603465606, 15.97798378892250426 ) ) ;
#29536=CIRCLE ( 'NONE', #42138, 125.0000000000000000 ) ;
#29539=CIRCLE ( 'NONE', #11895, 125.0000000000000000 ) ;
#29540=EDGE_CURVE ( 'NONE', #29932, #39444, #46160, .T. ) ;
#29543=LINE ( 'NONE', #25105, #40515 ) ;
#29545=CARTESIAN_POINT ( 'NONE',  ( -166.9492939735806090, -175.3837268820161057, 39.87254040532603483 ) ) ;
#29546=ORIENTED_EDGE ( 'NONE', *, *, #14633, .T. ) ;
#29548=CARTESIAN_POINT ( 'NONE',  ( -48.98765787015805984, -177.1207230881787780, -0.8610436117673551104 ) ) ;
#29549=FACE_OUTER_BOUND ( 'NONE', #43880, .T. ) ;
#29550=CARTESIAN_POINT ( 'NONE',  ( -131.1972941934623975, -183.6283474603465606, 92.37913469314123915 ) ) ;
#29551=ORIENTED_EDGE ( 'NONE', *, *, #50593, .F. ) ;
#29553=ORIENTED_EDGE ( 'NONE', *, *, #19546, .T. ) ;
#29556=FACE_OUTER_BOUND ( 'NONE', #19169, .T. ) ;
#29558=VECTOR ( 'NONE', #33247, 1000.000000000000000 ) ;
#29559=DIRECTION ( 'NONE',  ( 0.000000000000000000, 1.000000000000000000, 0.000000000000000000 ) ) ;
#29560=FACE_OUTER_BOUND ( 'NONE', #49567, .T. ) ;
#29561=ORIENTED_EDGE ( 'NONE', *, *, #20816, .F. ) ;
#29564=EDGE_CURVE ( 'NONE', #20792, #33649, #50356, .T. ) ;
#29566=ORIENTED_EDGE ( 'NONE', *, *, #48504, .T. ) ;
#29568=EDGE_LOOP ( 'NONE', ( #14386, #3493, #49351, #29207 ) ) ;
#29569=ORIENTED_EDGE ( 'NONE', *, *, #4343, .T. ) ;
#29572=CIRCLE ( 'NONE', #12797, 125.0000000000000000 ) ;
#29573=DIRECTION ( 'NONE',  ( -0.000000000000000000, 1.000000000000000000, -0.000000000000000000 ) ) ;
#29574=DIRECTION ( 'NONE',  ( 0.4566292373937140270, 0.000000000000000000, -0.8896570909947467687 ) ) ;
#29575=ORIENTED_EDGE ( 'NONE', *, *, #45149, .T. ) ;
#29576=CARTESIAN_POINT ( 'NONE',  ( -16.10442403432824321, -177.1207230881787780, -119.6996507684850428 ) ) ;
#29582=LINE ( 'NONE', #33540, #6856 ) ;
#29583=ORIENTED_EDGE ( 'NONE', *, *, #48758, .F. ) ;
#29584=DIRECTION ( 'NONE',  ( 0.000000000000000000, 1.000000000000000000, -0.000000000000000000 ) ) ;
#29586=CARTESIAN_POINT ( 'NONE',  ( -123.4791267515088435, -198.5000000000000000, 70.00000000000000000 ) ) ;
#29588=AXIS2_PLACEMENT_3D ( 'NONE', #48889, #28885, #9202 ) ;
#29589=AXIS2_PLACEMENT_3D ( 'NONE', #24020, #98, #26540 ) ;
#29590=EDGE_CURVE ( 'NONE', #13015, #45883, #40625, .T. ) ;
#29591=LINE ( 'NONE', #41681, #14393 ) ;
#29592=FACE_BOUND ( 'NONE', #48148, .T. ) ;
#29593=ORIENTED_EDGE ( 'NONE', *, *, #7672, .F. ) ;
#29594=AXIS2_PLACEMENT_3D ( 'NONE', #5951, #49582, #49839 ) ;
#29595=AXIS2_PLACEMENT_3D ( 'NONE', #17727, #34506, #29782 ) ;
#29596=DIRECTION ( 'NONE',  ( 0.4031234292879730674, 0.000000000000000000, -0.9151456172430181280 ) ) ;
#29598=ORIENTED_EDGE ( 'NONE', *, *, #24700, .T. ) ;
#29599=CARTESIAN_POINT ( 'NONE',  ( -170.0502155641509034, -183.6283474603465606, -29.07697310430886262 ) ) ;
#29600=CIRCLE ( 'NONE', #33805, 125.0000000000000000 ) ;
#29601=ORIENTED_EDGE ( 'NONE', *, *, #5069, .T. ) ;
#29603=DIRECTION ( 'NONE',  ( 0.000000000000000000, 0.000000000000000000, -1.000000000000000000 ) ) ;
#29604=CARTESIAN_POINT ( 'NONE',  ( -47.49008656418669005, -175.3837268820161057, 0.1476465640024920423 ) ) ;
#29606=CIRCLE ( 'NONE', #14508, 125.0000000000000000 ) ;
#29607=PLANE ( 'NONE',  #43669 ) ;
#29609=ORIENTED_EDGE ( 'NONE', *, *, #14789, .T. ) ;
#29610=CIRCLE ( 'NONE', #48947, 125.0000000000000000 ) ;
#29612=LINE ( 'NONE', #9144, #46893 ) ;
#29613=LINE ( 'NONE', #44877, #41929 ) ;
#29614=ORIENTED_EDGE ( 'NONE', *, *, #45888, .T. ) ;
#29617=FACE_OUTER_BOUND ( 'NONE', #41466, .T. ) ;
#29618=ORIENTED_EDGE ( 'NONE', *, *, #20245, .F. ) ;
#29619=EDGE_CURVE ( 'NONE', #31952, #21665, #8751, .T. ) ;
#29620=AXIS2_PLACEMENT_3D ( 'NONE', #48673, #4780, #50 ) ;
#29623=CARTESIAN_POINT ( 'NONE',  ( -48.24424070572787571, -175.3837268820161057, 0.9720229140804191870 ) ) ;
#29624=ORIENTED_EDGE ( 'NONE', *, *, #8636, .T. ) ;
#29625=DIRECTION ( 'NONE',  ( -0.2348860457809842095, 0.000000000000000000, 0.9720229140804107493 ) ) ;
#29627=AXIS2_PLACEMENT_3D ( 'NONE', #48418, #8458, #32368 ) ;
#29628=ORIENTED_EDGE ( 'NONE', *, *, #43704, .F. ) ;
#29629=ORIENTED_EDGE ( 'NONE', *, *, #29692, .F. ) ;
#29631=FACE_OUTER_BOUND ( 'NONE', #37648, .T. ) ;
#29634=AXIS2_PLACEMENT_3D ( 'NONE', #20420, #36440, #3615 ) ;
#29635=CARTESIAN_POINT ( 'NONE',  ( -48.47912675150885065, -177.1207230881787780, 6.938893903907228378E-15 ) ) ;
#29636=ORIENTED_EDGE ( 'NONE', *, *, #10840, .T. ) ;
#29637=FACE_OUTER_BOUND ( 'NONE', #43119, .T. ) ;
#29638=ORIENTED_EDGE ( 'NONE', *, *, #49998, .F. ) ;
#29639=EDGE_LOOP ( 'NONE', ( #46962, #27067, #47431, #15828 ) ) ;
#29640=CARTESIAN_POINT ( 'NONE',  ( -47.55243714407702527, -193.5000000000000000, 0.3758275821142491591 ) ) ;
#29641=DIRECTION ( 'NONE',  ( -0.8610436117673548884, 0.000000000000000000, -0.5085311186492216251 ) ) ;
#29642=ADVANCED_FACE ( 'NONE', ( #2764 ), #30891, .T. ) ;
#29644=PLANE ( 'NONE',  #48381 ) ;
#29645=ORIENTED_EDGE ( 'NONE', *, *, #20210, .T. ) ;
#29646=DIRECTION ( 'NONE',  ( 0.000000000000000000, -0.000000000000000000, -1.000000000000000000 ) ) ;
#29650=DIRECTION ( 'NONE',  ( -0.000000000000000000, 1.000000000000000000, -0.000000000000000000 ) ) ;
#29652=ORIENTED_EDGE ( 'NONE', *, *, #12124, .T. ) ;
#29653=CARTESIAN_POINT ( 'NONE',  ( -165.5546359831674295, -177.1207230881787780, 43.79868877201493405 ) ) ;
#29654=CARTESIAN_POINT ( 'NONE',  ( 36.84288420123322538, -183.6283474603465606, 91.35181687837501840 ) ) ;
#29655=VECTOR ( 'NONE', #28947, 1000.000000000000114 ) ;
#29656=CARTESIAN_POINT ( 'NONE',  ( -82.67254833784559764, -177.1207230881787780, -120.2323164553484105 ) ) ;
#29657=ORIENTED_EDGE ( 'NONE', *, *, #30977, .F. ) ;
#29658=ADVANCED_FACE ( 'NONE', ( #19067 ), #26154, .T. ) ;
#29659=PLANE ( 'NONE',  #39512 ) ;
#29660=DIRECTION ( 'NONE',  ( -0.000000000000000000, 1.000000000000000000, -0.000000000000000000 ) ) ;
#29661=ORIENTED_EDGE ( 'NONE', *, *, #34328, .F. ) ;
#29663=EDGE_CURVE ( 'NONE', #4180, #1918, #34780, .T. ) ;
#29664=VECTOR ( 'NONE', #9095, 1000.000000000000000 ) ;
#29665=ORIENTED_EDGE ( 'NONE', *, *, #23098, .F. ) ;
#29666=DIRECTION ( 'NONE',  ( 0.000000000000000000, -0.000000000000000000, -1.000000000000000000 ) ) ;
#29667=CIRCLE ( 'NONE', #11091, 125.0000000000000568 ) ;
#29669=CARTESIAN_POINT ( 'NONE',  ( -49.30901192927175458, -193.5000000000000000, -124.9972451320097093 ) ) ;
#29670=DIRECTION ( 'NONE',  ( 0.000000000000000000, -1.000000000000000000, 0.000000000000000000 ) ) ;
#29671=DIRECTION ( 'NONE',  ( 0.000000000000000000, 1.000000000000000000, 0.000000000000000000 ) ) ;
#29675=LINE ( 'NONE', #17099, #8015 ) ;
#29680=DIRECTION ( 'NONE',  ( -0.000000000000000000, 1.000000000000000000, 0.000000000000000000 ) ) ;
#29682=ORIENTED_EDGE ( 'NONE', *, *, #17286, .F. ) ;
#29683=ADVANCED_FACE ( 'NONE', ( #51918 ), #15907, .T. ) ;
#29684=ADVANCED_FACE ( 'NONE', ( #15382 ), #27710, .F. ) ;
#29690=DIRECTION ( 'NONE',  ( -0.6068001458185834363, 0.000000000000000000, -0.7948544414133608127 ) ) ;
#29691=VERTEX_POINT ( 'NONE', #35860 ) ;
#29692=EDGE_CURVE ( 'NONE', #47995, #51589, #7746, .T. ) ;
#29695=DIRECTION ( 'NONE',  ( -0.7175072570443395970, 0.000000000000000000, 0.6965510290629882695 ) ) ;
#29696=ORIENTED_EDGE ( 'NONE', *, *, #27781, .F. ) ;
#29700=ORIENTED_EDGE ( 'NONE', *, *, #36202, .T. ) ;
#29701=AXIS2_PLACEMENT_3D ( 'NONE', #9657, #5732, #33823 ) ;
#29702=ORIENTED_EDGE ( 'NONE', *, *, #9516, .F. ) ;
#29703=DIRECTION ( 'NONE',  ( 0.9473263538541899509, 0.000000000000000000, 0.3202698538628415692 ) ) ;
#29704=FACE_OUTER_BOUND ( 'NONE', #34998, .T. ) ;
#29705=PLANE ( 'NONE',  #11402 ) ;
#29707=ADVANCED_FACE ( 'NONE', ( #23776 ), #44525, .F. ) ;
#29708=CARTESIAN_POINT ( 'NONE',  ( -47.92047998570519951, -193.5000000000000000, -0.8294056854501942189 ) ) ;
#29710=DIRECTION ( 'NONE',  ( 0.000000000000000000, -1.000000000000000000, 0.000000000000000000 ) ) ;
#29711=FACE_OUTER_BOUND ( 'NONE', #12575, .T. ) ;
#29712=ORIENTED_EDGE ( 'NONE', *, *, #17844, .F. ) ;
#29714=PLANE ( 'NONE',  #23931 ) ;
#29719=AXIS2_PLACEMENT_3D ( 'NONE', #47682, #24271, #43720 ) ;
#29721=DIRECTION ( 'NONE',  ( 0.000000000000000000, 0.000000000000000000, 1.000000000000000000 ) ) ;
#29723=VECTOR ( 'NONE', #50871, 1000.000000000000114 ) ;
#29725=CARTESIAN_POINT ( 'NONE',  ( -48.47912675150885065, -189.7472609257535510, 6.938893903907228378E-15 ) ) ;
#29726=CYLINDRICAL_SURFACE ( 'NONE', #46366, 125.0000000000000000 ) ;
#29728=ORIENTED_EDGE ( 'NONE', *, *, #8682, .F. ) ;
#29729=ORIENTED_EDGE ( 'NONE', *, *, #27507, .T. ) ;
#29731=ADVANCED_FACE ( 'NONE', ( #51639 ), #7498, .T. ) ;
#29732=LINE ( 'NONE', #49484, #17411 ) ;
#29733=AXIS2_PLACEMENT_3D ( 'NONE', #16976, #1179, #5407 ) ;
#29734=CARTESIAN_POINT ( 'NONE',  ( -172.9701362814535912, -193.5000000000000000, -11.26891947860193177 ) ) ;
#29735=LINE ( 'NONE', #37888, #31237 ) ;
#29736=ORIENTED_EDGE ( 'NONE', *, *, #35634, .F. ) ;
#29740=EDGE_CURVE ( 'NONE', #48318, #42355, #7115, .T. ) ;
#29742=DIRECTION ( 'NONE',  ( -0.000000000000000000, -1.000000000000000000, 0.000000000000000000 ) ) ;
#29743=VERTEX_POINT ( 'NONE', #19826 ) ;
#29744=EDGE_CURVE ( 'NONE', #43853, #14242, #23519, .T. ) ;
#29745=CARTESIAN_POINT ( 'NONE',  ( -48.47912675150885065, -183.6283474603465606, 6.938893903907228378E-15 ) ) ;
#29746=CARTESIAN_POINT ( 'NONE',  ( -8.721998590732194856, -193.5000000000000000, -118.5089480183145270 ) ) ;
#29747=EDGE_LOOP ( 'NONE', ( #37777, #37254, #41482, #29813 ) ) ;
#29749=LINE ( 'NONE', #25822, #13842 ) ;
#29750=AXIS2_PLACEMENT_3D ( 'NONE', #44969, #29695, #20783 ) ;
#29755=VECTOR ( 'NONE', #19687, 1000.000000000000114 ) ;
#29756=DIRECTION ( 'NONE',  ( 0.000000000000000000, -0.000000000000000000, -1.000000000000000000 ) ) ;
#29757=FACE_OUTER_BOUND ( 'NONE', #35235, .T. ) ;
#29759=VECTOR ( 'NONE', #1682, 1000.000000000000000 ) ;
#29761=ORIENTED_EDGE ( 'NONE', *, *, #2236, .F. ) ;
#29762=DIRECTION ( 'NONE',  ( 0.000000000000000000, 0.000000000000000000, -1.000000000000000000 ) ) ;
#29763=LINE ( 'NONE', #21109, #17511 ) ;
#29765=DIRECTION ( 'NONE',  ( 0.6068001458185834363, 0.000000000000000000, 0.7948544414133608127 ) ) ;
#29766=ORIENTED_EDGE ( 'NONE', *, *, #13849, .T. ) ;
#29769=LINE ( 'NONE', #37924, #8816 ) ;
#29770=ORIENTED_EDGE ( 'NONE', *, *, #4152, .F. ) ;
#29771=CARTESIAN_POINT ( 'NONE',  ( 76.37123734610607073, -177.1207230881787780, 6.114457023561872262 ) ) ;
#29773=DIRECTION ( 'NONE',  ( -0.8610436117673621048, 0.000000000000000000, 0.5085311186492095237 ) ) ;
#29776=VERTEX_POINT ( 'NONE', #40562 ) ;
#29777=LINE ( 'NONE', #21913, #41622 ) ;
#29781=EDGE_LOOP ( 'NONE', ( #48951, #51237, #38227, #31176 ) ) ;
#29782=DIRECTION ( 'NONE',  ( 0.000000000000000000, 0.000000000000000000, -1.000000000000000000 ) ) ;
#29783=EDGE_CURVE ( 'NONE', #13545, #44193, #28736, .T. ) ;
#29784=VERTEX_POINT ( 'NONE', #49780 ) ;
#29785=VECTOR ( 'NONE', #9426, 1000.000000000000000 ) ;
#29789=AXIS2_PLACEMENT_3D ( 'NONE', #51131, #39272, #15622 ) ;
#29792=ORIENTED_EDGE ( 'NONE', *, *, #51071, .T. ) ;
#29794=ADVANCED_FACE ( 'NONE', ( #5641 ), #12708, .F. ) ;
#29795=VECTOR ( 'NONE', #31592, 1000.000000000000000 ) ;
#29798=EDGE_LOOP ( 'NONE', ( #4442, #45729, #51952, #11168 ) ) ;
#29799=CARTESIAN_POINT ( 'NONE',  ( -85.48706473349325563, -193.5000000000000000, -118.3487137068146637 ) ) ;
#29802=VERTEX_POINT ( 'NONE', #4858 ) ;
#29803=CARTESIAN_POINT ( 'NONE',  ( 36.10886851198521441, -177.1207230881787780, 92.03190238880813467 ) ) ;
#29804=CARTESIAN_POINT ( 'NONE',  ( -98.10897907742936752, -175.3837268820161057, 114.7252272087849292 ) ) ;
#29806=ADVANCED_FACE ( 'NONE', ( #28996 ), #36904, .T. ) ;
#29807=DIRECTION ( 'NONE',  ( -0.000000000000000000, 1.000000000000000000, -0.000000000000000000 ) ) ;
#29808=CIRCLE ( 'NONE', #20582, 125.0000000000000000 ) ;
#29809=FACE_OUTER_BOUND ( 'NONE', #45997, .T. ) ;
#29810=VERTEX_POINT ( 'NONE', #17722 ) ;
#29811=ORIENTED_EDGE ( 'NONE', *, *, #7024, .T. ) ;
#29812=ADVANCED_FACE ( 'NONE', ( #21386 ), #16692, .T. ) ;
#29813=ORIENTED_EDGE ( 'NONE', *, *, #39177, .T. ) ;
#29814=VECTOR ( 'NONE', #7584, 1000.000000000000114 ) ;
#29815=LINE ( 'NONE', #49557, #31635 ) ;
#29816=CARTESIAN_POINT ( 'NONE',  ( -47.50057025920934706, -183.6283474603465606, 0.2059786187411091207 ) ) ;
#29818=DIRECTION ( 'NONE',  ( 0.5085311186492216251, 0.000000000000000000, -0.8610436117673548884 ) ) ;
#29819=DIRECTION ( 'NONE',  ( 0.000000000000000000, 0.000000000000000000, -1.000000000000000000 ) ) ;
#29820=ORIENTED_EDGE ( 'NONE', *, *, #19102, .F. ) ;
#29823=VERTEX_POINT ( 'NONE', #9053 ) ;
#29825=EDGE_LOOP ( 'NONE', ( #3715, #43962, #43294, #40132 ) ) ;
#29830=AXIS2_PLACEMENT_3D ( 'NONE', #24795, #4564, #27695 ) ;
#29831=VECTOR ( 'NONE', #27654, 1000.000000000000114 ) ;
#29832=LINE ( 'NONE', #25629, #30413 ) ;
#29835=CARTESIAN_POINT ( 'NONE',  ( 58.12687231399077348, -183.6283474603465606, -63.33473559879917758 ) ) ;
#29837=EDGE_CURVE ( 'NONE', #10187, #44532, #35607, .T. ) ;
#29839=DIRECTION ( 'NONE',  ( 0.000000000000000000, 0.000000000000000000, 1.000000000000000000 ) ) ;
#29840=AXIS2_PLACEMENT_3D ( 'NONE', #32482, #20648, #48530 ) ;
#29841=DIRECTION ( 'NONE',  ( 0.3202698538628279690, 0.000000000000000000, 0.9473263538541946138 ) ) ;
#29842=VERTEX_POINT ( 'NONE', #1419 ) ;
#29844=DIRECTION ( 'NONE',  ( 0.000000000000000000, -1.000000000000000000, 0.000000000000000000 ) ) ;
#29845=CARTESIAN_POINT ( 'NONE',  ( -162.9896759831413249, -177.1207230881787780, -50.12318939043961308 ) ) ;
#29846=CARTESIAN_POINT ( 'NONE',  ( -47.92047998570519951, -183.6283474603465606, -0.8294056854501942189 ) ) ;
#29847=AXIS2_PLACEMENT_3D ( 'NONE', #48593, #20448, #8111 ) ;
#29848=CARTESIAN_POINT ( 'NONE',  ( 75.60865171534661044, -177.1207230881787780, -15.07392567185468302 ) ) ;
#29849=DIRECTION ( 'NONE',  ( -0.9646355819083614058, 0.000000000000000000, 0.2635871660690581320 ) ) ;
#29850=CIRCLE ( 'NONE', #12212, 125.0000000000000000 ) ;
#29852=EDGE_CURVE ( 'NONE', #2274, #43146, #2042, .T. ) ;
#29853=VERTEX_POINT ( 'NONE', #29525 ) ;
#29854=DIRECTION ( 'NONE',  ( -0.000000000000000000, 1.000000000000000000, -0.000000000000000000 ) ) ;
#29855=ORIENTED_EDGE ( 'NONE', *, *, #38040, .F. ) ;
#29856=EDGE_CURVE ( 'NONE', #38723, #30858, #33212, .T. ) ;
#29858=EDGE_CURVE ( 'NONE', #14785, #48301, #29273, .T. ) ;
#29860=EDGE_LOOP ( 'NONE', ( #33508, #47318, #5173, #30185 ) ) ;
#29861=EDGE_CURVE ( 'NONE', #14965, #22157, #41609, .T. ) ;
#29863=CARTESIAN_POINT ( 'NONE',  ( -162.3451783319732442, -177.1207230881787780, 51.57055649762783389 ) ) ;
#29864=CIRCLE ( 'NONE', #45822, 10.00000000000000000 ) ;
#29865=CARTESIAN_POINT ( 'NONE',  ( -49.32472275501068282, -177.1207230881787780, 0.5338233779647895139 ) ) ;
#29867=ORIENTED_EDGE ( 'NONE', *, *, #34902, .T. ) ;
#29869=CIRCLE ( 'NONE', #35751, 125.0000000000000000 ) ;
#29870=LINE ( 'NONE', #25929, #22704 ) ;
#29873=EDGE_LOOP ( 'NONE', ( #9967, #37642, #7363, #12232 ) ) ;
#29874=EDGE_LOOP ( 'NONE', ( #32897, #13932, #31104, #9126 ) ) ;
#29875=DIRECTION ( 'NONE',  ( 0.000000000000000000, -1.000000000000000000, -0.000000000000000000 ) ) ;
#29877=EDGE_CURVE ( 'NONE', #20319, #46485, #37306, .T. ) ;
#29878=AXIS2_PLACEMENT_3D ( 'NONE', #48661, #36822, #4241 ) ;
#29879=DIRECTION ( 'NONE',  ( 0.000000000000000000, 1.000000000000000000, -0.000000000000000000 ) ) ;
#29880=AXIS2_PLACEMENT_3D ( 'NONE', #41348, #13507, #45576 ) ;
#29881=DIRECTION ( 'NONE',  ( 0.000000000000000000, 0.000000000000000000, -1.000000000000000000 ) ) ;
#29883=ORIENTED_EDGE ( 'NONE', *, *, #9468, .T. ) ;
#29885=ADVANCED_FACE ( 'NONE', ( #42656 ), #22946, .T. ) ;
#29887=FACE_OUTER_BOUND ( 'NONE', #7774, .T. ) ;
#29888=VERTEX_POINT ( 'NONE', #10085 ) ;
#29889=DIRECTION ( 'NONE',  ( 0.000000000000000000, 0.000000000000000000, 1.000000000000000000 ) ) ;
#29890=ORIENTED_EDGE ( 'NONE', *, *, #13599, .F. ) ;
#29891=VERTEX_POINT ( 'NONE', #50299 ) ;
#29892=EDGE_LOOP ( 'NONE', ( #45077, #41066, #2865, #43893 ) ) ;
#29894=FACE_OUTER_BOUND ( 'NONE', #5902, .T. ) ;
#29895=ORIENTED_EDGE ( 'NONE', *, *, #40725, .F. ) ;
#29897=CARTESIAN_POINT ( 'NONE',  ( -115.4536696835168641, -193.5000000000000000, -105.5434062319793185 ) ) ;
#29898=ORIENTED_EDGE ( 'NONE', *, *, #17642, .T. ) ;
#29900=ORIENTED_EDGE ( 'NONE', *, *, #37281, .F. ) ;
#29902=CARTESIAN_POINT ( 'NONE',  ( 48.69345348225014192, -189.7472609257535510, -78.62880929222870918 ) ) ;
#29905=VECTOR ( 'NONE', #19377, 1000.000000000000114 ) ;
#29906=LINE ( 'NONE', #6781, #44846 ) ;
#29907=DIRECTION ( 'NONE',  ( 0.000000000000000000, -0.000000000000000000, -1.000000000000000000 ) ) ;
#29909=FACE_OUTER_BOUND ( 'NONE', #35593, .T. ) ;
#29911=AXIS2_PLACEMENT_3D ( 'NONE', #22353, #10786, #26546 ) ;
#29913=LINE ( 'NONE', #2051, #1972 ) ;
#29915=ORIENTED_EDGE ( 'NONE', *, *, #2173, .F. ) ;
#29916=DIRECTION ( 'NONE',  ( 0.000000000000000000, 0.000000000000000000, 1.000000000000000000 ) ) ;
#29917=CARTESIAN_POINT ( 'NONE',  ( -47.50057025920934706, -189.7472609257535510, 0.2059786187411091207 ) ) ;
#29922=CARTESIAN_POINT ( 'NONE',  ( -101.0675409952200283, -177.1207230881787780, 113.3995532942340958 ) ) ;
#29924=CIRCLE ( 'NONE', #9786, 125.0000000000000000 ) ;
#29925=FACE_OUTER_BOUND ( 'NONE', #23506, .T. ) ;
#29926=DIRECTION ( 'NONE',  ( 0.000000000000000000, 1.000000000000000000, 0.000000000000000000 ) ) ;
#29927=ORIENTED_EDGE ( 'NONE', *, *, #4927, .T. ) ;
#29928=EDGE_CURVE ( 'NONE', #46169, #38032, #5439, .T. ) ;
#29930=CARTESIAN_POINT ( 'NONE',  ( -63.43218022845228887, -175.3837268820161057, 124.1024020384604540 ) ) ;
#29931=VECTOR ( 'NONE', #16717, 1000.000000000000000 ) ;
#29932=VERTEX_POINT ( 'NONE', #2460 ) ;
#29933=CARTESIAN_POINT ( 'NONE',  ( -69.77312546433408613, -189.7472609257535510, 123.1729094355499967 ) ) ;
#29934=FACE_OUTER_BOUND ( 'NONE', #42099, .T. ) ;
#29935=CARTESIAN_POINT ( 'NONE',  ( -49.21696003055057389, -183.6283474603465606, -0.6749830015182127774 ) ) ;
#29937=DIRECTION ( 'NONE',  ( 0.000000000000000000, 1.000000000000000000, -0.000000000000000000 ) ) ;
#29938=ORIENTED_EDGE ( 'NONE', *, *, #29852, .F. ) ;
#29939=DIRECTION ( 'NONE',  ( -0.000000000000000000, 1.000000000000000000, -0.000000000000000000 ) ) ;
#29940=ORIENTED_EDGE ( 'NONE', *, *, #24208, .T. ) ;
#29941=FACE_OUTER_BOUND ( 'NONE', #13349, .T. ) ;
#29942=AXIS2_PLACEMENT_3D ( 'NONE', #20344, #8775, #28738 ) ;
#29944=EDGE_LOOP ( 'NONE', ( #43433, #20443, #12599, #1589 ) ) ;
#29945=EDGE_CURVE ( 'NONE', #1430, #13839, #51086, .T. ) ;
#29946=FACE_OUTER_BOUND ( 'NONE', #2377, .T. ) ;
#29947=AXIS2_PLACEMENT_3D ( 'NONE', #18754, #14829, #18249 ) ;
#29948=VERTEX_POINT ( 'NONE', #38183 ) ;
#29950=CARTESIAN_POINT ( 'NONE',  ( -34.51936650669028239, -175.3837268820161057, -124.2180546213278092 ) ) ;
#29953=LINE ( 'NONE', #2612, #7397 ) ;
#29954=LINE ( 'NONE', #17632, #44059 ) ;
#29956=VECTOR ( 'NONE', #33476, 1000.000000000000000 ) ;
#29957=AXIS2_PLACEMENT_3D ( 'NONE', #2632, #26802, #18671 ) ;
#29958=CIRCLE ( 'NONE', #9824, 125.0000000000000000 ) ;
#29961=ORIENTED_EDGE ( 'NONE', *, *, #39104, .T. ) ;
#29962=CARTESIAN_POINT ( 'NONE',  ( -23.99795575808071035, -183.6283474603465606, -122.5792489240757703 ) ) ;
#29965=CIRCLE ( 'NONE', #586, 125.0000000000000000 ) ;
#29967=DIRECTION ( 'NONE',  ( -0.000000000000000000, 1.000000000000000000, 0.000000000000000000 ) ) ;
#29968=DIRECTION ( 'NONE',  ( -0.000000000000000000, 0.000000000000000000, -1.000000000000000000 ) ) ;
#29971=CIRCLE ( 'NONE', #37504, 125.0000000000000000 ) ;
#29972=CARTESIAN_POINT ( 'NONE',  ( -86.93810158023210022, -177.1207230881787780, 117.8859915627477335 ) ) ;
#29976=EDGE_LOOP ( 'NONE', ( #1964, #42052, #25635, #21741 ) ) ;
#29979=LINE ( 'NONE', #9750, #36038 ) ;
#29980=CARTESIAN_POINT ( 'NONE',  ( -158.0280232639029236, -175.3837268820161057, 60.19999396110247147 ) ) ;
#29981=ORIENTED_EDGE ( 'NONE', *, *, #8851, .T. ) ;
#29984=FACE_OUTER_BOUND ( 'NONE', #51941, .T. ) ;
#29986=CARTESIAN_POINT ( 'NONE',  ( 47.04848625005566731, -193.5000000000000000, 80.61932246194658092 ) ) ;
#29988=AXIS2_PLACEMENT_3D ( 'NONE', #22263, #29183, #38290 ) ;
#29990=LINE ( 'NONE', #10030, #16419 ) ;
#29991=DIRECTION ( 'NONE',  ( 0.000000000000000000, 1.000000000000000000, 0.000000000000000000 ) ) ;
#29992=VECTOR ( 'NONE', #36795, 1000.000000000000227 ) ;
#29993=CARTESIAN_POINT ( 'NONE',  ( -96.65280530915691770, -183.6283474603465606, -115.3442529744087324 ) ) ;
#29995=EDGE_CURVE ( 'NONE', #35424, #15652, #48233, .T. ) ;
#29997=CARTESIAN_POINT ( 'NONE',  ( -151.5051191635538146, -177.1207230881787780, -69.00559874123518966 ) ) ;
#29998=CIRCLE ( 'NONE', #9858, 125.0000000000000000 ) ;
#30001=DIRECTION ( 'NONE',  ( 0.000000000000000000, 0.000000000000000000, 1.000000000000000000 ) ) ;
#30002=CARTESIAN_POINT ( 'NONE',  ( -159.0901268547125653, -193.5000000000000000, 58.22548115875957109 ) ) ;
#30003=DIRECTION ( 'NONE',  ( 0.9473263538541876194, 0.000000000000000000, 0.3202698538628486746 ) ) ;
#30007=AXIS2_PLACEMENT_3D ( 'NONE', #27812, #28069, #4185 ) ;
#30009=CARTESIAN_POINT ( 'NONE',  ( -154.0877180371535928, -175.3837268820161057, -66.87170886601927577 ) ) ;
#30013=ADVANCED_FACE ( 'NONE', ( #37936 ), #18485, .T. ) ;
#30014=CARTESIAN_POINT ( 'NONE',  ( -49.13194886969936448, -175.3837268820161057, -0.7575112421616214675 ) ) ;
#30015=DIRECTION ( 'NONE',  ( -0.9266896074318370369, 0.000000000000000000, 0.3758275821142292306 ) ) ;
#30016=DIRECTION ( 'NONE',  ( -0.000000000000000000, -1.000000000000000000, 0.000000000000000000 ) ) ;
#30017=ORIENTED_EDGE ( 'NONE', *, *, #22112, .T. ) ;
#30018=DIRECTION ( 'NONE',  ( 0.000000000000000000, 1.000000000000000000, 0.000000000000000000 ) ) ;
#30019=LINE ( 'NONE', #30791, #21869 ) ;
#30020=AXIS2_PLACEMENT_3D ( 'NONE', #9546, #5879, #36887 ) ;
#30022=ORIENTED_EDGE ( 'NONE', *, *, #14626, .T. ) ;
#30023=AXIS2_PLACEMENT_3D ( 'NONE', #22608, #25770, #21835 ) ;
#30024=DIRECTION ( 'NONE',  ( 0.000000000000000000, 1.000000000000000000, -0.000000000000000000 ) ) ;
#30027=VECTOR ( 'NONE', #9585, 1000.000000000000000 ) ;
#30032=ORIENTED_EDGE ( 'NONE', *, *, #24630, .F. ) ;
#30033=AXIS2_PLACEMENT_3D ( 'NONE', #12485, #8292, #51937 ) ;
#30034=ORIENTED_EDGE ( 'NONE', *, *, #14472, .T. ) ;
#30035=FACE_OUTER_BOUND ( 'NONE', #3893, .T. ) ;
#30038=CARTESIAN_POINT ( 'NONE',  ( -165.2002711502080672, -183.6283474603465606, 44.73448837594995098 ) ) ;
#30040=ORIENTED_EDGE ( 'NONE', *, *, #14390, .F. ) ;
#30042=DIRECTION ( 'NONE',  ( -0.6528221181905174975, 0.000000000000000000, -0.7575112421616236880 ) ) ;
#30043=AXIS2_PLACEMENT_3D ( 'NONE', #26780, #11001, #38862 ) ;
#30044=ORIENTED_EDGE ( 'NONE', *, *, #33425, .F. ) ;
#30045=CARTESIAN_POINT ( 'NONE',  ( 46.01898237923986557, -177.1207230881787780, -81.82363577055902226 ) ) ;
#30046=ORIENTED_EDGE ( 'NONE', *, *, #28354, .F. ) ;
#30047=CARTESIAN_POINT ( 'NONE',  ( -108.6269575285487576, -193.5000000000000000, -108.4360005853207127 ) ) ;
#30048=LINE ( 'NONE', #8834, #42402 ) ;
#30049=LINE ( 'NONE', #10591, #10973 ) ;
#30050=VERTEX_POINT ( 'NONE', #14034 ) ;
#30051=CARTESIAN_POINT ( 'NONE',  ( 72.31641062551800303, -189.7472609257535510, 32.14713283941989630 ) ) ;
#30052=LINE ( 'NONE', #15848, #33142 ) ;
#30054=EDGE_CURVE ( 'NONE', #34274, #31867, #30052, .T. ) ;
#30055=EDGE_CURVE ( 'NONE', #17649, #51370, #31333, .T. ) ;
#30057=DIRECTION ( 'NONE',  ( 0.000000000000000000, 0.000000000000000000, 1.000000000000000000 ) ) ;
#30058=VERTEX_POINT ( 'NONE', #23466 ) ;
#30059=VECTOR ( 'NONE', #22415, 1000.000000000000000 ) ;
#30061=ADVANCED_FACE ( 'NONE', ( #44205 ), #12396, .T. ) ;
#30063=DIRECTION ( 'NONE',  ( 0.000000000000000000, -0.000000000000000000, 1.000000000000000000 ) ) ;
#30064=LINE ( 'NONE', #42399, #15269 ) ;
#30065=VERTEX_POINT ( 'NONE', #27389 ) ;
#30066=AXIS2_PLACEMENT_3D ( 'NONE', #48901, #21290, #1311 ) ;
#30067=ORIENTED_EDGE ( 'NONE', *, *, #34317, .F. ) ;
#30068=LINE ( 'NONE', #10350, #11485 ) ;
#30070=VECTOR ( 'NONE', #42277, 1000.000000000000114 ) ;
#30072=DIRECTION ( 'NONE',  ( 0.000000000000000000, 0.000000000000000000, -1.000000000000000000 ) ) ;
#30073=EDGE_LOOP ( 'NONE', ( #24554, #10343, #43341, #20644 ) ) ;
#30075=CARTESIAN_POINT ( 'NONE',  ( 64.29733702426838704, -189.7472609257535510, 53.91167979418565182 ) ) ;
#30080=ORIENTED_EDGE ( 'NONE', *, *, #19214, .T. ) ;
#30081=LINE ( 'NONE', #26128, #6489 ) ;
#30082=DIRECTION ( 'NONE',  ( -0.9266896074318343723, 0.000000000000000000, 0.3758275821142357809 ) ) ;
#30083=CARTESIAN_POINT ( 'NONE',  ( -48.47912675150885065, -175.3837268820161057, 6.938893903907228378E-15 ) ) ;
#30084=CARTESIAN_POINT ( 'NONE',  ( -48.47912675150885065, -175.3837268820161057, 6.938893903907228378E-15 ) ) ;
#30087=DIRECTION ( 'NONE',  ( -0.2348860457809707758, 0.000000000000000000, -0.9720229140804138579 ) ) ;
#30088=ORIENTED_EDGE ( 'NONE', *, *, #49642, .F. ) ;
#30089=ORIENTED_EDGE ( 'NONE', *, *, #15406, .T. ) ;
#30090=AXIS2_PLACEMENT_3D ( 'NONE', #51903, #4062, #28468 ) ;
#30091=DIRECTION ( 'NONE',  ( 0.000000000000000000, 0.000000000000000000, -1.000000000000000000 ) ) ;
#30092=PLANE ( 'NONE',  #45120 ) ;
#30095=AXIS2_PLACEMENT_3D ( 'NONE', #20705, #9148, #45163 ) ;
#30096=EDGE_CURVE ( 'NONE', #39429, #40001, #23090, .T. ) ;
#30098=ADVANCED_FACE ( 'NONE', ( #27905 ), #47648, .T. ) ;
#30099=EDGE_CURVE ( 'NONE', #51271, #1772, #35793, .T. ) ;
#30102=LINE ( 'NONE', #46149, #20879 ) ;
#30103=ORIENTED_EDGE ( 'NONE', *, *, #7951, .F. ) ;
#30104=EDGE_CURVE ( 'NONE', #9410, #3078, #23711, .T. ) ;
#30105=ORIENTED_EDGE ( 'NONE', *, *, #48841, .F. ) ;
#30106=DIRECTION ( 'NONE',  ( 0.9982437317643217956, 0.000000000000000000, -0.05924062789370748011 ) ) ;
#30107=AXIS2_PLACEMENT_3D ( 'NONE', #10688, #22777, #38786 ) ;
#30108=EDGE_CURVE ( 'NONE', #41848, #20319, #43941, .T. ) ;
#30109=DIRECTION ( 'NONE',  ( 0.000000000000000000, 0.000000000000000000, -1.000000000000000000 ) ) ;
#30110=ORIENTED_EDGE ( 'NONE', *, *, #13550, .T. ) ;
#30111=EDGE_CURVE ( 'NONE', #18537, #17442, #36057, .T. ) ;
#30112=CARTESIAN_POINT ( 'NONE',  ( 15.80042947435468470, -175.3837268820161057, 107.2060569716377927 ) ) ;
#30114=CARTESIAN_POINT ( 'NONE',  ( -130.7087404384255080, -193.5000000000000000, -94.14505102712755047 ) ) ;
#30115=EDGE_CURVE ( 'NONE', #9866, #2431, #43164, .T. ) ;
#30118=VECTOR ( 'NONE', #49881, 1000.000000000000000 ) ;
#30119=CARTESIAN_POINT ( 'NONE',  ( 71.87891646118019651, -189.7472609257535510, -33.74820638215423685 ) ) ;
#30121=EDGE_CURVE ( 'NONE', #30483, #40790, #24237, .T. ) ;
#30122=DIRECTION ( 'NONE',  ( -0.000000000000000000, 1.000000000000000000, -0.000000000000000000 ) ) ;
#30125=ORIENTED_EDGE ( 'NONE', *, *, #906, .F. ) ;
#30126=FACE_OUTER_BOUND ( 'NONE', #923, .T. ) ;
#30127=ORIENTED_EDGE ( 'NONE', *, *, #11823, .T. ) ;
#30129=VECTOR ( 'NONE', #17607, 1000.000000000000227 ) ;
#30132=VERTEX_POINT ( 'NONE', #56 ) ;
#30133=DIRECTION ( 'NONE',  ( 0.000000000000000000, -0.000000000000000000, 1.000000000000000000 ) ) ;
#30135=FACE_OUTER_BOUND ( 'NONE', #46369, .T. ) ;
#30136=PLANE ( 'NONE',  #23183 ) ;
#30137=EDGE_CURVE ( 'NONE', #6231, #25260, #15522, .T. ) ;
#30138=ORIENTED_EDGE ( 'NONE', *, *, #36577, .T. ) ;
#30139=ORIENTED_EDGE ( 'NONE', *, *, #43704, .T. ) ;
#30141=DIRECTION ( 'NONE',  ( 0.000000000000000000, 1.000000000000000000, -0.000000000000000000 ) ) ;
#30142=VECTOR ( 'NONE', #46174, 1000.000000000000227 ) ;
#30144=CARTESIAN_POINT ( 'NONE',  ( 74.77174840718836890, -183.6283474603465606, 20.83798868929603643 ) ) ;
#30147=ORIENTED_EDGE ( 'NONE', *, *, #48637, .F. ) ;
#30149=CARTESIAN_POINT ( 'NONE',  ( 48.06131630543706734, -193.5000000000000000, -79.40367028273054473 ) ) ;
#30151=EDGE_LOOP ( 'NONE', ( #42440, #14410, #13848, #33230 ) ) ;
#30155=DIRECTION ( 'NONE',  ( 0.000000000000000000, -1.000000000000000000, 0.000000000000000000 ) ) ;
#30156=ORIENTED_EDGE ( 'NONE', *, *, #43929, .T. ) ;
#30157=DIRECTION ( 'NONE',  ( 0.9027978299657387629, 0.000000000000000000, 0.4300652022765304450 ) ) ;
#30159=EDGE_CURVE ( 'NONE', #28018, #34611, #3760, .T. ) ;
#30160=ADVANCED_FACE ( 'NONE', ( #3236 ), #19272, .T. ) ;
#30162=EDGE_CURVE ( 'NONE', #3300, #10662, #574, .T. ) ;
#30165=EDGE_LOOP ( 'NONE', ( #26124, #49723, #23756, #4563 ) ) ;
#30169=VERTEX_POINT ( 'NONE', #17845 ) ;
#30170=DIRECTION ( 'NONE',  ( 0.3482016354343995812, 0.000000000000000000, -0.9374196611341205632 ) ) ;
#30172=AXIS2_PLACEMENT_3D ( 'NONE', #13329, #34068, #45917 ) ;
#30174=ADVANCED_FACE ( 'NONE', ( #25983 ), #18370, .T. ) ;
#30175=CARTESIAN_POINT ( 'NONE',  ( 62.43652093785069468, -177.1207230881787780, 55.44293326708522329 ) ) ;
#30176=DIRECTION ( 'NONE',  ( -0.2635871660690783380, 0.000000000000000000, 0.9646355819083558547 ) ) ;
#30179=CIRCLE ( 'NONE', #25156, 125.0000000000000000 ) ;
#30182=FACE_OUTER_BOUND ( 'NONE', #50770, .T. ) ;
#30184=EDGE_CURVE ( 'NONE', #12871, #48304, #51602, .T. ) ;
#30185=ORIENTED_EDGE ( 'NONE', *, *, #20427, .T. ) ;
#30186=CARTESIAN_POINT ( 'NONE',  ( -65.47874029382339245, -193.5000000000000000, 122.8300162461137006 ) ) ;
#30190=VERTEX_POINT ( 'NONE', #29922 ) ;
#30191=EDGE_CURVE ( 'NONE', #17270, #47175, #28674, .T. ) ;
#30192=DIRECTION ( 'NONE',  ( 0.000000000000000000, 0.000000000000000000, 1.000000000000000000 ) ) ;
#30194=ADVANCED_FACE ( 'NONE', ( #24752 ), #9971, .T. ) ;
#30195=ORIENTED_EDGE ( 'NONE', *, *, #6041, .T. ) ;
#30196=DIRECTION ( 'NONE',  ( -0.000000000000000000, 1.000000000000000000, -0.000000000000000000 ) ) ;
#30197=EDGE_LOOP ( 'NONE', ( #45676, #1221, #10417, #47601 ) ) ;
#30198=ADVANCED_FACE ( 'NONE', ( #26225 ), #4789, .T. ) ;
#30199=VECTOR ( 'NONE', #2548, 1000.000000000000000 ) ;
#30200=CARTESIAN_POINT ( 'NONE',  ( -123.4791267515088435, -198.5000000000000000, 60.00000000000001421 ) ) ;
#30202=CARTESIAN_POINT ( 'NONE',  ( -169.8550585387150136, -189.7472609257535510, 25.37485791684378711 ) ) ;
#30203=DIRECTION ( 'NONE',  ( -0.000000000000000000, 1.000000000000000000, 0.000000000000000000 ) ) ;
#30204=CARTESIAN_POINT ( 'NONE',  ( -48.47912675150885065, -189.7472609257535510, 6.938893903907228378E-15 ) ) ;
#30206=CYLINDRICAL_SURFACE ( 'NONE', #17257, 125.0000000000000000 ) ;
#30207=EDGE_CURVE ( 'NONE', #40028, #15743, #12985, .T. ) ;
#30208=ORIENTED_EDGE ( 'NONE', *, *, #51138, .F. ) ;
#30209=CYLINDRICAL_SURFACE ( 'NONE', #10749, 124.9999999999999858 ) ;
#30210=VECTOR ( 'NONE', #13651, 1000.000000000000114 ) ;
#30216=VERTEX_POINT ( 'NONE', #48935 ) ;
#30217=DIRECTION ( 'NONE',  ( 0.9785564922995046988, 0.000000000000000000, -0.2059786187410953262 ) ) ;
#30222=LINE ( 'NONE', #14712, #44014 ) ;
#30223=EDGE_LOOP ( 'NONE', ( #4000, #33058, #30540, #26762 ) ) ;
#30225=EDGE_CURVE ( 'NONE', #25185, #18665, #37804, .T. ) ;
#30229=EDGE_LOOP ( 'NONE', ( #21994, #16093, #27460, #51212 ) ) ;
#30231=AXIS2_PLACEMENT_3D ( 'NONE', #31364, #47406, #27419 ) ;
#30232=AXIS2_PLACEMENT_3D ( 'NONE', #14886, #34565, #30898 ) ;
#30233=CARTESIAN_POINT ( 'NONE',  ( -48.47912675150885065, -188.5000000000000284, 6.938893903907228378E-15 ) ) ;
#30234=VERTEX_POINT ( 'NONE', #6276 ) ;
#30236=DIRECTION ( 'NONE',  ( 0.000000000000000000, 1.000000000000000000, 0.000000000000000000 ) ) ;
#30237=EDGE_LOOP ( 'NONE', ( #25363, #4585, #6715, #42737 ) ) ;
#30239=DIRECTION ( 'NONE',  ( 0.4566292373937140270, 0.000000000000000000, -0.8896570909947467687 ) ) ;
#30242=CARTESIAN_POINT ( 'NONE',  ( 64.29733702426838704, -189.7472609257535510, 53.91167979418565182 ) ) ;
#30243=ORIENTED_EDGE ( 'NONE', *, *, #20417, .T. ) ;
#30244=DIRECTION ( 'NONE',  ( 0.4827922027307366970, 0.000000000000000000, 0.8757349421956412971 ) ) ;
#30245=PLANE ( 'NONE',  #41563 ) ;
#30247=EDGE_LOOP ( 'NONE', ( #24104, #48172, #12620, #39631 ) ) ;
#30252=FACE_OUTER_BOUND ( 'NONE', #29976, .T. ) ;
#30253=DIRECTION ( 'NONE',  ( 0.000000000000000000, 0.000000000000000000, -1.000000000000000000 ) ) ;
#30254=ADVANCED_FACE ( 'NONE', ( #8455 ), #24483, .T. ) ;
#30256=DIRECTION ( 'NONE',  ( 0.000000000000000000, -0.000000000000000000, 1.000000000000000000 ) ) ;
#30257=CARTESIAN_POINT ( 'NONE',  ( 14.37129481273060172, -189.7472609257535510, -108.0501018472328099 ) ) ;
#30258=DIRECTION ( 'NONE',  ( -0.8896570909947467687, 0.000000000000000000, -0.4566292373937140270 ) ) ;
#30261=VECTOR ( 'NONE', #10305, 1000.000000000000000 ) ;
#30263=DIRECTION ( 'NONE',  ( 0.000000000000000000, 1.000000000000000000, 0.000000000000000000 ) ) ;
#30264=DIRECTION ( 'NONE',  ( 0.8455960035018234011, 0.000000000000000000, 0.5338233779647948429 ) ) ;
#30265=ORIENTED_EDGE ( 'NONE', *, *, #28901, .T. ) ;
#30270=CARTESIAN_POINT ( 'NONE',  ( -18.95304271317703382, -193.5000000000000000, -121.4627941443854837 ) ) ;
#30273=CARTESIAN_POINT ( 'NONE',  ( -48.07600332222088468, -175.3837268820161057, 0.9151456172430280089 ) ) ;
#30274=DIRECTION ( 'NONE',  ( 0.000000000000000000, 1.000000000000000000, -0.000000000000000000 ) ) ;
#30275=DIRECTION ( 'NONE',  ( -0.000000000000000000, 1.000000000000000000, -0.000000000000000000 ) ) ;
#30277=AXIS2_PLACEMENT_3D ( 'NONE', #36667, #40855, #8029 ) ;
#30278=PLANE ( 'NONE',  #44068 ) ;
#30279=VERTEX_POINT ( 'NONE', #18620 ) ;
#30280=LINE ( 'NONE', #26847, #22189 ) ;
#30281=VERTEX_POINT ( 'NONE', #18863 ) ;
#30282=EDGE_CURVE ( 'NONE', #19235, #51805, #30685, .T. ) ;
#30283=CARTESIAN_POINT ( 'NONE',  ( -120.5074237604784315, -183.6283474603465606, 100.9358816284415923 ) ) ;
#30284=CARTESIAN_POINT ( 'NONE',  ( 75.78974234412359579, -183.6283474603465606, 13.49993235881449394 ) ) ;
#30286=EDGE_LOOP ( 'NONE', ( #14218, #6730, #35705, #37050 ) ) ;
#30287=DIRECTION ( 'NONE',  ( 0.2920567706369628924, 0.000000000000000000, 0.9564009842765264224 ) ) ;
#30289=VERTEX_POINT ( 'NONE', #47262 ) ;
#30290=CARTESIAN_POINT ( 'NONE',  ( -102.0975050429524771, -193.5000000000000000, -111.8087531435654114 ) ) ;
#30291=VECTOR ( 'NONE', #6607, 1000.000000000000000 ) ;
#30292=LINE ( 'NONE', #11086, #6408 ) ;
#30295=DIRECTION ( 'NONE',  ( 0.5829794791144650157, 0.000000000000000000, 0.8124868780056864193 ) ) ;
#30296=AXIS2_PLACEMENT_3D ( 'NONE', #2341, #21535, #10461 ) ;
#30297=ORIENTED_EDGE ( 'NONE', *, *, #4412, .F. ) ;
#30299=ORIENTED_EDGE ( 'NONE', *, *, #40850, .F. ) ;
#30300=DIRECTION ( 'NONE',  ( 0.000000000000000000, -1.000000000000000000, 0.000000000000000000 ) ) ;
#30301=LINE ( 'NONE', #17719, #21901 ) ;
#30303=ORIENTED_EDGE ( 'NONE', *, *, #44246, .F. ) ;
#30306=CARTESIAN_POINT ( 'NONE',  ( -48.47912675150885065, -189.7472609257535510, 6.938893903907228378E-15 ) ) ;
#30307=ORIENTED_EDGE ( 'NONE', *, *, #42309, .T. ) ;
#30308=CARTESIAN_POINT ( 'NONE',  ( -47.48307690889363641, -183.6283474603465606, 0.08879589532294547560 ) ) ;
#30309=VERTEX_POINT ( 'NONE', #39085 ) ;
#30310=VECTOR ( 'NONE', #5599, 1000.000000000000000 ) ;
#30311=LINE ( 'NONE', #6158, #19406 ) ;
#30314=ORIENTED_EDGE ( 'NONE', *, *, #34960, .F. ) ;
#30315=VERTEX_POINT ( 'NONE', #10732 ) ;
#30317=CARTESIAN_POINT ( 'NONE',  ( -59.86929868745821182, -177.1207230881787780, -124.4799742258549600 ) ) ;
#30318=ORIENTED_EDGE ( 'NONE', *, *, #47325, .F. ) ;
#30319=DIRECTION ( 'NONE',  ( -0.000000000000000000, -1.000000000000000000, 0.000000000000000000 ) ) ;
#30321=DIRECTION ( 'NONE',  ( 0.000000000000000000, -1.000000000000000000, 0.000000000000000000 ) ) ;
#30322=CARTESIAN_POINT ( 'NONE',  ( 48.06131630543706734, -193.5000000000000000, -79.40367028273054473 ) ) ;
#30324=AXIS2_PLACEMENT_3D ( 'NONE', #47452, #8017, #24053 ) ;
#30326=DIRECTION ( 'NONE',  ( 0.000000000000000000, 1.000000000000000000, 0.000000000000000000 ) ) ;
#30327=ORIENTED_EDGE ( 'NONE', *, *, #43847, .F. ) ;
#30328=ORIENTED_EDGE ( 'NONE', *, *, #31088, .F. ) ;
#30331=EDGE_CURVE ( 'NONE', #50673, #45478, #41538, .T. ) ;
#30333=DIRECTION ( 'NONE',  ( 0.000000000000000000, 0.000000000000000000, -1.000000000000000000 ) ) ;
#30334=DIRECTION ( 'NONE',  ( -0.4827922027307551267, 0.000000000000000000, 0.8757349421956311941 ) ) ;
#30336=EDGE_LOOP ( 'NONE', ( #21221, #18761, #21371, #37957 ) ) ;
#30337=EDGE_CURVE ( 'NONE', #30190, #4219, #20531, .T. ) ;
#30340=EDGE_CURVE ( 'NONE', #40028, #787, #26756, .T. ) ;
#30341=EDGE_LOOP ( 'NONE', ( #20749, #10882, #14892, #324 ) ) ;
#30343=CARTESIAN_POINT ( 'NONE',  ( -47.64924157374594671, -189.7472609257535510, 124.9972451320097377 ) ) ;
#30344=EDGE_CURVE ( 'NONE', #33832, #18089, #33961, .T. ) ;
#30346=DIRECTION ( 'NONE',  ( -0.000000000000000000, 1.000000000000000000, 0.000000000000000000 ) ) ;
#30347=LINE ( 'NONE', #46395, #28333 ) ;
#30348=CARTESIAN_POINT ( 'NONE',  ( -167.1580984288390823, -189.7472609257535510, -39.24667733211878584 ) ) ;
#30350=EDGE_LOOP ( 'NONE', ( #37261, #35999, #40184, #46406 ) ) ;
#30351=CARTESIAN_POINT ( 'NONE',  ( -92.78132261338706144, -189.7472609257535510, -116.8859077982276631 ) ) ;
#30353=ORIENTED_EDGE ( 'NONE', *, *, #25830, .F. ) ;
#30355=DIRECTION ( 'NONE',  ( 0.000000000000000000, -1.000000000000000000, 0.000000000000000000 ) ) ;
#30356=EDGE_CURVE ( 'NONE', #19079, #50975, #14425, .T. ) ;
#30359=CARTESIAN_POINT ( 'NONE',  ( -101.9736325116273576, -183.6283474603465606, 112.9749434763330527 ) ) ;
#30360=CARTESIAN_POINT ( 'NONE',  ( -81.70897914701313880, -177.1207230881787780, -120.5021863277716534 ) ) ;
#30361=DIRECTION ( 'NONE',  ( 0.000000000000000000, 1.000000000000000000, 0.000000000000000000 ) ) ;
#30363=CIRCLE ( 'NONE', #17779, 125.0000000000000000 ) ;
#30364=ORIENTED_EDGE ( 'NONE', *, *, #34592, .F. ) ;
#30365=CARTESIAN_POINT ( 'NONE',  ( -49.46816693883101834, -193.5000000000000000, 0.1476465640024780257 ) ) ;
#30366=ORIENTED_EDGE ( 'NONE', *, *, #10244, .F. ) ;
#30367=VERTEX_POINT ( 'NONE', #30431 ) ;
#30368=FACE_OUTER_BOUND ( 'NONE', #9282, .T. ) ;
#30369=EDGE_LOOP ( 'NONE', ( #37554, #36549, #42960, #27485 ) ) ;
#30373=CIRCLE ( 'NONE', #17831, 125.0000000000000000 ) ;
#30374=ORIENTED_EDGE ( 'NONE', *, *, #7672, .T. ) ;
#30375=LINE ( 'NONE', #38004, #30142 ) ;
#30376=DIRECTION ( 'NONE',  ( -0.9027978299657477557, 0.000000000000000000, 0.4300652022765115712 ) ) ;
#30377=VERTEX_POINT ( 'NONE', #27006 ) ;
#30378=DIRECTION ( 'NONE',  ( -0.9995608365087944591, 0.000000000000000000, 0.02963332782255633305 ) ) ;
#30380=EDGE_CURVE ( 'NONE', #10133, #47358, #30959, .T. ) ;
#30382=CARTESIAN_POINT ( 'NONE',  ( 65.38692482895591240, -193.5000000000000000, -51.57055649762701677 ) ) ;
#30383=ORIENTED_EDGE ( 'NONE', *, *, #28475, .T. ) ;
#30384=ORIENTED_EDGE ( 'NONE', *, *, #41857, .F. ) ;
#30388=( LENGTH_UNIT ( ) NAMED_UNIT ( * ) SI_UNIT ( .MILLI., .METRE. ) );
#30391=AXIS2_PLACEMENT_3D ( 'NONE', #2883, #18666, #50729 ) ;
#30392=VERTEX_POINT ( 'NONE', #6546 ) ;
#30394=ADVANCED_FACE ( 'NONE', ( #23076 ), #3098, .T. ) ;
#30395=VECTOR ( 'NONE', #25800, 1000.000000000000000 ) ;
#30397=ORIENTED_EDGE ( 'NONE', *, *, #9938, .F. ) ;
#30398=DIRECTION ( 'NONE',  ( 0.000000000000000000, 0.000000000000000000, 1.000000000000000000 ) ) ;
#30401=EDGE_CURVE ( 'NONE', #7429, #41297, #39353, .T. ) ;
#30403=EDGE_LOOP ( 'NONE', ( #36341, #5966, #6683, #35096 ) ) ;
#30406=EDGE_CURVE ( 'NONE', #5648, #39766, #27527, .T. ) ;
#30407=DIRECTION ( 'NONE',  ( 0.000000000000000000, -1.000000000000000000, 0.000000000000000000 ) ) ;
#30411=VERTEX_POINT ( 'NONE', #47775 ) ;
#30412=VECTOR ( 'NONE', #14757, 1000.000000000000000 ) ;
#30413=VECTOR ( 'NONE', #14594, 1000.000000000000114 ) ;
#30414=EDGE_LOOP ( 'NONE', ( #1941, #47719, #4688, #30022 ) ) ;
#30415=DIRECTION ( 'NONE',  ( -0.9266896074318370369, 0.000000000000000000, 0.3758275821142292306 ) ) ;
#30416=AXIS2_PLACEMENT_3D ( 'NONE', #29330, #8333, #8837 ) ;
#30417=CARTESIAN_POINT ( 'NONE',  ( -163.0741914257288272, -193.5000000000000000, 47.37063079638402030 ) ) ;
#30419=DIRECTION ( 'NONE',  ( -0.2348860457809911206, 0.000000000000000000, 0.9720229140804089729 ) ) ;
#30423=CARTESIAN_POINT ( 'NONE',  ( -238.7407812814481076, -213.5000000000000000, 41.45482488023466772 ) ) ;
#30424=DIRECTION ( 'NONE',  ( -0.000000000000000000, 1.000000000000000000, 0.000000000000000000 ) ) ;
#30427=CARTESIAN_POINT ( 'NONE',  ( 24.63024857337166296, -177.1207230881787780, 101.3904297239426597 ) ) ;
#30428=CARTESIAN_POINT ( 'NONE',  ( -47.49008656418669005, -193.5000000000000000, 0.1476465640024920423 ) ) ;
#30429=CARTESIAN_POINT ( 'NONE',  ( -108.0638572795231624, -193.5000000000000000, 108.7464374498172788 ) ) ;
#30430=ORIENTED_EDGE ( 'NONE', *, *, #29092, .F. ) ;
#30431=CARTESIAN_POINT ( 'NONE',  ( 1.150725574412429175, -189.7472609257535510, -114.7252272087845739 ) ) ;
#30432=CARTESIAN_POINT ( 'NONE',  ( 72.71365293123227502, -177.1207230881787780, -30.61552143554913030 ) ) ;
#30433=EDGE_LOOP ( 'NONE', ( #43489, #14643, #4911, #39491 ) ) ;
#30436=VECTOR ( 'NONE', #17919, 1000.000000000000000 ) ;
#30437=EDGE_CURVE ( 'NONE', #49553, #11600, #12785, .T. ) ;
#30440=CARTESIAN_POINT ( 'NONE',  ( -123.4791267515088435, -198.5000000000000000, 70.00000000000000000 ) ) ;
#30441=ADVANCED_FACE ( 'NONE', ( #717 ), #28808, .T. ) ;
#30444=ADVANCED_FACE ( 'NONE', ( #44598 ), #12536, .T. ) ;
#30446=AXIS2_PLACEMENT_3D ( 'NONE', #37864, #38384, #38114 ) ;
#30448=ORIENTED_EDGE ( 'NONE', *, *, #3159, .F. ) ;
#30450=CARTESIAN_POINT ( 'NONE',  ( 57.61256176024323139, -177.1207230881787780, -64.19309449102733822 ) ) ;
#30455=ORIENTED_EDGE ( 'NONE', *, *, #32272, .T. ) ;
#30459=EDGE_CURVE ( 'NONE', #51292, #17406, #36182, .T. ) ;
#30460=CARTESIAN_POINT ( 'NONE',  ( 37.99238433767461487, -175.3837268820161057, -90.26448786734027863 ) ) ;
#30466=EDGE_CURVE ( 'NONE', #15488, #8881, #40630, .T. ) ;
#30467=DIRECTION ( 'NONE',  ( 0.000000000000000000, -0.000000000000000000, 1.000000000000000000 ) ) ;
#30468=ORIENTED_EDGE ( 'NONE', *, *, #26912, .T. ) ;
#30469=LINE ( 'NONE', #29962, #42357 ) ;
#30475=CARTESIAN_POINT ( 'NONE',  ( 43.12693905415815721, -189.7472609257535510, -83.57229767764155781 ) ) ;
#30476=ORIENTED_EDGE ( 'NONE', *, *, #43744, .T. ) ;
#30477=VERTEX_POINT ( 'NONE', #11749 ) ;
#30478=EDGE_CURVE ( 'NONE', #15102, #39679, #4928, .T. ) ;
#30479=DIRECTION ( 'NONE',  ( 0.000000000000000000, -1.000000000000000000, 0.000000000000000000 ) ) ;
#30480=ORIENTED_EDGE ( 'NONE', *, *, #22922, .T. ) ;
#30482=DIRECTION ( 'NONE',  ( 0.000000000000000000, 1.000000000000000000, 0.000000000000000000 ) ) ;
#30483=VERTEX_POINT ( 'NONE', #51718 ) ;
#30485=CARTESIAN_POINT ( 'NONE',  ( -71.40672220061267694, -175.3837268820161057, -122.8793122007208751 ) ) ;
#30488=CARTESIAN_POINT ( 'NONE',  ( -148.6149069237406195, -183.6283474603465606, -74.81861753132355375 ) ) ;
#30489=ORIENTED_EDGE ( 'NONE', *, *, #49889, .F. ) ;
#30492=EDGE_CURVE ( 'NONE', #27780, #22881, #42406, .T. ) ;
#30493=CARTESIAN_POINT ( 'NONE',  ( -134.7293151056888121, -189.7472609257535510, -89.08931047202582931 ) ) ;
#30496=VECTOR ( 'NONE', #16203, 1000.000000000000000 ) ;
#30497=DIRECTION ( 'NONE',  ( 0.000000000000000000, -0.000000000000000000, -1.000000000000000000 ) ) ;
#30499=CARTESIAN_POINT ( 'NONE',  ( -65.47874029382337824, -177.1207230881787780, 122.8300162461137006 ) ) ;
#30502=ORIENTED_EDGE ( 'NONE', *, *, #28902, .T. ) ;
#30504=DIRECTION ( 'NONE',  ( 0.000000000000000000, 0.000000000000000000, 1.000000000000000000 ) ) ;
#30508=EDGE_CURVE ( 'NONE', #24657, #23768, #3803, .T. ) ;
#30509=ADVANCED_FACE ( 'NONE', ( #32767 ), #27775, .T. ) ;
#30510=DIRECTION ( 'NONE',  ( 0.000000000000000000, 0.000000000000000000, 1.000000000000000000 ) ) ;
#30511=CIRCLE ( 'NONE', #51497, 125.0000000000000000 ) ;
#30513=EDGE_CURVE ( 'NONE', #50350, #23163, #4149, .T. ) ;
#30514=LINE ( 'NONE', #22896, #38911 ) ;
#30515=VERTEX_POINT ( 'NONE', #12267 ) ;
#30516=ORIENTED_EDGE ( 'NONE', *, *, #21536, .T. ) ;
#30517=ORIENTED_EDGE ( 'NONE', *, *, #32622, .T. ) ;
#30519=CARTESIAN_POINT ( 'NONE',  ( 35.45604639379470058, -193.5000000000000000, 91.27439114664650788 ) ) ;
#30520=LINE ( 'NONE', #42348, #25471 ) ;
#30525=DIRECTION ( 'NONE',  ( -0.000000000000000000, -1.000000000000000000, 0.000000000000000000 ) ) ;
#30527=ORIENTED_EDGE ( 'NONE', *, *, #46911, .F. ) ;
#30528=ADVANCED_FACE ( 'NONE', ( #21975 ), #37997, .T. ) ;
#30529=DIRECTION ( 'NONE',  ( 0.000000000000000000, 1.000000000000000000, 0.000000000000000000 ) ) ;
#30534=DIRECTION ( 'NONE',  ( -0.000000000000000000, 1.000000000000000000, -0.000000000000000000 ) ) ;
#30536=ADVANCED_FACE ( 'NONE', ( #42193 ), #41943, .T. ) ;
#30537=ORIENTED_EDGE ( 'NONE', *, *, #22155, .T. ) ;
#30538=CARTESIAN_POINT ( 'NONE',  ( -49.25565061422688728, -183.6283474603465606, -0.6300878435817132139 ) ) ;
#30539=DIRECTION ( 'NONE',  ( -0.000000000000000000, 1.000000000000000000, 0.000000000000000000 ) ) ;
#30540=ORIENTED_EDGE ( 'NONE', *, *, #140, .F. ) ;
#30542=AXIS2_PLACEMENT_3D ( 'NONE', #24877, #51611, #40537 ) ;
#30544=VECTOR ( 'NONE', #7859, 1000.000000000000000 ) ;
#30546=LINE ( 'NONE', #46597, #40175 ) ;
#30547=DIRECTION ( 'NONE',  ( 0.8124868780056863082, 0.000000000000000000, -0.5829794791144649047 ) ) ;
#30552=DIRECTION ( 'NONE',  ( -0.9266896074318291543, 0.000000000000000000, -0.3758275821142488260 ) ) ;
#30553=CARTESIAN_POINT ( 'NONE',  ( 74.49773146996547268, -193.5000000000000000, -22.39848972532282190 ) ) ;
#30554=ORIENTED_EDGE ( 'NONE', *, *, #49403, .T. ) ;
#30556=CARTESIAN_POINT ( 'NONE',  ( 76.04209377433248562, -175.3837268820161057, -10.93003379476866677 ) ) ;
#30557=DIRECTION ( 'NONE',  ( 0.000000000000000000, -0.000000000000000000, 1.000000000000000000 ) ) ;
#30558=VECTOR ( 'NONE', #50389, 1000.000000000000000 ) ;
#30560=PLANE ( 'NONE',  #22886 ) ;
#30561=ORIENTED_EDGE ( 'NONE', *, *, #18905, .F. ) ;
#30562=PLANE ( 'NONE',  #21105 ) ;
#30565=ORIENTED_EDGE ( 'NONE', *, *, #13978, .F. ) ;
#30566=ORIENTED_EDGE ( 'NONE', *, *, #7143, .T. ) ;
#30567=EDGE_CURVE ( 'NONE', #48304, #12908, #49845, .T. ) ;
#30568=DIRECTION ( 'NONE',  ( -0.9785564922995060311, 0.000000000000000000, 0.2059786187410889424 ) ) ;
#30570=EDGE_LOOP ( 'NONE', ( #32032, #30755, #13012, #6068 ) ) ;
#30571=FACE_OUTER_BOUND ( 'NONE', #44310, .T. ) ;
#30572=ORIENTED_EDGE ( 'NONE', *, *, #37450, .T. ) ;
#30574=CARTESIAN_POINT ( 'NONE',  ( -48.47912675150885065, -183.6283474603465606, 6.938893903907228378E-15 ) ) ;
#30575=VECTOR ( 'NONE', #25766, 1000.000000000000000 ) ;
#30576=VECTOR ( 'NONE', #23473, 1000.000000000000000 ) ;
#30577=LINE ( 'NONE', #6935, #12704 ) ;
#30578=PLANE ( 'NONE',  #18193 ) ;
#30580=VERTEX_POINT ( 'NONE', #25656 ) ;
#30581=VECTOR ( 'NONE', #18797, 1000.000000000000000 ) ;
#30583=DIRECTION ( 'NONE',  ( 0.000000000000000000, -1.000000000000000000, 0.000000000000000000 ) ) ;
#30585=EDGE_CURVE ( 'NONE', #15918, #32858, #31481, .T. ) ;
#30586=DIRECTION ( 'NONE',  ( 0.4031234292879665171, 0.000000000000000000, 0.9151456172430210145 ) ) ;
#30587=CARTESIAN_POINT ( 'NONE',  ( 48.33059356687144970, -175.3837268820161057, 77.48473115145309009 ) ) ;
#30588=ORIENTED_EDGE ( 'NONE', *, *, #32045, .T. ) ;
#30592=EDGE_CURVE ( 'NONE', #52027, #34819, #41688, .T. ) ;
#30593=VERTEX_POINT ( 'NONE', #961 ) ;
#30597=CARTESIAN_POINT ( 'NONE',  ( -7.223120065443615623, -193.5000000000000000, 117.9955164924470523 ) ) ;
#30598=CARTESIAN_POINT ( 'NONE',  ( -48.47912675150885065, -189.7472609257535510, 6.938893903907228378E-15 ) ) ;
#30599=ORIENTED_EDGE ( 'NONE', *, *, #51160, .F. ) ;
#30600=DIRECTION ( 'NONE',  ( 0.000000000000000000, 0.000000000000000000, 1.000000000000000000 ) ) ;
#30602=ORIENTED_EDGE ( 'NONE', *, *, #15519, .F. ) ;
#30604=VECTOR ( 'NONE', #34870, 1000.000000000000000 ) ;
#30608=DIRECTION ( 'NONE',  ( -0.000000000000000000, 1.000000000000000000, -0.000000000000000000 ) ) ;
#30613=ADVANCED_FACE ( 'NONE', ( #5445 ), #46167, .T. ) ;
#30614=CARTESIAN_POINT ( 'NONE',  ( -49.45768324380835423, -193.5000000000000000, -0.2059786187411025149 ) ) ;
#30615=EDGE_LOOP ( 'NONE', ( #29927, #47734, #22696, #40252 ) ) ;
#30616=CIRCLE ( 'NONE', #421, 125.0000000000000000 ) ;
#30621=DIRECTION ( 'NONE',  ( 0.2920567706369694982, 0.000000000000000000, 0.9564009842765243130 ) ) ;
#30622=EDGE_CURVE ( 'NONE', #43863, #42973, #21726, .T. ) ;
#30624=ORIENTED_EDGE ( 'NONE', *, *, #39424, .F. ) ;
#30625=AXIS2_PLACEMENT_3D ( 'NONE', #14705, #10756, #38860 ) ;
#30627=DIRECTION ( 'NONE',  ( -0.000000000000000000, 1.000000000000000000, -0.000000000000000000 ) ) ;
#30630=CARTESIAN_POINT ( 'NONE',  ( 64.72501964220592185, -175.3837268820161057, 53.00774697410174952 ) ) ;
#30631=LINE ( 'NONE', #38536, #35507 ) ;
#30636=EDGE_LOOP ( 'NONE', ( #38293, #17633, #11503, #43781 ) ) ;
#30637=VERTEX_POINT ( 'NONE', #33551 ) ;
#30638=EDGE_LOOP ( 'NONE', ( #18646, #17867, #23525, #2565 ) ) ;
#30639=CARTESIAN_POINT ( 'NONE',  ( 72.95485052494852596, -183.6283474603465606, -29.64437826672758192 ) ) ;
#30640=CARTESIAN_POINT ( 'NONE',  ( 65.79610465833508215, -177.1207230881787780, -50.65739320401928580 ) ) ;
#30641=VECTOR ( 'NONE', #36836, 1000.000000000000227 ) ;
#30642=ADVANCED_FACE ( 'NONE', ( #26161 ), #9125, .T. ) ;
#30647=VERTEX_POINT ( 'NONE', #5186 ) ;
#30648=AXIS2_PLACEMENT_3D ( 'NONE', #18227, #28538, #44584 ) ;
#30650=CARTESIAN_POINT ( 'NONE',  ( -37.67038537088846084, -177.1207230881787780, -124.5318076226586470 ) ) ;
#30651=EDGE_LOOP ( 'NONE', ( #11965, #48216, #31658, #27861 ) ) ;
#30652=DIRECTION ( 'NONE',  ( 0.000000000000000000, 0.000000000000000000, 1.000000000000000000 ) ) ;
#30654=ORIENTED_EDGE ( 'NONE', *, *, #436, .T. ) ;
#30655=CARTESIAN_POINT ( 'NONE',  ( 72.35619569422320296, -193.5000000000000000, 27.83926365844748574 ) ) ;
#30656=CIRCLE ( 'NONE', #27283, 125.0000000000000000 ) ;
#30659=VECTOR ( 'NONE', #32758, 1000.000000000000000 ) ;
#30661=CARTESIAN_POINT ( 'NONE',  ( -159.5526844214375615, -177.1207230881787780, 57.33816169485226055 ) ) ;
#30662=EDGE_LOOP ( 'NONE', ( #13557, #13390, #36946, #5510 ) ) ;
#30664=AXIS2_PLACEMENT_3D ( 'NONE', #47348, #43408, #31560 ) ;
#30666=AXIS2_PLACEMENT_3D ( 'NONE', #49613, #35068, #11140 ) ;
#30667=ORIENTED_EDGE ( 'NONE', *, *, #28579, .T. ) ;
#30669=DIRECTION ( 'NONE',  ( -0.000000000000000000, 1.000000000000000000, -0.000000000000000000 ) ) ;
#30670=DIRECTION ( 'NONE',  ( 0.000000000000000000, 0.000000000000000000, 1.000000000000000000 ) ) ;
#30671=DIRECTION ( 'NONE',  ( -0.000000000000000000, 1.000000000000000000, -0.000000000000000000 ) ) ;
#30673=DIRECTION ( 'NONE',  ( 0.000000000000000000, -1.000000000000000000, 0.000000000000000000 ) ) ;
#30675=EDGE_CURVE ( 'NONE', #19021, #33918, #17014, .T. ) ;
#30679=ORIENTED_EDGE ( 'NONE', *, *, #24893, .T. ) ;
#30681=CYLINDRICAL_SURFACE ( 'NONE', #19764, 125.0000000000000000 ) ;
#30682=FACE_BOUND ( 'NONE', #5165, .T. ) ;
#30683=VERTEX_POINT ( 'NONE', #41166 ) ;
#30684=AXIS2_PLACEMENT_3D ( 'NONE', #47316, #51510, #48343 ) ;
#30685=LINE ( 'NONE', #22573, #5474 ) ;
#30686=CIRCLE ( 'NONE', #11365, 125.0000000000000000 ) ;
#30687=VECTOR ( 'NONE', #34499, 1000.000000000000114 ) ;
#30688=CARTESIAN_POINT ( 'NONE',  ( -156.2577088867455473, -177.1207230881787780, -63.31490529818419333 ) ) ;
#30689=VERTEX_POINT ( 'NONE', #49331 ) ;
#30697=CIRCLE ( 'NONE', #34894, 125.0000000000000000 ) ;
#30698=DIRECTION ( 'NONE',  ( -0.000000000000000000, -1.000000000000000000, 0.000000000000000000 ) ) ;
#30699=CARTESIAN_POINT ( 'NONE',  ( -158.1873290247468447, -183.6283474603465606, 57.79541595648306185 ) ) ;
#30706=ORIENTED_EDGE ( 'NONE', *, *, #26620, .T. ) ;
#30707=VECTOR ( 'NONE', #7234, 1000.000000000000000 ) ;
#30709=VERTEX_POINT ( 'NONE', #51400 ) ;
#30710=CARTESIAN_POINT ( 'NONE',  ( -162.4844509910036265, -177.1207230881787780, -48.77484799213895172 ) ) ;
#30711=DIRECTION ( 'NONE',  ( 0.000000000000000000, 0.000000000000000000, 1.000000000000000000 ) ) ;
#30713=ORIENTED_EDGE ( 'NONE', *, *, #16889, .T. ) ;
#30715=CARTESIAN_POINT ( 'NONE',  ( -77.03256798524175508, -193.5000000000000000, 121.6951149130964893 ) ) ;
#30716=ORIENTED_EDGE ( 'NONE', *, *, #33303, .F. ) ;
#30718=CIRCLE ( 'NONE', #44156, 125.0000000000000000 ) ;
#30721=EDGE_LOOP ( 'NONE', ( #3053, #33575, #42741, #7239 ) ) ;
#30724=AXIS2_PLACEMENT_3D ( 'NONE', #8400, #498, #48346 ) ;
#30725=DIRECTION ( 'NONE',  ( 0.8124868780056783146, 0.000000000000000000, 0.5829794791144762289 ) ) ;
#30726=DIRECTION ( 'NONE',  ( 0.000000000000000000, -1.000000000000000000, -0.000000000000000000 ) ) ;
#30730=CARTESIAN_POINT ( 'NONE',  ( -47.74129347246712740, -189.7472609257535510, -0.6749830015182022303 ) ) ;
#30733=AXIS2_PLACEMENT_3D ( 'NONE', #18218, #14274, #17457 ) ;
#30734=CARTESIAN_POINT ( 'NONE',  ( 72.05536924052414349, -175.3837268820161057, 33.11246405730899056 ) ) ;
#30735=ORIENTED_EDGE ( 'NONE', *, *, #6740, .F. ) ;
#30739=PLANE ( 'NONE',  #25761 ) ;
#30742=VECTOR ( 'NONE', #10969, 1000.000000000000000 ) ;
#30743=PLANE ( 'NONE',  #34118 ) ;
#30744=ADVANCED_FACE ( 'NONE', ( #50616 ), #15392, .T. ) ;
#30750=DIRECTION ( 'NONE',  ( 0.000000000000000000, -0.000000000000000000, -1.000000000000000000 ) ) ;
#30751=EDGE_CURVE ( 'NONE', #43088, #121, #46944, .T. ) ;
#30753=EDGE_CURVE ( 'NONE', #44939, #24499, #11331, .T. ) ;
#30754=DIRECTION ( 'NONE',  ( 0.000000000000000000, 0.000000000000000000, -1.000000000000000000 ) ) ;
#30755=ORIENTED_EDGE ( 'NONE', *, *, #19246, .F. ) ;
#30756=PLANE ( 'NONE',  #42435 ) ;
#30757=EDGE_CURVE ( 'NONE', #43961, #37405, #47446, .T. ) ;
#30758=CARTESIAN_POINT ( 'NONE',  ( -48.24424070572787571, -183.6283474603465606, 0.9720229140804191870 ) ) ;
#30760=CARTESIAN_POINT ( 'NONE',  ( -89.73513343757491612, -183.6283474603465606, -117.9955164924467397 ) ) ;
#30761=CARTESIAN_POINT ( 'NONE',  ( -121.1142239062970276, -183.6283474603465606, 101.7307360698549417 ) ) ;
#30763=VERTEX_POINT ( 'NONE', #2523 ) ;
#30765=EDGE_CURVE ( 'NONE', #8260, #29691, #22256, .T. ) ;
#30767=LINE ( 'NONE', #25131, #27900 ) ;
#30769=EDGE_CURVE ( 'NONE', #3044, #30683, #18552, .T. ) ;
#30772=AXIS2_PLACEMENT_3D ( 'NONE', #25781, #41815, #2391 ) ;
#30773=EDGE_CURVE ( 'NONE', #17455, #47251, #10397, .T. ) ;
#30774=ORIENTED_EDGE ( 'NONE', *, *, #32115, .F. ) ;
#30777=ORIENTED_EDGE ( 'NONE', *, *, #39998, .F. ) ;
#30778=AXIS2_PLACEMENT_3D ( 'NONE', #27643, #26608, #19490 ) ;
#30779=ORIENTED_EDGE ( 'NONE', *, *, #9895, .F. ) ;
#30782=FACE_OUTER_BOUND ( 'NONE', #28992, .T. ) ;
#30783=AXIS2_PLACEMENT_3D ( 'NONE', #46078, #6381, #22404 ) ;
#30784=AXIS2_PLACEMENT_3D ( 'NONE', #46346, #2451, #18479 ) ;
#30785=DIRECTION ( 'NONE',  ( -0.3758275821142488260, 0.000000000000000000, 0.9266896074318291543 ) ) ;
#30788=ADVANCED_FACE ( 'NONE', ( #27464 ), #31146, .T. ) ;
#30791=CARTESIAN_POINT ( 'NONE',  ( 47.91692961953209817, -193.5000000000000000, -77.99872144864701795 ) ) ;
#30792=CARTESIAN_POINT ( 'NONE',  ( -157.4685091425930636, -189.7472609257535510, -59.13814366165043168 ) ) ;
#30793=CARTESIAN_POINT ( 'NONE',  ( 75.95066919219054569, -193.5000000000000000, -11.92584929509534852 ) ) ;
#30795=FACE_OUTER_BOUND ( 'NONE', #51820, .T. ) ;
#30799=CARTESIAN_POINT ( 'NONE',  ( 75.17589904515342880, -189.7472609257535510, -18.28755301364250840 ) ) ;
#30802=ADVANCED_FACE ( 'NONE', ( #11171 ), #22230, .T. ) ;
#30803=AXIS2_PLACEMENT_3D ( 'NONE', #47997, #11979, #40605 ) ;
#30804=ORIENTED_EDGE ( 'NONE', *, *, #27851, .T. ) ;
#30805=CARTESIAN_POINT ( 'NONE',  ( -7.223120065443615623, -193.5000000000000000, 117.9955164924470523 ) ) ;
#30807=CARTESIAN_POINT ( 'NONE',  ( 32.49319223169170812, -189.7472609257535510, -95.22858582633060109 ) ) ;
#30808=EDGE_LOOP ( 'NONE', ( #1665, #38608, #48495, #14151 ) ) ;
#30809=DIRECTION ( 'NONE',  ( 0.000000000000000000, -0.000000000000000000, 1.000000000000000000 ) ) ;
#30810=VECTOR ( 'NONE', #15591, 1000.000000000000000 ) ;
#30811=DIRECTION ( 'NONE',  ( -0.1768902751225592818, 0.000000000000000000, -0.9842305779475992722 ) ) ;
#30813=EDGE_CURVE ( 'NONE', #3759, #41311, #39297, .T. ) ;
#30819=ORIENTED_EDGE ( 'NONE', *, *, #5692, .T. ) ;
#30821=ORIENTED_EDGE ( 'NONE', *, *, #9188, .T. ) ;
#30824=VECTOR ( 'NONE', #26906, 999.9999999999998863 ) ;
#30826=EDGE_LOOP ( 'NONE', ( #45522, #52023, #39590, #41862 ) ) ;
#30827=AXIS2_PLACEMENT_3D ( 'NONE', #7789, #35911, #3073 ) ;
#30828=DIRECTION ( 'NONE',  ( 0.000000000000000000, 1.000000000000000000, 0.000000000000000000 ) ) ;
#30830=DIRECTION ( 'NONE',  ( 0.4566292373937077542, 0.000000000000000000, 0.8896570909947499883 ) ) ;
#30831=AXIS2_PLACEMENT_3D ( 'NONE', #327, #1379, #16374 ) ;
#30832=EDGE_CURVE ( 'NONE', #1307, #10059, #15655, .T. ) ;
#30834=LINE ( 'NONE', #5646, #46385 ) ;
#30835=AXIS2_PLACEMENT_3D ( 'NONE', #2429, #42872, #35240 ) ;
#30836=EDGE_CURVE ( 'NONE', #51603, #14259, #21006, .T. ) ;
#30837=CARTESIAN_POINT ( 'NONE',  ( -48.47912675150885065, -188.5000000000000284, 6.938893903907228378E-15 ) ) ;
#30838=DIRECTION ( 'NONE',  ( -0.000000000000000000, 1.000000000000000000, -0.000000000000000000 ) ) ;
#30841=EDGE_CURVE ( 'NONE', #30907, #13637, #27719, .T. ) ;
#30842=ORIENTED_EDGE ( 'NONE', *, *, #27851, .F. ) ;
#30843=CARTESIAN_POINT ( 'NONE',  ( 61.38599058177057799, -175.3837268820161057, 59.62093586438192006 ) ) ;
#30844=EDGE_CURVE ( 'NONE', #41127, #27780, #3810, .T. ) ;
#30845=LINE ( 'NONE', #46892, #7818 ) ;
#30846=VECTOR ( 'NONE', #2244, 1000.000000000000114 ) ;
#30847=VECTOR ( 'NONE', #10768, 1000.000000000000000 ) ;
#30848=VERTEX_POINT ( 'NONE', #48226 ) ;
#30849=LINE ( 'NONE', #6931, #49971 ) ;
#30850=ORIENTED_EDGE ( 'NONE', *, *, #35555, .F. ) ;
#30852=CARTESIAN_POINT ( 'NONE',  ( -48.47912675150885065, -183.6283474603465606, 6.938893903907228378E-15 ) ) ;
#30853=AXIS2_PLACEMENT_3D ( 'NONE', #24834, #3830, #8026 ) ;
#30854=DIRECTION ( 'NONE',  ( 0.000000000000000000, 0.000000000000000000, 1.000000000000000000 ) ) ;
#30855=PLANE ( 'NONE',  #39997 ) ;
#30856=ORIENTED_EDGE ( 'NONE', *, *, #17844, .T. ) ;
#30857=EDGE_LOOP ( 'NONE', ( #22078, #47905, #28459, #44087 ) ) ;
#30858=VERTEX_POINT ( 'NONE', #44283 ) ;
#30860=PLANE ( 'NONE',  #21606 ) ;
#30861=CARTESIAN_POINT ( 'NONE',  ( -47.66663987350317910, -177.1207230881787780, 0.5829794791144832233 ) ) ;
#30862=CIRCLE ( 'NONE', #19937, 125.0000000000000000 ) ;
#30863=CARTESIAN_POINT ( 'NONE',  ( -98.10897907742933910, -193.5000000000000000, 114.7252272087849434 ) ) ;
#30865=DIRECTION ( 'NONE',  ( 0.000000000000000000, 1.000000000000000000, 0.000000000000000000 ) ) ;
#30866=LINE ( 'NONE', #14072, #35619 ) ;
#30867=ORIENTED_EDGE ( 'NONE', *, *, #989, .F. ) ;
#30868=FACE_OUTER_BOUND ( 'NONE', #30826, .T. ) ;
#30869=CARTESIAN_POINT ( 'NONE',  ( -166.1003692892502102, -193.5000000000000000, -42.31126686685032467 ) ) ;
#30870=VECTOR ( 'NONE', #40403, 1000.000000000000000 ) ;
#30873=CARTESIAN_POINT ( 'NONE',  ( -238.7407812814481076, -193.5000000000000000, 41.45482488023466772 ) ) ;
#30874=DIRECTION ( 'NONE',  ( 0.000000000000000000, -1.000000000000000000, 0.000000000000000000 ) ) ;
#30875=CARTESIAN_POINT ( 'NONE',  ( 48.47907891923915003, -189.7472609257535510, 78.89300572996904748 ) ) ;
#30877=LINE ( 'NONE', #19055, #36301 ) ;
#30879=DIRECTION ( 'NONE',  ( -0.000000000000000000, 1.000000000000000000, -0.000000000000000000 ) ) ;
#30881=VERTEX_POINT ( 'NONE', #24306 ) ;
#30882=FACE_OUTER_BOUND ( 'NONE', #34628, .T. ) ;
#30883=ORIENTED_EDGE ( 'NONE', *, *, #43217, .T. ) ;
#30884=LINE ( 'NONE', #49833, #27915 ) ;
#30886=VECTOR ( 'NONE', #41405, 1000.000000000000000 ) ;
#30888=ORIENTED_EDGE ( 'NONE', *, *, #7626, .F. ) ;
#30889=AXIS2_PLACEMENT_3D ( 'NONE', #45530, #45019, #5595 ) ;
#30890=DIRECTION ( 'NONE',  ( -0.5085311186492273983, 0.000000000000000000, 0.8610436117673514467 ) ) ;
#30891=PLANE ( 'NONE',  #13832 ) ;
#30897=EDGE_CURVE ( 'NONE', #45491, #49617, #40572, .T. ) ;
#30898=DIRECTION ( 'NONE',  ( 0.000000000000000000, -0.000000000000000000, 1.000000000000000000 ) ) ;
#30899=FACE_OUTER_BOUND ( 'NONE', #38084, .T. ) ;
#30900=EDGE_LOOP ( 'NONE', ( #1716, #34184, #18963, #24745 ) ) ;
#30902=CARTESIAN_POINT ( 'NONE',  ( 41.41233698655026529, -177.1207230881787780, 86.85922373029363541 ) ) ;
#30903=ORIENTED_EDGE ( 'NONE', *, *, #12656, .F. ) ;
#30905=AXIS2_PLACEMENT_3D ( 'NONE', #25193, #8116, #40948 ) ;
#30907=VERTEX_POINT ( 'NONE', #4587 ) ;
#30910=VERTEX_POINT ( 'NONE', #36381 ) ;
#30911=PLANE ( 'NONE',  #22427 ) ;
#30913=DIRECTION ( 'NONE',  ( 0.8896570909947499883, 0.000000000000000000, -0.4566292373937077542 ) ) ;
#30914=ORIENTED_EDGE ( 'NONE', *, *, #33781, .T. ) ;
#30915=ORIENTED_EDGE ( 'NONE', *, *, #42927, .T. ) ;
#30916=ORIENTED_EDGE ( 'NONE', *, *, #50645, .F. ) ;
#30917=DIRECTION ( 'NONE',  ( -0.000000000000000000, 1.000000000000000000, -0.000000000000000000 ) ) ;
#30920=AXIS2_PLACEMENT_3D ( 'NONE', #8149, #24188, #12601 ) ;
#30921=FACE_OUTER_BOUND ( 'NONE', #39792, .T. ) ;
#30925=VECTOR ( 'NONE', #23164, 1000.000000000000000 ) ;
#30926=CARTESIAN_POINT ( 'NONE',  ( -170.7514454179067798, -193.5000000000000000, -20.63201007055400282 ) ) ;
#30927=ORIENTED_EDGE ( 'NONE', *, *, #35320, .F. ) ;
#30928=CARTESIAN_POINT ( 'NONE',  ( -37.78865854180983774, -193.5000000000000000, -123.5388265266451242 ) ) ;
#30930=VECTOR ( 'NONE', #12555, 1000.000000000000227 ) ;
#30931=ORIENTED_EDGE ( 'NONE', *, *, #47380, .T. ) ;
#30932=CARTESIAN_POINT ( 'NONE',  ( -137.9639882952644143, -177.1207230881787780, 87.27805883780241913 ) ) ;
#30935=ADVANCED_FACE ( 'NONE', ( #8012 ), #32184, .T. ) ;
#30936=CARTESIAN_POINT ( 'NONE',  ( -124.9871112439422092, -189.7472609257535510, -98.85104101073275729 ) ) ;
#30937=ORIENTED_EDGE ( 'NONE', *, *, #34012, .F. ) ;
#30938=CARTESIAN_POINT ( 'NONE',  ( -47.48307690889363641, -177.1207230881787780, -0.08879589532292464504 ) ) ;
#30939=ORIENTED_EDGE ( 'NONE', *, *, #39163, .T. ) ;
#30940=AXIS2_PLACEMENT_3D ( 'NONE', #10961, #15439, #43790 ) ;
#30941=ORIENTED_EDGE ( 'NONE', *, *, #46397, .F. ) ;
#30943=CARTESIAN_POINT ( 'NONE',  ( -105.8382074681672975, -175.3837268820161057, -109.9360785596604728 ) ) ;
#30945=VERTEX_POINT ( 'NONE', #656 ) ;
#30946=CARTESIAN_POINT ( 'NONE',  ( -164.3791542526839180, -193.5000000000000000, 46.82076062204521349 ) ) ;
#30947=DIRECTION ( 'NONE',  ( 0.000000000000000000, 0.000000000000000000, 1.000000000000000000 ) ) ;
#30948=CARTESIAN_POINT ( 'NONE',  ( -5.142695285147754980, -193.5000000000000000, -116.1806952091177578 ) ) ;
#30949=CARTESIAN_POINT ( 'NONE',  ( 12.99855592850622799, -183.6283474603465606, 108.8370090194295017 ) ) ;
#30950=ORIENTED_EDGE ( 'NONE', *, *, #18302, .T. ) ;
#30951=CARTESIAN_POINT ( 'NONE',  ( -11.47118876952529121, -193.5000000000000000, 118.3487137068149053 ) ) ;
#30952=PLANE ( 'NONE',  #8075 ) ;
#30953=LINE ( 'NONE', #30429, #31602 ) ;
#30955=ORIENTED_EDGE ( 'NONE', *, *, #12613, .T. ) ;
#30957=AXIS2_PLACEMENT_3D ( 'NONE', #991, #17565, #1244 ) ;
#30959=LINE ( 'NONE', #47002, #2940 ) ;
#30962=ORIENTED_EDGE ( 'NONE', *, *, #20503, .T. ) ;
#30963=LINE ( 'NONE', #18866, #48937 ) ;
#30964=EDGE_LOOP ( 'NONE', ( #36981, #51050, #34490, #41930 ) ) ;
#30966=PLANE ( 'NONE',  #36846 ) ;
#30967=FACE_BOUND ( 'NONE', #16164, .T. ) ;
#30968=CARTESIAN_POINT ( 'NONE',  ( -170.6250538923603131, -193.5000000000000000, 26.55884942729649723 ) ) ;
#30969=CARTESIAN_POINT ( 'NONE',  ( -169.0136227435421006, -175.3837268820161057, -33.11246405730812370 ) ) ;
#30971=CIRCLE ( 'NONE', #1651, 125.0000000000000000 ) ;
#30973=FACE_OUTER_BOUND ( 'NONE', #9714, .T. ) ;
#30974=VERTEX_POINT ( 'NONE', #28489 ) ;
#30975=CYLINDRICAL_SURFACE ( 'NONE', #20884, 125.0000000000000000 ) ;
#30976=EDGE_CURVE ( 'NONE', #39640, #17102, #44536, .T. ) ;
#30977=EDGE_CURVE ( 'NONE', #48594, #4839, #40256, .T. ) ;
#30978=PLANE ( 'NONE',  #9134 ) ;
#30981=FACE_OUTER_BOUND ( 'NONE', #23842, .T. ) ;
#30982=CARTESIAN_POINT ( 'NONE',  ( -25.55153130240594450, -175.3837268820161057, 122.8793122007210599 ) ) ;
#30983=ORIENTED_EDGE ( 'NONE', *, *, #2080, .T. ) ;
#30985=CARTESIAN_POINT ( 'NONE',  ( -138.3705904895685705, -193.5000000000000000, -86.85922373029296750 ) ) ;
#30986=ORIENTED_EDGE ( 'NONE', *, *, #16324, .T. ) ;
#30987=CARTESIAN_POINT ( 'NONE',  ( 52.98246549829696761, -175.3837268820161057, 73.01058346660533971 ) ) ;
#30988=AXIS2_PLACEMENT_3D ( 'NONE', #36676, #20640, #4890 ) ;
#30989=ORIENTED_EDGE ( 'NONE', *, *, #8869, .F. ) ;
#30991=DIRECTION ( 'NONE',  ( 0.000000000000000000, 0.000000000000000000, 1.000000000000000000 ) ) ;
#30992=ORIENTED_EDGE ( 'NONE', *, *, #32595, .F. ) ;
#30993=CARTESIAN_POINT ( 'NONE',  ( -48.47912675150885065, -175.3837268820161057, 6.938893903907228378E-15 ) ) ;
#30994=CARTESIAN_POINT ( 'NONE',  ( -84.19171550243319757, -175.3837268820161057, 119.7898618611247628 ) ) ;
#30995=ORIENTED_EDGE ( 'NONE', *, *, #27606, .T. ) ;
#30996=ORIENTED_EDGE ( 'NONE', *, *, #9880, .T. ) ;
#30997=EDGE_CURVE ( 'NONE', #11130, #49730, #17481, .T. ) ;
#30998=CARTESIAN_POINT ( 'NONE',  ( 49.27559354810669134, -193.5000000000000000, -76.29032973288636299 ) ) ;
#30999=ORIENTED_EDGE ( 'NONE', *, *, #661, .T. ) ;
#31001=EDGE_CURVE ( 'NONE', #28894, #18907, #25098, .T. ) ;
#31002=CARTESIAN_POINT ( 'NONE',  ( 21.21056010634072564, -193.5000000000000000, 103.7706487676302061 ) ) ;
#31003=ORIENTED_EDGE ( 'NONE', *, *, #48755, .T. ) ;
#31004=CARTESIAN_POINT ( 'NONE',  ( -172.4422607493951602, -183.6283474603465606, 16.06677968424543934 ) ) ;
#31007=PLANE ( 'NONE',  #5585 ) ;
#31009=DIRECTION ( 'NONE',  ( 0.000000000000000000, 0.000000000000000000, -1.000000000000000000 ) ) ;
#31010=DIRECTION ( 'NONE',  ( -0.8757349421956310831, 0.000000000000000000, -0.4827922027307550712 ) ) ;
#31011=AXIS2_PLACEMENT_3D ( 'NONE', #37977, #5687, #41661 ) ;
#31012=CARTESIAN_POINT ( 'NONE',  ( 71.09073365861578964, -175.3837268820161057, 32.84887689123991095 ) ) ;
#31014=DIRECTION ( 'NONE',  ( 0.000000000000000000, 0.000000000000000000, -1.000000000000000000 ) ) ;
#31015=CARTESIAN_POINT ( 'NONE',  ( -118.1688136093591908, -175.3837268820161057, -103.7706487676296661 ) ) ;
#31017=LINE ( 'NONE', #23643, #45397 ) ;
#31018=CARTESIAN_POINT ( 'NONE',  ( -49.42645310536304493, -193.5000000000000000, 0.3202698538628349079 ) ) ;
#31019=EDGE_LOOP ( 'NONE', ( #30480, #983, #19700, #1028 ) ) ;
#31021=LINE ( 'NONE', #6859, #27383 ) ;
#31023=DIRECTION ( 'NONE',  ( 0.1768902751225733261, 0.000000000000000000, -0.9842305779475966077 ) ) ;
#31024=PLANE ( 'NONE',  #42177 ) ;
#31025=DIRECTION ( 'NONE',  ( 0.000000000000000000, 1.000000000000000000, -0.000000000000000000 ) ) ;
#31027=DIRECTION ( 'NONE',  ( -0.000000000000000000, 1.000000000000000000, 0.000000000000000000 ) ) ;
#31028=CARTESIAN_POINT ( 'NONE',  ( 0.7476021451244497795, -175.3837268820161057, -113.8100815915415609 ) ) ;
#31029=ORIENTED_EDGE ( 'NONE', *, *, #24697, .F. ) ;
#31034=ADVANCED_FACE ( 'NONE', ( #37160 ), #13775, .T. ) ;
#31036=ORIENTED_EDGE ( 'NONE', *, *, #27417, .F. ) ;
#31037=VECTOR ( 'NONE', #21996, 1000.000000000000000 ) ;
#31038=VECTOR ( 'NONE', #33742, 1000.000000000000000 ) ;
#31041=DIRECTION ( 'NONE',  ( -0.000000000000000000, 1.000000000000000000, -0.000000000000000000 ) ) ;
#31042=CARTESIAN_POINT ( 'NONE',  ( -18.31235070009513421, -175.3837268820161057, 121.3052580173829966 ) ) ;
#31043=EDGE_LOOP ( 'NONE', ( #16718, #41781, #44427, #37039 ) ) ;
#31045=PLANE ( 'NONE',  #8798 ) ;
#31046=VERTEX_POINT ( 'NONE', #5380 ) ;
#31049=LINE ( 'NONE', #14786, #1416 ) ;
#31050=EDGE_CURVE ( 'NONE', #22956, #47477, #31156, .T. ) ;
#31052=DIRECTION ( 'NONE',  ( 0.1768902751225733261, 0.000000000000000000, -0.9842305779475966077 ) ) ;
#31054=VERTEX_POINT ( 'NONE', #50043 ) ;
#31058=CARTESIAN_POINT ( 'NONE',  ( -155.9608607592036833, -177.1207230881787780, 63.81752780153064464 ) ) ;
#31059=EDGE_CURVE ( 'NONE', #36633, #51798, #6719, .T. ) ;
#31060=DIRECTION ( 'NONE',  ( -0.000000000000000000, 1.000000000000000000, -0.000000000000000000 ) ) ;
#31061=VECTOR ( 'NONE', #514, 1000.000000000000000 ) ;
#31062=EDGE_LOOP ( 'NONE', ( #23583, #46565, #5185, #39888 ) ) ;
#31064=CARTESIAN_POINT ( 'NONE',  ( -84.19171550243321178, -189.7472609257535510, 119.7898618611247485 ) ) ;
#31067=LINE ( 'NONE', #27116, #20033 ) ;
#31068=DIRECTION ( 'NONE',  ( -0.000000000000000000, 1.000000000000000000, -0.000000000000000000 ) ) ;
#31071=ORIENTED_EDGE ( 'NONE', *, *, #51034, .F. ) ;
#31072=CARTESIAN_POINT ( 'NONE',  ( -18.95304271317703382, -189.7472609257535510, -121.4627941443854837 ) ) ;
#31073=CARTESIAN_POINT ( 'NONE',  ( -47.47956591500005885, -183.6283474603465606, -0.02963332782254939762 ) ) ;
#31074=EDGE_LOOP ( 'NONE', ( #23158, #17466, #36328, #24287 ) ) ;
#31075=CARTESIAN_POINT ( 'NONE',  ( 74.60098876342242136, -193.5000000000000000, 21.82395850507348811 ) ) ;
#31078=AXIS2_PLACEMENT_3D ( 'NONE', #30861, #26905, #30333 ) ;
#31079=AXIS2_PLACEMENT_3D ( 'NONE', #23963, #39980, #4008 ) ;
#31080=CARTESIAN_POINT ( 'NONE',  ( -48.47912675150885065, -183.6283474603465606, 6.938893903907228378E-15 ) ) ;
#31081=EDGE_CURVE ( 'NONE', #48517, #29101, #32953, .T. ) ;
#31084=CARTESIAN_POINT ( 'NONE',  ( 76.31829002442924548, -177.1207230881787780, 7.113702696402421033 ) ) ;
#31085=ORIENTED_EDGE ( 'NONE', *, *, #34593, .T. ) ;
#31086=ORIENTED_EDGE ( 'NONE', *, *, #23696, .T. ) ;
#31087=LINE ( 'NONE', #47134, #39171 ) ;
#31088=EDGE_CURVE ( 'NONE', #12031, #18822, #14043, .T. ) ;
#31089=PLANE ( 'NONE',  #31295 ) ;
#31090=ORIENTED_EDGE ( 'NONE', *, *, #34380, .F. ) ;
#31091=ORIENTED_EDGE ( 'NONE', *, *, #43461, .T. ) ;
#31093=CARTESIAN_POINT ( 'NONE',  ( -48.18706998087188254, -183.6283474603465606, 0.9564009842765313074 ) ) ;
#31095=DIRECTION ( 'NONE',  ( 0.000000000000000000, -1.000000000000000000, 0.000000000000000000 ) ) ;
#31096=FACE_OUTER_BOUND ( 'NONE', #22466, .T. ) ;
#31099=EDGE_CURVE ( 'NONE', #14253, #32264, #49538, .T. ) ;
#31100=EDGE_CURVE ( 'NONE', #31730, #23257, #41110, .T. ) ;
#31104=ORIENTED_EDGE ( 'NONE', *, *, #23750, .T. ) ;
#31105=EDGE_CURVE ( 'NONE', #16426, #18623, #5906, .T. ) ;
#31106=ORIENTED_EDGE ( 'NONE', *, *, #48461, .T. ) ;
#31108=CARTESIAN_POINT ( 'NONE',  ( 55.03325008324586776, -193.5000000000000000, -70.07273251429357686 ) ) ;
#31110=EDGE_CURVE ( 'NONE', #3616, #10162, #45074, .T. ) ;
#31111=PLANE ( 'NONE',  #45518 ) ;
#31113=ORIENTED_EDGE ( 'NONE', *, *, #20996, .F. ) ;
#31114=AXIS2_PLACEMENT_3D ( 'NONE', #6147, #25575, #5894 ) ;
#31115=EDGE_CURVE ( 'NONE', #38032, #39795, #6921, .T. ) ;
#31117=FACE_OUTER_BOUND ( 'NONE', #22949, .T. ) ;
#31118=EDGE_CURVE ( 'NONE', #28891, #150, #22953, .T. ) ;
#31119=VECTOR ( 'NONE', #48086, 1000.000000000000227 ) ;
#31121=ORIENTED_EDGE ( 'NONE', *, *, #51246, .T. ) ;
#31123=DIRECTION ( 'NONE',  ( 0.3482016354343866471, 0.000000000000000000, 0.9374196611341253371 ) ) ;
#31124=EDGE_CURVE ( 'NONE', #4082, #38866, #5903, .T. ) ;
#31125=CARTESIAN_POINT ( 'NONE',  ( -60.86541030502395699, -183.6283474603465606, -124.3848060646151481 ) ) ;
#31129=CARTESIAN_POINT ( 'NONE',  ( -173.4787860028527007, -193.5000000000000000, 0.2918682030023981300 ) ) ;
#31130=ORIENTED_EDGE ( 'NONE', *, *, #48451, .T. ) ;
#31131=DIRECTION ( 'NONE',  ( 0.000000000000000000, 1.000000000000000000, 0.000000000000000000 ) ) ;
#31135=VECTOR ( 'NONE', #42746, 1000.000000000000000 ) ;
#31136=DIRECTION ( 'NONE',  ( -0.4566292373937077542, 0.000000000000000000, -0.8896570909947499883 ) ) ;
#31137=EDGE_LOOP ( 'NONE', ( #36494, #4540, #13468, #5610 ) ) ;
#31138=DIRECTION ( 'NONE',  ( 0.000000000000000000, -0.000000000000000000, -1.000000000000000000 ) ) ;
#31139=DIRECTION ( 'NONE',  ( 0.000000000000000000, 1.000000000000000000, 0.000000000000000000 ) ) ;
#31140=CARTESIAN_POINT ( 'NONE',  ( -48.02249751411514467, -183.6283474603465606, 0.8896570909947569827 ) ) ;
#31145=ORIENTED_EDGE ( 'NONE', *, *, #25536, .F. ) ;
#31146=PLANE ( 'NONE',  #30232 ) ;
#31147=DIRECTION ( 'NONE',  ( -0.000000000000000000, 1.000000000000000000, -0.000000000000000000 ) ) ;
#31150=VERTEX_POINT ( 'NONE', #10863 ) ;
#31151=DIRECTION ( 'NONE',  ( -0.000000000000000000, 1.000000000000000000, -0.000000000000000000 ) ) ;
#31152=ORIENTED_EDGE ( 'NONE', *, *, #18548, .T. ) ;
#31153=CIRCLE ( 'NONE', #8490, 10.00000000000000178 ) ;
#31156=CIRCLE ( 'NONE', #846, 125.0000000000000000 ) ;
#31158=CARTESIAN_POINT ( 'NONE',  ( -48.47912675150885065, -189.7472609257535510, 6.938893903907228378E-15 ) ) ;
#31159=ORIENTED_EDGE ( 'NONE', *, *, #16714, .T. ) ;
#31161=EDGE_CURVE ( 'NONE', #38778, #18675, #42665, .T. ) ;
#31162=EDGE_CURVE ( 'NONE', #47705, #30169, #46617, .T. ) ;
#31163=DIRECTION ( 'NONE',  ( -0.000000000000000000, 1.000000000000000000, -0.000000000000000000 ) ) ;
#31165=ORIENTED_EDGE ( 'NONE', *, *, #36257, .T. ) ;
#31166=ORIENTED_EDGE ( 'NONE', *, *, #3467, .F. ) ;
#31168=ORIENTED_EDGE ( 'NONE', *, *, #32365, .F. ) ;
#31169=ADVANCED_FACE ( 'NONE', ( #10092 ), #22444, .T. ) ;
#31171=FACE_OUTER_BOUND ( 'NONE', #12423, .T. ) ;
#31174=CARTESIAN_POINT ( 'NONE',  ( -167.6453766917639427, -193.5000000000000000, 37.74128873232411507 ) ) ;
#31176=ORIENTED_EDGE ( 'NONE', *, *, #9075, .T. ) ;
#31177=CARTESIAN_POINT ( 'NONE',  ( 9.336583202542589888, -175.3837268820161057, 110.8257356506556306 ) ) ;
#31179=DIRECTION ( 'NONE',  ( 0.000000000000000000, -1.000000000000000000, -0.000000000000000000 ) ) ;
#31180=ORIENTED_EDGE ( 'NONE', *, *, #25675, .T. ) ;
#31182=ORIENTED_EDGE ( 'NONE', *, *, #29590, .F. ) ;
#31183=DIRECTION ( 'NONE',  ( 0.000000000000000000, -1.000000000000000000, 0.000000000000000000 ) ) ;
#31185=FACE_OUTER_BOUND ( 'NONE', #8659, .T. ) ;
#31186=CIRCLE ( 'NONE', #26120, 125.0000000000000000 ) ;
#31187=LINE ( 'NONE', #47238, #17940 ) ;
#31188=CARTESIAN_POINT ( 'NONE',  ( 57.66105628977221897, -189.7472609257535510, 66.02470404298190942 ) ) ;
#31191=AXIS2_PLACEMENT_3D ( 'NONE', #14344, #30355, #21962 ) ;
#31193=EDGE_CURVE ( 'NONE', #16796, #28863, #32737, .T. ) ;
#31194=VECTOR ( 'NONE', #39988, 1000.000000000000000 ) ;
#31196=CARTESIAN_POINT ( 'NONE',  ( -48.30223647638627682, -175.3837268820161057, -0.9842305779475897243 ) ) ;
#31197=DIRECTION ( 'NONE',  ( -0.9960498426152171181, 0.000000000000000000, 0.08879589532293157006 ) ) ;
#31199=LINE ( 'NONE', #39342, #50071 ) ;
#31200=DIRECTION ( 'NONE',  ( 0.000000000000000000, 1.000000000000000000, 0.000000000000000000 ) ) ;
#31201=LINE ( 'NONE', #10722, #49022 ) ;
#31202=CARTESIAN_POINT ( 'NONE',  ( -49.17567778057184569, -193.5000000000000000, -0.7175072570443327136 ) ) ;
#31203=VERTEX_POINT ( 'NONE', #46885 ) ;
#31204=FACE_OUTER_BOUND ( 'NONE', #12578, .T. ) ;
#31205=CARTESIAN_POINT ( 'NONE',  ( -156.7610986364826999, -177.1207230881787780, -62.45009659481510766 ) ) ;
#31206=AXIS2_PLACEMENT_3D ( 'NONE', #2713, #47128, #18751 ) ;
#31207=FACE_OUTER_BOUND ( 'NONE', #30350, .T. ) ;
#31208=EDGE_LOOP ( 'NONE', ( #29093, #9543, #39870, #5948 ) ) ;
#31209=AXIS2_PLACEMENT_3D ( 'NONE', #14251, #46316, #47083 ) ;
#31211=DIRECTION ( 'NONE',  ( -0.9646355819083614058, 0.000000000000000000, 0.2635871660690581320 ) ) ;
#31212=ORIENTED_EDGE ( 'NONE', *, *, #5692, .F. ) ;
#31216=FACE_BOUND ( 'NONE', #48644, .T. ) ;
#31217=DIRECTION ( 'NONE',  ( 0.000000000000000000, 1.000000000000000000, 0.000000000000000000 ) ) ;
#31218=ORIENTED_EDGE ( 'NONE', *, *, #41475, .T. ) ;
#31219=VECTOR ( 'NONE', #48132, 1000.000000000000114 ) ;
#31220=EDGE_CURVE ( 'NONE', #38204, #16314, #3246, .T. ) ;
#31222=CARTESIAN_POINT ( 'NONE',  ( 43.57032560458359427, -189.7472609257535510, 83.08371579725745448 ) ) ;
#31223=EDGE_LOOP ( 'NONE', ( #20825, #48173, #41755, #29661 ) ) ;
#31225=EDGE_LOOP ( 'NONE', ( #8549, #16009, #34107, #4698 ) ) ;
#31228=CARTESIAN_POINT ( 'NONE',  ( -167.1580984288390823, -193.5000000000000000, -39.24667733211878584 ) ) ;
#31229=AXIS2_PLACEMENT_3D ( 'NONE', #41555, #49722, #13456 ) ;
#31231=PLANE ( 'NONE',  #43529 ) ;
#31232=FACE_OUTER_BOUND ( 'NONE', #10002, .T. ) ;
#31233=ORIENTED_EDGE ( 'NONE', *, *, #32087, .T. ) ;
#31234=DIRECTION ( 'NONE',  ( 0.000000000000000000, -0.000000000000000000, -1.000000000000000000 ) ) ;
#31235=CARTESIAN_POINT ( 'NONE',  ( 26.10278175629141018, -175.3837268820161057, -99.06333546307678262 ) ) ;
#31236=ORIENTED_EDGE ( 'NONE', *, *, #25234, .T. ) ;
#31237=VECTOR ( 'NONE', #21345, 1000.000000000000000 ) ;
#31240=DIRECTION ( 'NONE',  ( -0.000000000000000000, 1.000000000000000000, -0.000000000000000000 ) ) ;
#31242=DIRECTION ( 'NONE',  ( -0.7948544414133608127, 0.000000000000000000, 0.6068001458185834363 ) ) ;
#31243=EDGE_LOOP ( 'NONE', ( #31507, #29696, #29414, #27043 ) ) ;
#31244=CARTESIAN_POINT ( 'NONE',  ( -47.47956591500005885, -193.5000000000000000, -0.02963332782254939762 ) ) ;
#31245=ORIENTED_EDGE ( 'NONE', *, *, #35913, .F. ) ;
#31246=LINE ( 'NONE', #27302, #19873 ) ;
#31248=EDGE_LOOP ( 'NONE', ( #12147, #47935, #51287, #49643 ) ) ;
#31252=DIRECTION ( 'NONE',  ( -0.5586467658036476935, 0.000000000000000000, -0.8294056854502049880 ) ) ;
#31253=ORIENTED_EDGE ( 'NONE', *, *, #16775, .F. ) ;
#31255=DIRECTION ( 'NONE',  ( 0.000000000000000000, 1.000000000000000000, -0.000000000000000000 ) ) ;
#31256=CARTESIAN_POINT ( 'NONE',  ( -62.43888699632653072, -175.3837268820161057, 124.2180546213279229 ) ) ;
#31257=AXIS2_PLACEMENT_3D ( 'NONE', #5494, #24936, #37015 ) ;
#31260=EDGE_CURVE ( 'NONE', #47114, #5997, #40656, .T. ) ;
#31261=CARTESIAN_POINT ( 'NONE',  ( -89.44307666693796932, -193.5000000000000000, -117.0391155081702266 ) ) ;
#31262=CARTESIAN_POINT ( 'NONE',  ( -2.174401709722246334, -193.5000000000000000, -115.0304316645280096 ) ) ;
#31263=VECTOR ( 'NONE', #45459, 1000.000000000000000 ) ;
#31264=CARTESIAN_POINT ( 'NONE',  ( 66.42899531795131907, -183.6283474603465606, 49.20491319441622124 ) ) ;
#31266=EDGE_CURVE ( 'NONE', #34274, #15102, #6159, .T. ) ;
#31267=DIRECTION ( 'NONE',  ( 0.000000000000000000, -1.000000000000000000, -0.000000000000000000 ) ) ;
#31269=FACE_OUTER_BOUND ( 'NONE', #37496, .T. ) ;
#31270=LINE ( 'NONE', #22365, #29111 ) ;
#31271=ORIENTED_EDGE ( 'NONE', *, *, #3441, .T. ) ;
#31275=CIRCLE ( 'NONE', #8620, 125.0000000000000000 ) ;
#31278=DIRECTION ( 'NONE',  ( 0.5085311186492154079, 0.000000000000000000, 0.8610436117673585521 ) ) ;
#31279=CARTESIAN_POINT ( 'NONE',  ( -48.47912675150885065, -177.1207230881787780, 1.000000000000006883 ) ) ;
#31280=DIRECTION ( 'NONE',  ( -0.9960498426152177842, 0.000000000000000000, 0.08879589532292482545 ) ) ;
#31282=ORIENTED_EDGE ( 'NONE', *, *, #44871, .T. ) ;
#31284=AXIS2_PLACEMENT_3D ( 'NONE', #25733, #30196, #9705 ) ;
#31286=EDGE_CURVE ( 'NONE', #29888, #32182, #7693, .T. ) ;
#31287=ORIENTED_EDGE ( 'NONE', *, *, #35692, .F. ) ;
#31289=ADVANCED_FACE ( 'NONE', ( #48422 ), #20037, .T. ) ;
#31290=VERTEX_POINT ( 'NONE', #35531 ) ;
#31291=CARTESIAN_POINT ( 'NONE',  ( 34.23904069044534992, -183.6283474603465606, -92.37913469314065651 ) ) ;
#31293=CYLINDRICAL_SURFACE ( 'NONE', #50477, 125.0000000000000000 ) ;
#31294=ORIENTED_EDGE ( 'NONE', *, *, #1355, .T. ) ;
#31295=AXIS2_PLACEMENT_3D ( 'NONE', #35043, #38967, #34272 ) ;
#31299=LINE ( 'NONE', #22910, #40904 ) ;
#31300=ORIENTED_EDGE ( 'NONE', *, *, #44958, .T. ) ;
#31301=EDGE_CURVE ( 'NONE', #43088, #30974, #15585, .T. ) ;
#31303=ORIENTED_EDGE ( 'NONE', *, *, #42980, .T. ) ;
#31304=DIRECTION ( 'NONE',  ( 0.000000000000000000, 0.000000000000000000, 1.000000000000000000 ) ) ;
#31305=ORIENTED_EDGE ( 'NONE', *, *, #21026, .F. ) ;
#31306=DIRECTION ( 'NONE',  ( 0.000000000000000000, 0.000000000000000000, 1.000000000000000000 ) ) ;
#31307=FACE_OUTER_BOUND ( 'NONE', #49075, .T. ) ;
#31308=CARTESIAN_POINT ( 'NONE',  ( 55.03325008324585355, -183.6283474603465606, -70.07273251429357686 ) ) ;
#31309=DIRECTION ( 'NONE',  ( 0.000000000000000000, 0.000000000000000000, 1.000000000000000000 ) ) ;
#31310=CIRCLE ( 'NONE', #38021, 125.0000000000000000 ) ;
#31312=ORIENTED_EDGE ( 'NONE', *, *, #5264, .T. ) ;
#31314=ORIENTED_EDGE ( 'NONE', *, *, #2798, .T. ) ;
#31315=AXIS2_PLACEMENT_3D ( 'NONE', #31080, #3734, #23213 ) ;
#31316=LINE ( 'NONE', #2442, #48295 ) ;
#31318=FACE_OUTER_BOUND ( 'NONE', #7539, .T. ) ;
#31320=ORIENTED_EDGE ( 'NONE', *, *, #19211, .T. ) ;
#31322=VECTOR ( 'NONE', #13575, 1000.000000000000000 ) ;
#31324=EDGE_CURVE ( 'NONE', #18133, #43502, #31865, .T. ) ;
#31325=ORIENTED_EDGE ( 'NONE', *, *, #28433, .T. ) ;
#31327=VERTEX_POINT ( 'NONE', #23716 ) ;
#31328=DIRECTION ( 'NONE',  ( 0.000000000000000000, 0.000000000000000000, -1.000000000000000000 ) ) ;
#31330=VERTEX_POINT ( 'NONE', #43694 ) ;
#31331=DIRECTION ( 'NONE',  ( 0.000000000000000000, 0.000000000000000000, 1.000000000000000000 ) ) ;
#31332=EDGE_CURVE ( 'NONE', #3078, #48105, #39831, .T. ) ;
#31333=LINE ( 'NONE', #23964, #29795 ) ;
#31335=EDGE_CURVE ( 'NONE', #18623, #52027, #51859, .T. ) ;
#31336=AXIS2_PLACEMENT_3D ( 'NONE', #26827, #42861, #34974 ) ;
#31338=CARTESIAN_POINT ( 'NONE',  ( 76.43863189440992301, -175.3837268820161057, -4.533605064403317009 ) ) ;
#31339=CARTESIAN_POINT ( 'NONE',  ( -106.4764934152196645, -213.5000000000000000, -110.7307791902283043 ) ) ;
#31341=VERTEX_POINT ( 'NONE', #3736 ) ;
#31342=ORIENTED_EDGE ( 'NONE', *, *, #49795, .T. ) ;
#31344=EDGE_CURVE ( 'NONE', #38174, #12681, #61, .T. ) ;
#31345=VECTOR ( 'NONE', #2166, 1000.000000000000000 ) ;
#31347=DIRECTION ( 'NONE',  ( 0.05924062789370748011, 0.000000000000000000, 0.9982437317643217956 ) ) ;
#31350=VECTOR ( 'NONE', #31442, 999.9999999999998863 ) ;
#31353=CARTESIAN_POINT ( 'NONE',  ( -154.0877180371535928, -193.5000000000000000, -66.87170886601927577 ) ) ;
#31354=VERTEX_POINT ( 'NONE', #36062 ) ;
#31355=CARTESIAN_POINT ( 'NONE',  ( -48.77118352214581876, -189.7472609257535510, -0.9564009842765195391 ) ) ;
#31356=DIRECTION ( 'NONE',  ( 0.000000000000000000, -1.000000000000000000, -0.000000000000000000 ) ) ;
#31357=EDGE_CURVE ( 'NONE', #48695, #37838, #16103, .T. ) ;
#31360=ORIENTED_EDGE ( 'NONE', *, *, #38759, .F. ) ;
#31361=ORIENTED_EDGE ( 'NONE', *, *, #21349, .T. ) ;
#31362=ORIENTED_EDGE ( 'NONE', *, *, #29520, .T. ) ;
#31364=CARTESIAN_POINT ( 'NONE',  ( -48.30223647638627682, -177.1207230881787780, -0.9842305779475897243 ) ) ;
#31365=CARTESIAN_POINT ( 'NONE',  ( -15.81236726369125023, -193.5000000000000000, -120.6560517527615417 ) ) ;
#31366=DIRECTION ( 'NONE',  ( -0.9890401873221633666, 0.000000000000000000, -0.1476465640024850756 ) ) ;
#31367=DIRECTION ( 'NONE',  ( 0.000000000000000000, -0.000000000000000000, 1.000000000000000000 ) ) ;
#31371=FACE_OUTER_BOUND ( 'NONE', #17689, .T. ) ;
#31372=CIRCLE ( 'NONE', #24665, 125.0000000000000000 ) ;
#31373=EDGE_LOOP ( 'NONE', ( #7877, #2014, #44553, #27406 ) ) ;
#31374=ORIENTED_EDGE ( 'NONE', *, *, #34957, .T. ) ;
#31375=LINE ( 'NONE', #27437, #34807 ) ;
#31378=CARTESIAN_POINT ( 'NONE',  ( -47.47956591500005885, -175.3837268820161057, -0.02963332782254939762 ) ) ;
#31381=ORIENTED_EDGE ( 'NONE', *, *, #12364, .T. ) ;
#31383=AXIS2_PLACEMENT_3D ( 'NONE', #22904, #27795, #40391 ) ;
#31387=DIRECTION ( 'NONE',  ( 0.000000000000000000, -1.000000000000000000, -0.000000000000000000 ) ) ;
#31388=ORIENTED_EDGE ( 'NONE', *, *, #25390, .F. ) ;
#31390=CARTESIAN_POINT ( 'NONE',  ( -125.5794209599708466, -193.5000000000000000, 97.11716833071892552 ) ) ;
#31392=DIRECTION ( 'NONE',  ( 0.4300652022765245608, 0.000000000000000000, -0.9027978299657416494 ) ) ;
#31393=CARTESIAN_POINT ( 'NONE',  ( -143.3583119192899744, -177.1207230881787780, -81.38144888055202841 ) ) ;
#31404=VECTOR ( 'NONE', #33954, 999.9999999999998863 ) ;
#31405=AXIS2_PLACEMENT_3D ( 'NONE', #35714, #19684, #11795 ) ;
#31407=LINE ( 'NONE', #124, #50084 ) ;
#31411=CARTESIAN_POINT ( 'NONE',  ( -170.2837019307126809, -193.5000000000000000, 23.23456943914129269 ) ) ;
#31413=ADVANCED_FACE ( 'NONE', ( #39648 ), #51505, .T. ) ;
#31414=CARTESIAN_POINT ( 'NONE',  ( -98.62206515315352817, -193.5000000000000000, 113.4093733337831367 ) ) ;
#31415=DIRECTION ( 'NONE',  ( 0.000000000000000000, -1.000000000000000000, 0.000000000000000000 ) ) ;
#31417=CARTESIAN_POINT ( 'NONE',  ( 26.52087324849106054, -198.5000000000000000, -70.00000000000002842 ) ) ;
#31418=ADVANCED_FACE ( 'NONE', ( #11798 ), #27824, .F. ) ;
#31420=AXIS2_PLACEMENT_3D ( 'NONE', #9600, #21693, #29307 ) ;
#31421=CARTESIAN_POINT ( 'NONE',  ( -172.2424017797220870, -177.1207230881787780, 7.666780576875857456 ) ) ;
#31422=ORIENTED_EDGE ( 'NONE', *, *, #3543, .F. ) ;
#31424=ADVANCED_FACE ( 'NONE', ( #40183 ), #23391, .T. ) ;
#31425=ORIENTED_EDGE ( 'NONE', *, *, #31741, .T. ) ;
#31426=CARTESIAN_POINT ( 'NONE',  ( -66.46933728415690723, -193.5000000000000000, 122.6885491605231522 ) ) ;
#31427=CARTESIAN_POINT ( 'NONE',  ( -28.86423599357335590, -183.6283474603465606, 122.4396006697296144 ) ) ;
#31429=CARTESIAN_POINT ( 'NONE',  ( -169.8550585387150136, -175.3837268820161057, 25.37485791684381553 ) ) ;
#31431=VERTEX_POINT ( 'NONE', #7369 ) ;
#31432=EDGE_CURVE ( 'NONE', #19489, #7086, #27583, .T. ) ;
#31433=CARTESIAN_POINT ( 'NONE',  ( -171.2727421180348415, -177.1207230881787780, 23.38221600314377113 ) ) ;
#31434=ORIENTED_EDGE ( 'NONE', *, *, #27835, .F. ) ;
#31435=CARTESIAN_POINT ( 'NONE',  ( -49.47517659412406488, -193.5000000000000000, -0.08879589532293878651 ) ) ;
#31436=ORIENTED_EDGE ( 'NONE', *, *, #5138, .F. ) ;
#31437=ORIENTED_EDGE ( 'NONE', *, *, #46239, .F. ) ;
#31439=CYLINDRICAL_SURFACE ( 'NONE', #7348, 125.0000000000000000 ) ;
#31441=VECTOR ( 'NONE', #37793, 1000.000000000000000 ) ;
#31442=DIRECTION ( 'NONE',  ( 0.2920567706369764371, 0.000000000000000000, -0.9564009842765223146 ) ) ;
#31444=ORIENTED_EDGE ( 'NONE', *, *, #22546, .F. ) ;
#31445=PLANE ( 'NONE',  #46839 ) ;
#31446=ORIENTED_EDGE ( 'NONE', *, *, #47213, .F. ) ;
#31447=VECTOR ( 'NONE', #11356, 1000.000000000000000 ) ;
#31449=ORIENTED_EDGE ( 'NONE', *, *, #39521, .T. ) ;
#31450=CARTESIAN_POINT ( 'NONE',  ( -104.3615810019516630, -175.3837268820161057, 110.6939782313525455 ) ) ;
#31451=CARTESIAN_POINT ( 'NONE',  ( -47.64924157374594671, -175.3837268820161057, 124.9972451320097377 ) ) ;
#31452=CIRCLE ( 'NONE', #51607, 124.9999999999999858 ) ;
#31454=DIRECTION ( 'NONE',  ( 0.000000000000000000, -0.000000000000000000, 1.000000000000000000 ) ) ;
#31456=ADVANCED_FACE ( 'NONE', ( #3661 ), #486, .T. ) ;
#31459=ORIENTED_EDGE ( 'NONE', *, *, #22043, .F. ) ;
#31460=AXIS2_PLACEMENT_3D ( 'NONE', #34475, #50521, #26590 ) ;
#31461=CARTESIAN_POINT ( 'NONE',  ( 70.02079272397770637, -193.5000000000000000, -36.52255268223056106 ) ) ;
#31462=DIRECTION ( 'NONE',  ( -0.000000000000000000, 1.000000000000000000, -0.000000000000000000 ) ) ;
#31463=EDGE_CURVE ( 'NONE', #11866, #34416, #15783, .T. ) ;
#31464=FACE_BOUND ( 'NONE', #37272, .T. ) ;
#31467=ORIENTED_EDGE ( 'NONE', *, *, #11762, .T. ) ;
#31470=FACE_OUTER_BOUND ( 'NONE', #17492, .T. ) ;
#31472=ADVANCED_FACE ( 'NONE', ( #39906 ), #42703, .T. ) ;
#31473=FACE_BOUND ( 'NONE', #29825, .T. ) ;
#31475=VERTEX_POINT ( 'NONE', #32286 ) ;
#31476=AXIS2_PLACEMENT_3D ( 'NONE', #3386, #31242, #44110 ) ;
#31477=VECTOR ( 'NONE', #50669, 1000.000000000000000 ) ;
#31478=ADVANCED_FACE ( 'NONE', ( #48339 ), #12323, .T. ) ;
#31480=ORIENTED_EDGE ( 'NONE', *, *, #9226, .F. ) ;
#31481=CIRCLE ( 'NONE', #14736, 125.0000000000000000 ) ;
#31483=ORIENTED_EDGE ( 'NONE', *, *, #51070, .T. ) ;
#31485=VERTEX_POINT ( 'NONE', #9687 ) ;
#31486=VECTOR ( 'NONE', #9664, 1000.000000000000227 ) ;
#31487=FACE_OUTER_BOUND ( 'NONE', #36931, .T. ) ;
#31491=LINE ( 'NONE', #23863, #24244 ) ;
#31492=CARTESIAN_POINT ( 'NONE',  ( 72.71365293123227502, -193.5000000000000000, -30.61552143554913030 ) ) ;
#31494=FACE_OUTER_BOUND ( 'NONE', #17370, .T. ) ;
#31497=DIRECTION ( 'NONE',  ( 0.000000000000000000, 1.000000000000000000, -0.000000000000000000 ) ) ;
#31498=ORIENTED_EDGE ( 'NONE', *, *, #24050, .T. ) ;
#31500=ORIENTED_EDGE ( 'NONE', *, *, #21138, .F. ) ;
#31502=ORIENTED_EDGE ( 'NONE', *, *, #18877, .T. ) ;
#31504=DIRECTION ( 'NONE',  ( -0.4566292373937018145, 0.000000000000000000, -0.8896570909947529859 ) ) ;
#31505=EDGE_LOOP ( 'NONE', ( #2367, #13467, #1957, #49861 ) ) ;
#31506=LINE ( 'NONE', #30998, #25686 ) ;
#31507=ORIENTED_EDGE ( 'NONE', *, *, #44512, .F. ) ;
#31508=PLANE ( 'NONE',  #16985 ) ;
#31511=CARTESIAN_POINT ( 'NONE',  ( -112.7586829773731267, -193.5000000000000000, -107.2060569716373379 ) ) ;
#31513=CARTESIAN_POINT ( 'NONE',  ( 2.669657140899367676, -189.7472609257535510, 114.0561348912355726 ) ) ;
#31514=VECTOR ( 'NONE', #25258, 1000.000000000000000 ) ;
#31515=CARTESIAN_POINT ( 'NONE',  ( -48.30223647638628393, -193.5000000000000000, 0.9842305779476049343 ) ) ;
#31516=AXIS2_PLACEMENT_3D ( 'NONE', #23206, #18738, #42899 ) ;
#31517=ORIENTED_EDGE ( 'NONE', *, *, #30207, .F. ) ;
#31518=EDGE_CURVE ( 'NONE', #27166, #47640, #45441, .T. ) ;
#31519=EDGE_CURVE ( 'NONE', #35003, #18053, #15515, .T. ) ;
#31522=CYLINDRICAL_SURFACE ( 'NONE', #18956, 124.9999999999999858 ) ;
#31527=AXIS2_PLACEMENT_3D ( 'NONE', #46407, #34557, #50870 ) ;
#31528=FACE_OUTER_BOUND ( 'NONE', #33312, .T. ) ;
#31530=ORIENTED_EDGE ( 'NONE', *, *, #39521, .F. ) ;
#31531=EDGE_LOOP ( 'NONE', ( #43215, #11390, #48189, #11247 ) ) ;
#31532=AXIS2_PLACEMENT_3D ( 'NONE', #51305, #3455, #28135 ) ;
#31533=ORIENTED_EDGE ( 'NONE', *, *, #38782, .T. ) ;
#31534=AXIS2_PLACEMENT_3D ( 'NONE', #16132, #24273, #20315 ) ;
#31535=LINE ( 'NONE', #19704, #36307 ) ;
#31536=LINE ( 'NONE', #23413, #39611 ) ;
#31538=CARTESIAN_POINT ( 'NONE',  ( 71.44208735029286572, -177.1207230881787780, 35.26900067126700833 ) ) ;
#31539=DIRECTION ( 'NONE',  ( 0.000000000000000000, -0.000000000000000000, -1.000000000000000000 ) ) ;
#31540=ORIENTED_EDGE ( 'NONE', *, *, #40065, .F. ) ;
#31542=EDGE_CURVE ( 'NONE', #21288, #46449, #44914, .T. ) ;
#31544=VERTEX_POINT ( 'NONE', #28605 ) ;
#31545=CIRCLE ( 'NONE', #33204, 124.9999999999999858 ) ;
#31547=ORIENTED_EDGE ( 'NONE', *, *, #15071, .T. ) ;
#31549=VECTOR ( 'NONE', #4191, 1000.000000000000000 ) ;
#31550=VECTOR ( 'NONE', #23453, 1000.000000000000000 ) ;
#31552=VERTEX_POINT ( 'NONE', #8645 ) ;
#31553=PLANE ( 'NONE',  #34262 ) ;
#31554=DIRECTION ( 'NONE',  ( -0.000000000000000000, 1.000000000000000000, -0.000000000000000000 ) ) ;
#31555=DIRECTION ( 'NONE',  ( -0.000000000000000000, 1.000000000000000000, -0.000000000000000000 ) ) ;
#31556=CARTESIAN_POINT ( 'NONE',  ( -19.28375372365793083, -189.7472609257535510, 121.5427093402341114 ) ) ;
#31557=ORIENTED_EDGE ( 'NONE', *, *, #9300, .T. ) ;
#31558=VECTOR ( 'NONE', #12107, 1000.000000000000114 ) ;
#31559=AXIS2_PLACEMENT_3D ( 'NONE', #40561, #20604, #46104 ) ;
#31560=DIRECTION ( 'NONE',  ( 0.000000000000000000, 0.000000000000000000, 1.000000000000000000 ) ) ;
#31561=VECTOR ( 'NONE', #30239, 1000.000000000000000 ) ;
#31562=VERTEX_POINT ( 'NONE', #29388 ) ;
#31563=CARTESIAN_POINT ( 'NONE',  ( -172.1341525481709880, -175.3837268820161057, 18.28755301364337527 ) ) ;
#31564=ORIENTED_EDGE ( 'NONE', *, *, #15276, .T. ) ;
#31565=DIRECTION ( 'NONE',  ( -0.1182731709213730997, 0.000000000000000000, 0.9929810960135161402 ) ) ;
#31568=FACE_OUTER_BOUND ( 'NONE', #14906, .T. ) ;
#31569=DIRECTION ( 'NONE',  ( 0.000000000000000000, -1.000000000000000000, 0.000000000000000000 ) ) ;
#31572=AXIS2_PLACEMENT_3D ( 'NONE', #1992, #50357, #18033 ) ;
#31573=DIRECTION ( 'NONE',  ( 0.4566292373937018145, 0.000000000000000000, 0.8896570909947529859 ) ) ;
#31574=DIRECTION ( 'NONE',  ( 0.000000000000000000, -1.000000000000000000, 0.000000000000000000 ) ) ;
#31577=DIRECTION ( 'NONE',  ( -0.9995608365087946812, 0.000000000000000000, 0.02963332782254913048 ) ) ;
#31579=EDGE_CURVE ( 'NONE', #46831, #44523, #12982, .T. ) ;
#31586=EDGE_CURVE ( 'NONE', #47414, #49045, #25713, .T. ) ;
#31588=CARTESIAN_POINT ( 'NONE',  ( -124.1938582159088469, -175.3837268820161057, -99.45993886622792957 ) ) ;
#31589=DIRECTION ( 'NONE',  ( 0.000000000000000000, 0.000000000000000000, -1.000000000000000000 ) ) ;
#31590=AXIS2_PLACEMENT_3D ( 'NONE', #39053, #22539, #6764 ) ;
#31591=CARTESIAN_POINT ( 'NONE',  ( -168.4003408533108086, -183.6283474603465606, -35.26900067126609173 ) ) ;
#31592=DIRECTION ( 'NONE',  ( -0.000000000000000000, 1.000000000000000000, -0.000000000000000000 ) ) ;
#31595=CIRCLE ( 'NONE', #14859, 125.0000000000000000 ) ;
#31596=VECTOR ( 'NONE', #16272, 999.9999999999998863 ) ;
#31597=FACE_OUTER_BOUND ( 'NONE', #29037, .T. ) ;
#31599=CARTESIAN_POINT ( 'NONE',  ( 8.448131207122518305, -189.7472609257535510, 111.2847127925100068 ) ) ;
#31600=DIRECTION ( 'NONE',  ( 0.000000000000000000, -1.000000000000000000, 0.000000000000000000 ) ) ;
#31601=VERTEX_POINT ( 'NONE', #45698 ) ;
#31602=VECTOR ( 'NONE', #47000, 1000.000000000000000 ) ;
#31603=CIRCLE ( 'NONE', #16503, 125.0000000000000000 ) ;
#31604=ORIENTED_EDGE ( 'NONE', *, *, #23287, .F. ) ;
#31605=EDGE_CURVE ( 'NONE', #6500, #37405, #28927, .T. ) ;
#31606=CARTESIAN_POINT ( 'NONE',  ( -95.72791768350688812, -177.1207230881787780, -115.7261930397105090 ) ) ;
#31607=VECTOR ( 'NONE', #29024, 1000.000000000000000 ) ;
#31608=AXIS2_PLACEMENT_3D ( 'NONE', #46331, #2439, #50530 ) ;
#31609=LINE ( 'NONE', #47660, #22080 ) ;
#31610=EDGE_LOOP ( 'NONE', ( #17225, #28381, #50390, #4160 ) ) ;
#31611=ORIENTED_EDGE ( 'NONE', *, *, #32113, .F. ) ;
#31612=CARTESIAN_POINT ( 'NONE',  ( -48.47912675150885065, -177.1207230881787780, 6.938893903907228378E-15 ) ) ;
#31614=LINE ( 'NONE', #43706, #18342 ) ;
#31615=DIRECTION ( 'NONE',  ( -0.5338233779647887367, 0.000000000000000000, -0.8455960035018273979 ) ) ;
#31616=CARTESIAN_POINT ( 'NONE',  ( 8.879953965148883910, -189.7472609257535510, 109.9360785596608707 ) ) ;
#31617=CARTESIAN_POINT ( 'NONE',  ( 44.30815888362531041, -189.7472609257535510, 83.75869879877569701 ) ) ;
#31618=EDGE_LOOP ( 'NONE', ( #452, #51185, #829, #10176 ) ) ;
#31620=ORIENTED_EDGE ( 'NONE', *, *, #8110, .F. ) ;
#31622=LINE ( 'NONE', #35061, #21005 ) ;
#31625=DIRECTION ( 'NONE',  ( 0.000000000000000000, 0.000000000000000000, -1.000000000000000000 ) ) ;
#31626=DIRECTION ( 'NONE',  ( -1.000000000000000000, 0.000000000000000000, -0.000000000000000000 ) ) ;
#31627=VERTEX_POINT ( 'NONE', #9433 ) ;
#31628=DIRECTION ( 'NONE',  ( 0.000000000000000000, -0.000000000000000000, 1.000000000000000000 ) ) ;
#31629=VECTOR ( 'NONE', #35902, 999.9999999999998863 ) ;
#31630=EDGE_CURVE ( 'NONE', #9931, #22453, #9622, .T. ) ;
#31632=DIRECTION ( 'NONE',  ( 0.000000000000000000, 0.000000000000000000, 1.000000000000000000 ) ) ;
#31633=ORIENTED_EDGE ( 'NONE', *, *, #48797, .T. ) ;
#31634=ORIENTED_EDGE ( 'NONE', *, *, #2103, .T. ) ;
#31635=VECTOR ( 'NONE', #9596, 1000.000000000000000 ) ;
#31636=ORIENTED_EDGE ( 'NONE', *, *, #49998, .T. ) ;
#31637=DIRECTION ( 'NONE',  ( -0.1768902751225802927, 0.000000000000000000, 0.9842305779475953864 ) ) ;
#31640=VERTEX_POINT ( 'NONE', #1545 ) ;
#31642=VECTOR ( 'NONE', #36613, 1000.000000000000114 ) ;
#31646=ORIENTED_EDGE ( 'NONE', *, *, #42687, .F. ) ;
#31647=ADVANCED_FACE ( 'NONE', ( #20999 ), #13107, .T. ) ;
#31651=ADVANCED_FACE ( 'NONE', ( #20739 ), #33855, .T. ) ;
#31655=EDGE_CURVE ( 'NONE', #15345, #16448, #11290, .T. ) ;
#31656=EDGE_CURVE ( 'NONE', #2545, #44250, #47398, .T. ) ;
#31657=LINE ( 'NONE', #27182, #48839 ) ;
#31658=ORIENTED_EDGE ( 'NONE', *, *, #31162, .F. ) ;
#31659=FACE_OUTER_BOUND ( 'NONE', #40129, .T. ) ;
#31661=DIRECTION ( 'NONE',  ( 0.000000000000000000, 0.000000000000000000, -1.000000000000000000 ) ) ;
#31666=ORIENTED_EDGE ( 'NONE', *, *, #52036, .T. ) ;
#31667=CIRCLE ( 'NONE', #40059, 125.0000000000000000 ) ;
#31668=AXIS2_PLACEMENT_3D ( 'NONE', #2402, #34956, #51022 ) ;
#31669=CARTESIAN_POINT ( 'NONE',  ( -3.104056038602976741, -193.5000000000000000, -115.4006183233321678 ) ) ;
#31671=ORIENTED_EDGE ( 'NONE', *, *, #8331, .T. ) ;
#31672=VECTOR ( 'NONE', #36392, 1000.000000000000000 ) ;
#31673=ORIENTED_EDGE ( 'NONE', *, *, #21553, .F. ) ;
#31674=PLANE ( 'NONE',  #27943 ) ;
#31679=CIRCLE ( 'NONE', #40076, 125.0000000000000000 ) ;
#31681=ORIENTED_EDGE ( 'NONE', *, *, #46940, .T. ) ;
#31685=AXIS2_PLACEMENT_3D ( 'NONE', #51503, #22617, #15502 ) ;
#31687=CARTESIAN_POINT ( 'NONE',  ( -63.09433862318517328, -193.5000000000000000, -124.1426420773539405 ) ) ;
#31688=ORIENTED_EDGE ( 'NONE', *, *, #4534, .F. ) ;
#31691=AXIS2_PLACEMENT_3D ( 'NONE', #19994, #47613, #31828 ) ;
#31692=CARTESIAN_POINT ( 'NONE',  ( -142.3192003680973414, -177.1207230881787780, 82.57748230379304744 ) ) ;
#31694=DIRECTION ( 'NONE',  ( 0.5338233779647826305, 0.000000000000000000, 0.8455960035018311727 ) ) ;
#31695=CARTESIAN_POINT ( 'NONE',  ( -88.23625491228470707, -183.6283474603465606, 118.5089480183148254 ) ) ;
#31696=CYLINDRICAL_SURFACE ( 'NONE', #39808, 125.0000000000000000 ) ;
#31697=ORIENTED_EDGE ( 'NONE', *, *, #9639, .T. ) ;
#31699=EDGE_CURVE ( 'NONE', #39182, #41471, #13628, .T. ) ;
#31700=EDGE_CURVE ( 'NONE', #37972, #22789, #34117, .T. ) ;
#31701=EDGE_CURVE ( 'NONE', #1446, #10636, #38048, .T. ) ;
#31702=LINE ( 'NONE', #31177, #32462 ) ;
#31704=CARTESIAN_POINT ( 'NONE',  ( 12.99855592850622443, -183.6283474603465606, 108.8370090194294875 ) ) ;
#31706=CIRCLE ( 'NONE', #8185, 125.0000000000000000 ) ;
#31707=VERTEX_POINT ( 'NONE', #22027 ) ;
#31709=LINE ( 'NONE', #28525, #17407 ) ;
#31713=CARTESIAN_POINT ( 'NONE',  ( -56.05401443572781517, -189.7472609257535510, 124.7702732086913073 ) ) ;
#31714=LINE ( 'NONE', #30936, #741 ) ;
#31715=ORIENTED_EDGE ( 'NONE', *, *, #19417, .F. ) ;
#31716=EDGE_CURVE ( 'NONE', #24085, #48695, #14162, .T. ) ;
#31717=DIRECTION ( 'NONE',  ( 0.000000000000000000, -0.000000000000000000, -1.000000000000000000 ) ) ;
#31718=ORIENTED_EDGE ( 'NONE', *, *, #30765, .F. ) ;
#31719=EDGE_CURVE ( 'NONE', #27526, #37757, #44925, .T. ) ;
#31721=DIRECTION ( 'NONE',  ( 0.8124868780056825335, 0.000000000000000000, -0.5829794791144703447 ) ) ;
#31723=ADVANCED_FACE ( 'NONE', ( #10197 ), #38576, .F. ) ;
#31724=LINE ( 'NONE', #31969, #23647 ) ;
#31728=CARTESIAN_POINT ( 'NONE',  ( -48.47912675150885065, -189.7472609257535510, 6.938893903907228378E-15 ) ) ;
#31730=VERTEX_POINT ( 'NONE', #7040 ) ;
#31733=VECTOR ( 'NONE', #35179, 1000.000000000000114 ) ;
#31734=FACE_BOUND ( 'NONE', #33203, .T. ) ;
#31735=ORIENTED_EDGE ( 'NONE', *, *, #25356, .T. ) ;
#31736=DIRECTION ( 'NONE',  ( 0.000000000000000000, -1.000000000000000000, 0.000000000000000000 ) ) ;
#31737=DIRECTION ( 'NONE',  ( 0.000000000000000000, 1.000000000000000000, 0.000000000000000000 ) ) ;
#31738=ORIENTED_EDGE ( 'NONE', *, *, #2542, .F. ) ;
#31740=ORIENTED_EDGE ( 'NONE', *, *, #42081, .T. ) ;
#31741=EDGE_CURVE ( 'NONE', #10636, #41581, #14412, .T. ) ;
#31742=AXIS2_PLACEMENT_3D ( 'NONE', #3714, #31843, #8438 ) ;
#31743=DIRECTION ( 'NONE',  ( 0.4566292373937018145, 0.000000000000000000, 0.8896570909947529859 ) ) ;
#31744=VECTOR ( 'NONE', #44576, 1000.000000000000114 ) ;
#31745=VECTOR ( 'NONE', #11836, 1000.000000000000000 ) ;
#31746=FACE_BOUND ( 'NONE', #38039, .T. ) ;
#31747=FACE_OUTER_BOUND ( 'NONE', #38270, .T. ) ;
#31748=ORIENTED_EDGE ( 'NONE', *, *, #5168, .T. ) ;
#31749=CIRCLE ( 'NONE', #49399, 124.9999999999999858 ) ;
#31750=CARTESIAN_POINT ( 'NONE',  ( 52.59568867645218404, -193.5000000000000000, -73.54509967498589162 ) ) ;
#31751=ORIENTED_EDGE ( 'NONE', *, *, #21827, .T. ) ;
#31752=ORIENTED_EDGE ( 'NONE', *, *, #22119, .F. ) ;
#31753=EDGE_CURVE ( 'NONE', #42165, #38881, #46222, .T. ) ;
#31754=DIRECTION ( 'NONE',  ( 0.8455960035018234011, 0.000000000000000000, 0.5338233779647948429 ) ) ;
#31756=EDGE_LOOP ( 'NONE', ( #20354, #17571, #45094, #35148 ) ) ;
#31758=LINE ( 'NONE', #40154, #17978 ) ;
#31759=EDGE_CURVE ( 'NONE', #39207, #21817, #46993, .T. ) ;
#31760=EDGE_CURVE ( 'NONE', #5462, #20620, #38310, .T. ) ;
#31762=EDGE_CURVE ( 'NONE', #40799, #12141, #18359, .T. ) ;
#31764=AXIS2_PLACEMENT_3D ( 'NONE', #31244, #47297, #19946 ) ;
#31765=DIRECTION ( 'NONE',  ( 0.000000000000000000, -1.000000000000000000, 0.000000000000000000 ) ) ;
#31766=CARTESIAN_POINT ( 'NONE',  ( -26.20043062753592977, -193.5000000000000000, -122.9986166548863196 ) ) ;
#31768=LINE ( 'NONE', #19665, #31733 ) ;
#31769=LINE ( 'NONE', #16790, #46592 ) ;
#31771=EDGE_CURVE ( 'NONE', #9203, #39625, #26744, .T. ) ;
#31772=LINE ( 'NONE', #43594, #44098 ) ;
#31773=ORIENTED_EDGE ( 'NONE', *, *, #18555, .T. ) ;
#31774=PLANE ( 'NONE',  #19728 ) ;
#31778=EDGE_CURVE ( 'NONE', #27687, #21993, #14685, .T. ) ;
#31779=PLANE ( 'NONE',  #22483 ) ;
#31780=CARTESIAN_POINT ( 'NONE',  ( -45.06671089634842531, -183.6283474603465606, -124.9534129907280686 ) ) ;
#31781=ORIENTED_EDGE ( 'NONE', *, *, #7479, .T. ) ;
#31782=ADVANCED_FACE ( 'NONE', ( #43032 ), #50936, .T. ) ;
#31784=VERTEX_POINT ( 'NONE', #23066 ) ;
#31785=CARTESIAN_POINT ( 'NONE',  ( -171.2399149993172500, -193.5000000000000000, -17.48697739784459415 ) ) ;
#31786=CIRCLE ( 'NONE', #4936, 125.0000000000000000 ) ;
#31787=DIRECTION ( 'NONE',  ( 0.000000000000000000, 0.000000000000000000, 1.000000000000000000 ) ) ;
#31788=EDGE_CURVE ( 'NONE', #22776, #48106, #39076, .T. ) ;
#31789=AXIS2_PLACEMENT_3D ( 'NONE', #28324, #31765, #35963 ) ;
#31790=DIRECTION ( 'NONE',  ( -0.7765238627180482966, 0.000000000000000000, 0.6300878435817038881 ) ) ;
#31792=FACE_OUTER_BOUND ( 'NONE', #12298, .T. ) ;
#31793=CIRCLE ( 'NONE', #25087, 125.0000000000000000 ) ;
#31794=DIRECTION ( 'NONE',  ( 0.9027978299657446470, 0.000000000000000000, -0.4300652022765183435 ) ) ;
#31795=ADVANCED_FACE ( 'NONE', ( #39343 ), #3348, .T. ) ;
#31796=ORIENTED_EDGE ( 'NONE', *, *, #19759, .F. ) ;
#31799=DIRECTION ( 'NONE',  ( -0.9564009842765264224, 0.000000000000000000, 0.2920567706369628924 ) ) ;
#31801=DIRECTION ( 'NONE',  ( -0.000000000000000000, 1.000000000000000000, -0.000000000000000000 ) ) ;
#31803=AXIS2_PLACEMENT_3D ( 'NONE', #21744, #29875, #45935 ) ;
#31804=CARTESIAN_POINT ( 'NONE',  ( -64.08700758308647494, -189.7472609257535510, -124.0217483183786840 ) ) ;
#31807=EDGE_LOOP ( 'NONE', ( #41278, #14804, #9295, #4621 ) ) ;
#31810=EDGE_LOOP ( 'NONE', ( #24551, #12606, #36915, #41841 ) ) ;
#31811=ADVANCED_FACE ( 'NONE', ( #28023 ), #15187, .F. ) ;
#31812=CARTESIAN_POINT ( 'NONE',  ( -159.5526844214375615, -177.1207230881787780, 57.33816169485226055 ) ) ;
#31813=LINE ( 'NONE', #23652, #23723 ) ;
#31815=ORIENTED_EDGE ( 'NONE', *, *, #23595, .T. ) ;
#31817=EDGE_LOOP ( 'NONE', ( #36964, #31980 ) ) ;
#31819=AXIS2_PLACEMENT_3D ( 'NONE', #10738, #22825, #42794 ) ;
#31820=ORIENTED_EDGE ( 'NONE', *, *, #50052, .T. ) ;
#31821=DIRECTION ( 'NONE',  ( -0.000000000000000000, 1.000000000000000000, -0.000000000000000000 ) ) ;
#31822=CIRCLE ( 'NONE', #3314, 125.0000000000000000 ) ;
#31823=EDGE_CURVE ( 'NONE', #29476, #728, #15710, .T. ) ;
#31824=EDGE_CURVE ( 'NONE', #13870, #29270, #22255, .T. ) ;
#31825=ORIENTED_EDGE ( 'NONE', *, *, #10118, .T. ) ;
#31826=CARTESIAN_POINT ( 'NONE',  ( -173.0563034899574859, -189.7472609257535510, -10.27263529369817618 ) ) ;
#31827=DIRECTION ( 'NONE',  ( 0.000000000000000000, 1.000000000000000000, 0.000000000000000000 ) ) ;
#31828=DIRECTION ( 'NONE',  ( 0.000000000000000000, 0.000000000000000000, 1.000000000000000000 ) ) ;
#31832=EDGE_LOOP ( 'NONE', ( #47892, #46961, #34358, #34505 ) ) ;
#31833=DIRECTION ( 'NONE',  ( -0.000000000000000000, 1.000000000000000000, -0.000000000000000000 ) ) ;
#31834=ORIENTED_EDGE ( 'NONE', *, *, #36509, .F. ) ;
#31835=CARTESIAN_POINT ( 'NONE',  ( -59.81005805956441179, -183.6283474603465606, -123.4817304940906126 ) ) ;
#31838=DIRECTION ( 'NONE',  ( -0.000000000000000000, 1.000000000000000000, -0.000000000000000000 ) ) ;
#31839=VERTEX_POINT ( 'NONE', #27518 ) ;
#31840=AXIS2_PLACEMENT_3D ( 'NONE', #21058, #37075, #9494 ) ;
#31842=CARTESIAN_POINT ( 'NONE',  ( 43.63512310656540905, -189.7472609257535510, 84.49831343337136502 ) ) ;
#31843=DIRECTION ( 'NONE',  ( 0.000000000000000000, 0.000000000000000000, 1.000000000000000000 ) ) ;
#31844=VERTEX_POINT ( 'NONE', #47253 ) ;
#31845=ADVANCED_FACE ( 'NONE', ( #11222 ), #24355, .T. ) ;
#31846=DIRECTION ( 'NONE',  ( 0.9564009842765202052, 0.000000000000000000, 0.2920567706369833760 ) ) ;
#31847=CARTESIAN_POINT ( 'NONE',  ( 48.06131630543706734, -189.7472609257535510, -79.40367028273054473 ) ) ;
#31848=LINE ( 'NONE', #19747, #19810 ) ;
#31849=ORIENTED_EDGE ( 'NONE', *, *, #50449, .T. ) ;
#31850=LINE ( 'NONE', #16086, #33484 ) ;
#31853=ORIENTED_EDGE ( 'NONE', *, *, #22600, .F. ) ;
#31854=DIRECTION ( 'NONE',  ( 0.000000000000000000, -1.000000000000000000, 0.000000000000000000 ) ) ;
#31856=AXIS2_PLACEMENT_3D ( 'NONE', #26703, #27203, #18560 ) ;
#31857=DIRECTION ( 'NONE',  ( 0.000000000000000000, -0.000000000000000000, -1.000000000000000000 ) ) ;
#31859=AXIS2_PLACEMENT_3D ( 'NONE', #39942, #43651, #3696 ) ;
#31860=DIRECTION ( 'NONE',  ( 0.000000000000000000, 0.000000000000000000, -1.000000000000000000 ) ) ;
#31861=CARTESIAN_POINT ( 'NONE',  ( -156.9880281022168447, -193.5000000000000000, -60.01515274640934194 ) ) ;
#31862=DIRECTION ( 'NONE',  ( 0.000000000000000000, 1.000000000000000000, 0.000000000000000000 ) ) ;
#31863=PLANE ( 'NONE',  #38027 ) ;
#31864=FACE_OUTER_BOUND ( 'NONE', #31248, .T. ) ;
#31865=LINE ( 'NONE', #31599, #16333 ) ;
#31866=CARTESIAN_POINT ( 'NONE',  ( -165.5546359831674295, -177.1207230881787780, 43.79868877201492694 ) ) ;
#31867=VERTEX_POINT ( 'NONE', #31971 ) ;
#31870=AXIS2_PLACEMENT_3D ( 'NONE', #46695, #26716, #10165 ) ;
#31872=ORIENTED_EDGE ( 'NONE', *, *, #34386, .F. ) ;
#31873=ORIENTED_EDGE ( 'NONE', *, *, #16609, .T. ) ;
#31874=ORIENTED_EDGE ( 'NONE', *, *, #3512, .T. ) ;
#31875=DIRECTION ( 'NONE',  ( 0.1182731709213660498, 0.000000000000000000, -0.9929810960135169173 ) ) ;
#31876=DIRECTION ( 'NONE',  ( 0.000000000000000000, -1.000000000000000000, 0.000000000000000000 ) ) ;
#31877=EDGE_CURVE ( 'NONE', #28119, #38913, #43290, .T. ) ;
#31878=DIRECTION ( 'NONE',  ( -0.000000000000000000, 1.000000000000000000, 0.000000000000000000 ) ) ;
#31879=CARTESIAN_POINT ( 'NONE',  ( -4.794493649713349015, -175.3837268820161057, -117.1181148702518726 ) ) ;
#31881=ORIENTED_EDGE ( 'NONE', *, *, #34534, .T. ) ;
#31882=ORIENTED_EDGE ( 'NONE', *, *, #48467, .T. ) ;
#31884=CARTESIAN_POINT ( 'NONE',  ( -23.99795575808070325, -183.6283474603465606, -122.5792489240757561 ) ) ;
#31885=CARTESIAN_POINT ( 'NONE',  ( 5.015379008610432621, -177.1207230881787780, -112.9749434763326832 ) ) ;
#31887=LINE ( 'NONE', #7966, #4391 ) ;
#31888=DIRECTION ( 'NONE',  ( 0.000000000000000000, 1.000000000000000000, 0.000000000000000000 ) ) ;
#31889=EDGE_LOOP ( 'NONE', ( #47288, #9742, #21122, #20634 ) ) ;
#31890=CARTESIAN_POINT ( 'NONE',  ( 15.23368049493604381, -193.5000000000000000, -107.5438431188757420 ) ) ;
#31891=DIRECTION ( 'NONE',  ( 0.000000000000000000, 0.000000000000000000, -1.000000000000000000 ) ) ;
#31892=LINE ( 'NONE', #11909, #27335 ) ;
#31893=CARTESIAN_POINT ( 'NONE',  ( -12.42681898335384538, -189.7472609257535510, 118.6432945265039507 ) ) ;
#31894=ORIENTED_EDGE ( 'NONE', *, *, #50392, .T. ) ;
#31895=EDGE_LOOP ( 'NONE', ( #22786, #21811, #48987, #38715 ) ) ;
#31896=ORIENTED_EDGE ( 'NONE', *, *, #16841, .T. ) ;
#31901=PLANE ( 'NONE',  #50905 ) ;
#31904=ORIENTED_EDGE ( 'NONE', *, *, #12668, .F. ) ;
#31906=VECTOR ( 'NONE', #6182, 1000.000000000000000 ) ;
#31907=AXIS2_PLACEMENT_3D ( 'NONE', #11870, #51325, #31331 ) ;
#31908=ORIENTED_EDGE ( 'NONE', *, *, #38757, .F. ) ;
#31909=CARTESIAN_POINT ( 'NONE',  ( -45.12595152424216138, -193.5000000000000000, -123.9551692589637213 ) ) ;
#31911=CARTESIAN_POINT ( 'NONE',  ( 74.60098876342242136, -193.5000000000000000, 21.82395850507348811 ) ) ;
#31912=ORIENTED_EDGE ( 'NONE', *, *, #51103, .T. ) ;
#31914=DIRECTION ( 'NONE',  ( 0.1768902751225592818, 0.000000000000000000, 0.9842305779475992722 ) ) ;
#31916=ADVANCED_FACE ( 'NONE', ( #39587 ), #43800, .T. ) ;
#31917=CARTESIAN_POINT ( 'NONE',  ( 24.15597040328004752, -177.1207230881787780, -101.7307360698543874 ) ) ;
#31918=EDGE_LOOP ( 'NONE', ( #21831, #3253, #29729, #47349 ) ) ;
#31919=LINE ( 'NONE', #27975, #950 ) ;
#31922=CIRCLE ( 'NONE', #21016, 125.0000000000000000 ) ;
#31924=CARTESIAN_POINT ( 'NONE',  ( -112.7586829773731267, -189.7472609257535510, -107.2060569716373379 ) ) ;
#31925=ORIENTED_EDGE ( 'NONE', *, *, #4453, .F. ) ;
#31927=EDGE_LOOP ( 'NONE', ( #25412, #31934, #13162, #10246 ) ) ;
#31928=LINE ( 'NONE', #16435, #45017 ) ;
#31930=CARTESIAN_POINT ( 'NONE',  ( -47.63353074800702558, -177.1207230881787780, -0.5338233779647817423 ) ) ;
#31932=DIRECTION ( 'NONE',  ( -0.4639789333096864810, 0.000000000000000000, -0.8858462335218260097 ) ) ;
#31933=DIRECTION ( 'NONE',  ( 0.000000000000000000, -0.000000000000000000, -1.000000000000000000 ) ) ;
#31934=ORIENTED_EDGE ( 'NONE', *, *, #42980, .F. ) ;
#31935=DIRECTION ( 'NONE',  ( 0.000000000000000000, -0.000000000000000000, 1.000000000000000000 ) ) ;
#31936=DIRECTION ( 'NONE',  ( 0.1182731709213523247, 0.000000000000000000, 0.9929810960135185827 ) ) ;
#31937=EDGE_CURVE ( 'NONE', #4302, #38037, #19891, .T. ) ;
#31938=DIRECTION ( 'NONE',  ( -0.000000000000000000, 1.000000000000000000, -0.000000000000000000 ) ) ;
#31942=ADVANCED_FACE ( 'NONE', ( #11994 ), #24110, .T. ) ;
#31945=EDGE_LOOP ( 'NONE', ( #4894, #31245, #43220, #46851 ) ) ;
#31946=CARTESIAN_POINT ( 'NONE',  ( -163.3872488209693756, -177.1207230881787780, -49.20491319441543254 ) ) ;
#31947=CARTESIAN_POINT ( 'NONE',  ( -137.9639882952644143, -193.5000000000000000, 87.27805883780241913 ) ) ;
#31949=CARTESIAN_POINT ( 'NONE',  ( -78.41101675714241992, -175.3837268820161057, -120.3332351033023286 ) ) ;
#31950=DIRECTION ( 'NONE',  ( 0.000000000000000000, 0.000000000000000000, -1.000000000000000000 ) ) ;
#31951=CARTESIAN_POINT ( 'NONE',  ( -101.9736325116273576, -193.5000000000000000, 112.9749434763330811 ) ) ;
#31952=VERTEX_POINT ( 'NONE', #51201 ) ;
#31953=CARTESIAN_POINT ( 'NONE',  ( -67.22356632362119910, -183.6283474603465606, -123.5865930638409793 ) ) ;
#31954=ORIENTED_EDGE ( 'NONE', *, *, #20750, .F. ) ;
#31955=CARTESIAN_POINT ( 'NONE',  ( -55.65514169787636689, -175.3837268820161057, -123.7921848946937331 ) ) ;
#31956=ORIENTED_EDGE ( 'NONE', *, *, #21761, .F. ) ;
#31957=ORIENTED_EDGE ( 'NONE', *, *, #24630, .T. ) ;
#31958=AXIS2_PLACEMENT_3D ( 'NONE', #33236, #38208, #46125 ) ;
#31959=CYLINDRICAL_SURFACE ( 'NONE', #9843, 125.0000000000000000 ) ;
#31960=ADVANCED_FACE ( 'NONE', ( #1678 ), #12768, .T. ) ;
#31961=PLANE ( 'NONE',  #30827 ) ;
#31962=DIRECTION ( 'NONE',  ( 0.000000000000000000, 0.000000000000000000, -1.000000000000000000 ) ) ;
#31964=EDGE_LOOP ( 'NONE', ( #29593, #40650, #36884, #31086 ) ) ;
#31965=CARTESIAN_POINT ( 'NONE',  ( -140.8230258362169707, -189.7472609257535510, 84.24728067916045404 ) ) ;
#31966=EDGE_LOOP ( 'NONE', ( #40045, #47793, #21728, #43012 ) ) ;
#31968=CARTESIAN_POINT ( 'NONE',  ( -40.24578378811990831, -189.7472609257535510, 124.7285535218268251 ) ) ;
#31969=CARTESIAN_POINT ( 'NONE',  ( -114.9600645115007467, -183.6283474603465606, 105.8550183720738147 ) ) ;
#31970=LINE ( 'NONE', #48009, #46680 ) ;
#31971=CARTESIAN_POINT ( 'NONE',  ( -62.97606545226378216, -189.7472609257535510, -123.1496609813404319 ) ) ;
#31972=AXIS2_PLACEMENT_3D ( 'NONE', #51017, #15012, #11035 ) ;
#31974=DIRECTION ( 'NONE',  ( -0.000000000000000000, 1.000000000000000000, -0.000000000000000000 ) ) ;
#31975=ORIENTED_EDGE ( 'NONE', *, *, #39739, .T. ) ;
#31976=DIRECTION ( 'NONE',  ( 0.6965510290629982615, 0.000000000000000000, -0.7175072570443298270 ) ) ;
#31977=DIRECTION ( 'NONE',  ( 0.9646355819083594074, 0.000000000000000000, -0.2635871660690647933 ) ) ;
#31978=VECTOR ( 'NONE', #34263, 1000.000000000000000 ) ;
#31979=FACE_BOUND ( 'NONE', #32013, .T. ) ;
#31980=ORIENTED_EDGE ( 'NONE', *, *, #23359, .F. ) ;
#31983=ADVANCED_FACE ( 'NONE', ( #48795 ), #1932, .T. ) ;
#31984=ORIENTED_EDGE ( 'NONE', *, *, #50645, .T. ) ;
#31985=EDGE_CURVE ( 'NONE', #7370, #45652, #37678, .T. ) ;
#31987=VERTEX_POINT ( 'NONE', #5634 ) ;
#31988=DIRECTION ( 'NONE',  ( 0.000000000000000000, 1.000000000000000000, -0.000000000000000000 ) ) ;
#31989=CIRCLE ( 'NONE', #9354, 125.0000000000000000 ) ;
#31990=FACE_BOUND ( 'NONE', #47036, .T. ) ;
#31991=CARTESIAN_POINT ( 'NONE',  ( 20.66186849114819069, -193.5000000000000000, -104.1370384486465070 ) ) ;
#31992=ORIENTED_EDGE ( 'NONE', *, *, #40635, .F. ) ;
#31997=ORIENTED_EDGE ( 'NONE', *, *, #1897, .T. ) ;
#31998=CARTESIAN_POINT ( 'NONE',  ( -4.794493649713342798, -175.3837268820161057, -117.1181148702518726 ) ) ;
#32000=VERTEX_POINT ( 'NONE', #33731 ) ;
#32001=CARTESIAN_POINT ( 'NONE',  ( 53.56330073376472711, -189.7472609257535510, 72.19655804062050208 ) ) ;
#32002=LINE ( 'NONE', #16249, #21310 ) ;
#32005=VECTOR ( 'NONE', #42720, 1000.000000000000000 ) ;
#32006=CIRCLE ( 'NONE', #23649, 125.0000000000000000 ) ;
#32008=DIRECTION ( 'NONE',  ( 0.9842305779475980509, 0.000000000000000000, -0.1768902751225666647 ) ) ;
#32011=FACE_OUTER_BOUND ( 'NONE', #50045, .T. ) ;
#32012=ORIENTED_EDGE ( 'NONE', *, *, #20678, .T. ) ;
#32013=EDGE_LOOP ( 'NONE', ( #11511, #39673, #7376, #39180 ) ) ;
#32014=CARTESIAN_POINT ( 'NONE',  ( -56.71246971489870958, -189.7472609257535510, -124.7285535218267682 ) ) ;
#32015=ORIENTED_EDGE ( 'NONE', *, *, #20646, .T. ) ;
#32019=ORIENTED_EDGE ( 'NONE', *, *, #8566, .F. ) ;
#32020=CARTESIAN_POINT ( 'NONE',  ( -85.14888725715768203, -193.5000000000000000, 119.5003291395398577 ) ) ;
#32021=DIRECTION ( 'NONE',  ( 0.000000000000000000, 0.000000000000000000, 1.000000000000000000 ) ) ;
#32024=ORIENTED_EDGE ( 'NONE', *, *, #15241, .T. ) ;
#32025=CARTESIAN_POINT ( 'NONE',  ( -144.2430459457361280, -189.7472609257535510, 78.77358243914956404 ) ) ;
#32028=CARTESIAN_POINT ( 'NONE',  ( 59.29945538372744807, -177.1207230881787780, 63.31490529818492519 ) ) ;
#32032=ORIENTED_EDGE ( 'NONE', *, *, #33560, .F. ) ;
#32033=CARTESIAN_POINT ( 'NONE',  ( -139.8555433305420195, -175.3837268820161057, -83.82333043185244037 ) ) ;
#32034=CARTESIAN_POINT ( 'NONE',  ( -48.93575598890257794, -183.6283474603465606, 0.8896570909947506545 ) ) ;
#32037=ORIENTED_EDGE ( 'NONE', *, *, #29172, .F. ) ;
#32039=VECTOR ( 'NONE', #36291, 1000.000000000000000 ) ;
#32040=EDGE_CURVE ( 'NONE', #7438, #35703, #26096, .T. ) ;
#32041=LINE ( 'NONE', #43623, #31119 ) ;
#32045=EDGE_CURVE ( 'NONE', #34518, #1575, #24871, .T. ) ;
#32047=AXIS2_PLACEMENT_3D ( 'NONE', #17192, #36901, #16416 ) ;
#32048=ORIENTED_EDGE ( 'NONE', *, *, #31771, .T. ) ;
#32049=EDGE_CURVE ( 'NONE', #50010, #20455, #44845, .T. ) ;
#32050=VECTOR ( 'NONE', #37570, 1000.000000000000000 ) ;
#32051=PLANE ( 'NONE',  #43562 ) ;
#32052=EDGE_CURVE ( 'NONE', #24430, #24544, #705, .T. ) ;
#32053=CARTESIAN_POINT ( 'NONE',  ( -111.8989814360438828, -175.3837268820161057, -107.7168604805787027 ) ) ;
#32054=CARTESIAN_POINT ( 'NONE',  ( 15.23368049493604381, -193.5000000000000000, -107.5438431188757420 ) ) ;
#32057=EDGE_CURVE ( 'NONE', #34863, #1466, #30048, .T. ) ;
#32059=AXIS2_PLACEMENT_3D ( 'NONE', #14240, #30258, #38398 ) ;
#32060=ORIENTED_EDGE ( 'NONE', *, *, #4561, .F. ) ;
#32061=EDGE_CURVE ( 'NONE', #9877, #40690, #13864, .T. ) ;
#32062=VERTEX_POINT ( 'NONE', #42125 ) ;
#32065=AXIS2_PLACEMENT_3D ( 'NONE', #14850, #30865, #10890 ) ;
#32066=ADVANCED_FACE ( 'NONE', ( #10080 ), #6146, .T. ) ;
#32068=FACE_OUTER_BOUND ( 'NONE', #42230, .T. ) ;
#32069=EDGE_CURVE ( 'NONE', #10459, #15796, #33169, .T. ) ;
#32071=ADVANCED_FACE ( 'NONE', ( #2701 ), #38949, .T. ) ;
#32072=ADVANCED_FACE ( 'NONE', ( #19266 ), #35021, .T. ) ;
#32073=DIRECTION ( 'NONE',  ( -0.000000000000000000, 1.000000000000000000, -0.000000000000000000 ) ) ;
#32077=ORIENTED_EDGE ( 'NONE', *, *, #13734, .T. ) ;
#32078=CARTESIAN_POINT ( 'NONE',  ( -77.67449977936057337, -189.7472609257535510, -121.5427093402339267 ) ) ;
#32079=ORIENTED_EDGE ( 'NONE', *, *, #15406, .F. ) ;
#32080=FACE_OUTER_BOUND ( 'NONE', #25074, .T. ) ;
#32083=DIRECTION ( 'NONE',  ( 0.000000000000000000, 0.000000000000000000, -1.000000000000000000 ) ) ;
#32084=CARTESIAN_POINT ( 'NONE',  ( 63.39453919430265927, -189.7472609257535510, 53.48161459190912126 ) ) ;
#32085=CARTESIAN_POINT ( 'NONE',  ( 14.43219681437621205, -189.7472609257535510, 106.8558168688117860 ) ) ;
#32087=EDGE_CURVE ( 'NONE', #17378, #34311, #46603, .T. ) ;
#32088=VERTEX_POINT ( 'NONE', #42652 ) ;
#32089=CIRCLE ( 'NONE', #4374, 125.0000000000000000 ) ;
#32090=DIRECTION ( 'NONE',  ( 0.000000000000000000, 0.000000000000000000, 1.000000000000000000 ) ) ;
#32091=LINE ( 'NONE', #4509, #31219 ) ;
#32092=ORIENTED_EDGE ( 'NONE', *, *, #19254, .T. ) ;
#32093=DIRECTION ( 'NONE',  ( 0.000000000000000000, 0.000000000000000000, 1.000000000000000000 ) ) ;
#32094=DIRECTION ( 'NONE',  ( 0.000000000000000000, 1.000000000000000000, 0.000000000000000000 ) ) ;
#32095=ORIENTED_EDGE ( 'NONE', *, *, #10533, .T. ) ;
#32096=FACE_OUTER_BOUND ( 'NONE', #14913, .T. ) ;
#32101=CARTESIAN_POINT ( 'NONE',  ( 47.04848625005566021, -177.1207230881787780, 80.61932246194658092 ) ) ;
#32102=ORIENTED_EDGE ( 'NONE', *, *, #7696, .F. ) ;
#32103=AXIS2_PLACEMENT_3D ( 'NONE', #37988, #50609, #9372 ) ;
#32104=CIRCLE ( 'NONE', #51449, 125.0000000000000000 ) ;
#32105=CARTESIAN_POINT ( 'NONE',  ( -48.47912675150885065, -189.7472609257535510, 6.938893903907228378E-15 ) ) ;
#32106=DIRECTION ( 'NONE',  ( 0.000000000000000000, 1.000000000000000000, 0.000000000000000000 ) ) ;
#32107=EDGE_CURVE ( 'NONE', #41052, #16634, #14807, .T. ) ;
#32108=DIRECTION ( 'NONE',  ( 0.5586467658036535777, 0.000000000000000000, -0.8294056854502011022 ) ) ;
#32109=DIRECTION ( 'NONE',  ( 0.000000000000000000, 0.000000000000000000, 1.000000000000000000 ) ) ;
#32110=DIRECTION ( 'NONE',  ( 0.000000000000000000, 0.000000000000000000, 1.000000000000000000 ) ) ;
#32113=EDGE_CURVE ( 'NONE', #19097, #14204, #22940, .T. ) ;
#32114=CARTESIAN_POINT ( 'NONE',  ( -30.31202594373734271, -177.1207230881787780, -123.6727797384706093 ) ) ;
#32115=EDGE_CURVE ( 'NONE', #21117, #7438, #43160, .T. ) ;
#32117=CARTESIAN_POINT ( 'NONE',  ( 14.72514937628681508, -193.5000000000000000, -106.6827995071083848 ) ) ;
#32122=LINE ( 'NONE', #7455, #7299 ) ;
#32124=FACE_OUTER_BOUND ( 'NONE', #50081, .T. ) ;
#32125=ORIENTED_EDGE ( 'NONE', *, *, #45914, .F. ) ;
#32126=ORIENTED_EDGE ( 'NONE', *, *, #6763, .T. ) ;
#32127=EDGE_CURVE ( 'NONE', #2085, #10130, #22682, .T. ) ;
#32128=ORIENTED_EDGE ( 'NONE', *, *, #51776, .F. ) ;
#32131=CARTESIAN_POINT ( 'NONE',  ( -165.1736796818183564, -183.6283474603465606, -41.93543928473609839 ) ) ;
#32132=DIRECTION ( 'NONE',  ( 0.000000000000000000, -0.000000000000000000, -1.000000000000000000 ) ) ;
#32136=VERTEX_POINT ( 'NONE', #38695 ) ;
#32137=ADVANCED_FACE ( 'NONE', ( #18998 ), #7165, .T. ) ;
#32144=CARTESIAN_POINT ( 'NONE',  ( 11.61413489515543418, -177.1207230881787780, -109.6074810615842381 ) ) ;
#32145=ORIENTED_EDGE ( 'NONE', *, *, #5139, .T. ) ;
#32146=LINE ( 'NONE', #35565, #17996 ) ;
#32147=AXIS2_PLACEMENT_3D ( 'NONE', #36184, #185, #43816 ) ;
#32148=DIRECTION ( 'NONE',  ( 0.9266896074318317078, 0.000000000000000000, 0.3758275821142421647 ) ) ;
#32149=DIRECTION ( 'NONE',  ( 0.000000000000000000, 1.000000000000000000, 0.000000000000000000 ) ) ;
#32150=CARTESIAN_POINT ( 'NONE',  ( -68.09401750944520870, -193.5000000000000000, -122.4396006697294581 ) ) ;
#32152=ORIENTED_EDGE ( 'NONE', *, *, #43277, .T. ) ;
#32154=CARTESIAN_POINT ( 'NONE',  ( -150.1390659022305840, -175.3837268820161057, 72.73415134496005408 ) ) ;
#32157=PLANE ( 'NONE',  #25726 ) ;
#32158=AXIS2_PLACEMENT_3D ( 'NONE', #7372, #35457, #31009 ) ;
#32163=CARTESIAN_POINT ( 'NONE',  ( -96.65280530915693191, -177.1207230881787780, -115.3442529744087466 ) ) ;
#32164=AXIS2_PLACEMENT_3D ( 'NONE', #16110, #20293, #48693 ) ;
#32165=VERTEX_POINT ( 'NONE', #27384 ) ;
#32166=LINE ( 'NONE', #48212, #30742 ) ;
#32168=CARTESIAN_POINT ( 'NONE',  ( 10.22625775207003507, -177.1207230881787780, -109.2239789693433352 ) ) ;
#32169=FACE_BOUND ( 'NONE', #10954, .T. ) ;
#32170=DIRECTION ( 'NONE',  ( -0.08879589532293158394, 0.000000000000000000, -0.9960498426152172291 ) ) ;
#32171=ORIENTED_EDGE ( 'NONE', *, *, #7066, .F. ) ;
#32172=DIRECTION ( 'NONE',  ( 0.000000000000000000, 0.000000000000000000, 1.000000000000000000 ) ) ;
#32173=DIRECTION ( 'NONE',  ( 0.000000000000000000, -0.000000000000000000, 1.000000000000000000 ) ) ;
#32175=EDGE_CURVE ( 'NONE', #21817, #6661, #35274, .T. ) ;
#32177=AXIS2_PLACEMENT_3D ( 'NONE', #42094, #26323, #33942 ) ;
#32178=PLANE ( 'NONE',  #48410 ) ;
#32180=DIRECTION ( 'NONE',  ( -0.000000000000000000, 1.000000000000000000, -0.000000000000000000 ) ) ;
#32182=VERTEX_POINT ( 'NONE', #31588 ) ;
#32184=CYLINDRICAL_SURFACE ( 'NONE', #26838, 125.0000000000000000 ) ;
#32185=CARTESIAN_POINT ( 'NONE',  ( -157.8637630444124795, -189.7472609257535510, -60.49794494914010556 ) ) ;
#32187=EDGE_LOOP ( 'NONE', ( #18862, #19030, #46935, #3443 ) ) ;
#32188=CARTESIAN_POINT ( 'NONE',  ( 1.663811650136611586, -189.7472609257535510, -113.4093733337827530 ) ) ;
#32190=ORIENTED_EDGE ( 'NONE', *, *, #31059, .F. ) ;
#32192=CARTESIAN_POINT ( 'NONE',  ( 75.67769207106684348, -183.6283474603465606, 14.49428645563876827 ) ) ;
#32193=EDGE_CURVE ( 'NONE', #25190, #26407, #11353, .T. ) ;
#32194=ORIENTED_EDGE ( 'NONE', *, *, #24644, .F. ) ;
#32195=CARTESIAN_POINT ( 'NONE',  ( -38.78589637709155369, -193.5000000000000000, -123.6213615703898654 ) ) ;
#32196=DIRECTION ( 'NONE',  ( 0.000000000000000000, 0.000000000000000000, 1.000000000000000000 ) ) ;
#32197=CIRCLE ( 'NONE', #46468, 125.0000000000000000 ) ;
#32199=PLANE ( 'NONE',  #24904 ) ;
#32200=EDGE_LOOP ( 'NONE', ( #4280, #2028, #38919, #43477 ) ) ;
#32202=AXIS2_PLACEMENT_3D ( 'NONE', #21344, #33161, #9265 ) ;
#32203=EDGE_CURVE ( 'NONE', #35744, #45569, #43681, .T. ) ;
#32204=VERTEX_POINT ( 'NONE', #2454 ) ;
#32205=DIRECTION ( 'NONE',  ( -0.9027978299657477557, 0.000000000000000000, 0.4300652022765115712 ) ) ;
#32210=ORIENTED_EDGE ( 'NONE', *, *, #31344, .F. ) ;
#32211=EDGE_CURVE ( 'NONE', #24136, #38799, #39977, .T. ) ;
#32212=VECTOR ( 'NONE', #36994, 1000.000000000000114 ) ;
#32217=DIRECTION ( 'NONE',  ( -0.000000000000000000, 1.000000000000000000, -0.000000000000000000 ) ) ;
#32219=CARTESIAN_POINT ( 'NONE',  ( -123.4791267515088435, -198.5000000000000000, 70.00000000000000000 ) ) ;
#32220=LINE ( 'NONE', #48264, #9987 ) ;
#32222=CARTESIAN_POINT ( 'NONE',  ( 27.42205759510524032, -189.7472609257535510, 98.05618656931997634 ) ) ;
#32225=ORIENTED_EDGE ( 'NONE', *, *, #4135, .F. ) ;
#32227=DIRECTION ( 'NONE',  ( 0.000000000000000000, -0.000000000000000000, -1.000000000000000000 ) ) ;
#32229=DIRECTION ( 'NONE',  ( -0.000000000000000000, 1.000000000000000000, 0.000000000000000000 ) ) ;
#32231=DIRECTION ( 'NONE',  ( 0.000000000000000000, 0.000000000000000000, 1.000000000000000000 ) ) ;
#32232=CARTESIAN_POINT ( 'NONE',  ( 73.79319191488886531, -193.5000000000000000, 20.63201007055492653 ) ) ;
#32234=VERTEX_POINT ( 'NONE', #39714 ) ;
#32235=DIRECTION ( 'NONE',  ( -0.000000000000000000, 1.000000000000000000, -0.000000000000000000 ) ) ;
#32237=CIRCLE ( 'NONE', #38945, 125.0000000000000000 ) ;
#32238=FACE_BOUND ( 'NONE', #41888, .T. ) ;
#32239=ORIENTED_EDGE ( 'NONE', *, *, #22996, .F. ) ;
#32240=EDGE_CURVE ( 'NONE', #29294, #24657, #28671, .T. ) ;
#32241=DIRECTION ( 'NONE',  ( -0.000000000000000000, 1.000000000000000000, -0.000000000000000000 ) ) ;
#32243=ORIENTED_EDGE ( 'NONE', *, *, #43430, .T. ) ;
#32244=PLANE ( 'NONE',  #27117 ) ;
#32245=AXIS2_PLACEMENT_3D ( 'NONE', #18518, #34532, #13802 ) ;
#32247=CARTESIAN_POINT ( 'NONE',  ( 1.150725574412418739, -193.5000000000000000, -114.7252272087845881 ) ) ;
#32250=ORIENTED_EDGE ( 'NONE', *, *, #17667, .T. ) ;
#32251=ADVANCED_FACE ( 'NONE', ( #19756 ), #11867, .T. ) ;
#32257=FACE_OUTER_BOUND ( 'NONE', #20099, .T. ) ;
#32258=VECTOR ( 'NONE', #35245, 1000.000000000000000 ) ;
#32259=DIRECTION ( 'NONE',  ( -0.000000000000000000, 1.000000000000000000, -0.000000000000000000 ) ) ;
#32260=AXIS2_PLACEMENT_3D ( 'NONE', #17330, #48868, #33349 ) ;
#32261=AXIS2_PLACEMENT_3D ( 'NONE', #6152, #42390, #42904 ) ;
#32262=DIRECTION ( 'NONE',  ( 0.000000000000000000, -0.000000000000000000, -1.000000000000000000 ) ) ;
#32263=DIRECTION ( 'NONE',  ( -0.000000000000000000, 1.000000000000000000, -0.000000000000000000 ) ) ;
#32264=VERTEX_POINT ( 'NONE', #35789 ) ;
#32265=CARTESIAN_POINT ( 'NONE',  ( 14.94072793302542124, -175.3837268820161057, 107.7168604805791574 ) ) ;
#32266=ORIENTED_EDGE ( 'NONE', *, *, #19428, .F. ) ;
#32269=ORIENTED_EDGE ( 'NONE', *, *, #24677, .F. ) ;
#32270=DIRECTION ( 'NONE',  ( 0.000000000000000000, 0.000000000000000000, 1.000000000000000000 ) ) ;
#32272=EDGE_CURVE ( 'NONE', #5202, #32545, #302, .T. ) ;
#32274=CARTESIAN_POINT ( 'NONE',  ( -63.31390705753092618, -193.5000000000000000, 123.1094209424469312 ) ) ;
#32275=ORIENTED_EDGE ( 'NONE', *, *, #17495, .F. ) ;
#32278=AXIS2_PLACEMENT_3D ( 'NONE', #45544, #12431, #40798 ) ;
#32282=PLANE ( 'NONE',  #4706 ) ;
#32283=LINE ( 'NONE', #15780, #46543 ) ;
#32285=PLANE ( 'NONE',  #38321 ) ;
#32286=CARTESIAN_POINT ( 'NONE',  ( 30.50828161901817381, -183.6283474603465606, 96.88131563365350019 ) ) ;
#32287=EDGE_LOOP ( 'NONE', ( #860, #18208, #429, #2568 ) ) ;
#32288=EDGE_CURVE ( 'NONE', #1472, #32182, #10551, .T. ) ;
#32290=DIRECTION ( 'NONE',  ( 0.5586467658036594619, 0.000000000000000000, -0.8294056854501971054 ) ) ;
#32292=CARTESIAN_POINT ( 'NONE',  ( -137.2624501260119985, -177.1207230881787780, 87.99159897727967916 ) ) ;
#32293=VERTEX_POINT ( 'NONE', #44724 ) ;
#32294=EDGE_CURVE ( 'NONE', #346, #24932, #24479, .T. ) ;
#32296=DIRECTION ( 'NONE',  ( 0.1182731709213592358, 0.000000000000000000, 0.9929810960135178055 ) ) ;
#32297=VECTOR ( 'NONE', #40943, 1000.000000000000000 ) ;
#32298=VECTOR ( 'NONE', #41993, 1000.000000000000227 ) ;
#32299=CARTESIAN_POINT ( 'NONE',  ( -49.32472275501068282, -193.5000000000000000, 0.5338233779647895139 ) ) ;
#32300=CARTESIAN_POINT ( 'NONE',  ( 16.59365244519688787, -193.5000000000000000, -105.5544085257710947 ) ) ;
#32301=VERTEX_POINT ( 'NONE', #7928 ) ;
#32306=LINE ( 'NONE', #1295, #19484 ) ;
#32308=CARTESIAN_POINT ( 'NONE',  ( -48.24424070572786860, -183.6283474603465606, -0.9720229140804037549 ) ) ;
#32310=AXIS2_PLACEMENT_3D ( 'NONE', #9331, #17737, #25352 ) ;
#32312=AXIS2_PLACEMENT_3D ( 'NONE', #37596, #33892, #49680 ) ;
#32313=FACE_OUTER_BOUND ( 'NONE', #47001, .T. ) ;
#32314=VERTEX_POINT ( 'NONE', #16094 ) ;
#32315=AXIS2_PLACEMENT_3D ( 'NONE', #8367, #32008, #16001 ) ;
#32316=EDGE_LOOP ( 'NONE', ( #47409, #7291, #31666, #43561 ) ) ;
#32319=DIRECTION ( 'NONE',  ( -0.000000000000000000, 1.000000000000000000, -0.000000000000000000 ) ) ;
#32324=VECTOR ( 'NONE', #35268, 1000.000000000000000 ) ;
#32325=CARTESIAN_POINT ( 'NONE',  ( -161.2555905272864436, -193.5000000000000000, -53.91167979418489864 ) ) ;
#32326=VECTOR ( 'NONE', #5878, 999.9999999999998863 ) ;
#32327=ORIENTED_EDGE ( 'NONE', *, *, #42310, .T. ) ;
#32328=LINE ( 'NONE', #24211, #18839 ) ;
#32329=ORIENTED_EDGE ( 'NONE', *, *, #5919, .F. ) ;
#32330=CIRCLE ( 'NONE', #8044, 125.0000000000000000 ) ;
#32331=EDGE_CURVE ( 'NONE', #6669, #20596, #14732, .T. ) ;
#32333=EDGE_CURVE ( 'NONE', #9325, #8246, #20536, .T. ) ;
#32334=PLANE ( 'NONE',  #17458 ) ;
#32337=LINE ( 'NONE', #12630, #46661 ) ;
#32338=VERTEX_POINT ( 'NONE', #12909 ) ;
#32339=EDGE_CURVE ( 'NONE', #51600, #48065, #46654, .T. ) ;
#32341=DIRECTION ( 'NONE',  ( 0.000000000000000000, -1.000000000000000000, -0.000000000000000000 ) ) ;
#32344=EDGE_CURVE ( 'NONE', #8272, #2850, #32330, .T. ) ;
#32350=CARTESIAN_POINT ( 'NONE',  ( -48.47912675150885065, -189.7472609257535510, 6.938893903907228378E-15 ) ) ;
#32352=CARTESIAN_POINT ( 'NONE',  ( -171.4559849729830603, -183.6283474603465606, 22.39848972532371718 ) ) ;
#32355=CARTESIAN_POINT ( 'NONE',  ( -172.5669052183642123, -177.1207230881787780, 15.07392567185553567 ) ) ;
#32357=AXIS2_PLACEMENT_3D ( 'NONE', #12436, #3273, #4296 ) ;
#32360=CARTESIAN_POINT ( 'NONE',  ( -33.52607327456453135, -189.7472609257535510, -124.1024020384603119 ) ) ;
#32362=EDGE_CURVE ( 'NONE', #48442, #49029, #49195, .T. ) ;
#32363=CARTESIAN_POINT ( 'NONE',  ( -48.47912675150885065, -189.7472609257535510, 6.938893903907228378E-15 ) ) ;
#32364=DIRECTION ( 'NONE',  ( -0.000000000000000000, 1.000000000000000000, -0.000000000000000000 ) ) ;
#32365=EDGE_CURVE ( 'NONE', #48376, #47640, #37085, .T. ) ;
#32367=LINE ( 'NONE', #27906, #44200 ) ;
#32368=DIRECTION ( 'NONE',  ( 0.000000000000000000, 0.000000000000000000, -1.000000000000000000 ) ) ;
#32369=AXIS2_PLACEMENT_3D ( 'NONE', #49645, #16556, #1020 ) ;
#32370=CARTESIAN_POINT ( 'NONE',  ( -172.4792251663439231, -193.5000000000000000, 0.3215015308249614123 ) ) ;
#32372=LINE ( 'NONE', #28163, #13577 ) ;
#32374=VECTOR ( 'NONE', #14217, 1000.000000000000341 ) ;
#32375=AXIS2_PLACEMENT_3D ( 'NONE', #28089, #44135, #40192 ) ;
#32376=VERTEX_POINT ( 'NONE', #9762 ) ;
#32383=VERTEX_POINT ( 'NONE', #5050 ) ;
#32384=VECTOR ( 'NONE', #20340, 1000.000000000000000 ) ;
#32385=DIRECTION ( 'NONE',  ( 0.000000000000000000, 0.000000000000000000, 1.000000000000000000 ) ) ;
#32386=CIRCLE ( 'NONE', #37467, 125.0000000000000000 ) ;
#32387=DIRECTION ( 'NONE',  ( 0.000000000000000000, 0.000000000000000000, 1.000000000000000000 ) ) ;
#32389=EDGE_LOOP ( 'NONE', ( #8937, #32926, #23319, #40376 ) ) ;
#32391=AXIS2_PLACEMENT_3D ( 'NONE', #6187, #23250, #22982 ) ;
#32392=EDGE_CURVE ( 'NONE', #8865, #1307, #25271, .T. ) ;
#32394=LINE ( 'NONE', #16902, #4225 ) ;
#32395=DIRECTION ( 'NONE',  ( 0.000000000000000000, -0.000000000000000000, -1.000000000000000000 ) ) ;
#32397=FACE_OUTER_BOUND ( 'NONE', #9696, .T. ) ;
#32398=LINE ( 'NONE', #4552, #18858 ) ;
#32401=EDGE_CURVE ( 'NONE', #44533, #22822, #25521, .T. ) ;
#32402=EDGE_CURVE ( 'NONE', #22956, #19332, #41822, .T. ) ;
#32403=EDGE_CURVE ( 'NONE', #12964, #42609, #21327, .T. ) ;
#32406=DIRECTION ( 'NONE',  ( -0.000000000000000000, 1.000000000000000000, -0.000000000000000000 ) ) ;
#32409=ORIENTED_EDGE ( 'NONE', *, *, #17666, .T. ) ;
#32411=ORIENTED_EDGE ( 'NONE', *, *, #34906, .T. ) ;
#32413=CIRCLE ( 'NONE', #18173, 125.0000000000000000 ) ;
#32414=DIRECTION ( 'NONE',  ( -0.3482016354344059095, 0.000000000000000000, 0.9374196611341183427 ) ) ;
#32418=CIRCLE ( 'NONE', #45869, 125.0000000000000000 ) ;
#32419=FACE_OUTER_BOUND ( 'NONE', #30223, .T. ) ;
#32420=EDGE_LOOP ( 'NONE', ( #29561, #50985, #1112, #39872 ) ) ;
#32422=EDGE_CURVE ( 'NONE', #20596, #46251, #1350, .T. ) ;
#32425=CARTESIAN_POINT ( 'NONE',  ( 58.48829670243886625, -183.6283474603465606, -64.67588669375805921 ) ) ;
#32426=ORIENTED_EDGE ( 'NONE', *, *, #18064, .F. ) ;
#32427=FACE_BOUND ( 'NONE', #6244, .T. ) ;
#32429=EDGE_CURVE ( 'NONE', #51235, #35050, #48296, .T. ) ;
#32430=AXIS2_PLACEMENT_3D ( 'NONE', #20268, #7915, #28142 ) ;
#32432=ORIENTED_EDGE ( 'NONE', *, *, #28624, .F. ) ;
#32436=CYLINDRICAL_SURFACE ( 'NONE', #21486, 10.00000000000000000 ) ;
#32438=CARTESIAN_POINT ( 'NONE',  ( -117.6201219941651601, -189.7472609257535510, 104.1370384486469760 ) ) ;
#32439=AXIS2_PLACEMENT_3D ( 'NONE', #12998, #12489, #40856 ) ;
#32441=EDGE_CURVE ( 'NONE', #10598, #12446, #29459, .T. ) ;
#32442=ORIENTED_EDGE ( 'NONE', *, *, #842, .T. ) ;
#32443=LINE ( 'NONE', #45331, #987 ) ;
#32444=AXIS2_PLACEMENT_3D ( 'NONE', #42364, #27366, #34733 ) ;
#32445=VERTEX_POINT ( 'NONE', #8983 ) ;
#32452=CARTESIAN_POINT ( 'NONE',  ( 18.49541618049842384, -177.1207230881787780, 105.5434062319798159 ) ) ;
#32456=AXIS2_PLACEMENT_3D ( 'NONE', #35527, #7171, #30557 ) ;
#32457=ORIENTED_EDGE ( 'NONE', *, *, #27192, .T. ) ;
#32458=DIRECTION ( 'NONE',  ( 0.000000000000000000, -1.000000000000000000, 0.000000000000000000 ) ) ;
#32459=ORIENTED_EDGE ( 'NONE', *, *, #4182, .F. ) ;
#32460=LINE ( 'NONE', #11706, #45135 ) ;
#32462=VECTOR ( 'NONE', #19874, 1000.000000000000114 ) ;
#32465=ORIENTED_EDGE ( 'NONE', *, *, #44164, .F. ) ;
#32466=EDGE_LOOP ( 'NONE', ( #14199, #42702, #10424, #18595 ) ) ;
#32467=ORIENTED_EDGE ( 'NONE', *, *, #41249, .T. ) ;
#32468=LINE ( 'NONE', #23805, #39986 ) ;
#32471=VECTOR ( 'NONE', #34937, 1000.000000000000000 ) ;
#32473=VECTOR ( 'NONE', #31306, 1000.000000000000000 ) ;
#32475=CIRCLE ( 'NONE', #39184, 125.0000000000000000 ) ;
#32477=ORIENTED_EDGE ( 'NONE', *, *, #16714, .F. ) ;
#32478=EDGE_CURVE ( 'NONE', #20725, #22344, #29990, .T. ) ;
#32479=VECTOR ( 'NONE', #15344, 1000.000000000000114 ) ;
#32482=CARTESIAN_POINT ( 'NONE',  ( 7.859956736328458149, -193.5000000000000000, -111.5836353223468649 ) ) ;
#32483=VERTEX_POINT ( 'NONE', #42069 ) ;
#32487=CARTESIAN_POINT ( 'NONE',  ( -169.6719064342497632, -183.6283474603465606, 30.61552143554992256 ) ) ;
#32488=DIRECTION ( 'NONE',  ( 0.000000000000000000, 0.000000000000000000, 1.000000000000000000 ) ) ;
#32489=ORIENTED_EDGE ( 'NONE', *, *, #3906, .F. ) ;
#32490=CARTESIAN_POINT ( 'NONE',  ( -48.47912675150885065, -177.1207230881787780, 6.938893903907228378E-15 ) ) ;
#32491=VERTEX_POINT ( 'NONE', #34191 ) ;
#32493=CARTESIAN_POINT ( 'NONE',  ( -48.47912675150885065, -175.3837268820161057, 6.938893903907228378E-15 ) ) ;
#32494=VECTOR ( 'NONE', #32217, 1000.000000000000000 ) ;
#32497=CARTESIAN_POINT ( 'NONE',  ( -47.51449116960048968, -183.6283474603465606, -0.2635871660690578544 ) ) ;
#32498=DIRECTION ( 'NONE',  ( -0.000000000000000000, 1.000000000000000000, -0.000000000000000000 ) ) ;
#32500=CARTESIAN_POINT ( 'NONE',  ( -55.71438232577004612, -189.7472609257535510, -124.7904286264580662 ) ) ;
#32501=CARTESIAN_POINT ( 'NONE',  ( -85.14888725715768203, -193.5000000000000000, 119.5003291395398577 ) ) ;
#32502=ORIENTED_EDGE ( 'NONE', *, *, #41, .T. ) ;
#32504=DIRECTION ( 'NONE',  ( -0.1182731709213592358, 0.000000000000000000, -0.9929810960135178055 ) ) ;
#32505=ADVANCED_FACE ( 'NONE', ( #26292 ), #38640, .T. ) ;
#32506=LINE ( 'NONE', #35463, #38684 ) ;
#32507=FACE_BOUND ( 'NONE', #10094, .T. ) ;
#32508=VERTEX_POINT ( 'NONE', #50490 ) ;
#32509=AXIS2_PLACEMENT_3D ( 'NONE', #6997, #2536, #46956 ) ;
#32510=AXIS2_PLACEMENT_3D ( 'NONE', #41574, #50519, #38145 ) ;
#32512=VECTOR ( 'NONE', #36690, 1000.000000000000000 ) ;
#32514=VERTEX_POINT ( 'NONE', #47060 ) ;
#32515=CARTESIAN_POINT ( 'NONE',  ( -48.47912675150885065, -175.3837268820161057, 6.938893903907228378E-15 ) ) ;
#32516=VECTOR ( 'NONE', #16329, 1000.000000000000114 ) ;
#32518=AXIS2_PLACEMENT_3D ( 'NONE', #6369, #47345, #22396 ) ;
#32519=PLANE ( 'NONE',  #22635 ) ;
#32520=FACE_OUTER_BOUND ( 'NONE', #19269, .T. ) ;
#32521=CARTESIAN_POINT ( 'NONE',  ( 68.79964045138288498, -183.6283474603465606, 43.25148278810711844 ) ) ;
#32523=LINE ( 'NONE', #28569, #15172 ) ;
#32524=ORIENTED_EDGE ( 'NONE', *, *, #4144, .F. ) ;
#32526=FACE_OUTER_BOUND ( 'NONE', #43797, .T. ) ;
#32529=VERTEX_POINT ( 'NONE', #11034 ) ;
#32530=CYLINDRICAL_SURFACE ( 'NONE', #30095, 125.0000000000000000 ) ;
#32531=DIRECTION ( 'NONE',  ( -0.2635871660690783380, 0.000000000000000000, 0.9646355819083558547 ) ) ;
#32532=DIRECTION ( 'NONE',  ( -0.9266896074318370369, 0.000000000000000000, 0.3758275821142292306 ) ) ;
#32533=CIRCLE ( 'NONE', #13264, 125.0000000000000000 ) ;
#32534=EDGE_CURVE ( 'NONE', #33013, #3044, #10275, .T. ) ;
#32537=ORIENTED_EDGE ( 'NONE', *, *, #6568, .T. ) ;
#32539=LINE ( 'NONE', #44628, #36467 ) ;
#32541=VECTOR ( 'NONE', #41631, 1000.000000000000000 ) ;
#32542=ORIENTED_EDGE ( 'NONE', *, *, #25012, .F. ) ;
#32544=CARTESIAN_POINT ( 'NONE',  ( -48.53836737940255119, -193.5000000000000000, -0.9982437317643153563 ) ) ;
#32545=VERTEX_POINT ( 'NONE', #50744 ) ;
#32547=EDGE_LOOP ( 'NONE', ( #2975, #35378, #21394, #24650 ) ) ;
#32549=DIRECTION ( 'NONE',  ( 0.000000000000000000, 0.000000000000000000, 1.000000000000000000 ) ) ;
#32550=ORIENTED_EDGE ( 'NONE', *, *, #35940, .T. ) ;
#32551=CARTESIAN_POINT ( 'NONE',  ( -48.47912675150885065, -189.7472609257535510, 6.938893903907228378E-15 ) ) ;
#32556=DIRECTION ( 'NONE',  ( -0.000000000000000000, 1.000000000000000000, -0.000000000000000000 ) ) ;
#32557=DIRECTION ( 'NONE',  ( 0.8124868780056825335, 0.000000000000000000, -0.5829794791144703447 ) ) ;
#32559=LINE ( 'NONE', #25201, #341 ) ;
#32560=DIRECTION ( 'NONE',  ( 0.6068001458185834363, 0.000000000000000000, 0.7948544414133608127 ) ) ;
#32561=DIRECTION ( 'NONE',  ( 0.000000000000000000, -0.000000000000000000, -1.000000000000000000 ) ) ;
#32564=CARTESIAN_POINT ( 'NONE',  ( 57.66105628977221897, -193.5000000000000000, 66.02470404298190942 ) ) ;
#32566=LINE ( 'NONE', #33082, #42464 ) ;
#32569=AXIS2_PLACEMENT_3D ( 'NONE', #27110, #30539, #23192 ) ;
#32571=AXIS2_PLACEMENT_3D ( 'NONE', #26205, #21507, #2317 ) ;
#32572=DIRECTION ( 'NONE',  ( 0.000000000000000000, -1.000000000000000000, 0.000000000000000000 ) ) ;
#32573=VECTOR ( 'NONE', #4813, 999.9999999999998863 ) ;
#32575=FACE_OUTER_BOUND ( 'NONE', #14328, .T. ) ;
#32576=ORIENTED_EDGE ( 'NONE', *, *, #39465, .F. ) ;
#32577=ORIENTED_EDGE ( 'NONE', *, *, #16934, .F. ) ;
#32578=ORIENTED_EDGE ( 'NONE', *, *, #18255, .F. ) ;
#32579=CIRCLE ( 'NONE', #42636, 125.0000000000000000 ) ;
#32582=CARTESIAN_POINT ( 'NONE',  ( -138.3705904895685705, -177.1207230881787780, -86.85922373029296750 ) ) ;
#32584=EDGE_LOOP ( 'NONE', ( #19664, #26266, #42155, #45305 ) ) ;
#32586=CARTESIAN_POINT ( 'NONE',  ( -168.3100285466275636, -189.7472609257535510, -31.88354567335001377 ) ) ;
#32587=DIRECTION ( 'NONE',  ( 0.000000000000000000, 0.000000000000000000, 1.000000000000000000 ) ) ;
#32588=VERTEX_POINT ( 'NONE', #22628 ) ;
#32590=CARTESIAN_POINT ( 'NONE',  ( -135.4449840867448813, -189.7472609257535510, -88.39086586114741806 ) ) ;
#32591=ADVANCED_FACE ( 'NONE', ( #2641 ), #30756, .T. ) ;
#32592=VERTEX_POINT ( 'NONE', #3164 ) ;
#32593=VERTEX_POINT ( 'NONE', #10524 ) ;
#32594=DIRECTION ( 'NONE',  ( -0.000000000000000000, 1.000000000000000000, -0.000000000000000000 ) ) ;
#32595=EDGE_CURVE ( 'NONE', #23874, #30234, #34949, .T. ) ;
#32597=DIRECTION ( 'NONE',  ( 0.000000000000000000, 1.000000000000000000, 0.000000000000000000 ) ) ;
#32598=LINE ( 'NONE', #24202, #5105 ) ;
#32599=PRODUCT_DEFINITION_FORMATION_WITH_SPECIFIED_SOURCE ( 'ANY', '', #49932, .NOT_KNOWN. ) ;
#32600=CARTESIAN_POINT ( 'NONE',  ( -169.6719064342497916, -183.6283474603465606, 30.61552143554989414 ) ) ;
#32603=AXIS2_PLACEMENT_3D ( 'NONE', #36895, #17182, #48983 ) ;
#32604=EDGE_CURVE ( 'NONE', #40906, #36985, #18428, .T. ) ;
#32606=DIRECTION ( 'NONE',  ( 0.000000000000000000, 1.000000000000000000, 0.000000000000000000 ) ) ;
#32607=ORIENTED_EDGE ( 'NONE', *, *, #6385, .F. ) ;
#32611=ORIENTED_EDGE ( 'NONE', *, *, #27507, .F. ) ;
#32612=CARTESIAN_POINT ( 'NONE',  ( -49.47517659412407198, -193.5000000000000000, 0.08879589532293177823 ) ) ;
#32613=DIRECTION ( 'NONE',  ( -0.5586467658036535777, 0.000000000000000000, 0.8294056854502011022 ) ) ;
#32614=CARTESIAN_POINT ( 'NONE',  ( -47.66663987350317910, -183.6283474603465606, 0.5829794791144832233 ) ) ;
#32616=EDGE_LOOP ( 'NONE', ( #39367, #19802, #9231, #40629 ) ) ;
#32617=CIRCLE ( 'NONE', #6605, 125.0000000000000000 ) ;
#32619=FACE_OUTER_BOUND ( 'NONE', #20992, .T. ) ;
#32620=DIRECTION ( 'NONE',  ( 0.000000000000000000, 1.000000000000000000, 0.000000000000000000 ) ) ;
#32622=EDGE_CURVE ( 'NONE', #26442, #9007, #43302, .T. ) ;
#32625=PLANE ( 'NONE',  #49207 ) ;
#32626=VERTEX_POINT ( 'NONE', #6606 ) ;
#32627=CARTESIAN_POINT ( 'NONE',  ( -167.9436818089035626, -183.6283474603465606, 36.78613984830037253 ) ) ;
#32629=ORIENTED_EDGE ( 'NONE', *, *, #6639, .T. ) ;
#32630=LINE ( 'NONE', #24232, #40868 ) ;
#32633=DIRECTION ( 'NONE',  ( 0.000000000000000000, 0.000000000000000000, -1.000000000000000000 ) ) ;
#32634=DIRECTION ( 'NONE',  ( 0.000000000000000000, 0.000000000000000000, -1.000000000000000000 ) ) ;
#32635=DIRECTION ( 'NONE',  ( 0.000000000000000000, -0.000000000000000000, -1.000000000000000000 ) ) ;
#32636=PLANE ( 'NONE',  #1435 ) ;
#32637=DIRECTION ( 'NONE',  ( 0.000000000000000000, -1.000000000000000000, 0.000000000000000000 ) ) ;
#32639=CYLINDRICAL_SURFACE ( 'NONE', #22799, 124.9999999999999858 ) ;
#32642=VERTEX_POINT ( 'NONE', #7378 ) ;
#32643=AXIS2_PLACEMENT_3D ( 'NONE', #17560, #21485, #24639 ) ;
#32645=EDGE_CURVE ( 'NONE', #16943, #9203, #18141, .T. ) ;
#32646=ADVANCED_FACE ( 'NONE', ( #10793 ), #23400, .T. ) ;
#32647=LINE ( 'NONE', #585, #40021 ) ;
#32648=DIRECTION ( 'NONE',  ( 0.000000000000000000, -1.000000000000000000, -0.000000000000000000 ) ) ;
#32649=VERTEX_POINT ( 'NONE', #46294 ) ;
#32651=VERTEX_POINT ( 'NONE', #46807 ) ;
#32652=EDGE_LOOP ( 'NONE', ( #13258, #47324, #1901, #28880 ) ) ;
#32653=PLANE ( 'NONE',  #27506 ) ;
#32654=EDGE_CURVE ( 'NONE', #21416, #20906, #34445, .T. ) ;
#32655=DIRECTION ( 'NONE',  ( 0.000000000000000000, 1.000000000000000000, 0.000000000000000000 ) ) ;
#32658=ORIENTED_EDGE ( 'NONE', *, *, #46606, .F. ) ;
#32659=EDGE_CURVE ( 'NONE', #39601, #31150, #34697, .T. ) ;
#32660=CIRCLE ( 'NONE', #41058, 125.0000000000000000 ) ;
#32663=CARTESIAN_POINT ( 'NONE',  ( -66.46933728415693565, -177.1207230881787780, 122.6885491605231522 ) ) ;
#32665=ADVANCED_FACE ( 'NONE', ( #19440 ), #35462, .F. ) ;
#32666=CARTESIAN_POINT ( 'NONE',  ( -31.47951320919342777, -183.6283474603465606, -122.8300162461135301 ) ) ;
#32667=CARTESIAN_POINT ( 'NONE',  ( -152.3176060415594861, -183.6283474603465606, -69.58857822034966034 ) ) ;
#32669=LINE ( 'NONE', #36611, #48188 ) ;
#32671=EDGE_LOOP ( 'NONE', ( #2178, #11351, #49654, #9521 ) ) ;
#32672=CARTESIAN_POINT ( 'NONE',  ( -160.9694636715425702, -189.7472609257535510, 54.50618404931039862 ) ) ;
#32673=DIRECTION ( 'NONE',  ( 0.000000000000000000, 0.000000000000000000, 1.000000000000000000 ) ) ;
#32674=CARTESIAN_POINT ( 'NONE',  ( 10.73478887071927623, -183.6283474603465606, -110.0850225811106924 ) ) ;
#32675=VERTEX_POINT ( 'NONE', #48622 ) ;
#32676=ORIENTED_EDGE ( 'NONE', *, *, #41095, .F. ) ;
#32677=DIRECTION ( 'NONE',  ( 0.000000000000000000, 0.000000000000000000, 1.000000000000000000 ) ) ;
#32681=DIRECTION ( 'NONE',  ( 0.000000000000000000, -0.000000000000000000, -1.000000000000000000 ) ) ;
#32683=DIRECTION ( 'NONE',  ( 0.000000000000000000, 1.000000000000000000, -0.000000000000000000 ) ) ;
#32684=ORIENTED_EDGE ( 'NONE', *, *, #39240, .T. ) ;
#32688=ORIENTED_EDGE ( 'NONE', *, *, #39706, .F. ) ;
#32689=DIRECTION ( 'NONE',  ( 0.4031234292879600778, 0.000000000000000000, 0.9151456172430237901 ) ) ;
#32692=VERTEX_POINT ( 'NONE', #15791 ) ;
#32693=CARTESIAN_POINT ( 'NONE',  ( 20.66186849114819069, -175.3837268820161057, -104.1370384486465070 ) ) ;
#32695=CYLINDRICAL_SURFACE ( 'NONE', #24058, 124.9999999999999858 ) ;
#32696=DIRECTION ( 'NONE',  ( 0.000000000000000000, -1.000000000000000000, -0.000000000000000000 ) ) ;
#32697=AXIS2_PLACEMENT_3D ( 'NONE', #18419, #50735, #21847 ) ;
#32698=EDGE_LOOP ( 'NONE', ( #21679, #45562, #5973, #49823 ) ) ;
#32699=CARTESIAN_POINT ( 'NONE',  ( 1.755575411425451593, -189.7472609257535510, 114.4616734920527108 ) ) ;
#32700=ORIENTED_EDGE ( 'NONE', *, *, #11850, .F. ) ;
#32701=ADVANCED_FACE ( 'NONE', ( #4204 ), #16283, .T. ) ;
#32703=DIRECTION ( 'NONE',  ( 0.000000000000000000, 0.000000000000000000, 1.000000000000000000 ) ) ;
#32704=DIRECTION ( 'NONE',  ( 0.000000000000000000, 0.000000000000000000, -1.000000000000000000 ) ) ;
#32705=ORIENTED_EDGE ( 'NONE', *, *, #24358, .T. ) ;
#32706=EDGE_CURVE ( 'NONE', #39306, #21525, #44412, .T. ) ;
#32707=EDGE_LOOP ( 'NONE', ( #40437, #5212, #41374, #46266 ) ) ;
#32708=EDGE_CURVE ( 'NONE', #34125, #50975, #24850, .T. ) ;
#32711=EDGE_CURVE ( 'NONE', #51319, #11294, #40775, .T. ) ;
#32713=EDGE_LOOP ( 'NONE', ( #21510, #36152, #36670, #29280 ) ) ;
#32714=AXIS2_PLACEMENT_3D ( 'NONE', #15804, #48104, #12075 ) ;
#32719=DIRECTION ( 'NONE',  ( -0.8294056854502090959, 0.000000000000000000, 0.5586467658036415873 ) ) ;
#32720=ADVANCED_FACE ( 'NONE', ( #7620 ), #3945, .F. ) ;
#32721=CARTESIAN_POINT ( 'NONE',  ( -32.87124591993210743, -193.5000000000000000, 124.0217483183788119 ) ) ;
#32722=FACE_OUTER_BOUND ( 'NONE', #45528, .T. ) ;
#32723=EDGE_LOOP ( 'NONE', ( #48945, #42238, #22478, #43229 ) ) ;
#32724=ORIENTED_EDGE ( 'NONE', *, *, #45780, .T. ) ;
#32726=ORIENTED_EDGE ( 'NONE', *, *, #33678, .F. ) ;
#32727=LINE ( 'NONE', #48247, #48419 ) ;
#32733=ORIENTED_EDGE ( 'NONE', *, *, #13500, .F. ) ;
#32736=AXIS2_PLACEMENT_3D ( 'NONE', #3506, #7203, #4285 ) ;
#32737=CIRCLE ( 'NONE', #10089, 125.0000000000000000 ) ;
#32738=VERTEX_POINT ( 'NONE', #16034 ) ;
#32739=DIRECTION ( 'NONE',  ( -0.000000000000000000, 1.000000000000000000, -0.000000000000000000 ) ) ;
#32741=DIRECTION ( 'NONE',  ( 0.1476465640024851034, 0.000000000000000000, -0.9890401873221634776 ) ) ;
#32742=ORIENTED_EDGE ( 'NONE', *, *, #46148, .T. ) ;
#32744=CARTESIAN_POINT ( 'NONE',  ( -48.77118352214583297, -193.5000000000000000, 0.9564009842765270886 ) ) ;
#32745=LINE ( 'NONE', #694, #8700 ) ;
#32747=VERTEX_POINT ( 'NONE', #48084 ) ;
#32749=VERTEX_POINT ( 'NONE', #12062 ) ;
#32750=EDGE_CURVE ( 'NONE', #41700, #794, #21521, .T. ) ;
#32751=EDGE_CURVE ( 'NONE', #33603, #34940, #36243, .T. ) ;
#32753=FACE_OUTER_BOUND ( 'NONE', #49923, .T. ) ;
#32755=DIRECTION ( 'NONE',  ( 0.000000000000000000, 0.000000000000000000, 1.000000000000000000 ) ) ;
#32756=CARTESIAN_POINT ( 'NONE',  ( 19.33815737959698566, -183.6283474603465606, 105.0038855142078091 ) ) ;
#32757=CARTESIAN_POINT ( 'NONE',  ( -173.0563034899574859, -193.5000000000000000, -10.27263529369817618 ) ) ;
#32758=DIRECTION ( 'NONE',  ( -0.000000000000000000, 1.000000000000000000, -0.000000000000000000 ) ) ;
#32759=CARTESIAN_POINT ( 'NONE',  ( 6.443011874827243801, -193.5000000000000000, 112.2878385610370771 ) ) ;
#32760=LINE ( 'NONE', #33279, #22022 ) ;
#32761=VERTEX_POINT ( 'NONE', #239 ) ;
#32762=DIRECTION ( 'NONE',  ( -0.000000000000000000, -1.000000000000000000, 0.000000000000000000 ) ) ;
#32764=CARTESIAN_POINT ( 'NONE',  ( -167.8725343822893024, -193.5000000000000000, 33.48461921608603120 ) ) ;
#32765=FACE_BOUND ( 'NONE', #44599, .T. ) ;
#32767=FACE_OUTER_BOUND ( 'NONE', #42446, .T. ) ;
#32769=CARTESIAN_POINT ( 'NONE',  ( -30.48891621885993430, -177.1207230881787780, -122.6885491605229959 ) ) ;
#32770=ADVANCED_FACE ( 'NONE', ( #24426 ), #4458, .T. ) ;
#32771=EDGE_LOOP ( 'NONE', ( #35742, #19627, #18714, #41575 ) ) ;
#32772=EDGE_CURVE ( 'NONE', #18907, #18264, #13940, .T. ) ;
#32774=ORIENTED_EDGE ( 'NONE', *, *, #21853, .T. ) ;
#32776=EDGE_CURVE ( 'NONE', #1404, #47168, #24956, .T. ) ;
#32777=VECTOR ( 'NONE', #32108, 1000.000000000000000 ) ;
#32779=CARTESIAN_POINT ( 'NONE',  ( 55.10060313344061456, -177.1207230881787780, 68.17212999877223467 ) ) ;
#32781=CARTESIAN_POINT ( 'NONE',  ( -98.31070548515602070, -193.5000000000000000, -113.5465278748093283 ) ) ;
#32782=VERTEX_POINT ( 'NONE', #8912 ) ;
#32787=DIRECTION ( 'NONE',  ( 0.6528221181905227155, 0.000000000000000000, -0.7575112421616191360 ) ) ;
#32792=CARTESIAN_POINT ( 'NONE',  ( 76.01188277843579044, -175.3837268820161057, 11.26891947860284482 ) ) ;
#32794=DIRECTION ( 'NONE',  ( 0.3482016354343928088, 0.000000000000000000, 0.9374196611341231167 ) ) ;
#32795=CARTESIAN_POINT ( 'NONE',  ( -96.65280530915693191, -193.5000000000000000, -115.3442529744087466 ) ) ;
#32802=VERTEX_POINT ( 'NONE', #31064 ) ;
#32803=AXIS2_PLACEMENT_3D ( 'NONE', #31073, #35023, #7929 ) ;
#32804=ORIENTED_EDGE ( 'NONE', *, *, #30121, .F. ) ;
#32805=DIRECTION ( 'NONE',  ( 0.000000000000000000, 0.000000000000000000, 1.000000000000000000 ) ) ;
#32806=DIRECTION ( 'NONE',  ( -0.000000000000000000, 1.000000000000000000, -0.000000000000000000 ) ) ;
#32809=CARTESIAN_POINT ( 'NONE',  ( 42.89728982752368580, -189.7472609257535510, 83.82333043185313670 ) ) ;
#32811=AXIS2_PLACEMENT_3D ( 'NONE', #27594, #19697, #35730 ) ;
#32813=DIRECTION ( 'NONE',  ( 0.9890401873221623674, 0.000000000000000000, 0.1476465640024917925 ) ) ;
#32815=FACE_OUTER_BOUND ( 'NONE', #51915, .T. ) ;
#32818=CARTESIAN_POINT ( 'NONE',  ( -87.88805327685028601, -193.5000000000000000, 117.5715283571807106 ) ) ;
#32819=FACE_OUTER_BOUND ( 'NONE', #46974, .T. ) ;
#32820=CARTESIAN_POINT ( 'NONE',  ( -158.6498865914718408, -183.6283474603465606, 56.90809649257569447 ) ) ;
#32825=AXIS2_PLACEMENT_3D ( 'NONE', #10050, #9271, #16898 ) ;
#32827=CARTESIAN_POINT ( 'NONE',  ( -48.65601702663141737, -175.3837268820161057, -0.9842305779475923888 ) ) ;
#32829=ORIENTED_EDGE ( 'NONE', *, *, #8860, .F. ) ;
#32830=ADVANCED_FACE ( 'NONE', ( #27113 ), #38940, .F. ) ;
#32831=ORIENTED_EDGE ( 'NONE', *, *, #36868, .F. ) ;
#32833=DIRECTION ( 'NONE',  ( -0.000000000000000000, 1.000000000000000000, -0.000000000000000000 ) ) ;
#32835=CARTESIAN_POINT ( 'NONE',  ( -69.59623518921149810, -193.5000000000000000, 122.1886788576024117 ) ) ;
#32836=DIRECTION ( 'NONE',  ( 0.000000000000000000, 0.000000000000000000, 1.000000000000000000 ) ) ;
#32837=VECTOR ( 'NONE', #17780, 1000.000000000000000 ) ;
#32838=EDGE_LOOP ( 'NONE', ( #47025, #11213, #1693, #38533 ) ) ;
#32846=EDGE_CURVE ( 'NONE', #42603, #23845, #3462, .T. ) ;
#32848=AXIS2_PLACEMENT_3D ( 'NONE', #3031, #44012, #35597 ) ;
#32854=DIRECTION ( 'NONE',  ( 0.000000000000000000, 1.000000000000000000, 0.000000000000000000 ) ) ;
#32855=EDGE_LOOP ( 'NONE', ( #26014, #33482, #50796, #36898 ) ) ;
#32856=DIRECTION ( 'NONE',  ( 0.000000000000000000, 0.000000000000000000, 1.000000000000000000 ) ) ;
#32858=VERTEX_POINT ( 'NONE', #34489 ) ;
#32859=EDGE_CURVE ( 'NONE', #16210, #23109, #42891, .T. ) ;
#32861=CARTESIAN_POINT ( 'NONE',  ( 32.34187644556187990, -193.5000000000000000, 94.04236105995857997 ) ) ;
#32862=DIRECTION ( 'NONE',  ( 0.000000000000000000, -1.000000000000000000, 0.000000000000000000 ) ) ;
#32863=EDGE_LOOP ( 'NONE', ( #44333, #1499, #3867, #12951 ) ) ;
#32864=DIRECTION ( 'NONE',  ( 0.9995608365087944591, 0.000000000000000000, -0.02963332782255633305 ) ) ;
#32867=EDGE_CURVE ( 'NONE', #5084, #28167, #8904, .T. ) ;
#32869=CARTESIAN_POINT ( 'NONE',  ( -49.47517659412407198, -183.6283474603465606, 0.08879589532293177823 ) ) ;
#32871=CARTESIAN_POINT ( 'NONE',  ( -48.47912675150885065, -183.6283474603465606, 6.938893903907228378E-15 ) ) ;
#32872=EDGE_LOOP ( 'NONE', ( #10418, #51303, #47656, #6224 ) ) ;
#32873=PLANE ( 'NONE',  #34035 ) ;
#32876=CARTESIAN_POINT ( 'NONE',  ( -165.5546359831674295, -183.6283474603465606, 43.79868877201490562 ) ) ;
#32877=VERTEX_POINT ( 'NONE', #51069 ) ;
#32878=DIRECTION ( 'NONE',  ( 0.6965510290629932655, 0.000000000000000000, 0.7175072570443347120 ) ) ;
#32879=CARTESIAN_POINT ( 'NONE',  ( -34.51936650669028239, -189.7472609257535510, -124.2180546213278092 ) ) ;
#32880=LINE ( 'NONE', #24751, #39478 ) ;
#32883=EDGE_CURVE ( 'NONE', #21993, #29517, #51313, .T. ) ;
#32885=EDGE_CURVE ( 'NONE', #9853, #33172, #30292, .T. ) ;
#32886=CARTESIAN_POINT ( 'NONE',  ( -92.16375985330356002, -193.5000000000000000, 117.1181148702521710 ) ) ;
#32887=CIRCLE ( 'NONE', #1877, 125.0000000000000000 ) ;
#32889=VECTOR ( 'NONE', #11904, 1000.000000000000000 ) ;
#32890=DIRECTION ( 'NONE',  ( -0.000000000000000000, 1.000000000000000000, -0.000000000000000000 ) ) ;
#32891=DIRECTION ( 'NONE',  ( -0.000000000000000000, 1.000000000000000000, -0.000000000000000000 ) ) ;
#32892=ORIENTED_EDGE ( 'NONE', *, *, #32203, .F. ) ;
#32893=ORIENTED_EDGE ( 'NONE', *, *, #36556, .T. ) ;
#32894=CARTESIAN_POINT ( 'NONE',  ( -22.44626007086656472, -183.6283474603465606, 122.2591094863196872 ) ) ;
#32896=VERTEX_POINT ( 'NONE', #3223 ) ;
#32897=ORIENTED_EDGE ( 'NONE', *, *, #28955, .F. ) ;
#32898=EDGE_LOOP ( 'NONE', ( #40289, #42276, #14624, #10653 ) ) ;
#32899=ADVANCED_FACE ( 'NONE', ( #26348 ), #19253, .T. ) ;
#32900=DIRECTION ( 'NONE',  ( 0.9266896074318343723, 0.000000000000000000, -0.3758275821142357809 ) ) ;
#32901=VECTOR ( 'NONE', #33592, 1000.000000000000000 ) ;
#32903=CARTESIAN_POINT ( 'NONE',  ( -49.13194886969938580, -175.3837268820161057, 0.7575112421616214675 ) ) ;
#32904=EDGE_LOOP ( 'NONE', ( #2618, #42567, #6295, #42163 ) ) ;
#32905=EDGE_CURVE ( 'NONE', #32592, #33172, #29869, .T. ) ;
#32907=AXIS2_PLACEMENT_3D ( 'NONE', #49658, #2348, #42795 ) ;
#32908=FACE_OUTER_BOUND ( 'NONE', #36329, .T. ) ;
#32909=DIRECTION ( 'NONE',  ( -0.6965510290629882695, 0.000000000000000000, -0.7175072570443395970 ) ) ;
#32910=ORIENTED_EDGE ( 'NONE', *, *, #17309, .T. ) ;
#32911=FACE_OUTER_BOUND ( 'NONE', #42295, .T. ) ;
#32913=CARTESIAN_POINT ( 'NONE',  ( -63.43218022845228887, -175.3837268820161057, 124.1024020384604540 ) ) ;
#32914=ORIENTED_EDGE ( 'NONE', *, *, #12121, .F. ) ;
#32915=DIRECTION ( 'NONE',  ( -0.6068001458186002006, 0.000000000000000000, 0.7948544414133481562 ) ) ;
#32916=DIRECTION ( 'NONE',  ( 0.000000000000000000, 0.000000000000000000, 1.000000000000000000 ) ) ;
#32917=DIRECTION ( 'NONE',  ( -0.000000000000000000, 1.000000000000000000, -0.000000000000000000 ) ) ;
#32919=CIRCLE ( 'NONE', #11129, 9.999999999999994671 ) ;
#32921=VECTOR ( 'NONE', #16218, 1000.000000000000000 ) ;
#32923=AXIS2_PLACEMENT_3D ( 'NONE', #5673, #22199, #21942 ) ;
#32924=PLANE ( 'NONE',  #1321 ) ;
#32925=CARTESIAN_POINT ( 'NONE',  ( -47.55243714407702527, -183.6283474603465606, 0.3758275821142491591 ) ) ;
#32926=ORIENTED_EDGE ( 'NONE', *, *, #537, .F. ) ;
#32927=DIRECTION ( 'NONE',  ( 0.000000000000000000, -1.000000000000000000, 0.000000000000000000 ) ) ;
#32929=EDGE_CURVE ( 'NONE', #35901, #15345, #11342, .T. ) ;
#32930=EDGE_CURVE ( 'NONE', #12684, #22789, #7431, .T. ) ;
#32931=ORIENTED_EDGE ( 'NONE', *, *, #43639, .T. ) ;
#32933=LINE ( 'NONE', #29261, #41641 ) ;
#32935=DIRECTION ( 'NONE',  ( -0.6965510290630033685, 0.000000000000000000, 0.7175072570443249420 ) ) ;
#32936=VERTEX_POINT ( 'NONE', #10326 ) ;
#32937=DIRECTION ( 'NONE',  ( -0.000000000000000000, 1.000000000000000000, -0.000000000000000000 ) ) ;
#32938=DIRECTION ( 'NONE',  ( 0.000000000000000000, -1.000000000000000000, 0.000000000000000000 ) ) ;
#32939=ORIENTED_EDGE ( 'NONE', *, *, #44336, .T. ) ;
#32940=CIRCLE ( 'NONE', #21218, 124.9999999999999858 ) ;
#32941=CARTESIAN_POINT ( 'NONE',  ( 46.01898237923985846, -177.1207230881787780, -81.82363577055903647 ) ) ;
#32945=LINE ( 'NONE', #12711, #38342 ) ;
#32946=EDGE_CURVE ( 'NONE', #44462, #22776, #10577, .T. ) ;
#32947=VECTOR ( 'NONE', #18175, 1000.000000000000000 ) ;
#32948=ORIENTED_EDGE ( 'NONE', *, *, #16894, .T. ) ;
#32949=PLANE ( 'NONE',  #6030 ) ;
#32951=ORIENTED_EDGE ( 'NONE', *, *, #48112, .T. ) ;
#32952=EDGE_CURVE ( 'NONE', #12133, #12684, #18730, .T. ) ;
#32953=LINE ( 'NONE', #25587, #14294 ) ;
#32954=PLANE ( 'NONE',  #22814 ) ;
#32956=EDGE_CURVE ( 'NONE', #31485, #728, #42472, .T. ) ;
#32957=ORIENTED_EDGE ( 'NONE', *, *, #23812, .T. ) ;
#32958=LINE ( 'NONE', #5127, #47525 ) ;
#32959=VECTOR ( 'NONE', #6806, 1000.000000000000000 ) ;
#32960=DIRECTION ( 'NONE',  ( 0.000000000000000000, 1.000000000000000000, 0.000000000000000000 ) ) ;
#32962=VECTOR ( 'NONE', #51401, 1000.000000000000000 ) ;
#32963=AXIS2_PLACEMENT_3D ( 'NONE', #39665, #46816, #23153 ) ;
#32964=VERTEX_POINT ( 'NONE', #7667 ) ;
#32966=ORIENTED_EDGE ( 'NONE', *, *, #50570, .T. ) ;
#32967=CARTESIAN_POINT ( 'NONE',  ( -165.7578939544008847, -177.1207230881787780, -43.25148278810626579 ) ) ;
#32972=ORIENTED_EDGE ( 'NONE', *, *, #4766, .T. ) ;
#32973=ORIENTED_EDGE ( 'NONE', *, *, #45549, .F. ) ;
#32974=ORIENTED_EDGE ( 'NONE', *, *, #46778, .T. ) ;
#32976=CARTESIAN_POINT ( 'NONE',  ( -145.0195698084541505, -189.7472609257535510, 79.40367028273128369 ) ) ;
#32981=VERTEX_POINT ( 'NONE', #20017 ) ;
#32982=VECTOR ( 'NONE', #25598, 1000.000000000000000 ) ;
#32983=EDGE_LOOP ( 'NONE', ( #33055, #33782, #45657, #35431 ) ) ;
#32984=DIRECTION ( 'NONE',  ( 0.000000000000000000, 0.000000000000000000, 1.000000000000000000 ) ) ;
#32986=ORIENTED_EDGE ( 'NONE', *, *, #51886, .T. ) ;
#32989=FACE_OUTER_BOUND ( 'NONE', #36094, .T. ) ;
#32991=EDGE_CURVE ( 'NONE', #13340, #21757, #31848, .T. ) ;
#32993=ADVANCED_FACE ( 'NONE', ( #15562 ), #32625, .T. ) ;
#32994=ADVANCED_FACE ( 'NONE', ( #43925 ), #12639, .T. ) ;
#32997=FACE_OUTER_BOUND ( 'NONE', #24063, .T. ) ;
#32998=AXIS2_PLACEMENT_3D ( 'NONE', #28152, #25018, #36304 ) ;
#33000=EDGE_CURVE ( 'NONE', #2282, #19065, #33250, .T. ) ;
#33001=VERTEX_POINT ( 'NONE', #47886 ) ;
#33002=DIRECTION ( 'NONE',  ( 0.7765238627180349740, 0.000000000000000000, 0.6300878435817203194 ) ) ;
#33003=AXIS2_PLACEMENT_3D ( 'NONE', #35529, #47651, #27391 ) ;
#33005=EDGE_CURVE ( 'NONE', #17543, #14548, #48137, .T. ) ;
#33007=EDGE_CURVE ( 'NONE', #46248, #33039, #21475, .T. ) ;
#33008=CARTESIAN_POINT ( 'NONE',  ( -114.1105527140175440, -183.6283474603465606, 106.3838142112217326 ) ) ;
#33009=DIRECTION ( 'NONE',  ( 0.000000000000000000, 0.000000000000000000, -1.000000000000000000 ) ) ;
#33011=AXIS2_PLACEMENT_3D ( 'NONE', #23014, #2526, #3035 ) ;
#33012=ADVANCED_FACE ( 'NONE', ( #48402 ), #35514, .T. ) ;
#33013=VERTEX_POINT ( 'NONE', #23693 ) ;
#33014=PLANE ( 'NONE',  #23011 ) ;
#33015=DIRECTION ( 'NONE',  ( 0.9929810960135178055, 0.000000000000000000, -0.1182731709213592358 ) ) ;
#33016=EDGE_CURVE ( 'NONE', #9665, #50565, #23952, .T. ) ;
#33017=CARTESIAN_POINT ( 'NONE',  ( 68.79964045138289919, -177.1207230881787780, 43.25148278810711133 ) ) ;
#33018=FACE_BOUND ( 'NONE', #9773, .T. ) ;
#33019=VERTEX_POINT ( 'NONE', #4249 ) ;
#33020=EDGE_CURVE ( 'NONE', #6834, #47944, #11439, .T. ) ;
#33021=CARTESIAN_POINT ( 'NONE',  ( -94.25732089370191602, -177.1207230881787780, 116.3157639405754935 ) ) ;
#33022=ORIENTED_EDGE ( 'NONE', *, *, #1355, .F. ) ;
#33025=EDGE_CURVE ( 'NONE', #26931, #12201, #28144, .T. ) ;
#33026=ORIENTED_EDGE ( 'NONE', *, *, #47370, .F. ) ;
#33027=DIRECTION ( 'NONE',  ( -0.3758275821142488260, 0.000000000000000000, 0.9266896074318291543 ) ) ;
#33028=ORIENTED_EDGE ( 'NONE', *, *, #39410, .F. ) ;
#33034=ORIENTED_EDGE ( 'NONE', *, *, #12656, .T. ) ;
#33035=DIRECTION ( 'NONE',  ( -0.000000000000000000, 1.000000000000000000, -0.000000000000000000 ) ) ;
#33036=AXIS2_PLACEMENT_3D ( 'NONE', #42633, #18978, #42363 ) ;
#33038=VERTEX_POINT ( 'NONE', #24739 ) ;
#33039=VERTEX_POINT ( 'NONE', #36554 ) ;
#33040=ORIENTED_EDGE ( 'NONE', *, *, #19845, .T. ) ;
#33042=FACE_OUTER_BOUND ( 'NONE', #41957, .T. ) ;
#33044=DIRECTION ( 'NONE',  ( -0.000000000000000000, 1.000000000000000000, -0.000000000000000000 ) ) ;
#33046=DIRECTION ( 'NONE',  ( 0.000000000000000000, 0.000000000000000000, 1.000000000000000000 ) ) ;
#33047=EDGE_CURVE ( 'NONE', #26606, #28239, #4773, .T. ) ;
#33050=CARTESIAN_POINT ( 'NONE',  ( -171.7589556598192360, -177.1207230881787780, -13.35228579481114863 ) ) ;
#33053=ORIENTED_EDGE ( 'NONE', *, *, #11956, .F. ) ;
#33054=CYLINDRICAL_SURFACE ( 'NONE', #49188, 125.0000000000000000 ) ;
#33055=ORIENTED_EDGE ( 'NONE', *, *, #21703, .F. ) ;
#33058=ORIENTED_EDGE ( 'NONE', *, *, #3836, .F. ) ;
#33060=EDGE_CURVE ( 'NONE', #16046, #9877, #40752, .T. ) ;
#33061=LINE ( 'NONE', #12825, #20401 ) ;
#33064=DIRECTION ( 'NONE',  ( -0.9473263538541946138, 0.000000000000000000, 0.3202698538628279690 ) ) ;
#33065=ORIENTED_EDGE ( 'NONE', *, *, #20435, .T. ) ;
#33066=PLANE ( 'NONE',  #45121 ) ;
#33067=ORIENTED_EDGE ( 'NONE', *, *, #3241, .T. ) ;
#33068=CIRCLE ( 'NONE', #42281, 125.0000000000000000 ) ;
#33070=ORIENTED_EDGE ( 'NONE', *, *, #31699, .F. ) ;
#33073=CARTESIAN_POINT ( 'NONE',  ( -34.63763967761164508, -189.7472609257535510, -123.2250735253142864 ) ) ;
#33074=CARTESIAN_POINT ( 'NONE',  ( 72.31641062551800303, -193.5000000000000000, 32.14713283941990341 ) ) ;
#33076=DIRECTION ( 'NONE',  ( 0.000000000000000000, 1.000000000000000000, -0.000000000000000000 ) ) ;
#33078=CARTESIAN_POINT ( 'NONE',  ( 42.89728982752369291, -175.3837268820161057, 83.82333043185313670 ) ) ;
#33079=PLANE ( 'NONE',  #42985 ) ;
#33081=FACE_OUTER_BOUND ( 'NONE', #38350, .T. ) ;
#33082=CARTESIAN_POINT ( 'NONE',  ( 74.49773146996547268, -177.1207230881787780, -22.39848972532282190 ) ) ;
#33083=LINE ( 'NONE', #28612, #44173 ) ;
#33084=ORIENTED_EDGE ( 'NONE', *, *, #7394, .T. ) ;
#33087=DIRECTION ( 'NONE',  ( -0.000000000000000000, 1.000000000000000000, -0.000000000000000000 ) ) ;
#33088=ADVANCED_FACE ( 'NONE', ( #12904 ), #20805, .T. ) ;
#33090=VERTEX_POINT ( 'NONE', #5043 ) ;
#33093=ADVANCED_FACE ( 'NONE', ( #9241 ), #37077, .T. ) ;
#33094=DIRECTION ( 'NONE',  ( -0.000000000000000000, 1.000000000000000000, -0.000000000000000000 ) ) ;
#33095=DIRECTION ( 'NONE',  ( -0.8124868780056783146, 0.000000000000000000, -0.5829794791144762289 ) ) ;
#33096=CARTESIAN_POINT ( 'NONE',  ( -79.88691714431335811, -193.5000000000000000, 119.9572859573367367 ) ) ;
#33097=CARTESIAN_POINT ( 'NONE',  ( 27.23560471289044571, -175.3837268820161057, 99.45993886622845537 ) ) ;
#33099=ORIENTED_EDGE ( 'NONE', *, *, #44227, .F. ) ;
#33101=CARTESIAN_POINT ( 'NONE',  ( 29.27398957514434130, -177.1207230881787780, -97.87467957287998388 ) ) ;
#33102=DIRECTION ( 'NONE',  ( 0.000000000000000000, 1.000000000000000000, 0.000000000000000000 ) ) ;
#33103=ORIENTED_EDGE ( 'NONE', *, *, #16293, .F. ) ;
#33104=VECTOR ( 'NONE', #40049, 1000.000000000000227 ) ;
#33105=CARTESIAN_POINT ( 'NONE',  ( 69.99104047056317768, -193.5000000000000000, -39.87254040532513244 ) ) ;
#33107=FACE_OUTER_BOUND ( 'NONE', #40088, .T. ) ;
#33109=FACE_OUTER_BOUND ( 'NONE', #45598, .T. ) ;
#33110=AXIS2_PLACEMENT_3D ( 'NONE', #44561, #49028, #679 ) ;
#33111=CARTESIAN_POINT ( 'NONE',  ( -169.0855799822425638, -177.1207230881787780, -28.81338593823975103 ) ) ;
#33113=CARTESIAN_POINT ( 'NONE',  ( -129.4514457347087273, -189.7472609257535510, 95.22858582633115532 ) ) ;
#33115=VERTEX_POINT ( 'NONE', #21320 ) ;
#33117=DIRECTION ( 'NONE',  ( 0.000000000000000000, 0.000000000000000000, 1.000000000000000000 ) ) ;
#33118=VERTEX_POINT ( 'NONE', #37339 ) ;
#33119=DIRECTION ( 'NONE',  ( 0.000000000000000000, 0.000000000000000000, -1.000000000000000000 ) ) ;
#33122=ADVANCED_FACE ( 'NONE', ( #9752 ), #49959, .T. ) ;
#33124=CARTESIAN_POINT ( 'NONE',  ( -47.74129347246712740, -193.5000000000000000, -0.6749830015182022303 ) ) ;
#33128=DIRECTION ( 'NONE',  ( 0.000000000000000000, 0.000000000000000000, 1.000000000000000000 ) ) ;
#33129=CARTESIAN_POINT ( 'NONE',  ( -69.59623518921151231, -189.7472609257535510, 122.1886788576023974 ) ) ;
#33130=AXIS2_PLACEMENT_3D ( 'NONE', #4444, #9174, #17065 ) ;
#33131=CARTESIAN_POINT ( 'NONE',  ( 76.37123734610607073, -183.6283474603465606, 6.114457023561872262 ) ) ;
#33135=PLANE ( 'NONE',  #47792 ) ;
#33137=CARTESIAN_POINT ( 'NONE',  ( 35.45604639379469347, -183.6283474603465606, 91.27439114664649367 ) ) ;
#33138=VECTOR ( 'NONE', #47902, 1000.000000000000114 ) ;
#33139=ORIENTED_EDGE ( 'NONE', *, *, #34439, .F. ) ;
#33140=CARTESIAN_POINT ( 'NONE',  ( -45.06671089634843952, -193.5000000000000000, -124.9534129907280402 ) ) ;
#33142=VECTOR ( 'NONE', #27658, 999.9999999999998863 ) ;
#33143=CARTESIAN_POINT ( 'NONE',  ( -172.7479958471413966, -183.6283474603465606, -13.49993235881363418 ) ) ;
#33144=EDGE_LOOP ( 'NONE', ( #42617, #27833, #35586, #33774 ) ) ;
#33146=CARTESIAN_POINT ( 'NONE',  ( -166.9492939735806090, -175.3837268820161057, 39.87254040532603483 ) ) ;
#33147=AXIS2_PLACEMENT_3D ( 'NONE', #35180, #15485, #34664 ) ;
#33148=EDGE_CURVE ( 'NONE', #34248, #51567, #10633, .T. ) ;
#33150=CARTESIAN_POINT ( 'NONE',  ( 6.443011874827243801, -183.6283474603465606, 112.2878385610370771 ) ) ;
#33151=DIRECTION ( 'NONE',  ( 0.6068001458186002006, 0.000000000000000000, -0.7948544414133481562 ) ) ;
#33153=EDGE_CURVE ( 'NONE', #22526, #13663, #41277, .T. ) ;
#33154=CARTESIAN_POINT ( 'NONE',  ( -47.53180039765466347, -175.3837268820161057, 0.3202698538628485636 ) ) ;
#33155=DIRECTION ( 'NONE',  ( 0.000000000000000000, 1.000000000000000000, 0.000000000000000000 ) ) ;
#33156=LINE ( 'NONE', #33681, #27878 ) ;
#33157=LINE ( 'NONE', #2409, #9422 ) ;
#33158=ORIENTED_EDGE ( 'NONE', *, *, #47286, .T. ) ;
#33159=VERTEX_POINT ( 'NONE', #25515 ) ;
#33160=CARTESIAN_POINT ( 'NONE',  ( -92.16375985330356002, -175.3837268820161057, 117.1181148702521710 ) ) ;
#33161=DIRECTION ( 'NONE',  ( 0.000000000000000000, -1.000000000000000000, -0.000000000000000000 ) ) ;
#33162=CYLINDRICAL_SURFACE ( 'NONE', #10242, 124.9999999999999858 ) ;
#33164=VERTEX_POINT ( 'NONE', #41024 ) ;
#33165=VECTOR ( 'NONE', #7160, 1000.000000000000000 ) ;
#33166=VERTEX_POINT ( 'NONE', #33137 ) ;
#33167=DIRECTION ( 'NONE',  ( 0.000000000000000000, 1.000000000000000000, 0.000000000000000000 ) ) ;
#33168=VECTOR ( 'NONE', #9415, 1000.000000000000114 ) ;
#33169=CIRCLE ( 'NONE', #19732, 125.0000000000000000 ) ;
#33171=CYLINDRICAL_SURFACE ( 'NONE', #22437, 125.0000000000000000 ) ;
#33172=VERTEX_POINT ( 'NONE', #29980 ) ;
#33175=CYLINDRICAL_SURFACE ( 'NONE', #37799, 125.0000000000000000 ) ;
#33176=LINE ( 'NONE', #49226, #18271 ) ;
#33180=LINE ( 'NONE', #41063, #50759 ) ;
#33181=EDGE_LOOP ( 'NONE', ( #24151, #581, #27111, #18070 ) ) ;
#33182=DIRECTION ( 'NONE',  ( 0.000000000000000000, 1.000000000000000000, 0.000000000000000000 ) ) ;
#33183=EDGE_LOOP ( 'NONE', ( #45404, #49537, #22421, #45055 ) ) ;
#33184=EDGE_CURVE ( 'NONE', #27201, #20956, #17400, .T. ) ;
#33185=CARTESIAN_POINT ( 'NONE',  ( 59.80284513346456521, -177.1207230881787780, 62.45009659481583242 ) ) ;
#33187=CARTESIAN_POINT ( 'NONE',  ( 74.18685885783123979, -189.7472609257535510, -18.13990644964003707 ) ) ;
#33188=DIRECTION ( 'NONE',  ( 0.8455960035018234011, 0.000000000000000000, 0.5338233779647948429 ) ) ;
#33191=EDGE_CURVE ( 'NONE', #39306, #5601, #5563, .T. ) ;
#33192=EDGE_LOOP ( 'NONE', ( #51555, #32128, #17133, #8533 ) ) ;
#33193=DIRECTION ( 'NONE',  ( 0.000000000000000000, 0.000000000000000000, -1.000000000000000000 ) ) ;
#33194=CARTESIAN_POINT ( 'NONE',  ( 26.52087324849106054, -198.5000000000000000, -80.00000000000002842 ) ) ;
#33196=FACE_OUTER_BOUND ( 'NONE', #40026, .T. ) ;
#33197=DIRECTION ( 'NONE',  ( 0.000000000000000000, 0.000000000000000000, 1.000000000000000000 ) ) ;
#33199=CARTESIAN_POINT ( 'NONE',  ( 62.13187335169531167, -177.1207230881787780, -58.22548115875872554 ) ) ;
#33201=ORIENTED_EDGE ( 'NONE', *, *, #21971, .F. ) ;
#33202=FACE_OUTER_BOUND ( 'NONE', #13944, .T. ) ;
#33203=EDGE_LOOP ( 'NONE', ( #49681, #31517, #11260, #39079 ) ) ;
#33204=AXIS2_PLACEMENT_3D ( 'NONE', #17337, #33356, #37024 ) ;
#33206=LINE ( 'NONE', #25330, #50529 ) ;
#33207=ADVANCED_FACE ( 'NONE', ( #29711 ), #45756, .F. ) ;
#33209=AXIS2_PLACEMENT_3D ( 'NONE', #12173, #20862, #44507 ) ;
#33210=AXIS2_PLACEMENT_3D ( 'NONE', #16873, #40242, #31857 ) ;
#33211=CARTESIAN_POINT ( 'NONE',  ( 59.00260725618641544, -183.6283474603465606, -63.81752780152991278 ) ) ;
#33212=LINE ( 'NONE', #36642, #27202 ) ;
#33213=CYLINDRICAL_SURFACE ( 'NONE', #16526, 125.0000000000000000 ) ;
#33215=EDGE_LOOP ( 'NONE', ( #3961, #42923, #18706, #42802 ) ) ;
#33217=VERTEX_POINT ( 'NONE', #30242 ) ;
#33218=ORIENTED_EDGE ( 'NONE', *, *, #11714, .F. ) ;
#33221=PLANE ( 'NONE',  #28752 ) ;
#33222=ORIENTED_EDGE ( 'NONE', *, *, #48615, .F. ) ;
#33224=EDGE_LOOP ( 'NONE', ( #4327, #19887, #28409, #5107 ) ) ;
#33226=VECTOR ( 'NONE', #45247, 1000.000000000000114 ) ;
#33229=LINE ( 'NONE', #50251, #35224 ) ;
#33230=ORIENTED_EDGE ( 'NONE', *, *, #26665, .T. ) ;
#33232=ORIENTED_EDGE ( 'NONE', *, *, #42848, .F. ) ;
#33233=CARTESIAN_POINT ( 'NONE',  ( -48.47912675150885065, -177.1207230881787780, 6.938893903907228378E-15 ) ) ;
#33234=LINE ( 'NONE', #41632, #24180 ) ;
#33235=ADVANCED_FACE ( 'NONE', ( #38379 ), #51258, .T. ) ;
#33236=CARTESIAN_POINT ( 'NONE',  ( -32.87124591993210743, -189.7472609257535510, 124.0217483183788119 ) ) ;
#33237=CYLINDRICAL_SURFACE ( 'NONE', #13992, 125.0000000000000000 ) ;
#33238=ORIENTED_EDGE ( 'NONE', *, *, #41691, .F. ) ;
#33240=ORIENTED_EDGE ( 'NONE', *, *, #27299, .F. ) ;
#33247=DIRECTION ( 'NONE',  ( -0.000000000000000000, 1.000000000000000000, -0.000000000000000000 ) ) ;
#33248=CARTESIAN_POINT ( 'NONE',  ( -117.0614752283615161, -189.7472609257535510, 103.3076327631967786 ) ) ;
#33250=CIRCLE ( 'NONE', #39940, 125.0000000000000000 ) ;
#33251=EDGE_CURVE ( 'NONE', #27409, #15990, #2112, .T. ) ;
#33252=ADVANCED_FACE ( 'NONE', ( #38888 ), #50483, .T. ) ;
#33254=ORIENTED_EDGE ( 'NONE', *, *, #14163, .T. ) ;
#33255=CARTESIAN_POINT ( 'NONE',  ( -152.3176060415594861, -193.5000000000000000, -69.58857822034967455 ) ) ;
#33256=ORIENTED_EDGE ( 'NONE', *, *, #49818, .T. ) ;
#33257=CARTESIAN_POINT ( 'NONE',  ( -154.0877180371535928, -175.3837268820161057, -66.87170886601927577 ) ) ;
#33259=ADVANCED_FACE ( 'NONE', ( #42308 ), #30743, .T. ) ;
#33260=DIRECTION ( 'NONE',  ( -0.9929810960135185827, 0.000000000000000000, 0.1182731709213523247 ) ) ;
#33264=AXIS2_PLACEMENT_3D ( 'NONE', #29708, #22348, #25261 ) ;
#33266=CARTESIAN_POINT ( 'NONE',  ( -10.02015192278479816, -183.6283474603465606, -117.8859915627474493 ) ) ;
#33267=CARTESIAN_POINT ( 'NONE',  ( -49.03777351731249468, -193.5000000000000000, -0.8294056854502022125 ) ) ;
#33268=ORIENTED_EDGE ( 'NONE', *, *, #44624, .F. ) ;
#33269=DIRECTION ( 'NONE',  ( -0.000000000000000000, 1.000000000000000000, -0.000000000000000000 ) ) ;
#33272=AXIS2_PLACEMENT_3D ( 'NONE', #4832, #32917, #48971 ) ;
#33273=ORIENTED_EDGE ( 'NONE', *, *, #32905, .T. ) ;
#33274=DIRECTION ( 'NONE',  ( 0.4031234292879600778, 0.000000000000000000, 0.9151456172430237901 ) ) ;
#33275=LINE ( 'NONE', #703, #34524 ) ;
#33276=ORIENTED_EDGE ( 'NONE', *, *, #5095, .T. ) ;
#33277=CARTESIAN_POINT ( 'NONE',  ( 75.95066919219054569, -189.7472609257535510, -11.92584929509535385 ) ) ;
#33278=CARTESIAN_POINT ( 'NONE',  ( -49.25565061422690150, -177.1207230881787780, 0.6300878435817109935 ) ) ;
#33279=CARTESIAN_POINT ( 'NONE',  ( -134.9506378406916554, -175.3837268820161057, 90.26448786734091811 ) ) ;
#33280=CARTESIAN_POINT ( 'NONE',  ( -68.09401750944518028, -177.1207230881787780, -122.4396006697294581 ) ) ;
#33281=DIRECTION ( 'NONE',  ( 0.000000000000000000, -1.000000000000000000, 0.000000000000000000 ) ) ;
#33286=AXIS2_PLACEMENT_3D ( 'NONE', #20819, #31862, #32110 ) ;
#33290=DIRECTION ( 'NONE',  ( -0.000000000000000000, 1.000000000000000000, -0.000000000000000000 ) ) ;
#33291=ORIENTED_EDGE ( 'NONE', *, *, #3178, .F. ) ;
#33293=ORIENTED_EDGE ( 'NONE', *, *, #33153, .T. ) ;
#33294=CARTESIAN_POINT ( 'NONE',  ( -48.47912675150885065, -189.7472609257535510, 6.938893903907228378E-15 ) ) ;
#33296=CARTESIAN_POINT ( 'NONE',  ( 21.21056010634072564, -175.3837268820161057, 103.7706487676302061 ) ) ;
#33297=AXIS2_PLACEMENT_3D ( 'NONE', #31365, #39505, #11133 ) ;
#33301=ADVANCED_FACE ( 'NONE', ( #10512 ), #46796, .T. ) ;
#33302=EDGE_CURVE ( 'NONE', #42355, #5112, #42582, .T. ) ;
#33303=EDGE_CURVE ( 'NONE', #35003, #5877, #14223, .T. ) ;
#33305=DIRECTION ( 'NONE',  ( 0.000000000000000000, -0.000000000000000000, 1.000000000000000000 ) ) ;
#33307=ORIENTED_EDGE ( 'NONE', *, *, #2039, .F. ) ;
#33308=ORIENTED_EDGE ( 'NONE', *, *, #49284, .T. ) ;
#33309=CIRCLE ( 'NONE', #49300, 125.0000000000000000 ) ;
#33310=DIRECTION ( 'NONE',  ( 0.9564009842765244240, 0.000000000000000000, -0.2920567706369695538 ) ) ;
#33311=DIRECTION ( 'NONE',  ( 0.000000000000000000, 0.000000000000000000, -1.000000000000000000 ) ) ;
#33312=EDGE_LOOP ( 'NONE', ( #35570, #30916, #51783, #19192 ) ) ;
#33313=CARTESIAN_POINT ( 'NONE',  ( -145.4373324222573842, -189.7472609257535510, -78.89300572996837957 ) ) ;
#33316=CARTESIAN_POINT ( 'NONE',  ( -166.6265240196292439, -189.7472609257535510, 40.81902153125349741 ) ) ;
#33317=EDGE_LOOP ( 'NONE', ( #35969, #33099, #12403, #46096 ) ) ;
#33318=EDGE_CURVE ( 'NONE', #34006, #46012, #24066, .T. ) ;
#33319=ADVANCED_FACE ( 'NONE', ( #15001 ), #31007, .T. ) ;
#33322=ORIENTED_EDGE ( 'NONE', *, *, #51421, .T. ) ;
#33325=ORIENTED_EDGE ( 'NONE', *, *, #43430, .F. ) ;
#33326=CIRCLE ( 'NONE', #35826, 125.0000000000000000 ) ;
#33327=ORIENTED_EDGE ( 'NONE', *, *, #23639, .F. ) ;
#33331=PLANE ( 'NONE',  #41532 ) ;
#33335=DIRECTION ( 'NONE',  ( -0.4566292373937140270, 0.000000000000000000, 0.8896570909947467687 ) ) ;
#33336=LINE ( 'NONE', #20454, #25064 ) ;
#33338=DIRECTION ( 'NONE',  ( -0.4031234292879600778, 0.000000000000000000, -0.9151456172430237901 ) ) ;
#33339=ORIENTED_EDGE ( 'NONE', *, *, #15984, .F. ) ;
#33341=DIRECTION ( 'NONE',  ( -0.000000000000000000, 1.000000000000000000, -0.000000000000000000 ) ) ;
#33342=AXIS2_PLACEMENT_3D ( 'NONE', #46381, #14845, #15104 ) ;
#33344=AXIS2_PLACEMENT_3D ( 'NONE', #25055, #41061, #5078 ) ;
#33345=DIRECTION ( 'NONE',  ( -0.000000000000000000, 1.000000000000000000, -0.000000000000000000 ) ) ;
#33347=AXIS2_PLACEMENT_3D ( 'NONE', #40222, #24459, #8431 ) ;
#33349=DIRECTION ( 'NONE',  ( 0.000000000000000000, 0.000000000000000000, -1.000000000000000000 ) ) ;
#33352=FACE_OUTER_BOUND ( 'NONE', #31895, .T. ) ;
#33356=DIRECTION ( 'NONE',  ( 0.000000000000000000, 1.000000000000000000, 0.000000000000000000 ) ) ;
#33357=AXIS2_PLACEMENT_3D ( 'NONE', #38419, #18455, #22137 ) ;
#33358=DIRECTION ( 'NONE',  ( -0.000000000000000000, 1.000000000000000000, -0.000000000000000000 ) ) ;
#33361=DIRECTION ( 'NONE',  ( 0.000000000000000000, -0.000000000000000000, -1.000000000000000000 ) ) ;
#33362=ORIENTED_EDGE ( 'NONE', *, *, #5746, .F. ) ;
#33363=CARTESIAN_POINT ( 'NONE',  ( 76.48781641346532467, -193.5000000000000000, 2.874563619424060246 ) ) ;
#33364=VERTEX_POINT ( 'NONE', #25947 ) ;
#33365=ADVANCED_FACE ( 'NONE', ( #38023 ), #45943, .T. ) ;
#33367=CARTESIAN_POINT ( 'NONE',  ( -17.07133635870349408, -183.6283474603465606, -119.9572859573364809 ) ) ;
#33368=AXIS2_PLACEMENT_3D ( 'NONE', #24163, #35979, #32021 ) ;
#33371=LINE ( 'NONE', #25994, #5306 ) ;
#33372=AXIS2_PLACEMENT_3D ( 'NONE', #28889, #41237, #1301 ) ;
#33373=ORIENTED_EDGE ( 'NONE', *, *, #2516, .F. ) ;
#33375=EDGE_CURVE ( 'NONE', #18747, #11111, #41969, .T. ) ;
#33376=EDGE_CURVE ( 'NONE', #30289, #44345, #51756, .T. ) ;
#33377=EDGE_CURVE ( 'NONE', #16002, #51805, #38555, .T. ) ;
#33378=CARTESIAN_POINT ( 'NONE',  ( -24.23284180386169240, -177.1207230881787780, -121.6072260099953439 ) ) ;
#33380=EDGE_CURVE ( 'NONE', #48966, #42243, #32418, .T. ) ;
#33382=ORIENTED_EDGE ( 'NONE', *, *, #6550, .T. ) ;
#33384=CIRCLE ( 'NONE', #38433, 125.0000000000000000 ) ;
#33386=VERTEX_POINT ( 'NONE', #6238 ) ;
#33387=ADVANCED_FACE ( 'NONE', ( #29887 ), #10695, .T. ) ;
#33388=CARTESIAN_POINT ( 'NONE',  ( 12.12533326292403935, -177.1207230881787780, 109.3256576763158847 ) ) ;
#33393=ADVANCED_FACE ( 'NONE', ( #38285 ), #26193, .T. ) ;
#33394=AXIS2_PLACEMENT_3D ( 'NONE', #50459, #6820, #18647 ) ;
#33395=DIRECTION ( 'NONE',  ( -0.000000000000000000, 1.000000000000000000, -0.000000000000000000 ) ) ;
#33396=ORIENTED_EDGE ( 'NONE', *, *, #22494, .T. ) ;
#33397=PLANE ( 'NONE',  #3187 ) ;
#33398=DIRECTION ( 'NONE',  ( -0.000000000000000000, 1.000000000000000000, -0.000000000000000000 ) ) ;
#33400=EDGE_CURVE ( 'NONE', #48052, #32649, #34355, .T. ) ;
#33401=DIRECTION ( 'NONE',  ( 0.000000000000000000, 1.000000000000000000, -0.000000000000000000 ) ) ;
#33402=VERTEX_POINT ( 'NONE', #10951 ) ;
#33403=CARTESIAN_POINT ( 'NONE',  ( 24.63024857337166296, -177.1207230881787780, 101.3904297239426597 ) ) ;
#33407=CARTESIAN_POINT ( 'NONE',  ( -95.37971604807246706, -177.1207230881787780, -114.7887733785763942 ) ) ;
#33408=CARTESIAN_POINT ( 'NONE',  ( -163.6979789053106629, -189.7472609257535510, -45.83253885719557985 ) ) ;
#33411=ADVANCED_FACE ( 'NONE', ( #14915 ), #14383, .F. ) ;
#33412=DIRECTION ( 'NONE',  ( 0.000000000000000000, 1.000000000000000000, 0.000000000000000000 ) ) ;
#33413=CIRCLE ( 'NONE', #10737, 125.0000000000000000 ) ;
#33414=LINE ( 'NONE', #41807, #35417 ) ;
#33415=VECTOR ( 'NONE', #7794, 1000.000000000000000 ) ;
#33416=LINE ( 'NONE', #44981, #31514 ) ;
#33417=VERTEX_POINT ( 'NONE', #34852 ) ;
#33418=FACE_OUTER_BOUND ( 'NONE', #50862, .T. ) ;
#33420=DIRECTION ( 'NONE',  ( -0.000000000000000000, 1.000000000000000000, -0.000000000000000000 ) ) ;
#33423=ORIENTED_EDGE ( 'NONE', *, *, #23322, .F. ) ;
#33425=EDGE_CURVE ( 'NONE', #16252, #31640, #3920, .T. ) ;
#33428=DIRECTION ( 'NONE',  ( 0.2635871660690581320, 0.000000000000000000, 0.9646355819083614058 ) ) ;
#33429=VERTEX_POINT ( 'NONE', #2803 ) ;
#33430=DIRECTION ( 'NONE',  ( 0.000000000000000000, 0.000000000000000000, 1.000000000000000000 ) ) ;
#33431=CARTESIAN_POINT ( 'NONE',  ( -49.32472275501067571, -189.7472609257535510, -0.5338233779647935107 ) ) ;
#33433=DIRECTION ( 'NONE',  ( 0.000000000000000000, 0.000000000000000000, 1.000000000000000000 ) ) ;
#33435=VECTOR ( 'NONE', #30217, 999.9999999999998863 ) ;
#33438=FACE_OUTER_BOUND ( 'NONE', #36197, .T. ) ;
#33441=ADVANCED_FACE ( 'NONE', ( #50915 ), #3065, .F. ) ;
#33442=EDGE_CURVE ( 'NONE', #48594, #177, #7783, .T. ) ;
#33443=DIRECTION ( 'NONE',  ( -0.9890401873221644768, 0.000000000000000000, 0.1476465640024779702 ) ) ;
#33444=EDGE_CURVE ( 'NONE', #37576, #30515, #43263, .T. ) ;
#33445=DIRECTION ( 'NONE',  ( 0.1182731709213660498, 0.000000000000000000, -0.9929810960135169173 ) ) ;
#33446=CARTESIAN_POINT ( 'NONE',  ( -141.5426765053792906, -177.1207230881787780, 81.94739446021134199 ) ) ;
#33447=ORIENTED_EDGE ( 'NONE', *, *, #32362, .T. ) ;
#33449=VECTOR ( 'NONE', #32319, 1000.000000000000000 ) ;
#33450=ORIENTED_EDGE ( 'NONE', *, *, #16775, .T. ) ;
#33451=CARTESIAN_POINT ( 'NONE',  ( -143.3583119192899744, -177.1207230881787780, -81.38144888055202841 ) ) ;
#33457=CARTESIAN_POINT ( 'NONE',  ( -172.5669052183642123, -193.5000000000000000, 15.07392567185553567 ) ) ;
#33459=DIRECTION ( 'NONE',  ( 0.000000000000000000, -1.000000000000000000, 0.000000000000000000 ) ) ;
#33461=ADVANCED_FACE ( 'NONE', ( #23313 ), #11974, .T. ) ;
#33462=DIRECTION ( 'NONE',  ( 0.000000000000000000, 0.000000000000000000, 1.000000000000000000 ) ) ;
#33464=CARTESIAN_POINT ( 'NONE',  ( -49.21696003055058810, -183.6283474603465606, 0.6749830015182108900 ) ) ;
#33466=FACE_OUTER_BOUND ( 'NONE', #38366, .T. ) ;
#33467=CARTESIAN_POINT ( 'NONE',  ( -142.6204786402482227, -183.6283474603465606, -80.70646587903385694 ) ) ;
#33471=EDGE_LOOP ( 'NONE', ( #11295, #9147, #36321, #4065 ) ) ;
#33472=ORIENTED_EDGE ( 'NONE', *, *, #4473, .F. ) ;
#33473=CARTESIAN_POINT ( 'NONE',  ( 49.10711742958948633, -189.7472609257535510, 78.11481899503480975 ) ) ;
#33474=DIRECTION ( 'NONE',  ( -0.7378332790417333475, 0.000000000000000000, 0.6749830015182038956 ) ) ;
#33476=DIRECTION ( 'NONE',  ( -0.000000000000000000, 1.000000000000000000, -0.000000000000000000 ) ) ;
#33477=ORIENTED_EDGE ( 'NONE', *, *, #42864, .T. ) ;
#33481=CARTESIAN_POINT ( 'NONE',  ( -150.1390659022305840, -175.3837268820161057, 72.73415134496006829 ) ) ;
#33482=ORIENTED_EDGE ( 'NONE', *, *, #42970, .F. ) ;
#33484=VECTOR ( 'NONE', #44459, 1000.000000000000000 ) ;
#33485=LINE ( 'NONE', #30047, #39626 ) ;
#33486=CARTESIAN_POINT ( 'NONE',  ( -48.47912675150885065, -183.6283474603465606, 6.938893903907228378E-15 ) ) ;
#33487=ORIENTED_EDGE ( 'NONE', *, *, #23854, .F. ) ;
#33488=CIRCLE ( 'NONE', #17549, 125.0000000000000000 ) ;
#33489=FACE_OUTER_BOUND ( 'NONE', #24809, .T. ) ;
#33490=DIRECTION ( 'NONE',  ( 0.000000000000000000, -1.000000000000000000, -0.000000000000000000 ) ) ;
#33491=DIRECTION ( 'NONE',  ( -0.05924062789372142729, 0.000000000000000000, 0.9982437317643209074 ) ) ;
#33492=CARTESIAN_POINT ( 'NONE',  ( -170.4669447856608997, -183.6283474603465606, 22.25084316132123874 ) ) ;
#33493=ORIENTED_EDGE ( 'NONE', *, *, #2418, .T. ) ;
#33494=LINE ( 'NONE', #24817, #25344 ) ;
#33495=EDGE_LOOP ( 'NONE', ( #3233, #19152, #28201, #5987 ) ) ;
#33499=DIRECTION ( 'NONE',  ( -0.08879589532294572540, 0.000000000000000000, 0.9960498426152160079 ) ) ;
#33501=ORIENTED_EDGE ( 'NONE', *, *, #47800, .F. ) ;
#33506=VERTEX_POINT ( 'NONE', #15430 ) ;
#33508=ORIENTED_EDGE ( 'NONE', *, *, #9012, .F. ) ;
#33509=CARTESIAN_POINT ( 'NONE',  ( 11.61413489515543418, -193.5000000000000000, -109.6074810615842381 ) ) ;
#33511=CARTESIAN_POINT ( 'NONE',  ( 60.19403481868997829, -193.5000000000000000, -59.71720175837096889 ) ) ;
#33513=ORIENTED_EDGE ( 'NONE', *, *, #33555, .T. ) ;
#33514=EDGE_LOOP ( 'NONE', ( #23657, #46708, #35843, #51278 ) ) ;
#33515=ORIENTED_EDGE ( 'NONE', *, *, #30813, .T. ) ;
#33517=FACE_OUTER_BOUND ( 'NONE', #50804, .T. ) ;
#33518=AXIS2_PLACEMENT_3D ( 'NONE', #24376, #44080, #51996 ) ;
#33519=EDGE_CURVE ( 'NONE', #9591, #39115, #35374, .T. ) ;
#33520=PLANE ( 'NONE',  #34573 ) ;
#33522=ORIENTED_EDGE ( 'NONE', *, *, #22392, .T. ) ;
#33524=ORIENTED_EDGE ( 'NONE', *, *, #7696, .T. ) ;
#33526=ORIENTED_EDGE ( 'NONE', *, *, #43916, .F. ) ;
#33529=EDGE_CURVE ( 'NONE', #18469, #7899, #22418, .T. ) ;
#33530=CARTESIAN_POINT ( 'NONE',  ( -72.96029774493611342, -177.1207230881787780, 122.5792489240759409 ) ) ;
#33531=CARTESIAN_POINT ( 'NONE',  ( -166.8403286750647680, -193.5000000000000000, -40.19484891389966918 ) ) ;
#33533=ORIENTED_EDGE ( 'NONE', *, *, #14000, .F. ) ;
#33534=DIRECTION ( 'NONE',  ( -0.000000000000000000, 1.000000000000000000, -0.000000000000000000 ) ) ;
#33535=EDGE_CURVE ( 'NONE', #26711, #28978, #19107, .T. ) ;
#33537=CIRCLE ( 'NONE', #32697, 125.0000000000000000 ) ;
#33538=VERTEX_POINT ( 'NONE', #11724 ) ;
#33540=CARTESIAN_POINT ( 'NONE',  ( -171.6469053867625121, -193.5000000000000000, -14.34663989163543008 ) ) ;
#33542=FACE_OUTER_BOUND ( 'NONE', #29860, .T. ) ;
#33543=CARTESIAN_POINT ( 'NONE',  ( -48.47912675150885065, -175.3837268820161057, 6.938893903907228378E-15 ) ) ;
#33544=CARTESIAN_POINT ( 'NONE',  ( -109.0835867659424565, -177.1207230881787780, -109.3256576763154726 ) ) ;
#33546=EDGE_CURVE ( 'NONE', #36985, #28401, #31702, .T. ) ;
#33551=CARTESIAN_POINT ( 'NONE',  ( 75.48400724637755843, -177.1207230881787780, -16.06677968424457958 ) ) ;
#33552=VERTEX_POINT ( 'NONE', #31953 ) ;
#33553=ORIENTED_EDGE ( 'NONE', *, *, #51576, .F. ) ;
#33554=DIRECTION ( 'NONE',  ( 0.000000000000000000, -1.000000000000000000, 0.000000000000000000 ) ) ;
#33555=EDGE_CURVE ( 'NONE', #47219, #49227, #23814, .T. ) ;
#33556=EDGE_LOOP ( 'NONE', ( #26399, #47811, #51722, #5971 ) ) ;
#33557=EDGE_CURVE ( 'NONE', #38799, #11493, #27222, .T. ) ;
#33559=CARTESIAN_POINT ( 'NONE',  ( -31.30262293407085039, -193.5000000000000000, -123.8142468240611294 ) ) ;
#33560=EDGE_CURVE ( 'NONE', #50970, #35187, #12343, .T. ) ;
#33561=LINE ( 'NONE', #30630, #40191 ) ;
#33562=LINE ( 'NONE', #5719, #22054 ) ;
#33563=VERTEX_POINT ( 'NONE', #27747 ) ;
#33564=PLANE ( 'NONE',  #44535 ) ;
#33566=EDGE_LOOP ( 'NONE', ( #19298, #33487, #4998, #7585 ) ) ;
#33567=VECTOR ( 'NONE', #4672, 1000.000000000000000 ) ;
#33570=LINE ( 'NONE', #20970, #34395 ) ;
#33572=EDGE_CURVE ( 'NONE', #27694, #20353, #51687, .T. ) ;
#33573=CARTESIAN_POINT ( 'NONE',  ( -48.07600332222088468, -193.5000000000000000, 0.9151456172430280089 ) ) ;
#33574=CARTESIAN_POINT ( 'NONE',  ( -48.30901192927175458, -193.5000000000000000, -123.9998842437354227 ) ) ;
#33575=ORIENTED_EDGE ( 'NONE', *, *, #10517, .F. ) ;
#33578=CARTESIAN_POINT ( 'NONE',  ( 50.08808042611237710, -183.6283474603465606, -76.87330921200083367 ) ) ;
#33579=ORIENTED_EDGE ( 'NONE', *, *, #40249, .F. ) ;
#33581=CIRCLE ( 'NONE', #32714, 125.0000000000000000 ) ;
#33582=ORIENTED_EDGE ( 'NONE', *, *, #27023, .F. ) ;
#33585=ORIENTED_EDGE ( 'NONE', *, *, #22338, .T. ) ;
#33586=CARTESIAN_POINT ( 'NONE',  ( -26.71218532227686637, -189.7472609257535510, 122.0745693923550732 ) ) ;
#33588=VERTEX_POINT ( 'NONE', #47992 ) ;
#33590=ORIENTED_EDGE ( 'NONE', *, *, #9888, .T. ) ;
#33591=ORIENTED_EDGE ( 'NONE', *, *, #5138, .T. ) ;
#33592=DIRECTION ( 'NONE',  ( -0.000000000000000000, -0.000000000000000000, 1.000000000000000000 ) ) ;
#33594=DIRECTION ( 'NONE',  ( -0.000000000000000000, 1.000000000000000000, -0.000000000000000000 ) ) ;
#33595=DIRECTION ( 'NONE',  ( 0.8455960035018272869, 0.000000000000000000, -0.5338233779647886257 ) ) ;
#33596=EDGE_LOOP ( 'NONE', ( #33803, #8299, #35508, #43770 ) ) ;
#33598=CARTESIAN_POINT ( 'NONE',  ( -48.47912675150885065, -183.6283474603465606, 6.938893903907228378E-15 ) ) ;
#33599=EDGE_CURVE ( 'NONE', #26525, #10132, #14562, .T. ) ;
#33601=CARTESIAN_POINT ( 'NONE',  ( -171.0948786228703113, -189.7472609257535510, -18.47640724094506126 ) ) ;
#33603=VERTEX_POINT ( 'NONE', #10096 ) ;
#33605=CARTESIAN_POINT ( 'NONE',  ( -48.47912675150885065, -175.3837268820161057, 6.938893903907228378E-15 ) ) ;
#33606=CIRCLE ( 'NONE', #19320, 125.0000000000000000 ) ;
#33607=VECTOR ( 'NONE', #22685, 1000.000000000000000 ) ;
#33608=PLANE ( 'NONE',  #24033 ) ;
#33614=EDGE_CURVE ( 'NONE', #2659, #15614, #42670, .T. ) ;
#33615=EDGE_LOOP ( 'NONE', ( #19860, #47688, #35178, #15030 ) ) ;
#33617=CARTESIAN_POINT ( 'NONE',  ( 65.38692482895591240, -177.1207230881787780, -51.57055649762701677 ) ) ;
#33618=EDGE_CURVE ( 'NONE', #2420, #40551, #11112, .T. ) ;
#33619=CIRCLE ( 'NONE', #37815, 125.0000000000000000 ) ;
#33620=DIRECTION ( 'NONE',  ( -0.000000000000000000, 0.000000000000000000, -1.000000000000000000 ) ) ;
#33621=PLANE ( 'NONE',  #41352 ) ;
#33622=DIRECTION ( 'NONE',  ( -0.000000000000000000, 1.000000000000000000, -0.000000000000000000 ) ) ;
#33625=DIRECTION ( 'NONE',  ( -0.000000000000000000, 1.000000000000000000, -0.000000000000000000 ) ) ;
#33626=ORIENTED_EDGE ( 'NONE', *, *, #19102, .T. ) ;
#33627=CARTESIAN_POINT ( 'NONE',  ( 67.66641500972446011, -175.3837268820161057, 46.20836643931067300 ) ) ;
#33628=ORIENTED_EDGE ( 'NONE', *, *, #18036, .T. ) ;
#33629=PLANE ( 'NONE',  #9932 ) ;
#33630=EDGE_LOOP ( 'NONE', ( #123, #19031, #10061, #21304 ) ) ;
#33632=CIRCLE ( 'NONE', #1860, 124.9999999999999858 ) ;
#33633=ORIENTED_EDGE ( 'NONE', *, *, #866, .F. ) ;
#33634=AXIS2_PLACEMENT_3D ( 'NONE', #50180, #45452, #45709 ) ;
#33637=ORIENTED_EDGE ( 'NONE', *, *, #47006, .F. ) ;
#33638=DIRECTION ( 'NONE',  ( 0.2920567706369764371, 0.000000000000000000, -0.9564009842765223146 ) ) ;
#33639=DIRECTION ( 'NONE',  ( -0.000000000000000000, 1.000000000000000000, -0.000000000000000000 ) ) ;
#33640=ORIENTED_EDGE ( 'NONE', *, *, #37358, .T. ) ;
#33641=PLANE ( 'NONE',  #32312 ) ;
#33645=LINE ( 'NONE', #1602, #40952 ) ;
#33649=VERTEX_POINT ( 'NONE', #22957 ) ;
#33650=ADVANCED_FACE ( 'NONE', ( #26884 ), #50824, .T. ) ;
#33651=DIRECTION ( 'NONE',  ( -0.9995608365087942371, 0.000000000000000000, -0.02963332782256331357 ) ) ;
#33653=CARTESIAN_POINT ( 'NONE',  ( -48.47912675150885065, -177.1207230881787780, 6.938893903907228378E-15 ) ) ;
#33654=AXIS2_PLACEMENT_3D ( 'NONE', #34776, #18510, #6436 ) ;
#33655=ORIENTED_EDGE ( 'NONE', *, *, #20786, .F. ) ;
#33656=DIRECTION ( 'NONE',  ( -0.000000000000000000, -1.000000000000000000, 0.000000000000000000 ) ) ;
#33657=DIRECTION ( 'NONE',  ( -0.000000000000000000, 1.000000000000000000, -0.000000000000000000 ) ) ;
#33658=CARTESIAN_POINT ( 'NONE',  ( -64.08700758308647494, -193.5000000000000000, -124.0217483183786840 ) ) ;
#33659=EDGE_CURVE ( 'NONE', #46918, #26606, #34766, .T. ) ;
#33660=EDGE_CURVE ( 'NONE', #50992, #28039, #44245, .T. ) ;
#33662=EDGE_CURVE ( 'NONE', #28777, #41926, #30068, .T. ) ;
#33667=ORIENTED_EDGE ( 'NONE', *, *, #24520, .T. ) ;
#33669=EDGE_CURVE ( 'NONE', #43478, #47044, #43175, .T. ) ;
#33670=DIRECTION ( 'NONE',  ( -0.000000000000000000, 1.000000000000000000, 0.000000000000000000 ) ) ;
#33672=DIRECTION ( 'NONE',  ( -0.9995608365087940150, 0.000000000000000000, -0.02963332782257007206 ) ) ;
#33673=CARTESIAN_POINT ( 'NONE',  ( 52.16997862029127475, -193.5000000000000000, 72.42760398749085482 ) ) ;
#33675=EDGE_CURVE ( 'NONE', #11325, #5201, #46764, .T. ) ;
#33676=AXIS2_PLACEMENT_3D ( 'NONE', #23844, #39855, #35667 ) ;
#33678=EDGE_CURVE ( 'NONE', #23489, #36830, #46365, .T. ) ;
#33680=CARTESIAN_POINT ( 'NONE',  ( 54.18765407974402848, -183.6283474603465606, -69.53890913632879744 ) ) ;
#33681=CARTESIAN_POINT ( 'NONE',  ( 60.90550954139435902, -175.3837268820161057, 60.49794494914085874 ) ) ;
#33682=PLANE ( 'NONE',  #42982 ) ;
#33684=EDGE_CURVE ( 'NONE', #50065, #14521, #35042, .T. ) ;
#33685=VERTEX_POINT ( 'NONE', #42405 ) ;
#33686=DIRECTION ( 'NONE',  ( 0.000000000000000000, -0.000000000000000000, 1.000000000000000000 ) ) ;
#33687=EDGE_CURVE ( 'NONE', #6776, #21227, #31087, .T. ) ;
#33688=CARTESIAN_POINT ( 'NONE',  ( -172.9701362814535912, -189.7472609257535510, -11.26891947860197440 ) ) ;
#33690=ORIENTED_EDGE ( 'NONE', *, *, #23861, .T. ) ;
#33692=VECTOR ( 'NONE', #7463, 1000.000000000000000 ) ;
#33693=ORIENTED_EDGE ( 'NONE', *, *, #50958, .T. ) ;
#33697=ORIENTED_EDGE ( 'NONE', *, *, #36828, .F. ) ;
#33698=ADVANCED_FACE ( 'NONE', ( #3251 ), #46116, .T. ) ;
#33699=DIRECTION ( 'NONE',  ( -0.000000000000000000, 1.000000000000000000, -0.000000000000000000 ) ) ;
#33701=ORIENTED_EDGE ( 'NONE', *, *, #26085, .T. ) ;
#33702=DIRECTION ( 'NONE',  ( -0.000000000000000000, 1.000000000000000000, -0.000000000000000000 ) ) ;
#33703=ORIENTED_EDGE ( 'NONE', *, *, #21077, .F. ) ;
#33704=PLANE ( 'NONE',  #49051 ) ;
#33705=VECTOR ( 'NONE', #28805, 1000.000000000000000 ) ;
#33706=EDGE_LOOP ( 'NONE', ( #42511, #17030, #14561, #19566 ) ) ;
#33707=DIRECTION ( 'NONE',  ( 0.9890401873221633666, 0.000000000000000000, 0.1476465640024850756 ) ) ;
#33708=DIRECTION ( 'NONE',  ( 0.6965510290629932655, 0.000000000000000000, 0.7175072570443347120 ) ) ;
#33709=AXIS2_PLACEMENT_3D ( 'NONE', #167, #3346, #12254 ) ;
#33710=LINE ( 'NONE', #26079, #7276 ) ;
#33711=VECTOR ( 'NONE', #13454, 1000.000000000000114 ) ;
#33712=VERTEX_POINT ( 'NONE', #27918 ) ;
#33713=ORIENTED_EDGE ( 'NONE', *, *, #22870, .F. ) ;
#33714=PLANE ( 'NONE',  #41567 ) ;
#33717=LINE ( 'NONE', #26086, #35064 ) ;
#33720=ORIENTED_EDGE ( 'NONE', *, *, #38531, .T. ) ;
#33721=FACE_OUTER_BOUND ( 'NONE', #51173, .T. ) ;
#33722=AXIS2_PLACEMENT_3D ( 'NONE', #17920, #17419, #13974 ) ;
#33723=DIRECTION ( 'NONE',  ( 0.7575112421616236880, 0.000000000000000000, -0.6528221181905174975 ) ) ;
#33724=EDGE_CURVE ( 'NONE', #34754, #51254, #32122, .T. ) ;
#33725=EDGE_CURVE ( 'NONE', #25328, #8967, #7940, .T. ) ;
#33726=ORIENTED_EDGE ( 'NONE', *, *, #8613, .T. ) ;
#33730=DIRECTION ( 'NONE',  ( 0.5085311186492094127, 0.000000000000000000, 0.8610436117673619938 ) ) ;
#33731=CARTESIAN_POINT ( 'NONE',  ( 62.86098202833237281, -183.6283474603465606, 56.81883646197908888 ) ) ;
#33732=FACE_OUTER_BOUND ( 'NONE', #33224, .T. ) ;
#33733=VERTEX_POINT ( 'NONE', #51584 ) ;
#33734=CARTESIAN_POINT ( 'NONE',  ( -126.2322430781613605, -193.5000000000000000, 97.87467957288053810 ) ) ;
#33735=CARTESIAN_POINT ( 'NONE',  ( 11.61413489515543418, -177.1207230881787780, -109.6074810615842381 ) ) ;
#33737=CARTESIAN_POINT ( 'NONE',  ( 34.98161733638497850, -183.6283474603465606, -91.70840728318314916 ) ) ;
#33740=ORIENTED_EDGE ( 'NONE', *, *, #18488, .F. ) ;
#33741=EDGE_CURVE ( 'NONE', #14876, #40260, #15711, .T. ) ;
#33742=DIRECTION ( 'NONE',  ( -0.000000000000000000, 1.000000000000000000, -0.000000000000000000 ) ) ;
#33744=VECTOR ( 'NONE', #18149, 1000.000000000000114 ) ;
#33749=AXIS2_PLACEMENT_3D ( 'NONE', #29669, #17609, #33620 ) ;
#33752=PLANE ( 'NONE',  #10484 ) ;
#33756=CARTESIAN_POINT ( 'NONE',  ( -172.4422607493951602, -177.1207230881787780, 16.06677968424543934 ) ) ;
#33758=VERTEX_POINT ( 'NONE', #11368 ) ;
#33761=CIRCLE ( 'NONE', #43918, 125.0000000000000000 ) ;
#33762=ORIENTED_EDGE ( 'NONE', *, *, #2236, .T. ) ;
#33766=CIRCLE ( 'NONE', #8586, 125.0000000000000000 ) ;
#33771=ORIENTED_EDGE ( 'NONE', *, *, #36486, .F. ) ;
#33772=LINE ( 'NONE', #5681, #8871 ) ;
#33774=ORIENTED_EDGE ( 'NONE', *, *, #22474, .T. ) ;
#33776=FACE_OUTER_BOUND ( 'NONE', #6519, .T. ) ;
#33777=AXIS2_PLACEMENT_3D ( 'NONE', #29640, #41208, #5235 ) ;
#33779=EDGE_CURVE ( 'NONE', #49533, #8359, #36066, .T. ) ;
#33781=EDGE_CURVE ( 'NONE', #44141, #8140, #27400, .T. ) ;
#33782=ORIENTED_EDGE ( 'NONE', *, *, #23151, .F. ) ;
#33783=CARTESIAN_POINT ( 'NONE',  ( -113.5519059482138857, -183.6283474603465606, 105.5544085257715210 ) ) ;
#33785=ORIENTED_EDGE ( 'NONE', *, *, #43268, .T. ) ;
#33787=LINE ( 'NONE', #2509, #32005 ) ;
#33788=VERTEX_POINT ( 'NONE', #31606 ) ;
#33789=CARTESIAN_POINT ( 'NONE',  ( 61.22907552172956969, -183.6283474603465606, -57.79541595648220920 ) ) ;
#33790=PLANE ( 'NONE',  #17139 ) ;
#33791=CARTESIAN_POINT ( 'NONE',  ( -48.47912675150885065, -175.3837268820161057, 6.938893903907228378E-15 ) ) ;
#33796=FACE_BOUND ( 'NONE', #34213, .T. ) ;
#33797=EDGE_LOOP ( 'NONE', ( #20242, #3503, #47673, #28649 ) ) ;
#33799=VECTOR ( 'NONE', #22172, 1000.000000000000000 ) ;
#33800=EDGE_CURVE ( 'NONE', #37750, #35361, #35012, .T. ) ;
#33801=DIRECTION ( 'NONE',  ( 0.000000000000000000, 0.000000000000000000, 1.000000000000000000 ) ) ;
#33802=ORIENTED_EDGE ( 'NONE', *, *, #33741, .F. ) ;
#33803=ORIENTED_EDGE ( 'NONE', *, *, #36196, .F. ) ;
#33804=LINE ( 'NONE', #49338, #7833 ) ;
#33805=AXIS2_PLACEMENT_3D ( 'NONE', #17348, #42008, #6280 ) ;
#33808=FACE_OUTER_BOUND ( 'NONE', #248, .T. ) ;
#33809=LINE ( 'NONE', #5454, #26763 ) ;
#33810=LINE ( 'NONE', #24899, #4417 ) ;
#33813=CARTESIAN_POINT ( 'NONE',  ( -115.7878797639662025, -177.1207230881787780, -104.1428419024399687 ) ) ;
#33820=DIRECTION ( 'NONE',  ( -0.000000000000000000, 1.000000000000000000, -0.000000000000000000 ) ) ;
#33821=DIRECTION ( 'NONE',  ( 0.000000000000000000, 1.000000000000000000, 0.000000000000000000 ) ) ;
#33822=DIRECTION ( 'NONE',  ( -0.7378332790417333475, 0.000000000000000000, 0.6749830015182038956 ) ) ;
#33823=DIRECTION ( 'NONE',  ( 0.000000000000000000, 0.000000000000000000, 1.000000000000000000 ) ) ;
#33824=ORIENTED_EDGE ( 'NONE', *, *, #2218, .T. ) ;
#33826=VECTOR ( 'NONE', #35104, 1000.000000000000000 ) ;
#33827=EDGE_CURVE ( 'NONE', #41514, #15304, #23477, .T. ) ;
#33828=CARTESIAN_POINT ( 'NONE',  ( 76.28370911321322012, -193.5000000000000000, -7.696413904697510411 ) ) ;
#33832=VERTEX_POINT ( 'NONE', #8465 ) ;
#33834=ORIENTED_EDGE ( 'NONE', *, *, #42022, .T. ) ;
#33835=VERTEX_POINT ( 'NONE', #11642 ) ;
#33836=FACE_OUTER_BOUND ( 'NONE', #21778, .T. ) ;
#33837=CARTESIAN_POINT ( 'NONE',  ( 69.04371411670899761, -189.7472609257535510, -39.55227055146231407 ) ) ;
#33839=CARTESIAN_POINT ( 'NONE',  ( -48.47912675150885065, -193.5000000000000000, 1.000000000000006883 ) ) ;
#33841=VECTOR ( 'NONE', #39025, 1000.000000000000000 ) ;
#33842=LINE ( 'NONE', #29897, #30118 ) ;
#33844=EDGE_CURVE ( 'NONE', #45175, #27293, #12306, .T. ) ;
#33845=CARTESIAN_POINT ( 'NONE',  ( -170.4669447856608997, -177.1207230881787780, 22.25084316132123519 ) ) ;
#33847=VERTEX_POINT ( 'NONE', #319 ) ;
#33849=ADVANCED_FACE ( 'NONE', ( #44479 ), #16363, .T. ) ;
#33850=LINE ( 'NONE', #46464, #39826 ) ;
#33852=ORIENTED_EDGE ( 'NONE', *, *, #12016, .T. ) ;
#33853=LINE ( 'NONE', #49893, #38261 ) ;
#33854=CIRCLE ( 'NONE', #27954, 10.00000000000000000 ) ;
#33855=PLANE ( 'NONE',  #33956 ) ;
#33857=DIRECTION ( 'NONE',  ( -0.000000000000000000, 1.000000000000000000, -0.000000000000000000 ) ) ;
#33859=DIRECTION ( 'NONE',  ( 0.5085311186492154079, 0.000000000000000000, 0.8610436117673585521 ) ) ;
#33862=ORIENTED_EDGE ( 'NONE', *, *, #16794, .F. ) ;
#33864=DIRECTION ( 'NONE',  ( -0.000000000000000000, 1.000000000000000000, -0.000000000000000000 ) ) ;
#33865=LINE ( 'NONE', #13906, #41248 ) ;
#33866=ORIENTED_EDGE ( 'NONE', *, *, #41424, .T. ) ;
#33867=EDGE_LOOP ( 'NONE', ( #34251, #2775, #48531, #19461 ) ) ;
#33868=VECTOR ( 'NONE', #22665, 1000.000000000000000 ) ;
#33869=ORIENTED_EDGE ( 'NONE', *, *, #555, .T. ) ;
#33870=CARTESIAN_POINT ( 'NONE',  ( 67.29303306501927295, -175.3837268820161057, 47.13604789772129777 ) ) ;
#33871=VECTOR ( 'NONE', #23821, 1000.000000000000000 ) ;
#33874=DIRECTION ( 'NONE',  ( 0.000000000000000000, -0.000000000000000000, 1.000000000000000000 ) ) ;
#33875=CARTESIAN_POINT ( 'NONE',  ( 60.90550954139435902, -193.5000000000000000, 60.49794494914085874 ) ) ;
#33876=EDGE_LOOP ( 'NONE', ( #46582, #49587, #30034, #39761 ) ) ;
#33877=CARTESIAN_POINT ( 'NONE',  ( -238.7407812814481076, -213.5000000000000000, -41.45482488023466061 ) ) ;
#33878=EDGE_LOOP ( 'NONE', ( #2261, #31459, #7162, #17173 ) ) ;
#33879=CARTESIAN_POINT ( 'NONE',  ( -129.3001299485802917, -193.5000000000000000, -94.04236105995796891 ) ) ;
#33880=ORIENTED_EDGE ( 'NONE', *, *, #31286, .T. ) ;
#33881=FACE_OUTER_BOUND ( 'NONE', #3796, .T. ) ;
#33882=VECTOR ( 'NONE', #31976, 1000.000000000000114 ) ;
#33883=ADVANCED_FACE ( 'NONE', ( #13205 ), #9262, .T. ) ;
#33884=ORIENTED_EDGE ( 'NONE', *, *, #43033, .F. ) ;
#33885=AXIS2_PLACEMENT_3D ( 'NONE', #50422, #35396, #43035 ) ;
#33886=DIRECTION ( 'NONE',  ( -0.7948544414133608127, 0.000000000000000000, 0.6068001458185834363 ) ) ;
#33888=ORIENTED_EDGE ( 'NONE', *, *, #27553, .F. ) ;
#33890=CARTESIAN_POINT ( 'NONE',  ( -22.44626007086657182, -193.5000000000000000, 122.2591094863196730 ) ) ;
#33892=DIRECTION ( 'NONE',  ( 0.9842305779475954974, 0.000000000000000000, 0.1768902751225803205 ) ) ;
#33893=ORIENTED_EDGE ( 'NONE', *, *, #23067, .F. ) ;
#33894=CARTESIAN_POINT ( 'NONE',  ( -108.0638572795231909, -177.1207230881787780, 108.7464374498172646 ) ) ;
#33895=ORIENTED_EDGE ( 'NONE', *, *, #45894, .T. ) ;
#33897=CARTESIAN_POINT ( 'NONE',  ( -130.2106798473772642, -189.7472609257535510, 94.57776286494221551 ) ) ;
#33900=ORIENTED_EDGE ( 'NONE', *, *, #9171, .F. ) ;
#33903=EDGE_CURVE ( 'NONE', #37732, #1758, #25283, .T. ) ;
#33904=LINE ( 'NONE', #10257, #7235 ) ;
#33906=LINE ( 'NONE', #17647, #43788 ) ;
#33907=EDGE_CURVE ( 'NONE', #48520, #36852, #32647, .T. ) ;
#33909=ORIENTED_EDGE ( 'NONE', *, *, #48158, .F. ) ;
#33910=CARTESIAN_POINT ( 'NONE',  ( -238.7407812814481076, -213.5000000000000000, -41.45482488023466061 ) ) ;
#33911=DIRECTION ( 'NONE',  ( 0.000000000000000000, 0.000000000000000000, 1.000000000000000000 ) ) ;
#33913=DIRECTION ( 'NONE',  ( -0.2920567706369694982, 0.000000000000000000, -0.9564009842765243130 ) ) ;
#33914=ORIENTED_EDGE ( 'NONE', *, *, #19463, .F. ) ;
#33918=VERTEX_POINT ( 'NONE', #29472 ) ;
#33919=CARTESIAN_POINT ( 'NONE',  ( -160.9694636715425702, -193.5000000000000000, 54.50618404931040573 ) ) ;
#33926=DIRECTION ( 'NONE',  ( 0.6528221181905227155, 0.000000000000000000, -0.7575112421616191360 ) ) ;
#33927=CARTESIAN_POINT ( 'NONE',  ( 55.03325008324586776, -177.1207230881787780, -70.07273251429357686 ) ) ;
#33928=DIRECTION ( 'NONE',  ( -0.3202698538628487301, 0.000000000000000000, 0.9473263538541877304 ) ) ;
#33929=VERTEX_POINT ( 'NONE', #32894 ) ;
#33930=VERTEX_POINT ( 'NONE', #17147 ) ;
#33935=ORIENTED_EDGE ( 'NONE', *, *, #1641, .T. ) ;
#33936=ORIENTED_EDGE ( 'NONE', *, *, #42050, .F. ) ;
#33937=FACE_OUTER_BOUND ( 'NONE', #1536, .T. ) ;
#33938=ADVANCED_FACE ( 'NONE', ( #29224 ), #1639, .T. ) ;
#33939=ADVANCED_FACE ( 'NONE', ( #45280 ), #17675, .F. ) ;
#33940=EDGE_CURVE ( 'NONE', #47336, #37757, #5325, .T. ) ;
#33942=DIRECTION ( 'NONE',  ( 0.000000000000000000, -0.000000000000000000, -1.000000000000000000 ) ) ;
#33944=EDGE_CURVE ( 'NONE', #37834, #28928, #29732, .T. ) ;
#33946=FACE_OUTER_BOUND ( 'NONE', #12464, .T. ) ;
#33947=CARTESIAN_POINT ( 'NONE',  ( -153.7737137892885073, -175.3837268820161057, -65.49088066501643368 ) ) ;
#33949=EDGE_CURVE ( 'NONE', #46831, #3996, #13460, .T. ) ;
#33950=EDGE_CURVE ( 'NONE', #25168, #37719, #25535, .T. ) ;
#33952=AXIS2_PLACEMENT_3D ( 'NONE', #43075, #46776, #2617 ) ;
#33954=DIRECTION ( 'NONE',  ( 0.9473263538541923934, 0.000000000000000000, -0.3202698538628350744 ) ) ;
#33955=ORIENTED_EDGE ( 'NONE', *, *, #33025, .T. ) ;
#33956=AXIS2_PLACEMENT_3D ( 'NONE', #13375, #17835, #49894 ) ;
#33957=DIRECTION ( 'NONE',  ( 0.000000000000000000, -0.000000000000000000, 1.000000000000000000 ) ) ;
#33958=ADVANCED_FACE ( 'NONE', ( #41046 ), #44739, .T. ) ;
#33959=CARTESIAN_POINT ( 'NONE',  ( -1.771278280434267272, -177.1207230881787780, -115.9455772817710226 ) ) ;
#33960=FACE_OUTER_BOUND ( 'NONE', #36454, .T. ) ;
#33961=CIRCLE ( 'NONE', #48268, 125.0000000000000000 ) ;
#33964=EDGE_CURVE ( 'NONE', #15918, #29184, #16636, .T. ) ;
#33966=LINE ( 'NONE', #41864, #32326 ) ;
#33970=VECTOR ( 'NONE', #33398, 1000.000000000000000 ) ;
#33972=EDGE_CURVE ( 'NONE', #39607, #30848, #13650, .T. ) ;
#33975=VECTOR ( 'NONE', #3509, 1000.000000000000000 ) ;
#33976=DIRECTION ( 'NONE',  ( 0.000000000000000000, 0.000000000000000000, 1.000000000000000000 ) ) ;
#33979=LINE ( 'NONE', #50026, #46745 ) ;
#33980=ORIENTED_EDGE ( 'NONE', *, *, #14170, .T. ) ;
#33983=FACE_OUTER_BOUND ( 'NONE', #43522, .T. ) ;
#33987=CARTESIAN_POINT ( 'NONE',  ( -80.17897391495031911, -177.1207230881787780, 120.9136869416132498 ) ) ;
#33988=LINE ( 'NONE', #45834, #50929 ) ;
#33990=ORIENTED_EDGE ( 'NONE', *, *, #38305, .T. ) ;
#33991=DIRECTION ( 'NONE',  ( 0.000000000000000000, 1.000000000000000000, -0.000000000000000000 ) ) ;
#33993=AXIS2_PLACEMENT_3D ( 'NONE', #10075, #1673, #13757 ) ;
#33994=DIRECTION ( 'NONE',  ( 0.000000000000000000, 0.000000000000000000, -1.000000000000000000 ) ) ;
#33996=ORIENTED_EDGE ( 'NONE', *, *, #14250, .F. ) ;
#33999=ORIENTED_EDGE ( 'NONE', *, *, #43796, .T. ) ;
#34002=CARTESIAN_POINT ( 'NONE',  ( -30.48891621885994496, -183.6283474603465606, -122.6885491605230101 ) ) ;
#34003=ORIENTED_EDGE ( 'NONE', *, *, #15792, .T. ) ;
#34005=AXIS2_PLACEMENT_3D ( 'NONE', #2026, #14141, #41971 ) ;
#34006=VERTEX_POINT ( 'NONE', #16575 ) ;
#34007=CARTESIAN_POINT ( 'NONE',  ( -25.72842157752850056, -189.7472609257535510, 121.8950816227734606 ) ) ;
#34009=VECTOR ( 'NONE', #25870, 1000.000000000000000 ) ;
#34011=EDGE_CURVE ( 'NONE', #664, #31150, #35053, .T. ) ;
#34012=EDGE_CURVE ( 'NONE', #42165, #6625, #41496, .T. ) ;
#34013=EDGE_CURVE ( 'NONE', #4631, #32588, #25478, .T. ) ;
#34021=VECTOR ( 'NONE', #17045, 1000.000000000000000 ) ;
#34022=DIRECTION ( 'NONE',  ( 0.000000000000000000, -1.000000000000000000, 0.000000000000000000 ) ) ;
#34028=VERTEX_POINT ( 'NONE', #32586 ) ;
#34030=EDGE_CURVE ( 'NONE', #33013, #50209, #51020, .T. ) ;
#34031=ORIENTED_EDGE ( 'NONE', *, *, #24184, .T. ) ;
#34032=CARTESIAN_POINT ( 'NONE',  ( -104.9497554727472561, -175.3837268820161057, -110.3950557015148775 ) ) ;
#34033=EDGE_LOOP ( 'NONE', ( #27226, #14653, #31253, #7356 ) ) ;
#34035=AXIS2_PLACEMENT_3D ( 'NONE', #37862, #9757, #48927 ) ;
#34036=ADVANCED_FACE ( 'NONE', ( #44943 ), #5263, .T. ) ;
#34037=DIRECTION ( 'NONE',  ( 0.4827922027307366970, 0.000000000000000000, 0.8757349421956412971 ) ) ;
#34038=DIRECTION ( 'NONE',  ( 0.9720229140804123036, 0.000000000000000000, -0.2348860457809775759 ) ) ;
#34039=AXIS2_PLACEMENT_3D ( 'NONE', #39208, #39452, #27372 ) ;
#34040=VECTOR ( 'NONE', #48412, 1000.000000000000000 ) ;
#34042=LINE ( 'NONE', #33531, #49754 ) ;
#34044=VERTEX_POINT ( 'NONE', #21805 ) ;
#34045=DIRECTION ( 'NONE',  ( 0.000000000000000000, -1.000000000000000000, 0.000000000000000000 ) ) ;
#34046=ORIENTED_EDGE ( 'NONE', *, *, #21077, .T. ) ;
#34047=EDGE_CURVE ( 'NONE', #16943, #13171, #46491, .T. ) ;
#34050=VECTOR ( 'NONE', #24999, 1000.000000000000000 ) ;
#34051=LINE ( 'NONE', #38242, #36206 ) ;
#34052=ORIENTED_EDGE ( 'NONE', *, *, #6385, .T. ) ;
#34053=AXIS2_PLACEMENT_3D ( 'NONE', #22963, #2980, #51591 ) ;
#34054=CARTESIAN_POINT ( 'NONE',  ( -118.9967449635792462, -193.5000000000000000, -103.2098131075562009 ) ) ;
#34055=CARTESIAN_POINT ( 'NONE',  ( 53.18081239921338721, -175.3837268820161057, -72.73415134495935774 ) ) ;
#34057=VECTOR ( 'NONE', #14330, 1000.000000000000000 ) ;
#34058=CARTESIAN_POINT ( 'NONE',  ( -162.0868781531755474, -183.6283474603465606, -49.69312418816313226 ) ) ;
#34059=EDGE_CURVE ( 'NONE', #50178, #13839, #14187, .T. ) ;
#34060=CARTESIAN_POINT ( 'NONE',  ( 36.10886851198520731, -183.6283474603465606, 92.03190238880812046 ) ) ;
#34062=ORIENTED_EDGE ( 'NONE', *, *, #27452, .T. ) ;
#34065=EDGE_LOOP ( 'NONE', ( #44285, #22126, #48544, #38926 ) ) ;
#34068=DIRECTION ( 'NONE',  ( 0.6749830015182142207, 0.000000000000000000, -0.7378332790417239107 ) ) ;
#34069=CIRCLE ( 'NONE', #17276, 125.0000000000000000 ) ;
#34071=DIRECTION ( 'NONE',  ( -0.000000000000000000, 1.000000000000000000, -0.000000000000000000 ) ) ;
#34072=ORIENTED_EDGE ( 'NONE', *, *, #17202, .T. ) ;
#34073=PLANE ( 'NONE',  #16579 ) ;
#34075=VECTOR ( 'NONE', #15011, 1000.000000000000227 ) ;
#34079=CARTESIAN_POINT ( 'NONE',  ( -172.2289551866394106, -175.3837268820161057, -17.63462396184710101 ) ) ;
#34084=DIRECTION ( 'NONE',  ( -0.7765238627180393038, 0.000000000000000000, -0.6300878435817147682 ) ) ;
#34085=AXIS2_PLACEMENT_3D ( 'NONE', #20016, #36832, #44456 ) ;
#34087=AXIS2_PLACEMENT_3D ( 'NONE', #33734, #12970, #28995 ) ;
#34088=LINE ( 'NONE', #42218, #19460 ) ;
#34092=AXIS2_PLACEMENT_3D ( 'NONE', #11393, #26914, #27430 ) ;
#34093=DIRECTION ( 'NONE',  ( -0.000000000000000000, 1.000000000000000000, -0.000000000000000000 ) ) ;
#34095=DIRECTION ( 'NONE',  ( 0.9890401873221633666, 0.000000000000000000, 0.1476465640024850756 ) ) ;
#34096=ORIENTED_EDGE ( 'NONE', *, *, #13093, .T. ) ;
#34097=ORIENTED_EDGE ( 'NONE', *, *, #42376, .F. ) ;
#34098=PLANE ( 'NONE',  #29988 ) ;
#34100=VERTEX_POINT ( 'NONE', #9711 ) ;
#34101=DIRECTION ( 'NONE',  ( 0.000000000000000000, 1.000000000000000000, 0.000000000000000000 ) ) ;
#34102=ORIENTED_EDGE ( 'NONE', *, *, #43287, .T. ) ;
#34103=CARTESIAN_POINT ( 'NONE',  ( -81.70897914701313880, -177.1207230881787780, -120.5021863277716534 ) ) ;
#34104=DIRECTION ( 'NONE',  ( -0.000000000000000000, -1.000000000000000000, 0.000000000000000000 ) ) ;
#34107=ORIENTED_EDGE ( 'NONE', *, *, #313, .T. ) ;
#34108=EDGE_CURVE ( 'NONE', #30169, #25631, #10474, .T. ) ;
#34109=ORIENTED_EDGE ( 'NONE', *, *, #35560, .T. ) ;
#34111=AXIS2_PLACEMENT_3D ( 'NONE', #29917, #45978, #50427 ) ;
#34112=DIRECTION ( 'NONE',  ( -0.5085311186492216251, 0.000000000000000000, 0.8610436117673548884 ) ) ;
#34114=CARTESIAN_POINT ( 'NONE',  ( -59.28786813212838069, -193.5000000000000000, 124.5318076226587323 ) ) ;
#34115=ORIENTED_EDGE ( 'NONE', *, *, #30406, .F. ) ;
#34117=LINE ( 'NONE', #18091, #24770 ) ;
#34118=AXIS2_PLACEMENT_3D ( 'NONE', #30488, #42834, #6328 ) ;
#34123=CARTESIAN_POINT ( 'NONE',  ( -47.49008656418669005, -193.5000000000000000, 0.1476465640024920423 ) ) ;
#34124=CARTESIAN_POINT ( 'NONE',  ( 27.42205759510524032, -175.3837268820161057, 98.05618656931997634 ) ) ;
#34125=VERTEX_POINT ( 'NONE', #37820 ) ;
#34126=EDGE_LOOP ( 'NONE', ( #35228, #22911, #31287, #5109 ) ) ;
#34128=VECTOR ( 'NONE', #45590, 1000.000000000000000 ) ;
#34130=VECTOR ( 'NONE', #33358, 1000.000000000000000 ) ;
#34131=CIRCLE ( 'NONE', #45063, 125.0000000000000000 ) ;
#34132=CYLINDRICAL_SURFACE ( 'NONE', #30296, 125.0000000000000000 ) ;
#34133=VERTEX_POINT ( 'NONE', #2070 ) ;
#34134=FACE_OUTER_BOUND ( 'NONE', #43825, .T. ) ;
#34136=ORIENTED_EDGE ( 'NONE', *, *, #13638, .F. ) ;
#34137=AXIS2_PLACEMENT_3D ( 'NONE', #5090, #37659, #50014 ) ;
#34138=DIRECTION ( 'NONE',  ( -0.000000000000000000, 1.000000000000000000, -0.000000000000000000 ) ) ;
#34140=CYLINDRICAL_SURFACE ( 'NONE', #14528, 125.0000000000000000 ) ;
#34141=CARTESIAN_POINT ( 'NONE',  ( -15.24927435600541692, -177.1207230881787780, 120.5021863277719234 ) ) ;
#34145=DIRECTION ( 'NONE',  ( -0.9785564922995017012, 0.000000000000000000, -0.2059786187411094538 ) ) ;
#34146=ORIENTED_EDGE ( 'NONE', *, *, #49889, .T. ) ;
#34147=DIRECTION ( 'NONE',  ( 0.000000000000000000, 1.000000000000000000, 0.000000000000000000 ) ) ;
#34148=AXIS2_PLACEMENT_3D ( 'NONE', #30306, #6153, #25855 ) ;
#34152=FACE_OUTER_BOUND ( 'NONE', #45357, .T. ) ;
#34154=EDGE_LOOP ( 'NONE', ( #20767, #18341, #41541, #28358 ) ) ;
#34156=DIRECTION ( 'NONE',  ( 0.000000000000000000, 0.000000000000000000, 1.000000000000000000 ) ) ;
#34161=CIRCLE ( 'NONE', #42557, 125.0000000000000000 ) ;
#34165=CARTESIAN_POINT ( 'NONE',  ( -47.49008656418669005, -177.1207230881787780, -0.1476465640024710591 ) ) ;
#34166=ORIENTED_EDGE ( 'NONE', *, *, #47505, .T. ) ;
#34167=CIRCLE ( 'NONE', #7315, 125.0000000000000000 ) ;
#34172=ORIENTED_EDGE ( 'NONE', *, *, #5451, .F. ) ;
#34173=AXIS2_PLACEMENT_3D ( 'NONE', #30993, #30726, #38617 ) ;
#34174=DIRECTION ( 'NONE',  ( -0.000000000000000000, 1.000000000000000000, -0.000000000000000000 ) ) ;
#34175=VERTEX_POINT ( 'NONE', #22583 ) ;
#34176=DIRECTION ( 'NONE',  ( 0.000000000000000000, 0.000000000000000000, -1.000000000000000000 ) ) ;
#34178=ORIENTED_EDGE ( 'NONE', *, *, #33725, .T. ) ;
#34179=CARTESIAN_POINT ( 'NONE',  ( -121.1142239062970276, -183.6283474603465606, 101.7307360698549417 ) ) ;
#34180=CARTESIAN_POINT ( 'NONE',  ( -105.7090724259147976, -189.7472609257535510, 111.1293539894142839 ) ) ;
#34181=CARTESIAN_POINT ( 'NONE',  ( 55.35935253854128746, -177.1207230881787780, 69.58857822035042773 ) ) ;
#34182=CARTESIAN_POINT ( 'NONE',  ( -76.79768193946081567, -175.3837268820161057, 120.7230919990160629 ) ) ;
#34184=ORIENTED_EDGE ( 'NONE', *, *, #8663, .F. ) ;
#34185=DIRECTION ( 'NONE',  ( -0.000000000000000000, 1.000000000000000000, -0.000000000000000000 ) ) ;
#34187=DIRECTION ( 'NONE',  ( -0.9890401873221623674, 0.000000000000000000, -0.1476465640024917925 ) ) ;
#34189=AXIS2_PLACEMENT_3D ( 'NONE', #20389, #39828, #4121 ) ;
#34190=VECTOR ( 'NONE', #35218, 1000.000000000000114 ) ;
#34191=CARTESIAN_POINT ( 'NONE',  ( 5.139251539934009294, -177.1207230881787780, 111.8087531435658093 ) ) ;
#34193=AXIS2_PLACEMENT_3D ( 'NONE', #12486, #15927, #31936 ) ;
#34194=DIRECTION ( 'NONE',  ( -0.5586467658036594619, 0.000000000000000000, 0.8294056854501971054 ) ) ;
#34195=ADVANCED_FACE ( 'NONE', ( #46755 ), #25742, .T. ) ;
#34196=DIRECTION ( 'NONE',  ( 0.4300652022765245608, 0.000000000000000000, -0.9027978299657416494 ) ) ;
#34198=EDGE_CURVE ( 'NONE', #1575, #46127, #10220, .T. ) ;
#34199=VECTOR ( 'NONE', #36082, 1000.000000000000000 ) ;
#34201=FACE_OUTER_BOUND ( 'NONE', #40588, .T. ) ;
#34202=CARTESIAN_POINT ( 'NONE',  ( -128.2395503755045638, -177.1207230881787780, -96.24590808611421267 ) ) ;
#34204=AXIS2_PLACEMENT_3D ( 'NONE', #8557, #20653, #8819 ) ;
#34207=AXIS2_PLACEMENT_3D ( 'NONE', #2631, #23129, #50733 ) ;
#34210=AXIS2_PLACEMENT_3D ( 'NONE', #43900, #525, #12086 ) ;
#34212=DIRECTION ( 'NONE',  ( -0.000000000000000000, -1.000000000000000000, 0.000000000000000000 ) ) ;
#34213=EDGE_LOOP ( 'NONE', ( #11021, #51656, #48320, #43524 ) ) ;
#34216=VERTEX_POINT ( 'NONE', #2598 ) ;
#34218=DIRECTION ( 'NONE',  ( 0.9027978299657477557, 0.000000000000000000, -0.4300652022765115712 ) ) ;
#34219=DIRECTION ( 'NONE',  ( -0.000000000000000000, 1.000000000000000000, -0.000000000000000000 ) ) ;
#34220=ORIENTED_EDGE ( 'NONE', *, *, #45601, .F. ) ;
#34221=CARTESIAN_POINT ( 'NONE',  ( -161.6832731452239784, -175.3837268820161057, -53.00774697410100345 ) ) ;
#34225=ORIENTED_EDGE ( 'NONE', *, *, #51330, .T. ) ;
#34228=CARTESIAN_POINT ( 'NONE',  ( -4.176930889631405464, -193.5000000000000000, 116.8859077982279615 ) ) ;
#34230=CARTESIAN_POINT ( 'NONE',  ( -156.2577088867455473, -183.6283474603465606, -63.31490529818422885 ) ) ;
#34231=VECTOR ( 'NONE', #29021, 1000.000000000000000 ) ;
#34234=CARTESIAN_POINT ( 'NONE',  ( 75.67769207106684348, -193.5000000000000000, 14.49428645563876650 ) ) ;
#34237=ORIENTED_EDGE ( 'NONE', *, *, #28367, .T. ) ;
#34238=CARTESIAN_POINT ( 'NONE',  ( -155.0851258170080769, -183.6283474603465606, 63.33473559879983128 ) ) ;
#34241=CARTESIAN_POINT ( 'NONE',  ( -113.5519059482138573, -193.5000000000000000, 105.5544085257715494 ) ) ;
#34244=LINE ( 'NONE', #6397, #16415 ) ;
#34245=CIRCLE ( 'NONE', #51890, 125.0000000000000000 ) ;
#34248=VERTEX_POINT ( 'NONE', #14686 ) ;
#34251=ORIENTED_EDGE ( 'NONE', *, *, #3057, .F. ) ;
#34255=CARTESIAN_POINT ( 'NONE',  ( -46.06708674231131084, -183.6283474603465606, -124.9767260852756863 ) ) ;
#34256=EDGE_CURVE ( 'NONE', #14713, #8894, #17444, .T. ) ;
#34257=EDGE_LOOP ( 'NONE', ( #16594, #18586, #4896, #2605 ) ) ;
#34260=AXIS2_PLACEMENT_3D ( 'NONE', #46086, #10069, #48397 ) ;
#34262=AXIS2_PLACEMENT_3D ( 'NONE', #44165, #28115, #19991 ) ;
#34263=DIRECTION ( 'NONE',  ( -0.000000000000000000, 1.000000000000000000, -0.000000000000000000 ) ) ;
#34266=ORIENTED_EDGE ( 'NONE', *, *, #20939, .F. ) ;
#34267=AXIS2_PLACEMENT_3D ( 'NONE', #1647, #33167, #41306 ) ;
#34268=VERTEX_POINT ( 'NONE', #24319 ) ;
#34270=EDGE_CURVE ( 'NONE', #39314, #28401, #27732, .T. ) ;
#34271=EDGE_CURVE ( 'NONE', #38037, #30945, #43765, .T. ) ;
#34272=DIRECTION ( 'NONE',  ( -0.6068001458185890984, 0.000000000000000000, -0.7948544414133565938 ) ) ;
#34273=AXIS2_PLACEMENT_3D ( 'NONE', #18388, #23361, #39369 ) ;
#34274=VERTEX_POINT ( 'NONE', #11707 ) ;
#34275=EDGE_CURVE ( 'NONE', #36109, #265, #20908, .T. ) ;
#34277=VERTEX_POINT ( 'NONE', #39804 ) ;
#34279=DIRECTION ( 'NONE',  ( -0.000000000000000000, 1.000000000000000000, -0.000000000000000000 ) ) ;
#34280=ADVANCED_FACE ( 'NONE', ( #12732 ), #28758, .F. ) ;
#34283=ORIENTED_EDGE ( 'NONE', *, *, #47873, .T. ) ;
#34285=ORIENTED_EDGE ( 'NONE', *, *, #32045, .F. ) ;
#34286=VECTOR ( 'NONE', #44390, 1000.000000000000114 ) ;
#34288=LINE ( 'NONE', #38728, #41137 ) ;
#34290=CARTESIAN_POINT ( 'NONE',  ( 45.24245851652179340, -183.6283474603465606, -81.19354792697733103 ) ) ;
#34291=ORIENTED_EDGE ( 'NONE', *, *, #51644, .F. ) ;
#34293=ORIENTED_EDGE ( 'NONE', *, *, #15930, .F. ) ;
#34294=ORIENTED_EDGE ( 'NONE', *, *, #22523, .F. ) ;
#34295=LINE ( 'NONE', #10376, #12210 ) ;
#34296=FACE_OUTER_BOUND ( 'NONE', #3036, .T. ) ;
#34297=AXIS2_PLACEMENT_3D ( 'NONE', #205, #16250, #32262 ) ;
#34300=AXIS2_PLACEMENT_3D ( 'NONE', #35688, #51741, #7335 ) ;
#34301=LINE ( 'NONE', #30348, #27894 ) ;
#34302=DIRECTION ( 'NONE',  ( -0.000000000000000000, 1.000000000000000000, -0.000000000000000000 ) ) ;
#34304=CARTESIAN_POINT ( 'NONE',  ( 51.05451324771860300, -193.5000000000000000, 75.61781872352698031 ) ) ;
#34306=EDGE_CURVE ( 'NONE', #8881, #33712, #18259, .T. ) ;
#34309=AXIS2_PLACEMENT_3D ( 'NONE', #39316, #2295, #6755 ) ;
#34311=VERTEX_POINT ( 'NONE', #15669 ) ;
#34312=ADVANCED_FACE ( 'NONE', ( #16444 ), #16181, .T. ) ;
#34313=PLANE ( 'NONE',  #25682 ) ;
#34314=ADVANCED_FACE ( 'NONE', ( #47977 ), #24570, .T. ) ;
#34315=DIRECTION ( 'NONE',  ( 0.000000000000000000, -0.000000000000000000, -1.000000000000000000 ) ) ;
#34316=DIRECTION ( 'NONE',  ( 0.000000000000000000, 1.000000000000000000, 0.000000000000000000 ) ) ;
#34317=EDGE_CURVE ( 'NONE', #25328, #51645, #48241, .T. ) ;
#34320=VECTOR ( 'NONE', #20932, 1000.000000000000000 ) ;
#34321=CARTESIAN_POINT ( 'NONE',  ( 26.70958190211001337, -189.7472609257535510, -99.85818990449013199 ) ) ;
#34323=ADVANCED_FACE ( 'NONE', ( #40080 ), #16713, .T. ) ;
#34327=CARTESIAN_POINT ( 'NONE',  ( 76.47090317495664635, -193.5000000000000000, -3.534122433557446374 ) ) ;
#34328=EDGE_CURVE ( 'NONE', #44193, #37366, #35875, .T. ) ;
#34329=EDGE_LOOP ( 'NONE', ( #14264, #32019, #48717, #42421 ) ) ;
#34331=DIRECTION ( 'NONE',  ( 0.000000000000000000, -1.000000000000000000, 0.000000000000000000 ) ) ;
#34332=ADVANCED_FACE ( 'NONE', ( #44302 ), #388, .T. ) ;
#34335=ORIENTED_EDGE ( 'NONE', *, *, #21803, .F. ) ;
#34336=DIRECTION ( 'NONE',  ( -0.000000000000000000, 1.000000000000000000, 0.000000000000000000 ) ) ;
#34337=MECHANICAL_DESIGN_GEOMETRIC_PRESENTATION_REPRESENTATION('',(#10041),#46957);
#34338=EDGE_CURVE ( 'NONE', #25155, #14931, #42593, .T. ) ;
#34340=LINE ( 'NONE', #49858, #19829 ) ;
#34341=ORIENTED_EDGE ( 'NONE', *, *, #14614, .F. ) ;
#34345=ADVANCED_FACE ( 'NONE', ( #16962 ), #50060, .T. ) ;
#34346=LINE ( 'NONE', #31426, #15009 ) ;
#34348=LINE ( 'NONE', #30640, #37731 ) ;
#34349=PRESENTATION_STYLE_ASSIGNMENT (( #17801 ) ) ;
#34352=VERTEX_POINT ( 'NONE', #29804 ) ;
#34354=CIRCLE ( 'NONE', #31840, 125.0000000000000000 ) ;
#34355=LINE ( 'NONE', #30650, #38311 ) ;
#34358=ORIENTED_EDGE ( 'NONE', *, *, #28541, .T. ) ;
#34360=FACE_OUTER_BOUND ( 'NONE', #46304, .T. ) ;
#34362=DIRECTION ( 'NONE',  ( -0.4300652022765304450, 0.000000000000000000, 0.9027978299657387629 ) ) ;
#34363=ORIENTED_EDGE ( 'NONE', *, *, #2896, .T. ) ;
#34365=DIRECTION ( 'NONE',  ( 0.000000000000000000, -1.000000000000000000, 0.000000000000000000 ) ) ;
#34370=LINE ( 'NONE', #43024, #10266 ) ;
#34372=AXIS2_PLACEMENT_3D ( 'NONE', #49595, #13845, #1225 ) ;
#34373=LINE ( 'NONE', #2325, #21968 ) ;
#34376=FACE_OUTER_BOUND ( 'NONE', #50868, .T. ) ;
#34380=EDGE_CURVE ( 'NONE', #14469, #41991, #11568, .T. ) ;
#34381=DIRECTION ( 'NONE',  ( 0.000000000000000000, 0.000000000000000000, 1.000000000000000000 ) ) ;
#34382=LINE ( 'NONE', #10454, #4426 ) ;
#34383=ORIENTED_EDGE ( 'NONE', *, *, #13267, .T. ) ;
#34384=CARTESIAN_POINT ( 'NONE',  ( 72.95485052494851175, -193.5000000000000000, -29.64437826672757481 ) ) ;
#34386=EDGE_CURVE ( 'NONE', #1671, #14956, #33234, .T. ) ;
#34387=EDGE_CURVE ( 'NONE', #33217, #14916, #5662, .T. ) ;
#34388=DIRECTION ( 'NONE',  ( 0.000000000000000000, 0.000000000000000000, 1.000000000000000000 ) ) ;
#34392=ORIENTED_EDGE ( 'NONE', *, *, #46878, .T. ) ;
#34393=CARTESIAN_POINT ( 'NONE',  ( 34.93559171950835918, -183.6283474603465606, -93.09664195018497423 ) ) ;
#34394=ORIENTED_EDGE ( 'NONE', *, *, #12355, .F. ) ;
#34395=VECTOR ( 'NONE', #5464, 1000.000000000000000 ) ;
#34397=EDGE_CURVE ( 'NONE', #20906, #33364, #5394, .T. ) ;
#34398=CARTESIAN_POINT ( 'NONE',  ( -70.75782287548088334, -189.7472609257535510, 122.9986166548864901 ) ) ;
#34400=LINE ( 'NONE', #7062, #17042 ) ;
#34402=DIRECTION ( 'NONE',  ( 0.000000000000000000, 1.000000000000000000, 0.000000000000000000 ) ) ;
#34403=VERTEX_POINT ( 'NONE', #46124 ) ;
#34404=EDGE_CURVE ( 'NONE', #44579, #27840, #21151, .T. ) ;
#34405=FACE_OUTER_BOUND ( 'NONE', #44289, .T. ) ;
#34406=VERTEX_POINT ( 'NONE', #10103 ) ;
#34407=DIRECTION ( 'NONE',  ( -0.000000000000000000, 1.000000000000000000, -0.000000000000000000 ) ) ;
#34409=ORIENTED_EDGE ( 'NONE', *, *, #43576, .T. ) ;
#34414=DIRECTION ( 'NONE',  ( 0.000000000000000000, 1.000000000000000000, -0.000000000000000000 ) ) ;
#34415=PLANE ( 'NONE',  #13837 ) ;
#34416=VERTEX_POINT ( 'NONE', #25111 ) ;
#34417=DIRECTION ( 'NONE',  ( 0.8455960035018199594, 0.000000000000000000, 0.5338233779648003940 ) ) ;
#34420=ORIENTED_EDGE ( 'NONE', *, *, #34011, .T. ) ;
#34421=CARTESIAN_POINT ( 'NONE',  ( -40.30502441601360886, -189.7472609257535510, 123.7303097900624920 ) ) ;
#34422=CARTESIAN_POINT ( 'NONE',  ( -48.47912675150885065, -189.7472609257535510, 6.938893903907228378E-15 ) ) ;
#34423=DIRECTION ( 'NONE',  ( -0.000000000000000000, 1.000000000000000000, 0.000000000000000000 ) ) ;
#34425=VERTEX_POINT ( 'NONE', #26119 ) ;
#34426=VECTOR ( 'NONE', #39504, 1000.000000000000000 ) ;
#34427=AXIS2_PLACEMENT_3D ( 'NONE', #31075, #43163, #15847 ) ;
#34428=CARTESIAN_POINT ( 'NONE',  ( -68.21229068036657850, -193.5000000000000000, -123.4325817657429809 ) ) ;
#34429=ORIENTED_EDGE ( 'NONE', *, *, #35608, .T. ) ;
#34430=DIRECTION ( 'NONE',  ( 0.000000000000000000, 1.000000000000000000, 0.000000000000000000 ) ) ;
#34431=CARTESIAN_POINT ( 'NONE',  ( -169.1033029113419559, -193.5000000000000000, 32.78426643622745473 ) ) ;
#34432=ORIENTED_EDGE ( 'NONE', *, *, #4271, .F. ) ;
#34433=DIRECTION ( 'NONE',  ( 0.02963332782254913048, 0.000000000000000000, 0.9995608365087946812 ) ) ;
#34434=CARTESIAN_POINT ( 'NONE',  ( 74.77174840718836890, -183.6283474603465606, 20.83798868929603643 ) ) ;
#34435=LINE ( 'NONE', #6596, #44209 ) ;
#34439=EDGE_CURVE ( 'NONE', #42496, #35050, #9849, .T. ) ;
#34440=DIRECTION ( 'NONE',  ( -0.05924062789370006937, 0.000000000000000000, -0.9982437317643222396 ) ) ;
#34441=LINE ( 'NONE', #2116, #44081 ) ;
#34443=ORIENTED_EDGE ( 'NONE', *, *, #4211, .T. ) ;
#34444=AXIS2_PLACEMENT_3D ( 'NONE', #4943, #20698, #45153 ) ;
#34445=LINE ( 'NONE', #51015, #34075 ) ;
#34447=CARTESIAN_POINT ( 'NONE',  ( 30.67449672666758431, -193.5000000000000000, 95.45105364470144593 ) ) ;
#34448=LINE ( 'NONE', #14491, #5657 ) ;
#34449=EDGE_LOOP ( 'NONE', ( #8847, #5294, #35220, #20612 ) ) ;
#34450=PLANE ( 'NONE',  #13701 ) ;
#34451=PRODUCT_DEFINITION ( 'UNKNOWN', '', #32599, #25373 ) ;
#34454=PLANE ( 'NONE',  #47230 ) ;
#34457=DIRECTION ( 'NONE',  ( 0.000000000000000000, 1.000000000000000000, 0.000000000000000000 ) ) ;
#34459=AXIS2_PLACEMENT_3D ( 'NONE', #24482, #8715, #40764 ) ;
#34460=CARTESIAN_POINT ( 'NONE',  ( -130.2106798473772926, -175.3837268820161057, 94.57776286494220130 ) ) ;
#34461=ORIENTED_EDGE ( 'NONE', *, *, #46073, .T. ) ;
#34462=ORIENTED_EDGE ( 'NONE', *, *, #11531, .T. ) ;
#34463=EDGE_LOOP ( 'NONE', ( #13739, #33339, #18350, #21089 ) ) ;
#34467=FACE_OUTER_BOUND ( 'NONE', #51493, .T. ) ;
#34469=FACE_OUTER_BOUND ( 'NONE', #36894, .T. ) ;
#34472=CARTESIAN_POINT ( 'NONE',  ( -62.32061382540516092, -189.7472609257535510, 123.2250735253144285 ) ) ;
#34473=ORIENTED_EDGE ( 'NONE', *, *, #29856, .T. ) ;
#34475=CARTESIAN_POINT ( 'NONE',  ( -48.41988612361514299, -193.5000000000000000, -0.9982437317643144681 ) ) ;
#34480=CARTESIAN_POINT ( 'NONE',  ( -49.29161362951453640, -193.5000000000000000, 0.5829794791144718991 ) ) ;
#34481=CARTESIAN_POINT ( 'NONE',  ( -44.48323084606168720, -177.1207230881787780, 124.9361149384469769 ) ) ;
#34483=ORIENTED_EDGE ( 'NONE', *, *, #2802, .T. ) ;
#34484=FACE_OUTER_BOUND ( 'NONE', #18821, .T. ) ;
#34485=PLANE ( 'NONE',  #35082 ) ;
#34486=VERTEX_POINT ( 'NONE', #2215 ) ;
#34487=CARTESIAN_POINT ( 'NONE',  ( 72.05536924052414349, -189.7472609257535510, 33.11246405730899056 ) ) ;
#34488=VECTOR ( 'NONE', #570, 1000.000000000000000 ) ;
#34489=CARTESIAN_POINT ( 'NONE',  ( -75.48985759771373694, -183.6283474603465606, -122.0467960216648748 ) ) ;
#34490=ORIENTED_EDGE ( 'NONE', *, *, #32708, .T. ) ;
#34491=EDGE_CURVE ( 'NONE', #26145, #4313, #9067, .T. ) ;
#34495=VERTEX_POINT ( 'NONE', #6934 ) ;
#34498=EDGE_CURVE ( 'NONE', #15701, #35294, #39250, .T. ) ;
#34499=DIRECTION ( 'NONE',  ( -0.1182731709213523247, 0.000000000000000000, -0.9929810960135185827 ) ) ;
#34502=DIRECTION ( 'NONE',  ( 0.9646355819083576311, 0.000000000000000000, 0.2635871660690715101 ) ) ;
#34503=DIRECTION ( 'NONE',  ( 0.000000000000000000, 0.000000000000000000, -1.000000000000000000 ) ) ;
#34504=DIRECTION ( 'NONE',  ( -0.000000000000000000, 1.000000000000000000, -0.000000000000000000 ) ) ;
#34505=ORIENTED_EDGE ( 'NONE', *, *, #31463, .T. ) ;
#34506=DIRECTION ( 'NONE',  ( 0.000000000000000000, -1.000000000000000000, -0.000000000000000000 ) ) ;
#34507=ORIENTED_EDGE ( 'NONE', *, *, #44228, .T. ) ;
#34510=DIRECTION ( 'NONE',  ( -0.000000000000000000, 1.000000000000000000, -0.000000000000000000 ) ) ;
#34512=VERTEX_POINT ( 'NONE', #38973 ) ;
#34513=VERTEX_POINT ( 'NONE', #18258 ) ;
#34514=DIRECTION ( 'NONE',  ( -0.000000000000000000, 1.000000000000000000, -0.000000000000000000 ) ) ;
#34515=DIRECTION ( 'NONE',  ( 0.4566292373937018145, 0.000000000000000000, 0.8896570909947529859 ) ) ;
#34517=DIRECTION ( 'NONE',  ( -0.000000000000000000, 1.000000000000000000, -0.000000000000000000 ) ) ;
#34518=VERTEX_POINT ( 'NONE', #14571 ) ;
#34520=CARTESIAN_POINT ( 'NONE',  ( -171.0948786228703113, -175.3837268820161057, -18.47640724094507192 ) ) ;
#34521=VECTOR ( 'NONE', #3805, 999.9999999999998863 ) ;
#34524=VECTOR ( 'NONE', #49318, 1000.000000000000000 ) ;
#34527=AXIS2_PLACEMENT_3D ( 'NONE', #13048, #24123, #40131 ) ;
#34528=VERTEX_POINT ( 'NONE', #22966 ) ;
#34529=LINE ( 'NONE', #46130, #37540 ) ;
#34532=DIRECTION ( 'NONE',  ( -0.6749830015182196608, 0.000000000000000000, 0.7378332790417189146 ) ) ;
#34534=EDGE_CURVE ( 'NONE', #1446, #30190, #22708, .T. ) ;
#34535=EDGE_CURVE ( 'NONE', #19679, #3624, #10619, .T. ) ;
#34537=VECTOR ( 'NONE', #34818, 1000.000000000000000 ) ;
#34538=ORIENTED_EDGE ( 'NONE', *, *, #31655, .F. ) ;
#34539=ORIENTED_EDGE ( 'NONE', *, *, #37420, .F. ) ;
#34541=CIRCLE ( 'NONE', #17790, 125.0000000000000000 ) ;
#34542=CARTESIAN_POINT ( 'NONE',  ( 75.48400724637755843, -183.6283474603465606, -16.06677968424457958 ) ) ;
#34545=CARTESIAN_POINT ( 'NONE',  ( -131.8938452225253855, -183.6283474603465606, 93.09664195018558530 ) ) ;
#34546=ORIENTED_EDGE ( 'NONE', *, *, #45212, .F. ) ;
#34547=EDGE_CURVE ( 'NONE', #17157, #15990, #18763, .T. ) ;
#34548=CARTESIAN_POINT ( 'NONE',  ( 20.66186849114819069, -175.3837268820161057, -104.1370384486464928 ) ) ;
#34551=CARTESIAN_POINT ( 'NONE',  ( -19.18792875895802652, -189.7472609257535510, -120.4907712303050715 ) ) ;
#34552=EDGE_CURVE ( 'NONE', #36214, #46127, #22501, .T. ) ;
#34554=ORIENTED_EDGE ( 'NONE', *, *, #36766, .F. ) ;
#34555=CIRCLE ( 'NONE', #42103, 125.0000000000000000 ) ;
#34556=ADVANCED_FACE ( 'NONE', ( #31096 ), #34772, .T. ) ;
#34557=DIRECTION ( 'NONE',  ( -0.000000000000000000, 1.000000000000000000, 0.000000000000000000 ) ) ;
#34558=CARTESIAN_POINT ( 'NONE',  ( -155.9155026329808607, -177.1207230881787780, -61.91627321685029983 ) ) ;
#34559=DIRECTION ( 'NONE',  ( 0.000000000000000000, -1.000000000000000000, 0.000000000000000000 ) ) ;
#34565=DIRECTION ( 'NONE',  ( 0.000000000000000000, 1.000000000000000000, 0.000000000000000000 ) ) ;
#34567=ORIENTED_EDGE ( 'NONE', *, *, #31161, .F. ) ;
#34568=CARTESIAN_POINT ( 'NONE',  ( -48.47912675150885065, -175.3837268820161057, 6.938893903907228378E-15 ) ) ;
#34570=VECTOR ( 'NONE', #5057, 1000.000000000000000 ) ;
#34572=CIRCLE ( 'NONE', #9425, 125.0000000000000000 ) ;
#34573=AXIS2_PLACEMENT_3D ( 'NONE', #1710, #13538, #46133 ) ;
#34574=ORIENTED_EDGE ( 'NONE', *, *, #29331, .T. ) ;
#34575=CARTESIAN_POINT ( 'NONE',  ( -123.6678354051270077, -189.7472609257535510, 99.85818990449067201 ) ) ;
#34578=FACE_OUTER_BOUND ( 'NONE', #50504, .T. ) ;
#34580=DIRECTION ( 'NONE',  ( -0.000000000000000000, 1.000000000000000000, 0.000000000000000000 ) ) ;
#34583=EDGE_LOOP ( 'NONE', ( #41518, #37258, #21563, #28281 ) ) ;
#34585=LINE ( 'NONE', #34842, #28483 ) ;
#34586=FACE_OUTER_BOUND ( 'NONE', #3779, .T. ) ;
#34587=CARTESIAN_POINT ( 'NONE',  ( -47.55243714407701816, -183.6283474603465606, -0.3758275821142288420 ) ) ;
#34589=VECTOR ( 'NONE', #30170, 1000.000000000000227 ) ;
#34591=EDGE_CURVE ( 'NONE', #34528, #5079, #9889, .T. ) ;
#34592=EDGE_CURVE ( 'NONE', #32588, #16076, #18296, .T. ) ;
#34593=EDGE_CURVE ( 'NONE', #10828, #45319, #2481, .T. ) ;
#34594=EDGE_CURVE ( 'NONE', #23726, #34940, #48539, .T. ) ;
#34595=VECTOR ( 'NONE', #24690, 1000.000000000000114 ) ;
#34597=EDGE_LOOP ( 'NONE', ( #24865, #8483, #47103, #44280 ) ) ;
#34598=DIRECTION ( 'NONE',  ( 0.000000000000000000, 0.000000000000000000, 1.000000000000000000 ) ) ;
#34600=VERTEX_POINT ( 'NONE', #34520 ) ;
#34601=EDGE_CURVE ( 'NONE', #41076, #7058, #47669, .T. ) ;
#34604=EDGE_LOOP ( 'NONE', ( #27717, #16909, #8891, #45868 ) ) ;
#34607=CARTESIAN_POINT ( 'NONE',  ( 41.40822382563629134, -193.5000000000000000, 85.41934182508082074 ) ) ;
#34609=EDGE_CURVE ( 'NONE', #3937, #5817, #40106, .T. ) ;
#34610=LINE ( 'NONE', #26467, #16639 ) ;
#34611=VERTEX_POINT ( 'NONE', #43459 ) ;
#34612=AXIS2_PLACEMENT_3D ( 'NONE', #51525, #22891, #31539 ) ;
#34613=AXIS2_PLACEMENT_3D ( 'NONE', #37136, #4308, #49245 ) ;
#34614=EDGE_CURVE ( 'NONE', #27304, #22201, #14093, .T. ) ;
#34615=ORIENTED_EDGE ( 'NONE', *, *, #32883, .F. ) ;
#34616=CARTESIAN_POINT ( 'NONE',  ( -55.05561436132772002, -189.7472609257535510, 124.8268793598474105 ) ) ;
#34617=CIRCLE ( 'NONE', #18690, 9.999999999999994671 ) ;
#34618=CARTESIAN_POINT ( 'NONE',  ( -108.5723883981723930, -193.5000000000000000, 109.6074810615846360 ) ) ;
#34619=AXIS2_PLACEMENT_3D ( 'NONE', #5161, #49308, #4904 ) ;
#34621=DIRECTION ( 'NONE',  ( -0.000000000000000000, -1.000000000000000000, 0.000000000000000000 ) ) ;
#34622=ORIENTED_EDGE ( 'NONE', *, *, #16805, .T. ) ;
#34624=DIRECTION ( 'NONE',  ( -0.05924062789372142729, 0.000000000000000000, 0.9982437317643209074 ) ) ;
#34626=PLANE ( 'NONE',  #46475 ) ;
#34628=EDGE_LOOP ( 'NONE', ( #45529, #12421, #23802, #37811 ) ) ;
#34629=DIRECTION ( 'NONE',  ( 0.000000000000000000, 0.000000000000000000, 1.000000000000000000 ) ) ;
#34631=DIRECTION ( 'NONE',  ( 0.9473263538541899509, 0.000000000000000000, 0.3202698538628415692 ) ) ;
#34632=ORIENTED_EDGE ( 'NONE', *, *, #16997, .T. ) ;
#34634=AXIS2_PLACEMENT_3D ( 'NONE', #3343, #40114, #20146 ) ;
#34635=CYLINDRICAL_SURFACE ( 'NONE', #25276, 9.999999999999994671 ) ;
#34637=DIRECTION ( 'NONE',  ( 0.000000000000000000, 0.000000000000000000, 1.000000000000000000 ) ) ;
#34638=ORIENTED_EDGE ( 'NONE', *, *, #34047, .T. ) ;
#34639=EDGE_CURVE ( 'NONE', #42167, #50918, #4031, .T. ) ;
#34640=AXIS2_PLACEMENT_3D ( 'NONE', #25223, #48888, #37298 ) ;
#34641=PLANE ( 'NONE',  #22599 ) ;
#34642=CARTESIAN_POINT ( 'NONE',  ( -164.2512865680372727, -175.3837268820161057, -47.13604789772047354 ) ) ;
#34643=DIRECTION ( 'NONE',  ( 0.000000000000000000, 1.000000000000000000, -0.000000000000000000 ) ) ;
#34645=DIRECTION ( 'NONE',  ( -0.8455960035018199594, 0.000000000000000000, -0.5338233779648003940 ) ) ;
#34646=CIRCLE ( 'NONE', #10351, 125.0000000000000000 ) ;
#34647=VECTOR ( 'NONE', #22050, 999.9999999999998863 ) ;
#34650=ORIENTED_EDGE ( 'NONE', *, *, #41670, .T. ) ;
#34652=CARTESIAN_POINT ( 'NONE',  ( 47.28479244271900939, -175.3837268820161057, -78.77358243914883928 ) ) ;
#34653=CIRCLE ( 'NONE', #31315, 125.0000000000000000 ) ;
#34655=DIRECTION ( 'NONE',  ( -0.000000000000000000, 1.000000000000000000, -0.000000000000000000 ) ) ;
#34657=EDGE_CURVE ( 'NONE', #6242, #20061, #45167, .T. ) ;
#34658=EDGE_CURVE ( 'NONE', #23290, #42327, #28691, .T. ) ;
#34660=ADVANCED_FACE ( 'NONE', ( #12414 ), #11650, .T. ) ;
#34661=DIRECTION ( 'NONE',  ( -0.000000000000000000, 1.000000000000000000, -0.000000000000000000 ) ) ;
#34663=VERTEX_POINT ( 'NONE', #36075 ) ;
#34664=DIRECTION ( 'NONE',  ( 0.000000000000000000, 0.000000000000000000, 1.000000000000000000 ) ) ;
#34665=ORIENTED_EDGE ( 'NONE', *, *, #33800, .T. ) ;
#34666=FACE_OUTER_BOUND ( 'NONE', #42997, .T. ) ;
#34667=ORIENTED_EDGE ( 'NONE', *, *, #21032, .T. ) ;
#34668=LINE ( 'NONE', #6825, #27231 ) ;
#34669=VECTOR ( 'NONE', #47055, 999.9999999999998863 ) ;
#34670=ORIENTED_EDGE ( 'NONE', *, *, #14747, .F. ) ;
#34671=LINE ( 'NONE', #38363, #51077 ) ;
#34672=LINE ( 'NONE', #27041, #29138 ) ;
#34674=EDGE_LOOP ( 'NONE', ( #13632, #27652, #49701, #15200 ) ) ;
#34677=FACE_OUTER_BOUND ( 'NONE', #17797, .T. ) ;
#34679=CARTESIAN_POINT ( 'NONE',  ( -159.0901268547125653, -183.6283474603465606, 58.22548115875957109 ) ) ;
#34683=CARTESIAN_POINT ( 'NONE',  ( -76.79768193946077304, -193.5000000000000000, 120.7230919990160771 ) ) ;
#34684=DIRECTION ( 'NONE',  ( 0.000000000000000000, 0.000000000000000000, 1.000000000000000000 ) ) ;
#34685=PLANE ( 'NONE',  #23256 ) ;
#34687=CARTESIAN_POINT ( 'NONE',  ( 49.10711742958949344, -175.3837268820161057, 78.11481899503480975 ) ) ;
#34688=ADVANCED_FACE ( 'NONE', ( #28440 ), #3751, .T. ) ;
#34689=ORIENTED_EDGE ( 'NONE', *, *, #10937, .F. ) ;
#34690=VECTOR ( 'NONE', #5874, 1000.000000000000114 ) ;
#34691=CARTESIAN_POINT ( 'NONE',  ( -151.9915035862630646, -177.1207230881787780, 70.07273251429430161 ) ) ;
#34692=DIRECTION ( 'NONE',  ( 0.000000000000000000, 0.000000000000000000, 1.000000000000000000 ) ) ;
#34694=CARTESIAN_POINT ( 'NONE',  ( -48.47912675150885065, -177.1207230881787780, 6.938893903907228378E-15 ) ) ;
#34695=VERTEX_POINT ( 'NONE', #20297 ) ;
#34696=AXIS2_PLACEMENT_3D ( 'NONE', #40107, #47757, #3859 ) ;
#34697=LINE ( 'NONE', #3414, #26526 ) ;
#34698=DIRECTION ( 'NONE',  ( -0.000000000000000000, 1.000000000000000000, -0.000000000000000000 ) ) ;
#34699=CARTESIAN_POINT ( 'NONE',  ( 5.542374969221969039, -183.6283474603465606, 112.7238987608088223 ) ) ;
#34700=CARTESIAN_POINT ( 'NONE',  ( 44.58442300236217903, -193.5000000000000000, -81.94739446021067408 ) ) ;
#34704=LINE ( 'NONE', #26050, #37913 ) ;
#34705=LINE ( 'NONE', #49979, #30436 ) ;
#34706=LINE ( 'NONE', #19454, #23697 ) ;
#34707=VECTOR ( 'NONE', #6270, 1000.000000000000000 ) ;
#34708=VERTEX_POINT ( 'NONE', #36330 ) ;
#34709=LINE ( 'NONE', #37171, #39420 ) ;
#34710=CIRCLE ( 'NONE', #16266, 125.0000000000000000 ) ;
#34712=ORIENTED_EDGE ( 'NONE', *, *, #12235, .F. ) ;
#34713=EDGE_LOOP ( 'NONE', ( #5229, #51715, #31881, #47257 ) ) ;
#34715=CARTESIAN_POINT ( 'NONE',  ( 11.10560377650620723, -193.5000000000000000, -108.7464374498168951 ) ) ;
#34716=EDGE_CURVE ( 'NONE', #41529, #37529, #51594, .T. ) ;
#34717=ADVANCED_FACE ( 'NONE', ( #15600 ), #43958, .T. ) ;
#34718=FACE_OUTER_BOUND ( 'NONE', #22216, .T. ) ;
#34719=CARTESIAN_POINT ( 'NONE',  ( -49.13194886969938580, -193.5000000000000000, 0.7575112421616214675 ) ) ;
#34720=AXIS2_PLACEMENT_3D ( 'NONE', #4679, #26834, #3631 ) ;
#34721=EDGE_LOOP ( 'NONE', ( #51403, #21495, #45510, #2148 ) ) ;
#34724=DIRECTION ( 'NONE',  ( 0.000000000000000000, 0.000000000000000000, -1.000000000000000000 ) ) ;
#34725=CARTESIAN_POINT ( 'NONE',  ( -56.65322908700500193, -189.7472609257535510, -123.7303097900624351 ) ) ;
#34726=EDGE_LOOP ( 'NONE', ( #31671, #51789, #20488, #8724 ) ) ;
#34729=PLANE ( 'NONE',  #49915 ) ;
#34732=DIRECTION ( 'NONE',  ( -0.000000000000000000, 1.000000000000000000, -0.000000000000000000 ) ) ;
#34733=DIRECTION ( 'NONE',  ( 0.000000000000000000, 0.000000000000000000, -1.000000000000000000 ) ) ;
#34735=VERTEX_POINT ( 'NONE', #4541 ) ;
#34736=DIRECTION ( 'NONE',  ( 0.000000000000000000, -1.000000000000000000, 0.000000000000000000 ) ) ;
#34737=DIRECTION ( 'NONE',  ( -0.9151456172430181280, 0.000000000000000000, -0.4031234292879730674 ) ) ;
#34738=EDGE_LOOP ( 'NONE', ( #35632, #51825, #23208, #40477 ) ) ;
#34739=ADVANCED_FACE ( 'NONE', ( #16643 ), #32653, .T. ) ;
#34740=CARTESIAN_POINT ( 'NONE',  ( -12.76653800058364574, -193.5000000000000000, -119.7898618611244927 ) ) ;
#34746=DIRECTION ( 'NONE',  ( -0.000000000000000000, 1.000000000000000000, -0.000000000000000000 ) ) ;
#34747=VECTOR ( 'NONE', #41676, 1000.000000000000114 ) ;
#34748=EDGE_CURVE ( 'NONE', #10180, #6855, #29200, .T. ) ;
#34750=CARTESIAN_POINT ( 'NONE',  ( -167.6453766917639427, -183.6283474603465606, 37.74128873232410086 ) ) ;
#34752=CARTESIAN_POINT ( 'NONE',  ( -157.5429198988176438, -189.7472609257535510, 61.07445476073480961 ) ) ;
#34754=VERTEX_POINT ( 'NONE', #13212 ) ;
#34755=FACE_OUTER_BOUND ( 'NONE', #11557, .T. ) ;
#34759=ORIENTED_EDGE ( 'NONE', *, *, #5448, .T. ) ;
#34760=CARTESIAN_POINT ( 'NONE',  ( 141.7825277784304205, -213.5000000000000000, 41.45482488023466772 ) ) ;
#34761=CYLINDRICAL_SURFACE ( 'NONE', #47969, 125.0000000000000000 ) ;
#34762=CARTESIAN_POINT ( 'NONE',  ( -173.2419626162308646, -183.6283474603465606, 7.696413904698412800 ) ) ;
#34763=DIRECTION ( 'NONE',  ( 0.000000000000000000, 0.000000000000000000, 1.000000000000000000 ) ) ;
#34765=ORIENTED_EDGE ( 'NONE', *, *, #3295, .T. ) ;
#34766=LINE ( 'NONE', #38197, #24929 ) ;
#34767=DIRECTION ( 'NONE',  ( 0.9960498426152165630, 0.000000000000000000, 0.08879589532293852283 ) ) ;
#34769=DIRECTION ( 'NONE',  ( -0.000000000000000000, 1.000000000000000000, -0.000000000000000000 ) ) ;
#34770=ORIENTED_EDGE ( 'NONE', *, *, #37525, .F. ) ;
#34771=DIRECTION ( 'NONE',  ( -0.000000000000000000, 1.000000000000000000, -0.000000000000000000 ) ) ;
#34772=PLANE ( 'NONE',  #4871 ) ;
#34773=VECTOR ( 'NONE', #8690, 1000.000000000000114 ) ;
#34774=VECTOR ( 'NONE', #39482, 1000.000000000000114 ) ;
#34775=ADVANCED_FACE ( 'NONE', ( #37643 ), #37110, .T. ) ;
#34776=CARTESIAN_POINT ( 'NONE',  ( -173.4724443937511751, -193.5000000000000000, 1.292495564989516454 ) ) ;
#34778=EDGE_LOOP ( 'NONE', ( #20394, #39941, #24197, #49671 ) ) ;
#34779=EDGE_LOOP ( 'NONE', ( #47629, #50385, #533, #9015 ) ) ;
#34780=CIRCLE ( 'NONE', #42329, 125.0000000000000000 ) ;
#34783=CARTESIAN_POINT ( 'NONE',  ( -115.4536696835168641, -177.1207230881787780, -105.5434062319793185 ) ) ;
#34784=EDGE_CURVE ( 'NONE', #17312, #39795, #14963, .T. ) ;
#34785=CARTESIAN_POINT ( 'NONE',  ( -46.06708674231131084, -183.6283474603465606, -124.9767260852756863 ) ) ;
#34788=AXIS2_PLACEMENT_3D ( 'NONE', #19305, #47680, #31367 ) ;
#34790=DIRECTION ( 'NONE',  ( -0.9266896074318317078, 0.000000000000000000, -0.3758275821142421647 ) ) ;
#34792=VERTEX_POINT ( 'NONE', #33451 ) ;
#34794=CARTESIAN_POINT ( 'NONE',  ( -16.10442403432825387, -183.6283474603465606, -119.6996507684850428 ) ) ;
#34796=EDGE_CURVE ( 'NONE', #9382, #24476, #32533, .T. ) ;
#34798=DIRECTION ( 'NONE',  ( -0.000000000000000000, 1.000000000000000000, -0.000000000000000000 ) ) ;
#34800=ORIENTED_EDGE ( 'NONE', *, *, #10006, .T. ) ;
#34803=DIRECTION ( 'NONE',  ( -0.000000000000000000, 1.000000000000000000, -0.000000000000000000 ) ) ;
#34807=VECTOR ( 'NONE', #11669, 1000.000000000000000 ) ;
#34808=AXIS2_PLACEMENT_3D ( 'NONE', #23335, #35395, #27763 ) ;
#34809=FACE_OUTER_BOUND ( 'NONE', #8213, .T. ) ;
#34811=DIRECTION ( 'NONE',  ( 0.000000000000000000, -1.000000000000000000, 0.000000000000000000 ) ) ;
#34814=LINE ( 'NONE', #25915, #39542 ) ;
#34818=DIRECTION ( 'NONE',  ( -0.000000000000000000, 1.000000000000000000, -0.000000000000000000 ) ) ;
#34819=VERTEX_POINT ( 'NONE', #41053 ) ;
#34820=VECTOR ( 'NONE', #47457, 1000.000000000000000 ) ;
#34821=EDGE_CURVE ( 'NONE', #2545, #22186, #17930, .T. ) ;
#34822=ORIENTED_EDGE ( 'NONE', *, *, #38400, .T. ) ;
#34823=AXIS2_PLACEMENT_3D ( 'NONE', #12365, #16852, #12884 ) ;
#34825=EDGE_CURVE ( 'NONE', #194, #35836, #3167, .T. ) ;
#34826=CIRCLE ( 'NONE', #47454, 125.0000000000000000 ) ;
#34827=CARTESIAN_POINT ( 'NONE',  ( -164.2529447963538871, -183.6283474603465606, 44.41421852208711840 ) ) ;
#34830=CARTESIAN_POINT ( 'NONE',  ( -59.81005805956448995, -177.1207230881787780, -123.4817304940906126 ) ) ;
#34831=ORIENTED_EDGE ( 'NONE', *, *, #8351, .T. ) ;
#34832=CARTESIAN_POINT ( 'NONE',  ( 27.50603775690333563, -193.5000000000000000, -99.25348746834811209 ) ) ;
#34833=ADVANCED_FACE ( 'NONE', ( #13469 ), #1106, .T. ) ;
#34836=ORIENTED_EDGE ( 'NONE', *, *, #25980, .T. ) ;
#34837=ORIENTED_EDGE ( 'NONE', *, *, #46564, .T. ) ;
#34838=EDGE_CURVE ( 'NONE', #993, #51627, #5783, .T. ) ;
#34839=ADVANCED_FACE ( 'NONE', ( #33937 ), #17154, .T. ) ;
#34840=ORIENTED_EDGE ( 'NONE', *, *, #33000, .T. ) ;
#34841=LINE ( 'NONE', #10419, #12467 ) ;
#34842=CARTESIAN_POINT ( 'NONE',  ( -122.3978016498073345, -193.5000000000000000, -100.8019320314827070 ) ) ;
#34843=EDGE_CURVE ( 'NONE', #19400, #21155, #49216, .T. ) ;
#34844=VECTOR ( 'NONE', #38892, 1000.000000000000000 ) ;
#34845=DIRECTION ( 'NONE',  ( -0.000000000000000000, 1.000000000000000000, -0.000000000000000000 ) ) ;
#34846=VECTOR ( 'NONE', #13234, 1000.000000000000000 ) ;
#34851=AXIS2_PLACEMENT_3D ( 'NONE', #48023, #43813, #23843 ) ;
#34852=CARTESIAN_POINT ( 'NONE',  ( -12.76653800058363863, -175.3837268820161057, -119.7898618611245070 ) ) ;
#34853=ORIENTED_EDGE ( 'NONE', *, *, #17232, .F. ) ;
#34854=DIRECTION ( 'NONE',  ( 0.000000000000000000, 1.000000000000000000, -0.000000000000000000 ) ) ;
#34856=ORIENTED_EDGE ( 'NONE', *, *, #19254, .F. ) ;
#34857=CARTESIAN_POINT ( 'NONE',  ( -48.47912675150885065, -177.1207230881787780, 6.938893903907228378E-15 ) ) ;
#34859=DIRECTION ( 'NONE',  ( 0.000000000000000000, 0.000000000000000000, 1.000000000000000000 ) ) ;
#34860=VECTOR ( 'NONE', #9623, 1000.000000000000000 ) ;
#34861=DIRECTION ( 'NONE',  ( 0.000000000000000000, 0.000000000000000000, 1.000000000000000000 ) ) ;
#34862=LINE ( 'NONE', #50923, #44377 ) ;
#34863=VERTEX_POINT ( 'NONE', #1374 ) ;
#34864=DIRECTION ( 'NONE',  ( -0.9564009842765264224, 0.000000000000000000, 0.2920567706369628924 ) ) ;
#34865=VECTOR ( 'NONE', #37003, 1000.000000000000114 ) ;
#34866=ORIENTED_EDGE ( 'NONE', *, *, #17495, .T. ) ;
#34869=CARTESIAN_POINT ( 'NONE',  ( 65.79610465833508215, -177.1207230881787780, -50.65739320401928580 ) ) ;
#34870=DIRECTION ( 'NONE',  ( -0.000000000000000000, 1.000000000000000000, -0.000000000000000000 ) ) ;
#34871=DIRECTION ( 'NONE',  ( 0.000000000000000000, -0.000000000000000000, -1.000000000000000000 ) ) ;
#34874=CARTESIAN_POINT ( 'NONE',  ( 15.23368049493606335, -189.7472609257535510, -107.5438431188757136 ) ) ;
#34876=FACE_OUTER_BOUND ( 'NONE', #39468, .T. ) ;
#34877=ORIENTED_EDGE ( 'NONE', *, *, #38966, .T. ) ;
#34878=DIRECTION ( 'NONE',  ( 0.000000000000000000, -1.000000000000000000, 0.000000000000000000 ) ) ;
#34881=ORIENTED_EDGE ( 'NONE', *, *, #37816, .F. ) ;
#34882=VECTOR ( 'NONE', #22100, 1000.000000000000114 ) ;
#34885=VECTOR ( 'NONE', #6897, 1000.000000000000000 ) ;
#34886=DIRECTION ( 'NONE',  ( -0.000000000000000000, 1.000000000000000000, -0.000000000000000000 ) ) ;
#34887=EDGE_CURVE ( 'NONE', #7641, #31987, #9784, .T. ) ;
#34888=ORIENTED_EDGE ( 'NONE', *, *, #47907, .T. ) ;
#34889=EDGE_CURVE ( 'NONE', #21667, #20982, #31749, .T. ) ;
#34890=CARTESIAN_POINT ( 'NONE',  ( 69.88207517204676833, -189.7472609257535510, 40.19484891390058579 ) ) ;
#34891=ORIENTED_EDGE ( 'NONE', *, *, #7951, .T. ) ;
#34892=DIRECTION ( 'NONE',  ( -0.4827922027307427477, 0.000000000000000000, -0.8757349421956379665 ) ) ;
#34893=FACE_BOUND ( 'NONE', #50472, .T. ) ;
#34894=AXIS2_PLACEMENT_3D ( 'NONE', #36036, #31569, #15295 ) ;
#34895=CARTESIAN_POINT ( 'NONE',  ( 70.49476099643868565, -193.5000000000000000, 34.94873081740416154 ) ) ;
#34897=CIRCLE ( 'NONE', #29047, 125.0000000000000000 ) ;
#34899=AXIS2_PLACEMENT_3D ( 'NONE', #21991, #30913, #14903 ) ;
#34900=DIRECTION ( 'NONE',  ( 0.000000000000000000, -0.000000000000000000, 1.000000000000000000 ) ) ;
#34901=ORIENTED_EDGE ( 'NONE', *, *, #11935, .F. ) ;
#34902=EDGE_CURVE ( 'NONE', #15667, #26081, #25812, .T. ) ;
#34903=ORIENTED_EDGE ( 'NONE', *, *, #38703, .F. ) ;
#34906=EDGE_CURVE ( 'NONE', #30515, #14242, #14768, .T. ) ;
#34907=ORIENTED_EDGE ( 'NONE', *, *, #20807, .F. ) ;
#34908=CARTESIAN_POINT ( 'NONE',  ( 73.87536152799695799, -189.7472609257535510, -25.58083653558412252 ) ) ;
#34909=ADVANCED_FACE ( 'NONE', ( #30782 ), #14249, .F. ) ;
#34911=CARTESIAN_POINT ( 'NONE',  ( -118.1688136093591908, -175.3837268820161057, -103.7706487676296661 ) ) ;
#34912=ORIENTED_EDGE ( 'NONE', *, *, #48234, .F. ) ;
#34913=DIRECTION ( 'NONE',  ( -0.9785564922995017012, 0.000000000000000000, -0.2059786187411094538 ) ) ;
#34914=CARTESIAN_POINT ( 'NONE',  ( 30.50828161901820224, -193.5000000000000000, 96.88131563365348597 ) ) ;
#34915=EDGE_LOOP ( 'NONE', ( #38074, #29072, #46444, #10693 ) ) ;
#34916=AXIS2_PLACEMENT_3D ( 'NONE', #40624, #28804, #12775 ) ;
#34918=DIRECTION ( 'NONE',  ( -0.000000000000000000, 1.000000000000000000, -0.000000000000000000 ) ) ;
#34919=AXIS2_PLACEMENT_3D ( 'NONE', #16924, #5886, #33976 ) ;
#34924=PLANE ( 'NONE',  #36798 ) ;
#34926=CARTESIAN_POINT ( 'NONE',  ( -165.5546359831674295, -177.1207230881787780, 43.79868877201493405 ) ) ;
#34927=DIRECTION ( 'NONE',  ( 0.8610436117673585521, 0.000000000000000000, -0.5085311186492154079 ) ) ;
#34928=ORIENTED_EDGE ( 'NONE', *, *, #27835, .T. ) ;
#34929=VERTEX_POINT ( 'NONE', #10812 ) ;
#34931=ORIENTED_EDGE ( 'NONE', *, *, #52009, .T. ) ;
#34932=CARTESIAN_POINT ( 'NONE',  ( -49.44376233341721161, -177.1207230881787780, 0.2635871660690650709 ) ) ;
#34933=CIRCLE ( 'NONE', #48512, 125.0000000000000000 ) ;
#34934=ORIENTED_EDGE ( 'NONE', *, *, #20231, .T. ) ;
#34935=DIRECTION ( 'NONE',  ( 0.1768902751225592818, 0.000000000000000000, 0.9842305779475992722 ) ) ;
#34937=DIRECTION ( 'NONE',  ( -0.1182731709213730997, 0.000000000000000000, 0.9929810960135161402 ) ) ;
#34938=VECTOR ( 'NONE', #44783, 1000.000000000000000 ) ;
#34940=VERTEX_POINT ( 'NONE', #18188 ) ;
#34942=CIRCLE ( 'NONE', #6427, 10.00000000000000178 ) ;
#34944=LINE ( 'NONE', #18164, #28160 ) ;
#34946=EDGE_CURVE ( 'NONE', #20567, #45186, #43122, .T. ) ;
#34948=EDGE_LOOP ( 'NONE', ( #2396, #30468, #25909, #46996 ) ) ;
#34949=LINE ( 'NONE', #27324, #19770 ) ;
#34950=FACE_OUTER_BOUND ( 'NONE', #28235, .T. ) ;
#34951=CIRCLE ( 'NONE', #19024, 125.0000000000000000 ) ;
#34956=DIRECTION ( 'NONE',  ( -0.000000000000000000, 1.000000000000000000, -0.000000000000000000 ) ) ;
#34957=EDGE_CURVE ( 'NONE', #32738, #10210, #2140, .T. ) ;
#34959=ORIENTED_EDGE ( 'NONE', *, *, #45496, .F. ) ;
#34960=EDGE_CURVE ( 'NONE', #2310, #37251, #35233, .T. ) ;
#34961=AXIS2_PLACEMENT_3D ( 'NONE', #48911, #25246, #12887 ) ;
#34962=DIRECTION ( 'NONE',  ( 0.000000000000000000, 0.000000000000000000, -1.000000000000000000 ) ) ;
#34963=VECTOR ( 'NONE', #33491, 1000.000000000000114 ) ;
#34967=DIRECTION ( 'NONE',  ( 0.3758275821142422202, 0.000000000000000000, -0.9266896074318318188 ) ) ;
#34968=FACE_OUTER_BOUND ( 'NONE', #3835, .T. ) ;
#34972=CARTESIAN_POINT ( 'NONE',  ( -167.1668396246903114, -193.5000000000000000, -35.90758392117659525 ) ) ;
#34974=DIRECTION ( 'NONE',  ( 0.000000000000000000, 0.000000000000000000, 1.000000000000000000 ) ) ;
#34975=ORIENTED_EDGE ( 'NONE', *, *, #8083, .T. ) ;
#34982=AXIS2_PLACEMENT_3D ( 'NONE', #46584, #19240, #18976 ) ;
#34983=AXIS2_PLACEMENT_3D ( 'NONE', #51320, #31854, #15572 ) ;
#34985=LINE ( 'NONE', #3194, #16929 ) ;
#34986=AXIS2_PLACEMENT_3D ( 'NONE', #41125, #16965, #4606 ) ;
#34988=ADVANCED_FACE ( 'NONE', ( #22382 ), #38409, .F. ) ;
#34990=CARTESIAN_POINT ( 'NONE',  ( -60.80616967713025645, -183.6283474603465606, -123.3865623328508150 ) ) ;
#34991=FACE_OUTER_BOUND ( 'NONE', #213, .T. ) ;
#34994=ORIENTED_EDGE ( 'NONE', *, *, #51362, .F. ) ;
#34995=CARTESIAN_POINT ( 'NONE',  ( -67.22356632362125595, -177.1207230881787780, -123.5865930638409793 ) ) ;
#34997=CARTESIAN_POINT ( 'NONE',  ( -4.525132525065792777, -193.5000000000000000, 115.9484881370938325 ) ) ;
#34998=EDGE_LOOP ( 'NONE', ( #38440, #16703, #34759, #9881 ) ) ;
#34999=LINE ( 'NONE', #2937, #40866 ) ;
#35000=CARTESIAN_POINT ( 'NONE',  ( -48.47912675150885065, -183.6283474603465606, -0.9999999999999931166 ) ) ;
#35001=FACE_OUTER_BOUND ( 'NONE', #5324, .T. ) ;
#35003=VERTEX_POINT ( 'NONE', #38660 ) ;
#35005=VECTOR ( 'NONE', #24995, 1000.000000000000000 ) ;
#35006=ORIENTED_EDGE ( 'NONE', *, *, #3471, .F. ) ;
#35007=DIRECTION ( 'NONE',  ( 0.000000000000000000, -1.000000000000000000, -0.000000000000000000 ) ) ;
#35008=AXIS2_PLACEMENT_3D ( 'NONE', #15016, #11292, #50495 ) ;
#35010=ORIENTED_EDGE ( 'NONE', *, *, #19774, .F. ) ;
#35011=LINE ( 'NONE', #51068, #35798 ) ;
#35012=CIRCLE ( 'NONE', #14017, 125.0000000000000000 ) ;
#35013=DIRECTION ( 'NONE',  ( 0.000000000000000000, 0.000000000000000000, -1.000000000000000000 ) ) ;
#35014=ORIENTED_EDGE ( 'NONE', *, *, #34889, .F. ) ;
#35017=VERTEX_POINT ( 'NONE', #47081 ) ;
#35018=LINE ( 'NONE', #23458, #36679 ) ;
#35020=AXIS2_PLACEMENT_3D ( 'NONE', #42690, #14066, #42935 ) ;
#35021=PLANE ( 'NONE',  #3798 ) ;
#35022=CIRCLE ( 'NONE', #8161, 125.0000000000000000 ) ;
#35023=DIRECTION ( 'NONE',  ( 0.000000000000000000, 1.000000000000000000, -0.000000000000000000 ) ) ;
#35024=VERTEX_POINT ( 'NONE', #11059 ) ;
#35026=ADVANCED_FACE ( 'NONE', ( #32068 ), #51536, .F. ) ;
#35027=DIRECTION ( 'NONE',  ( 0.000000000000000000, 0.000000000000000000, 1.000000000000000000 ) ) ;
#35029=LINE ( 'NONE', #50810, #47592 ) ;
#35030=EDGE_CURVE ( 'NONE', #13288, #29108, #3690, .T. ) ;
#35032=EDGE_CURVE ( 'NONE', #21876, #20693, #15535, .T. ) ;
#35033=EDGE_LOOP ( 'NONE', ( #49007, #10892, #34866, #37603 ) ) ;
#35035=CIRCLE ( 'NONE', #12358, 125.0000000000000000 ) ;
#35037=DIRECTION ( 'NONE',  ( 0.000000000000000000, 0.000000000000000000, -1.000000000000000000 ) ) ;
#35040=ORIENTED_EDGE ( 'NONE', *, *, #18610, .F. ) ;
#35041=EDGE_LOOP ( 'NONE', ( #27867, #49348, #19457, #37927 ) ) ;
#35042=LINE ( 'NONE', #51102, #16531 ) ;
#35043=CARTESIAN_POINT ( 'NONE',  ( -124.9871112439422092, -193.5000000000000000, -98.85104101073275729 ) ) ;
#35045=AXIS2_PLACEMENT_3D ( 'NONE', #45366, #21704, #50083 ) ;
#35047=ORIENTED_EDGE ( 'NONE', *, *, #19285, .F. ) ;
#35048=DIRECTION ( 'NONE',  ( 0.000000000000000000, 1.000000000000000000, 0.000000000000000000 ) ) ;
#35050=VERTEX_POINT ( 'NONE', #44158 ) ;
#35052=DIRECTION ( 'NONE',  ( -0.000000000000000000, -1.000000000000000000, 0.000000000000000000 ) ) ;
#35053=CIRCLE ( 'NONE', #13225, 125.0000000000000000 ) ;
#35054=CARTESIAN_POINT ( 'NONE',  ( -94.25732089370191602, -193.5000000000000000, 116.3157639405754935 ) ) ;
#35057=ORIENTED_EDGE ( 'NONE', *, *, #19669, .F. ) ;
#35058=EDGE_CURVE ( 'NONE', #30216, #50878, #15821, .T. ) ;
#35059=ORIENTED_EDGE ( 'NONE', *, *, #12911, .T. ) ;
#35060=DIRECTION ( 'NONE',  ( -0.5085311186492273983, 0.000000000000000000, 0.8610436117673514467 ) ) ;
#35061=CARTESIAN_POINT ( 'NONE',  ( -168.0489871616337325, -193.5000000000000000, -32.84887689123904408 ) ) ;
#35064=VECTOR ( 'NONE', #41867, 1000.000000000000000 ) ;
#35068=DIRECTION ( 'NONE',  ( 0.000000000000000000, 1.000000000000000000, 0.000000000000000000 ) ) ;
#35069=CARTESIAN_POINT ( 'NONE',  ( -142.9772358822569629, -183.6283474603465606, 81.82363577055970438 ) ) ;
#35070=AXIS2_PLACEMENT_3D ( 'NONE', #5549, #41520, #10766 ) ;
#35071=ORIENTED_EDGE ( 'NONE', *, *, #23669, .F. ) ;
#35072=ORIENTED_EDGE ( 'NONE', *, *, #47444, .F. ) ;
#35073=DIRECTION ( 'NONE',  ( -0.9374196611341254481, 0.000000000000000000, 0.3482016354343867026 ) ) ;
#35074=DIRECTION ( 'NONE',  ( 0.000000000000000000, 0.000000000000000000, -1.000000000000000000 ) ) ;
#35076=LINE ( 'NONE', #51899, #16172 ) ;
#35077=DIRECTION ( 'NONE',  ( 0.000000000000000000, -1.000000000000000000, -0.000000000000000000 ) ) ;
#35078=ORIENTED_EDGE ( 'NONE', *, *, #23200, .F. ) ;
#35079=DIRECTION ( 'NONE',  ( 0.000000000000000000, -0.000000000000000000, 1.000000000000000000 ) ) ;
#35080=ORIENTED_EDGE ( 'NONE', *, *, #7610, .F. ) ;
#35081=DIRECTION ( 'NONE',  ( 0.000000000000000000, 0.000000000000000000, 1.000000000000000000 ) ) ;
#35082=AXIS2_PLACEMENT_3D ( 'NONE', #22670, #34737, #50790 ) ;
#35083=CIRCLE ( 'NONE', #4899, 125.0000000000000000 ) ;
#35084=DIRECTION ( 'NONE',  ( -0.000000000000000000, 1.000000000000000000, 0.000000000000000000 ) ) ;
#35086=AXIS2_PLACEMENT_3D ( 'NONE', #14058, #25355, #914 ) ;
#35088=DIRECTION ( 'NONE',  ( 0.000000000000000000, -1.000000000000000000, 0.000000000000000000 ) ) ;
#35089=DIRECTION ( 'NONE',  ( 0.000000000000000000, -0.000000000000000000, -1.000000000000000000 ) ) ;
#35090=EDGE_CURVE ( 'NONE', #36830, #29101, #8163, .T. ) ;
#35091=PLANE ( 'NONE',  #11479 ) ;
#35092=DIRECTION ( 'NONE',  ( 0.000000000000000000, -1.000000000000000000, -0.000000000000000000 ) ) ;
#35093=ORIENTED_EDGE ( 'NONE', *, *, #3831, .T. ) ;
#35095=DIRECTION ( 'NONE',  ( -0.6068001458186002006, 0.000000000000000000, 0.7948544414133481562 ) ) ;
#35096=ORIENTED_EDGE ( 'NONE', *, *, #31877, .T. ) ;
#35097=VERTEX_POINT ( 'NONE', #16306 ) ;
#35098=CARTESIAN_POINT ( 'NONE',  ( -85.77912150413021664, -189.7472609257535510, -119.3051146910911768 ) ) ;
#35100=AXIS2_PLACEMENT_3D ( 'NONE', #16534, #20198, #28338 ) ;
#35101=CARTESIAN_POINT ( 'NONE',  ( 43.86477233319988756, -193.5000000000000000, -84.24728067915975771 ) ) ;
#35102=ORIENTED_EDGE ( 'NONE', *, *, #268, .T. ) ;
#35104=DIRECTION ( 'NONE',  ( -0.000000000000000000, 1.000000000000000000, -0.000000000000000000 ) ) ;
#35105=ADVANCED_FACE ( 'NONE', ( #39430 ), #44432, .T. ) ;
#35106=ORIENTED_EDGE ( 'NONE', *, *, #48491, .T. ) ;
#35107=FACE_OUTER_BOUND ( 'NONE', #46352, .T. ) ;
#35109=CARTESIAN_POINT ( 'NONE',  ( 48.69345348225014902, -193.5000000000000000, -78.62880929222872339 ) ) ;
#35110=ORIENTED_EDGE ( 'NONE', *, *, #9405, .F. ) ;
#35111=VERTEX_POINT ( 'NONE', #3433 ) ;
#35112=ORIENTED_EDGE ( 'NONE', *, *, #51093, .F. ) ;
#35116=VECTOR ( 'NONE', #17808, 1000.000000000000000 ) ;
#35118=LINE ( 'NONE', #51176, #42743 ) ;
#35119=PLANE ( 'NONE',  #21163 ) ;
#35120=DIRECTION ( 'NONE',  ( 0.000000000000000000, 0.000000000000000000, -1.000000000000000000 ) ) ;
#35121=VERTEX_POINT ( 'NONE', #266 ) ;
#35124=DIRECTION ( 'NONE',  ( -0.000000000000000000, 1.000000000000000000, -0.000000000000000000 ) ) ;
#35125=ORIENTED_EDGE ( 'NONE', *, *, #13149, .T. ) ;
#35126=DIRECTION ( 'NONE',  ( 0.000000000000000000, 1.000000000000000000, 0.000000000000000000 ) ) ;
#35128=VECTOR ( 'NONE', #20433, 1000.000000000000000 ) ;
#35130=CARTESIAN_POINT ( 'NONE',  ( -48.47912675150885065, -189.7472609257535510, 6.938893903907228378E-15 ) ) ;
#35131=FACE_OUTER_BOUND ( 'NONE', #7578, .T. ) ;
#35132=CARTESIAN_POINT ( 'NONE',  ( -70.42295845586433245, -193.5000000000000000, -123.0587999703024877 ) ) ;
#35133=DIRECTION ( 'NONE',  ( -0.000000000000000000, 1.000000000000000000, -0.000000000000000000 ) ) ;
#35134=ORIENTED_EDGE ( 'NONE', *, *, #32859, .T. ) ;
#35135=CARTESIAN_POINT ( 'NONE',  ( -30.31202594373734627, -177.1207230881787780, -123.6727797384705809 ) ) ;
#35136=ORIENTED_EDGE ( 'NONE', *, *, #38531, .F. ) ;
#35138=EDGE_CURVE ( 'NONE', #10684, #34133, #51806, .T. ) ;
#35141=DIRECTION ( 'NONE',  ( -0.000000000000000000, 1.000000000000000000, -0.000000000000000000 ) ) ;
#35142=ORIENTED_EDGE ( 'NONE', *, *, #33964, .T. ) ;
#35143=DIRECTION ( 'NONE',  ( 0.000000000000000000, 0.000000000000000000, -1.000000000000000000 ) ) ;
#35144=CARTESIAN_POINT ( 'NONE',  ( -101.0675409952199999, -183.6283474603465606, 113.3995532942341100 ) ) ;
#35145=DIRECTION ( 'NONE',  ( -0.000000000000000000, 1.000000000000000000, -0.000000000000000000 ) ) ;
#35146=CARTESIAN_POINT ( 'NONE',  ( -168.9345475356665531, -183.6283474603465606, 29.43839964798724296 ) ) ;
#35147=ADVANCED_FACE ( 'NONE', ( #47604 ), #4222, .T. ) ;
#35148=ORIENTED_EDGE ( 'NONE', *, *, #29455, .F. ) ;
#35149=LINE ( 'NONE', #51984, #23798 ) ;
#35151=EDGE_CURVE ( 'NONE', #15345, #25387, #27615, .T. ) ;
#35152=LINE ( 'NONE', #18616, #28224 ) ;
#35154=AXIS2_PLACEMENT_3D ( 'NONE', #7921, #39708, #51839 ) ;
#35155=EDGE_CURVE ( 'NONE', #37521, #27989, #43644, .T. ) ;
#35157=AXIS2_PLACEMENT_3D ( 'NONE', #31228, #43322, #39371 ) ;
#35158=PLANE ( 'NONE',  #26950 ) ;
#35161=ORIENTED_EDGE ( 'NONE', *, *, #12722, .T. ) ;
#35163=FACE_OUTER_BOUND ( 'NONE', #36478, .T. ) ;
#35164=FACE_BOUND ( 'NONE', #31531, .T. ) ;
#35165=LINE ( 'NONE', #51219, #25432 ) ;
#35167=ADVANCED_FACE ( 'NONE', ( #27860 ), #4484, .T. ) ;
#35169=ORIENTED_EDGE ( 'NONE', *, *, #5440, .F. ) ;
#35170=CIRCLE ( 'NONE', #3297, 125.0000000000000000 ) ;
#35176=CARTESIAN_POINT ( 'NONE',  ( -123.6678354051270077, -189.7472609257535510, 99.85818990449067201 ) ) ;
#35177=DIRECTION ( 'NONE',  ( 0.5586467658036476935, 0.000000000000000000, 0.8294056854502049880 ) ) ;
#35178=ORIENTED_EDGE ( 'NONE', *, *, #23167, .T. ) ;
#35179=DIRECTION ( 'NONE',  ( 0.2920567706369694982, 0.000000000000000000, 0.9564009842765243130 ) ) ;
#35180=CARTESIAN_POINT ( 'NONE',  ( -48.47912675150885065, -189.7472609257535510, 6.938893903907228378E-15 ) ) ;
#35182=VECTOR ( 'NONE', #16496, 1000.000000000000000 ) ;
#35183=LINE ( 'NONE', #30985, #15603 ) ;
#35187=VERTEX_POINT ( 'NONE', #31291 ) ;
#35191=ORIENTED_EDGE ( 'NONE', *, *, #40145, .T. ) ;
#35192=DIRECTION ( 'NONE',  ( 0.5829794791144762289, 0.000000000000000000, -0.8124868780056783146 ) ) ;
#35193=LINE ( 'NONE', #15494, #19113 ) ;
#35194=EDGE_LOOP ( 'NONE', ( #50724, #39895, #18513, #32831 ) ) ;
#35195=CARTESIAN_POINT ( 'NONE',  ( -163.6979789053106629, -175.3837268820161057, -45.83253885719557985 ) ) ;
#35197=CARTESIAN_POINT ( 'NONE',  ( -49.35486169370449971, -189.7472609257535510, 0.4827922027307437469 ) ) ;
#35199=ORIENTED_EDGE ( 'NONE', *, *, #7832, .T. ) ;
#35201=LINE ( 'NONE', #3152, #29173 ) ;
#35206=EDGE_CURVE ( 'NONE', #24408, #49251, #17518, .T. ) ;
#35207=LINE ( 'NONE', #19436, #48110 ) ;
#35208=CARTESIAN_POINT ( 'NONE',  ( 54.46899307705341187, -177.1207230881787780, -70.89911581792812001 ) ) ;
#35209=ADVANCED_FACE ( 'NONE', ( #1583 ), #17625, .F. ) ;
#35210=VECTOR ( 'NONE', #36673, 1000.000000000000114 ) ;
#35211=CARTESIAN_POINT ( 'NONE',  ( -48.47912675150885065, -177.1207230881787780, 6.938893903907228378E-15 ) ) ;
#35212=ORIENTED_EDGE ( 'NONE', *, *, #50939, .T. ) ;
#35213=ADVANCED_FACE ( 'NONE', ( #12614 ), #37831, .F. ) ;
#35215=LINE ( 'NONE', #36434, #7634 ) ;
#35216=EDGE_CURVE ( 'NONE', #35836, #3435, #45227, .T. ) ;
#35217=CARTESIAN_POINT ( 'NONE',  ( -121.5885020763900997, -177.1207230881787780, -101.3904297239420913 ) ) ;
#35218=DIRECTION ( 'NONE',  ( 0.6965510290629932655, 0.000000000000000000, 0.7175072570443347120 ) ) ;
#35220=ORIENTED_EDGE ( 'NONE', *, *, #14413, .F. ) ;
#35223=DIRECTION ( 'NONE',  ( -0.5085311186492273983, 0.000000000000000000, 0.8610436117673514467 ) ) ;
#35224=VECTOR ( 'NONE', #13269, 1000.000000000000000 ) ;
#35227=CARTESIAN_POINT ( 'NONE',  ( 20.66186849114819069, -189.7472609257535510, -104.1370384486465070 ) ) ;
#35228=ORIENTED_EDGE ( 'NONE', *, *, #21925, .T. ) ;
#35232=EDGE_LOOP ( 'NONE', ( #21923, #39929, #637, #35598 ) ) ;
#35233=LINE ( 'NONE', #38137, #30925 ) ;
#35235=EDGE_LOOP ( 'NONE', ( #6774, #19518, #29855, #19224 ) ) ;
#35236=VECTOR ( 'NONE', #26393, 1000.000000000000227 ) ;
#35238=DIRECTION ( 'NONE',  ( 0.000000000000000000, 1.000000000000000000, 0.000000000000000000 ) ) ;
#35239=DIRECTION ( 'NONE',  ( 0.000000000000000000, 1.000000000000000000, 0.000000000000000000 ) ) ;
#35240=DIRECTION ( 'NONE',  ( 0.000000000000000000, 0.000000000000000000, 1.000000000000000000 ) ) ;
#35242=ORIENTED_EDGE ( 'NONE', *, *, #16190, .T. ) ;
#35243=DIRECTION ( 'NONE',  ( 0.000000000000000000, -1.000000000000000000, 0.000000000000000000 ) ) ;
#35244=ORIENTED_EDGE ( 'NONE', *, *, #33678, .T. ) ;
#35245=DIRECTION ( 'NONE',  ( -0.000000000000000000, 1.000000000000000000, -0.000000000000000000 ) ) ;
#35246=ORIENTED_EDGE ( 'NONE', *, *, #23345, .T. ) ;
#35247=EDGE_CURVE ( 'NONE', #47918, #24476, #16582, .T. ) ;
#35248=EDGE_CURVE ( 'NONE', #21906, #25767, #51099, .T. ) ;
#35250=LINE ( 'NONE', #15291, #32473 ) ;
#35251=CARTESIAN_POINT ( 'NONE',  ( -85.14888725715769624, -175.3837268820161057, 119.5003291395398577 ) ) ;
#35252=DIRECTION ( 'NONE',  ( 0.9266896074318291543, 0.000000000000000000, 0.3758275821142488260 ) ) ;
#35253=DIRECTION ( 'NONE',  ( 0.000000000000000000, 1.000000000000000000, 0.000000000000000000 ) ) ;
#35254=VERTEX_POINT ( 'NONE', #21558 ) ;
#35255=EDGE_CURVE ( 'NONE', #15087, #49860, #25232, .T. ) ;
#35258=LINE ( 'NONE', #22925, #18103 ) ;
#35259=PLANE ( 'NONE',  #19146 ) ;
#35260=CIRCLE ( 'NONE', #6769, 125.0000000000000000 ) ;
#35261=VERTEX_POINT ( 'NONE', #37312 ) ;
#35262=EDGE_CURVE ( 'NONE', #17251, #21890, #23355, .T. ) ;
#35263=DIRECTION ( 'NONE',  ( 0.2920567706369833760, 0.000000000000000000, -0.9564009842765202052 ) ) ;
#35264=DIRECTION ( 'NONE',  ( -0.000000000000000000, 1.000000000000000000, -0.000000000000000000 ) ) ;
#35268=DIRECTION ( 'NONE',  ( -0.000000000000000000, 1.000000000000000000, -0.000000000000000000 ) ) ;
#35269=EDGE_CURVE ( 'NONE', #51645, #26457, #9139, .T. ) ;
#35272=ORIENTED_EDGE ( 'NONE', *, *, #202, .T. ) ;
#35274=LINE ( 'NONE', #46871, #17281 ) ;
#35275=DIRECTION ( 'NONE',  ( 0.05924062789372142729, 0.000000000000000000, -0.9982437317643209074 ) ) ;
#35276=ORIENTED_EDGE ( 'NONE', *, *, #38428, .F. ) ;
#35277=ADVANCED_FACE ( 'NONE', ( #17103 ), #4745, .F. ) ;
#35278=FACE_OUTER_BOUND ( 'NONE', #43018, .T. ) ;
#35279=DIRECTION ( 'NONE',  ( -0.8455960035018199594, 0.000000000000000000, -0.5338233779648003940 ) ) ;
#35280=CARTESIAN_POINT ( 'NONE',  ( 36.10886851198521441, -177.1207230881787780, 92.03190238880813467 ) ) ;
#35281=ADVANCED_FACE ( 'NONE', ( #33109 ), #17367, .F. ) ;
#35283=CIRCLE ( 'NONE', #43690, 125.0000000000000000 ) ;
#35286=DIRECTION ( 'NONE',  ( 0.000000000000000000, 0.000000000000000000, -1.000000000000000000 ) ) ;
#35289=EDGE_LOOP ( 'NONE', ( #22403, #23783, #51041, #43628 ) ) ;
#35291=EDGE_CURVE ( 'NONE', #46556, #26846, #5802, .T. ) ;
#35292=DIRECTION ( 'NONE',  ( -0.8896570909947530970, 0.000000000000000000, 0.4566292373937018700 ) ) ;
#35293=EDGE_LOOP ( 'NONE', ( #38522, #14321, #27680, #32724 ) ) ;
#35294=VERTEX_POINT ( 'NONE', #48645 ) ;
#35295=AXIS2_PLACEMENT_3D ( 'NONE', #33875, #9453, #42020 ) ;
#35296=FACE_OUTER_BOUND ( 'NONE', #43266, .T. ) ;
#35297=ORIENTED_EDGE ( 'NONE', *, *, #44663, .F. ) ;
#35298=DIRECTION ( 'NONE',  ( -0.000000000000000000, 1.000000000000000000, -0.000000000000000000 ) ) ;
#35299=CARTESIAN_POINT ( 'NONE',  ( -49.35486169370449971, -175.3837268820161057, 0.4827922027307437469 ) ) ;
#35300=CARTESIAN_POINT ( 'NONE',  ( -133.0671220150036334, -177.1207230881787780, -92.03190238880748097 ) ) ;
#35303=ORIENTED_EDGE ( 'NONE', *, *, #385, .F. ) ;
#35304=ORIENTED_EDGE ( 'NONE', *, *, #38493, .F. ) ;
#35305=EDGE_CURVE ( 'NONE', #22071, #22595, #38604, .T. ) ;
#35306=CARTESIAN_POINT ( 'NONE',  ( -132.6364218684650211, -183.6283474603465606, 92.42591454022807795 ) ) ;
#35308=CYLINDRICAL_SURFACE ( 'NONE', #16545, 125.0000000000000000 ) ;
#35311=EDGE_LOOP ( 'NONE', ( #44267, #29532, #51072, #42287 ) ) ;
#35312=AXIS2_PLACEMENT_3D ( 'NONE', #23143, #11567, #19441 ) ;
#35313=EDGE_CURVE ( 'NONE', #8712, #194, #50202, .T. ) ;
#35315=EDGE_CURVE ( 'NONE', #5249, #15815, #2606, .T. ) ;
#35317=CYLINDRICAL_SURFACE ( 'NONE', #507, 125.0000000000000000 ) ;
#35320=EDGE_CURVE ( 'NONE', #51319, #18264, #22315, .T. ) ;
#35321=ORIENTED_EDGE ( 'NONE', *, *, #13150, .F. ) ;
#35322=ORIENTED_EDGE ( 'NONE', *, *, #14951, .T. ) ;
#35323=DIRECTION ( 'NONE',  ( -0.000000000000000000, 1.000000000000000000, -0.000000000000000000 ) ) ;
#35324=DIRECTION ( 'NONE',  ( 0.000000000000000000, 1.000000000000000000, 0.000000000000000000 ) ) ;
#35325=ORIENTED_EDGE ( 'NONE', *, *, #31332, .T. ) ;
#35330=DIRECTION ( 'NONE',  ( 0.08879589532292483933, 0.000000000000000000, 0.9960498426152178952 ) ) ;
#35331=ORIENTED_EDGE ( 'NONE', *, *, #16805, .F. ) ;
#35333=CIRCLE ( 'NONE', #26929, 125.0000000000000000 ) ;
#35334=ADVANCED_FACE ( 'NONE', ( #18642 ), #30975, .T. ) ;
#35340=DIRECTION ( 'NONE',  ( 0.000000000000000000, 1.000000000000000000, 0.000000000000000000 ) ) ;
#35341=DIRECTION ( 'NONE',  ( -0.000000000000000000, 1.000000000000000000, 0.000000000000000000 ) ) ;
#35342=ADVANCED_FACE ( 'NONE', ( #29946 ), #47020, .T. ) ;
#35343=FACE_OUTER_BOUND ( 'NONE', #21557, .T. ) ;
#35344=EDGE_LOOP ( 'NONE', ( #50618, #21640, #936, #46336 ) ) ;
#35348=VERTEX_POINT ( 'NONE', #30710 ) ;
#35353=DIRECTION ( 'NONE',  ( -0.000000000000000000, 1.000000000000000000, -0.000000000000000000 ) ) ;
#35355=DIRECTION ( 'NONE',  ( -0.000000000000000000, 1.000000000000000000, -0.000000000000000000 ) ) ;
#35356=PLANE ( 'NONE',  #44648 ) ;
#35358=CYLINDRICAL_SURFACE ( 'NONE', #40072, 125.0000000000000000 ) ;
#35359=LINE ( 'NONE', #14627, #21920 ) ;
#35360=LINE ( 'NONE', #15672, #45067 ) ;
#35361=VERTEX_POINT ( 'NONE', #50453 ) ;
#35364=ORIENTED_EDGE ( 'NONE', *, *, #10893, .F. ) ;
#35365=LINE ( 'NONE', #38273, #40151 ) ;
#35367=AXIS2_PLACEMENT_3D ( 'NONE', #23731, #27927, #47670 ) ;
#35369=DIRECTION ( 'NONE',  ( 0.5338233779647948429, 0.000000000000000000, -0.8455960035018234011 ) ) ;
#35371=ORIENTED_EDGE ( 'NONE', *, *, #43007, .F. ) ;
#35372=ADVANCED_FACE ( 'NONE', ( #6043 ), #7070, .T. ) ;
#35373=ADVANCED_FACE ( 'NONE', ( #46004 ), #42806, .T. ) ;
#35374=LINE ( 'NONE', #47475, #1441 ) ;
#35377=ORIENTED_EDGE ( 'NONE', *, *, #35269, .F. ) ;
#35378=ORIENTED_EDGE ( 'NONE', *, *, #10777, .F. ) ;
#35380=CARTESIAN_POINT ( 'NONE',  ( -53.47502265695602119, -193.5000000000000000, -124.9001241957025883 ) ) ;
#35382=FACE_OUTER_BOUND ( 'NONE', #48912, .T. ) ;
#35383=DIRECTION ( 'NONE',  ( 0.000000000000000000, 1.000000000000000000, 0.000000000000000000 ) ) ;
#35384=ORIENTED_EDGE ( 'NONE', *, *, #48329, .F. ) ;
#35385=DIRECTION ( 'NONE',  ( 0.2920567706369628924, 0.000000000000000000, 0.9564009842765264224 ) ) ;
#35387=ORIENTED_EDGE ( 'NONE', *, *, #30675, .T. ) ;
#35391=CYLINDRICAL_SURFACE ( 'NONE', #4622, 125.0000000000000000 ) ;
#35393=CARTESIAN_POINT ( 'NONE',  ( 67.04262753014327814, -175.3837268820161057, -47.74645837849745078 ) ) ;
#35394=CARTESIAN_POINT ( 'NONE',  ( -169.0136227435421006, -189.7472609257535510, -33.11246405730813080 ) ) ;
#35395=DIRECTION ( 'NONE',  ( 0.000000000000000000, -1.000000000000000000, 0.000000000000000000 ) ) ;
#35396=DIRECTION ( 'NONE',  ( 0.000000000000000000, 1.000000000000000000, 0.000000000000000000 ) ) ;
#35397=CARTESIAN_POINT ( 'NONE',  ( -154.0877180371535928, -175.3837268820161057, -66.87170886601928999 ) ) ;
#35399=LINE ( 'NONE', #48555, #20451 ) ;
#35400=CARTESIAN_POINT ( 'NONE',  ( -168.1141659785444915, -177.1207230881787780, -36.22785377503944204 ) ) ;
#35401=VECTOR ( 'NONE', #35803, 1000.000000000000000 ) ;
#35402=EDGE_CURVE ( 'NONE', #2850, #34268, #6813, .T. ) ;
#35405=CIRCLE ( 'NONE', #15271, 125.0000000000000000 ) ;
#35406=CIRCLE ( 'NONE', #16101, 125.0000000000000000 ) ;
#35409=EDGE_LOOP ( 'NONE', ( #20117, #13117, #46844, #30999 ) ) ;
#35412=ORIENTED_EDGE ( 'NONE', *, *, #36933, .T. ) ;
#35413=CARTESIAN_POINT ( 'NONE',  ( -169.6464974000608379, -189.7472609257535510, 26.35287080855539088 ) ) ;
#35414=FACE_BOUND ( 'NONE', #14648, .T. ) ;
#35417=VECTOR ( 'NONE', #45248, 1000.000000000000000 ) ;
#35418=DIRECTION ( 'NONE',  ( -0.000000000000000000, 1.000000000000000000, -0.000000000000000000 ) ) ;
#35421=ADVANCED_FACE ( 'NONE', ( #33881 ), #10483, .F. ) ;
#35422=ORIENTED_EDGE ( 'NONE', *, *, #36528, .T. ) ;
#35424=VERTEX_POINT ( 'NONE', #34908 ) ;
#35425=DIRECTION ( 'NONE',  ( 0.000000000000000000, 1.000000000000000000, 0.000000000000000000 ) ) ;
#35426=EDGE_CURVE ( 'NONE', #21993, #12738, #14970, .T. ) ;
#35428=VECTOR ( 'NONE', #10645, 1000.000000000000000 ) ;
#35430=LINE ( 'NONE', #31766, #18893 ) ;
#35431=ORIENTED_EDGE ( 'NONE', *, *, #32595, .T. ) ;
#35434=EDGE_LOOP ( 'NONE', ( #20528, #23537, #19878, #44257 ) ) ;
#35435=AXIS2_PLACEMENT_3D ( 'NONE', #16755, #4139, #36707 ) ;
#35437=LINE ( 'NONE', #43338, #3820 ) ;
#35439=DIRECTION ( 'NONE',  ( -0.9646355819083594074, 0.000000000000000000, 0.2635871660690647933 ) ) ;
#35440=DIRECTION ( 'NONE',  ( -0.000000000000000000, 1.000000000000000000, -0.000000000000000000 ) ) ;
#35441=ORIENTED_EDGE ( 'NONE', *, *, #29149, .F. ) ;
#35442=DIRECTION ( 'NONE',  ( -0.2920567706369764371, 0.000000000000000000, 0.9564009842765223146 ) ) ;
#35443=CARTESIAN_POINT ( 'NONE',  ( 41.40822382563629134, -177.1207230881787780, 85.41934182508082074 ) ) ;
#35444=ORIENTED_EDGE ( 'NONE', *, *, #3178, .T. ) ;
#35446=ORIENTED_EDGE ( 'NONE', *, *, #29337, .F. ) ;
#35449=EDGE_CURVE ( 'NONE', #3470, #47114, #46252, .T. ) ;
#35450=LINE ( 'NONE', #11275, #30544 ) ;
#35451=CARTESIAN_POINT ( 'NONE',  ( 60.51025563957495734, -189.7472609257535510, 59.13814366165117065 ) ) ;
#35452=CARTESIAN_POINT ( 'NONE',  ( -168.1141659785444915, -177.1207230881787780, -36.22785377503943494 ) ) ;
#35453=AXIS2_PLACEMENT_3D ( 'NONE', #9681, #36765, #32813 ) ;
#35457=DIRECTION ( 'NONE',  ( 0.000000000000000000, -1.000000000000000000, -0.000000000000000000 ) ) ;
#35458=PLANE ( 'NONE',  #12227 ) ;
#35459=AXIS2_PLACEMENT_3D ( 'NONE', #41554, #21609, #37630 ) ;
#35460=LINE ( 'NONE', #22874, #43057 ) ;
#35461=ORIENTED_EDGE ( 'NONE', *, *, #8818, .F. ) ;
#35462=PLANE ( 'NONE',  #29038 ) ;
#35463=CARTESIAN_POINT ( 'NONE',  ( -31.30262293407085039, -183.6283474603465606, -123.8142468240611294 ) ) ;
#35464=DIRECTION ( 'NONE',  ( 0.000000000000000000, -0.000000000000000000, -1.000000000000000000 ) ) ;
#35468=ORIENTED_EDGE ( 'NONE', *, *, #40065, .T. ) ;
#35469=CIRCLE ( 'NONE', #15386, 125.0000000000000000 ) ;
#35470=CIRCLE ( 'NONE', #17050, 125.0000000000000000 ) ;
#35471=DIRECTION ( 'NONE',  ( -0.000000000000000000, -1.000000000000000000, 0.000000000000000000 ) ) ;
#35472=AXIS2_PLACEMENT_3D ( 'NONE', #10599, #33991, #2709 ) ;
#35473=DIRECTION ( 'NONE',  ( -0.000000000000000000, 1.000000000000000000, -0.000000000000000000 ) ) ;
#35475=LINE ( 'NONE', #15527, #30412 ) ;
#35478=EDGE_CURVE ( 'NONE', #20971, #38288, #20040, .T. ) ;
#35481=ORIENTED_EDGE ( 'NONE', *, *, #31432, .T. ) ;
#35482=ORIENTED_EDGE ( 'NONE', *, *, #649, .F. ) ;
#35483=EDGE_LOOP ( 'NONE', ( #24886, #18896, #12303, #30303 ) ) ;
#35484=DIRECTION ( 'NONE',  ( 0.000000000000000000, -0.000000000000000000, -1.000000000000000000 ) ) ;
#35485=AXIS2_PLACEMENT_3D ( 'NONE', #35856, #7742, #22998 ) ;
#35486=EDGE_CURVE ( 'NONE', #25387, #12506, #31793, .T. ) ;
#35488=ORIENTED_EDGE ( 'NONE', *, *, #50692, .F. ) ;
#35490=VECTOR ( 'NONE', #7700, 1000.000000000000000 ) ;
#35491=DIRECTION ( 'NONE',  ( 0.000000000000000000, 0.000000000000000000, 1.000000000000000000 ) ) ;
#35493=FACE_OUTER_BOUND ( 'NONE', #3522, .T. ) ;
#35496=ADVANCED_FACE ( 'NONE', ( #31487 ), #39615, .T. ) ;
#35497=ADVANCED_FACE ( 'NONE', ( #47539 ), #8362, .T. ) ;
#35499=EDGE_LOOP ( 'NONE', ( #47246, #19653 ) ) ;
#35500=DIRECTION ( 'NONE',  ( -0.6528221181905119463, 0.000000000000000000, -0.7575112421616284619 ) ) ;
#35501=VERTEX_POINT ( 'NONE', #19160 ) ;
#35504=CARTESIAN_POINT ( 'NONE',  ( -21.64528618042744412, -177.1207230881787780, 121.0625654437174887 ) ) ;
#35505=CYLINDRICAL_SURFACE ( 'NONE', #25680, 124.9999999999999858 ) ;
#35507=VECTOR ( 'NONE', #34071, 1000.000000000000000 ) ;
#35508=ORIENTED_EDGE ( 'NONE', *, *, #14171, .T. ) ;
#35509=CARTESIAN_POINT ( 'NONE',  ( -171.4559849729830603, -193.5000000000000000, 22.39848972532369942 ) ) ;
#35510=VECTOR ( 'NONE', #23966, 1000.000000000000227 ) ;
#35511=FACE_OUTER_BOUND ( 'NONE', #28049, .T. ) ;
#35512=ORIENTED_EDGE ( 'NONE', *, *, #16380, .F. ) ;
#35513=CARTESIAN_POINT ( 'NONE',  ( -47.74129347246713451, -183.6283474603465606, 0.6749830015182212151 ) ) ;
#35514=PLANE ( 'NONE',  #28166 ) ;
#35515=ORIENTED_EDGE ( 'NONE', *, *, #38659, .F. ) ;
#35516=DIRECTION ( 'NONE',  ( 0.000000000000000000, 0.000000000000000000, -1.000000000000000000 ) ) ;
#35517=VECTOR ( 'NONE', #14616, 1000.000000000000341 ) ;
#35519=EDGE_LOOP ( 'NONE', ( #11962, #24444, #29551, #33628 ) ) ;
#35523=DIRECTION ( 'NONE',  ( 0.000000000000000000, 0.000000000000000000, 1.000000000000000000 ) ) ;
#35527=CARTESIAN_POINT ( 'NONE',  ( 54.46899307705341187, -183.6283474603465606, -70.89911581792813422 ) ) ;
#35529=CARTESIAN_POINT ( 'NONE',  ( 75.60865171534658202, -177.1207230881787780, -15.07392567185468124 ) ) ;
#35530=DIRECTION ( 'NONE',  ( 0.000000000000000000, 0.000000000000000000, 1.000000000000000000 ) ) ;
#35531=CARTESIAN_POINT ( 'NONE',  ( -48.30901192927175458, -175.3837268820161057, -123.9998842437354227 ) ) ;
#35532=DIRECTION ( 'NONE',  ( -0.000000000000000000, 1.000000000000000000, -0.000000000000000000 ) ) ;
#35533=ORIENTED_EDGE ( 'NONE', *, *, #1245, .F. ) ;
#35534=ADVANCED_FACE ( 'NONE', ( #28050 ), #36201, .T. ) ;
#35536=EDGE_CURVE ( 'NONE', #47044, #41906, #7582, .T. ) ;
#35539=AXIS2_PLACEMENT_3D ( 'NONE', #33257, #8814, #49036 ) ;
#35540=EDGE_CURVE ( 'NONE', #39811, #5648, #4113, .T. ) ;
#35542=ORIENTED_EDGE ( 'NONE', *, *, #22003, .F. ) ;
#35545=DIRECTION ( 'NONE',  ( -0.9473263538541923934, 0.000000000000000000, 0.3202698538628350744 ) ) ;
#35546=ORIENTED_EDGE ( 'NONE', *, *, #51006, .T. ) ;
#35547=DIRECTION ( 'NONE',  ( 0.000000000000000000, 0.000000000000000000, 1.000000000000000000 ) ) ;
#35549=ADVANCED_FACE ( 'NONE', ( #47797 ), #43585, .F. ) ;
#35551=CARTESIAN_POINT ( 'NONE',  ( -48.13092511607445800, -189.7472609257535510, 0.9374196611341301111 ) ) ;
#35552=DIRECTION ( 'NONE',  ( -0.000000000000000000, 1.000000000000000000, -0.000000000000000000 ) ) ;
#35553=EDGE_LOOP ( 'NONE', ( #28439, #18121, #29342, #29652 ) ) ;
#35554=VERTEX_POINT ( 'NONE', #32001 ) ;
#35555=EDGE_CURVE ( 'NONE', #32165, #1159, #33488, .T. ) ;
#35556=EDGE_LOOP ( 'NONE', ( #42637, #10941, #2623, #41941 ) ) ;
#35557=CARTESIAN_POINT ( 'NONE',  ( 30.05499637021958392, -193.5000000000000000, -97.24912084693205827 ) ) ;
#35558=CARTESIAN_POINT ( 'NONE',  ( 40.30419662299490113, -193.5000000000000000, -87.99159897727903967 ) ) ;
#35559=DIRECTION ( 'NONE',  ( 0.000000000000000000, 0.000000000000000000, 1.000000000000000000 ) ) ;
#35560=EDGE_CURVE ( 'NONE', #14995, #3996, #37681, .T. ) ;
#35562=CARTESIAN_POINT ( 'NONE',  ( 9.518239912201957864, -213.5000000000000000, -110.7307791902283043 ) ) ;
#35565=CARTESIAN_POINT ( 'NONE',  ( 76.48781641346532467, -189.7472609257535510, 2.874563619424060246 ) ) ;
#35566=ADVANCED_FACE ( 'NONE', ( #32257 ), #12290, .F. ) ;
#35567=CARTESIAN_POINT ( 'NONE',  ( -21.46839590530488096, -183.6283474603465606, 122.0467960216650880 ) ) ;
#35568=DIRECTION ( 'NONE',  ( 0.000000000000000000, 0.000000000000000000, 1.000000000000000000 ) ) ;
#35570=ORIENTED_EDGE ( 'NONE', *, *, #24401, .F. ) ;
#35574=DIRECTION ( 'NONE',  ( -0.9785564922995032555, 0.000000000000000000, -0.2059786187411021818 ) ) ;
#35575=VERTEX_POINT ( 'NONE', #37509 ) ;
#35577=DIRECTION ( 'NONE',  ( -0.8455960035018311727, 0.000000000000000000, 0.5338233779647826305 ) ) ;
#35579=ORIENTED_EDGE ( 'NONE', *, *, #3170, .F. ) ;
#35581=AXIS2_PLACEMENT_3D ( 'NONE', #34719, #32259, #35690 ) ;
#35582=EDGE_CURVE ( 'NONE', #22595, #16314, #44617, .T. ) ;
#35585=LINE ( 'NONE', #11929, #16118 ) ;
#35586=ORIENTED_EDGE ( 'NONE', *, *, #32069, .T. ) ;
#35587=LINE ( 'NONE', #31390, #32384 ) ;
#35589=CARTESIAN_POINT ( 'NONE',  ( -48.47912675150885065, -177.1207230881787780, 6.938893903907228378E-15 ) ) ;
#35590=LINE ( 'NONE', #46939, #39164 ) ;
#35591=ORIENTED_EDGE ( 'NONE', *, *, #44040, .T. ) ;
#35593=EDGE_LOOP ( 'NONE', ( #42809, #39049, #23041, #49561 ) ) ;
#35594=EDGE_CURVE ( 'NONE', #37599, #21393, #36992, .T. ) ;
#35595=EDGE_LOOP ( 'NONE', ( #25836, #10101, #19729, #21829 ) ) ;
#35597=DIRECTION ( 'NONE',  ( 0.000000000000000000, 0.000000000000000000, 1.000000000000000000 ) ) ;
#35598=ORIENTED_EDGE ( 'NONE', *, *, #27543, .T. ) ;
#35599=VECTOR ( 'NONE', #42102, 1000.000000000000000 ) ;
#35600=AXIS2_PLACEMENT_3D ( 'NONE', #13624, #17066, #20734 ) ;
#35602=EDGE_CURVE ( 'NONE', #47240, #1324, #12558, .T. ) ;
#35603=EDGE_LOOP ( 'NONE', ( #34483, #1385, #38952, #51601 ) ) ;
#35604=ADVANCED_FACE ( 'NONE', ( #13071 ), #40929, .T. ) ;
#35606=EDGE_CURVE ( 'NONE', #653, #41184, #16783, .T. ) ;
#35607=CIRCLE ( 'NONE', #12948, 125.0000000000000000 ) ;
#35608=EDGE_CURVE ( 'NONE', #19641, #35121, #21737, .T. ) ;
#35610=EDGE_LOOP ( 'NONE', ( #3783, #40601, #36973, #49205 ) ) ;
#35612=EDGE_CURVE ( 'NONE', #3976, #24651, #4676, .T. ) ;
#35613=PLANE ( 'NONE',  #40459 ) ;
#35614=ORIENTED_EDGE ( 'NONE', *, *, #3441, .F. ) ;
#35616=DIRECTION ( 'NONE',  ( -0.2348860457809707758, 0.000000000000000000, -0.9720229140804138579 ) ) ;
#35619=VECTOR ( 'NONE', #6184, 1000.000000000000227 ) ;
#35620=DIRECTION ( 'NONE',  ( -0.000000000000000000, 1.000000000000000000, 0.000000000000000000 ) ) ;
#35622=ORIENTED_EDGE ( 'NONE', *, *, #22257, .F. ) ;
#35623=ADVANCED_FACE ( 'NONE', ( #5208 ), #32530, .T. ) ;
#35625=CARTESIAN_POINT ( 'NONE',  ( -133.0671220150036334, -193.5000000000000000, -92.03190238880748097 ) ) ;
#35626=CARTESIAN_POINT ( 'NONE',  ( 13.86276369408137477, -175.3837268820161057, -107.1890582354654526 ) ) ;
#35627=EDGE_CURVE ( 'NONE', #46556, #975, #36739, .T. ) ;
#35631=DIRECTION ( 'NONE',  ( -0.000000000000000000, 1.000000000000000000, -0.000000000000000000 ) ) ;
#35632=ORIENTED_EDGE ( 'NONE', *, *, #14268, .T. ) ;
#35633=EDGE_CURVE ( 'NONE', #9665, #8060, #31822, .T. ) ;
#35634=EDGE_CURVE ( 'NONE', #25060, #36281, #29359, .T. ) ;
#35635=DIRECTION ( 'NONE',  ( 0.000000000000000000, 0.000000000000000000, 1.000000000000000000 ) ) ;
#35637=DIRECTION ( 'NONE',  ( 0.5829794791144762289, 0.000000000000000000, -0.8124868780056783146 ) ) ;
#35638=EDGE_LOOP ( 'NONE', ( #30566, #22955, #40258, #18803 ) ) ;
#35639=ORIENTED_EDGE ( 'NONE', *, *, #4076, .F. ) ;
#35640=FACE_OUTER_BOUND ( 'NONE', #33181, .T. ) ;
#35642=CIRCLE ( 'NONE', #12981, 125.0000000000000000 ) ;
#35644=PLANE ( 'NONE',  #5343 ) ;
#35645=CARTESIAN_POINT ( 'NONE',  ( 65.52619748798558419, -183.6283474603465606, 48.77484799213969069 ) ) ;
#35646=ORIENTED_EDGE ( 'NONE', *, *, #23696, .F. ) ;
#35647=CARTESIAN_POINT ( 'NONE',  ( 55.91309001144629320, -183.6283474603465606, 68.75510947788671956 ) ) ;
#35649=AXIS2_PLACEMENT_3D ( 'NONE', #48416, #3731, #16350 ) ;
#35651=ORIENTED_EDGE ( 'NONE', *, *, #31788, .T. ) ;
#35654=CARTESIAN_POINT ( 'NONE',  ( -38.66762320617017679, -193.5000000000000000, -124.6143426664033740 ) ) ;
#35656=CIRCLE ( 'NONE', #48274, 125.0000000000000000 ) ;
#35657=DIRECTION ( 'NONE',  ( 0.000000000000000000, 0.000000000000000000, 1.000000000000000000 ) ) ;
#35658=DIRECTION ( 'NONE',  ( 0.000000000000000000, 0.000000000000000000, 1.000000000000000000 ) ) ;
#35660=ORIENTED_EDGE ( 'NONE', *, *, #7394, .F. ) ;
#35663=LINE ( 'NONE', #48281, #50070 ) ;
#35666=DIRECTION ( 'NONE',  ( 0.000000000000000000, 1.000000000000000000, 0.000000000000000000 ) ) ;
#35667=DIRECTION ( 'NONE',  ( 0.000000000000000000, 0.000000000000000000, 1.000000000000000000 ) ) ;
#35671=DIRECTION ( 'NONE',  ( -0.8757349421956310831, 0.000000000000000000, -0.4827922027307550712 ) ) ;
#35672=ORIENTED_EDGE ( 'NONE', *, *, #30340, .T. ) ;
#35675=FACE_BOUND ( 'NONE', #7050, .T. ) ;
#35676=DIRECTION ( 'NONE',  ( 0.5586467658036535777, 0.000000000000000000, -0.8294056854502011022 ) ) ;
#35677=ORIENTED_EDGE ( 'NONE', *, *, #11468, .T. ) ;
#35678=AXIS2_PLACEMENT_3D ( 'NONE', #14861, #30874, #10899 ) ;
#35680=CARTESIAN_POINT ( 'NONE',  ( -48.47912675150885065, -188.5000000000000284, 15.00000000000000711 ) ) ;
#35681=ORIENTED_EDGE ( 'NONE', *, *, #20192, .T. ) ;
#35684=DIRECTION ( 'NONE',  ( -0.000000000000000000, 1.000000000000000000, -0.000000000000000000 ) ) ;
#35685=EDGE_LOOP ( 'NONE', ( #41804, #7198, #20861, #393 ) ) ;
#35686=CIRCLE ( 'NONE', #3809, 125.0000000000000000 ) ;
#35687=ADVANCED_FACE ( 'NONE', ( #34586 ), #25681, .T. ) ;
#35688=CARTESIAN_POINT ( 'NONE',  ( -171.4559849729830603, -177.1207230881787780, 22.39848972532369942 ) ) ;
#35690=DIRECTION ( 'NONE',  ( 0.000000000000000000, 0.000000000000000000, 1.000000000000000000 ) ) ;
#35691=AXIS2_PLACEMENT_3D ( 'NONE', #16593, #32606, #33117 ) ;
#35692=EDGE_CURVE ( 'NONE', #22760, #16305, #38788, .T. ) ;
#35696=VERTEX_POINT ( 'NONE', #2794 ) ;
#35697=LINE ( 'NONE', #51746, #30870 ) ;
#35698=ORIENTED_EDGE ( 'NONE', *, *, #48821, .T. ) ;
#35701=ORIENTED_EDGE ( 'NONE', *, *, #31001, .T. ) ;
#35702=CARTESIAN_POINT ( 'NONE',  ( -7.223120065443615623, -183.6283474603465606, 117.9955164924470523 ) ) ;
#35703=VERTEX_POINT ( 'NONE', #6758 ) ;
#35705=ORIENTED_EDGE ( 'NONE', *, *, #19539, .T. ) ;
#35706=DIRECTION ( 'NONE',  ( -0.000000000000000000, 1.000000000000000000, 0.000000000000000000 ) ) ;
#35709=CARTESIAN_POINT ( 'NONE',  ( -149.9407190013152160, -193.5000000000000000, -73.01058346660458653 ) ) ;
#35710=EDGE_LOOP ( 'NONE', ( #35014, #32426, #13357, #17922 ) ) ;
#35711=DIRECTION ( 'NONE',  ( 0.000000000000000000, 0.000000000000000000, 1.000000000000000000 ) ) ;
#35713=FACE_OUTER_BOUND ( 'NONE', #17749, .T. ) ;
#35714=CARTESIAN_POINT ( 'NONE',  ( -48.13092511607445090, -183.6283474603465606, -0.9374196611341135688 ) ) ;
#35716=LINE ( 'NONE', #48610, #7308 ) ;
#35718=DIRECTION ( 'NONE',  ( 0.000000000000000000, 1.000000000000000000, 0.000000000000000000 ) ) ;
#35720=EDGE_LOOP ( 'NONE', ( #28814, #28823, #28613, #5400 ) ) ;
#35722=FACE_OUTER_BOUND ( 'NONE', #2661, .T. ) ;
#35725=ORIENTED_EDGE ( 'NONE', *, *, #48478, .T. ) ;
#35730=DIRECTION ( 'NONE',  ( 0.6528221181905280446, 0.000000000000000000, -0.7575112421616145841 ) ) ;
#35732=ORIENTED_EDGE ( 'NONE', *, *, #11193, .F. ) ;
#35734=ORIENTED_EDGE ( 'NONE', *, *, #19919, .T. ) ;
#35735=AXIS2_PLACEMENT_3D ( 'NONE', #4964, #12032, #5223 ) ;
#35736=ORIENTED_EDGE ( 'NONE', *, *, #34439, .T. ) ;
#35737=CIRCLE ( 'NONE', #45848, 10.00000000000000000 ) ;
#35741=DIRECTION ( 'NONE',  ( 0.000000000000000000, 0.000000000000000000, -1.000000000000000000 ) ) ;
#35742=ORIENTED_EDGE ( 'NONE', *, *, #40974, .F. ) ;
#35744=VERTEX_POINT ( 'NONE', #46188 ) ;
#35746=VECTOR ( 'NONE', #9686, 1000.000000000000000 ) ;
#35748=EDGE_CURVE ( 'NONE', #1934, #25631, #5978, .T. ) ;
#35749=DIRECTION ( 'NONE',  ( 0.8455960035018272869, 0.000000000000000000, -0.5338233779647886257 ) ) ;
#35750=VECTOR ( 'NONE', #20798, 1000.000000000000114 ) ;
#35751=AXIS2_PLACEMENT_3D ( 'NONE', #15303, #6393, #39457 ) ;
#35752=ORIENTED_EDGE ( 'NONE', *, *, #12417, .F. ) ;
#35754=CARTESIAN_POINT ( 'NONE',  ( 50.88012955800437709, -177.1207230881787780, 74.18852968774250201 ) ) ;
#35756=CARTESIAN_POINT ( 'NONE',  ( -48.47912675150885065, -177.1207230881787780, 6.938893903907228378E-15 ) ) ;
#35758=CIRCLE ( 'NONE', #50906, 125.0000000000000000 ) ;
#35762=ORIENTED_EDGE ( 'NONE', *, *, #26907, .F. ) ;
#35765=DIRECTION ( 'NONE',  ( -0.7378332790417285736, 0.000000000000000000, 0.6749830015182091136 ) ) ;
#35768=DIRECTION ( 'NONE',  ( 0.05924062789371441901, 0.000000000000000000, -0.9982437317643214625 ) ) ;
#35769=DIRECTION ( 'NONE',  ( -0.000000000000000000, 1.000000000000000000, -0.000000000000000000 ) ) ;
#35771=CIRCLE ( 'NONE', #20662, 125.0000000000000000 ) ;
#35772=DIRECTION ( 'NONE',  ( -0.000000000000000000, 1.000000000000000000, -0.000000000000000000 ) ) ;
#35773=PLANE ( 'NONE',  #48838 ) ;
#35776=DIRECTION ( 'NONE',  ( 0.000000000000000000, 1.000000000000000000, 0.000000000000000000 ) ) ;
#35777=CARTESIAN_POINT ( 'NONE',  ( -238.7407812814481076, -193.5000000000000000, 10.00000000000000178 ) ) ;
#35778=CARTESIAN_POINT ( 'NONE',  ( -47.97059563285963435, -175.3837268820161057, 0.8610436117673654355 ) ) ;
#35780=ORIENTED_EDGE ( 'NONE', *, *, #36002, .F. ) ;
#35781=LINE ( 'NONE', #43428, #4107 ) ;
#35783=ADVANCED_FACE ( 'NONE', ( #30921 ), #2019, .T. ) ;
#35787=VECTOR ( 'NONE', #46736, 1000.000000000000000 ) ;
#35789=CARTESIAN_POINT ( 'NONE',  ( 64.72501964220592185, -175.3837268820161057, 53.00774697410174952 ) ) ;
#35790=LINE ( 'NONE', #51848, #27764 ) ;
#35791=AXIS2_PLACEMENT_3D ( 'NONE', #28408, #44192, #12110 ) ;
#35792=FACE_OUTER_BOUND ( 'NONE', #37211, .T. ) ;
#35793=LINE ( 'NONE', #47376, #31447 ) ;
#35794=DIRECTION ( 'NONE',  ( -0.05924062789370006937, 0.000000000000000000, -0.9982437317643222396 ) ) ;
#35798=VECTOR ( 'NONE', #39456, 1000.000000000000000 ) ;
#35799=EDGE_CURVE ( 'NONE', #24349, #31431, #37766, .T. ) ;
#35801=CARTESIAN_POINT ( 'NONE',  ( 2.066935079424583765, -193.5000000000000000, -114.3245189510257802 ) ) ;
#35803=DIRECTION ( 'NONE',  ( -0.000000000000000000, 1.000000000000000000, -0.000000000000000000 ) ) ;
#35805=MANIFOLD_SOLID_BREP ( 'Cut-Extrude10', #14540 ) ;
#35807=VECTOR ( 'NONE', #37926, 1000.000000000000000 ) ;
#35812=CARTESIAN_POINT ( 'NONE',  ( -48.47912675150885065, -188.5000000000000284, 6.938893903907228378E-15 ) ) ;
#35815=ORIENTED_EDGE ( 'NONE', *, *, #31162, .T. ) ;
#35819=CARTESIAN_POINT ( 'NONE',  ( -47.92047998570520662, -183.6283474603465606, 0.8294056854502119824 ) ) ;
#35820=CARTESIAN_POINT ( 'NONE',  ( -62.32061382540516092, -175.3837268820161057, 123.2250735253144285 ) ) ;
#35821=VERTEX_POINT ( 'NONE', #31949 ) ;
#35824=DIRECTION ( 'NONE',  ( 0.000000000000000000, 1.000000000000000000, 0.000000000000000000 ) ) ;
#35825=FACE_OUTER_BOUND ( 'NONE', #14369, .T. ) ;
#35826=AXIS2_PLACEMENT_3D ( 'NONE', #24815, #32696, #9316 ) ;
#35827=FACE_OUTER_BOUND ( 'NONE', #42651, .T. ) ;
#35829=LINE ( 'NONE', #23744, #20322 ) ;
#35832=DIRECTION ( 'NONE',  ( -0.9995608365087940150, 0.000000000000000000, -0.02963332782257007206 ) ) ;
#35834=DIRECTION ( 'NONE',  ( 0.000000000000000000, 0.000000000000000000, 1.000000000000000000 ) ) ;
#35835=CARTESIAN_POINT ( 'NONE',  ( 72.89680503569744019, -193.5000000000000000, -25.37485791684304459 ) ) ;
#35836=VERTEX_POINT ( 'NONE', #7777 ) ;
#35838=AXIS2_PLACEMENT_3D ( 'NONE', #47921, #35824, #7716 ) ;
#35839=VERTEX_POINT ( 'NONE', #3058 ) ;
#35841=DIRECTION ( 'NONE',  ( 0.000000000000000000, 1.000000000000000000, 0.000000000000000000 ) ) ;
#35843=ORIENTED_EDGE ( 'NONE', *, *, #38691, .T. ) ;
#35844=CARTESIAN_POINT ( 'NONE',  ( -117.6101668435555325, -193.5000000000000000, -102.9412430821794544 ) ) ;
#35846=DIRECTION ( 'NONE',  ( -0.000000000000000000, 1.000000000000000000, -0.000000000000000000 ) ) ;
#35847=ADVANCED_FACE ( 'NONE', ( #43002 ), #7008, .T. ) ;
#35849=CARTESIAN_POINT ( 'NONE',  ( -48.47912675150885065, -177.1207230881787780, 6.938893903907228378E-15 ) ) ;
#35850=VERTEX_POINT ( 'NONE', #15161 ) ;
#35851=LINE ( 'NONE', #43735, #6589 ) ;
#35854=ORIENTED_EDGE ( 'NONE', *, *, #13734, .F. ) ;
#35855=DIRECTION ( 'NONE',  ( 0.000000000000000000, 0.000000000000000000, 1.000000000000000000 ) ) ;
#35856=CARTESIAN_POINT ( 'NONE',  ( -49.08592689732743963, -177.1207230881787780, -0.7948544414133539293 ) ) ;
#35857=DIRECTION ( 'NONE',  ( 0.1768902751225733261, 0.000000000000000000, -0.9842305779475966077 ) ) ;
#35860=CARTESIAN_POINT ( 'NONE',  ( -74.33510315702946514, -177.1207230881787780, -121.2748789083718748 ) ) ;
#35861=LINE ( 'NONE', #7499, #28186 ) ;
#35862=ADVANCED_FACE ( 'NONE', ( #51426 ), #39045, .F. ) ;
#35863=LINE ( 'NONE', #39784, #9804 ) ;
#35865=ORIENTED_EDGE ( 'NONE', *, *, #8050, .T. ) ;
#35868=EDGE_LOOP ( 'NONE', ( #41064, #40147, #38687, #752 ) ) ;
#35869=CIRCLE ( 'NONE', #24106, 125.0000000000000000 ) ;
#35871=EDGE_CURVE ( 'NONE', #21665, #13211, #19103, .T. ) ;
#35873=DIRECTION ( 'NONE',  ( 0.000000000000000000, 1.000000000000000000, 0.000000000000000000 ) ) ;
#35875=CIRCLE ( 'NONE', #19116, 125.0000000000000000 ) ;
#35876=ADVANCED_FACE ( 'NONE', ( #23549 ), #47469, .T. ) ;
#35879=PLANE ( 'NONE',  #5011 ) ;
#35880=VECTOR ( 'NONE', #6434, 1000.000000000000000 ) ;
#35884=DIRECTION ( 'NONE',  ( 0.000000000000000000, 0.000000000000000000, 1.000000000000000000 ) ) ;
#35885=ORIENTED_EDGE ( 'NONE', *, *, #14472, .F. ) ;
#35886=CARTESIAN_POINT ( 'NONE',  ( -2.174401709722249887, -177.1207230881787780, -115.0304316645280096 ) ) ;
#35887=CARTESIAN_POINT ( 'NONE',  ( 76.46082103836693022, -175.3837268820161057, 3.874202661595785191 ) ) ;
#35890=DIRECTION ( 'NONE',  ( -0.000000000000000000, 1.000000000000000000, 0.000000000000000000 ) ) ;
#35891=DIRECTION ( 'NONE',  ( -0.8455960035018199594, 0.000000000000000000, -0.5338233779648003940 ) ) ;
#35892=ORIENTED_EDGE ( 'NONE', *, *, #3999, .T. ) ;
#35896=LINE ( 'NONE', #15936, #12314 ) ;
#35901=VERTEX_POINT ( 'NONE', #43530 ) ;
#35902=DIRECTION ( 'NONE',  ( -0.3482016354344059095, 0.000000000000000000, 0.9374196611341183427 ) ) ;
#35905=CARTESIAN_POINT ( 'NONE',  ( 12.54192669111252734, -183.6283474603465606, 107.9473519284347418 ) ) ;
#35907=AXIS2_PLACEMENT_3D ( 'NONE', #6711, #51376, #42950 ) ;
#35908=ORIENTED_EDGE ( 'NONE', *, *, #21324, .T. ) ;
#35910=FACE_OUTER_BOUND ( 'NONE', #12066, .T. ) ;
#35911=DIRECTION ( 'NONE',  ( 0.000000000000000000, -1.000000000000000000, 0.000000000000000000 ) ) ;
#35912=AXIS2_PLACEMENT_3D ( 'NONE', #41566, #37894, #13988 ) ;
#35913=EDGE_CURVE ( 'NONE', #50038, #30132, #24079, .T. ) ;
#35914=DIRECTION ( 'NONE',  ( 0.000000000000000000, -1.000000000000000000, 0.000000000000000000 ) ) ;
#35916=EDGE_CURVE ( 'NONE', #10098, #7641, #35118, .T. ) ;
#35917=DIRECTION ( 'NONE',  ( 0.6068001458186002006, 0.000000000000000000, -0.7948544414133481562 ) ) ;
#35918=ORIENTED_EDGE ( 'NONE', *, *, #18982, .T. ) ;
#35920=ORIENTED_EDGE ( 'NONE', *, *, #14677, .F. ) ;
#35921=ADVANCED_FACE ( 'NONE', ( #19607 ), #15680, .T. ) ;
#35922=ORIENTED_EDGE ( 'NONE', *, *, #30096, .F. ) ;
#35923=VECTOR ( 'NONE', #37828, 999.9999999999998863 ) ;
#35924=ADVANCED_FACE ( 'NONE', ( #51949 ), #15938, .T. ) ;
#35929=ADVANCED_FACE ( 'NONE', ( #20120 ), #36149, .T. ) ;
#35930=ORIENTED_EDGE ( 'NONE', *, *, #29152, .F. ) ;
#35932=CARTESIAN_POINT ( 'NONE',  ( 45.66222513722992460, -193.5000000000000000, 80.70646587903453906 ) ) ;
#35934=AXIS2_PLACEMENT_3D ( 'NONE', #29427, #28905, #9472 ) ;
#35935=FACE_BOUND ( 'NONE', #9178, .T. ) ;
#35936=ORIENTED_EDGE ( 'NONE', *, *, #3849, .F. ) ;
#35938=DIRECTION ( 'NONE',  ( -0.000000000000000000, 1.000000000000000000, -0.000000000000000000 ) ) ;
#35940=EDGE_CURVE ( 'NONE', #48835, #41991, #48773, .T. ) ;
#35941=VERTEX_POINT ( 'NONE', #44315 ) ;
#35942=DIRECTION ( 'NONE',  ( 0.000000000000000000, 1.000000000000000000, 0.000000000000000000 ) ) ;
#35943=ORIENTED_EDGE ( 'NONE', *, *, #5838, .F. ) ;
#35944=EDGE_CURVE ( 'NONE', #37865, #41127, #24283, .T. ) ;
#35948=VECTOR ( 'NONE', #17711, 1000.000000000000000 ) ;
#35950=FACE_BOUND ( 'NONE', #18641, .T. ) ;
#35951=LINE ( 'NONE', #16499, #10317 ) ;
#35952=VECTOR ( 'NONE', #11831, 1000.000000000000114 ) ;
#35953=CARTESIAN_POINT ( 'NONE',  ( -33.52607327456454556, -175.3837268820161057, -124.1024020384603119 ) ) ;
#35956=EDGE_LOOP ( 'NONE', ( #864, #19022, #42554, #34507 ) ) ;
#35957=CARTESIAN_POINT ( 'NONE',  ( 75.01583293582056911, -175.3837268820161057, 11.18012358327989375 ) ) ;
#35959=ORIENTED_EDGE ( 'NONE', *, *, #29216, .F. ) ;
#35961=DIRECTION ( 'NONE',  ( 0.000000000000000000, 0.000000000000000000, -1.000000000000000000 ) ) ;
#35962=AXIS2_PLACEMENT_3D ( 'NONE', #23875, #3921, #35976 ) ;
#35963=DIRECTION ( 'NONE',  ( 0.000000000000000000, 0.000000000000000000, -1.000000000000000000 ) ) ;
#35964=CARTESIAN_POINT ( 'NONE',  ( -50.83192613281180172, -193.5000000000000000, 123.9784823535113816 ) ) ;
#35965=EDGE_LOOP ( 'NONE', ( #40149, #16200, #14063, #11204 ) ) ;
#35966=CARTESIAN_POINT ( 'NONE',  ( 42.10477485469927927, -183.6283474603465606, 86.13684908212515268 ) ) ;
#35969=ORIENTED_EDGE ( 'NONE', *, *, #8935, .T. ) ;
#35970=LINE ( 'NONE', #47030, #14750 ) ;
#35971=ORIENTED_EDGE ( 'NONE', *, *, #4849, .F. ) ;
#35972=CARTESIAN_POINT ( 'NONE',  ( 66.42899531795131907, -183.6283474603465606, 49.20491319441622124 ) ) ;
#35973=ORIENTED_EDGE ( 'NONE', *, *, #6971, .T. ) ;
#35974=ADVANCED_FACE ( 'NONE', ( #13005 ), #20378, .T. ) ;
#35976=DIRECTION ( 'NONE',  ( 0.000000000000000000, 0.000000000000000000, -1.000000000000000000 ) ) ;
#35978=LINE ( 'NONE', #40170, #39233 ) ;
#35979=DIRECTION ( 'NONE',  ( 0.000000000000000000, 1.000000000000000000, 0.000000000000000000 ) ) ;
#35982=EDGE_CURVE ( 'NONE', #31431, #2085, #8344, .T. ) ;
#35984=ORIENTED_EDGE ( 'NONE', *, *, #38093, .F. ) ;
#35987=CARTESIAN_POINT ( 'NONE',  ( -122.3978016498073345, -193.5000000000000000, -100.8019320314827070 ) ) ;
#35989=DIRECTION ( 'NONE',  ( 0.6300878435817038881, 0.000000000000000000, 0.7765238627180482966 ) ) ;
#35991=CARTESIAN_POINT ( 'NONE',  ( -140.1460956102404509, -175.3837268820161057, 84.98333260264820410 ) ) ;
#35996=CARTESIAN_POINT ( 'NONE',  ( 73.80528149577284580, -175.3837268820161057, 25.91377046305969145 ) ) ;
#35997=CARTESIAN_POINT ( 'NONE',  ( -47.64924157374594671, -175.3837268820161057, 123.9972451320097377 ) ) ;
#35998=DIRECTION ( 'NONE',  ( -0.000000000000000000, -1.000000000000000000, 0.000000000000000000 ) ) ;
#35999=ORIENTED_EDGE ( 'NONE', *, *, #27910, .F. ) ;
#36000=CIRCLE ( 'NONE', #41850, 125.0000000000000000 ) ;
#36001=DIRECTION ( 'NONE',  ( 0.000000000000000000, 0.000000000000000000, 1.000000000000000000 ) ) ;
#36002=EDGE_CURVE ( 'NONE', #5608, #11764, #41914, .T. ) ;
#36004=CYLINDRICAL_SURFACE ( 'NONE', #11874, 125.0000000000000000 ) ;
#36005=ORIENTED_EDGE ( 'NONE', *, *, #45737, .F. ) ;
#36006=ORIENTED_EDGE ( 'NONE', *, *, #42575, .F. ) ;
#36010=DIRECTION ( 'NONE',  ( 0.5085311186492273983, 0.000000000000000000, -0.8610436117673514467 ) ) ;
#36013=DIRECTION ( 'NONE',  ( -0.000000000000000000, 1.000000000000000000, 0.000000000000000000 ) ) ;
#36016=ORIENTED_EDGE ( 'NONE', *, *, #9468, .F. ) ;
#36017=EDGE_LOOP ( 'NONE', ( #9151, #28087, #28551, #2789 ) ) ;
#36019=AXIS2_PLACEMENT_3D ( 'NONE', #48291, #20960, #28563 ) ;
#36020=ORIENTED_EDGE ( 'NONE', *, *, #35602, .F. ) ;
#36022=EDGE_LOOP ( 'NONE', ( #38063, #13437, #16887, #30983 ) ) ;
#36023=DIRECTION ( 'NONE',  ( 0.000000000000000000, -1.000000000000000000, -0.000000000000000000 ) ) ;
#36028=CARTESIAN_POINT ( 'NONE',  ( -162.0868781531755758, -177.1207230881787780, -49.69312418816311094 ) ) ;
#36029=ORIENTED_EDGE ( 'NONE', *, *, #24731, .F. ) ;
#36031=ORIENTED_EDGE ( 'NONE', *, *, #3239, .T. ) ;
#36032=ADVANCED_FACE ( 'NONE', ( #29033 ), #16974, .T. ) ;
#36034=CARTESIAN_POINT ( 'NONE',  ( 57.31108707223382481, -193.5000000000000000, -66.58401203837755133 ) ) ;
#36035=LINE ( 'NONE', #43912, #26583 ) ;
#36036=CARTESIAN_POINT ( 'NONE',  ( -49.42645310536303782, -175.3837268820161057, -0.3202698538628417357 ) ) ;
#36037=ORIENTED_EDGE ( 'NONE', *, *, #35402, .F. ) ;
#36038=VECTOR ( 'NONE', #22350, 1000.000000000000114 ) ;
#36039=LINE ( 'NONE', #36826, #16436 ) ;
#36040=CARTESIAN_POINT ( 'NONE',  ( -129.9529520667707629, -189.7472609257535510, -94.79987230211962412 ) ) ;
#36041=FACE_OUTER_BOUND ( 'NONE', #23252, .T. ) ;
#36044=LINE ( 'NONE', #24737, #19008 ) ;
#36045=DIRECTION ( 'NONE',  ( 0.000000000000000000, -0.000000000000000000, 1.000000000000000000 ) ) ;
#36047=DIRECTION ( 'NONE',  ( -0.4031234292879665171, 0.000000000000000000, -0.9151456172430210145 ) ) ;
#36050=CARTESIAN_POINT ( 'NONE',  ( -98.62206515315352817, -175.3837268820161057, 113.4093733337831225 ) ) ;
#36057=LINE ( 'NONE', #7442, #39837 ) ;
#36060=DIRECTION ( 'NONE',  ( -1.000000000000000000, 0.000000000000000000, -4.884776371667511665E-16 ) ) ;
#36061=CARTESIAN_POINT ( 'NONE',  ( -120.2975302769383177, -193.5000000000000000, 102.3089288139533863 ) ) ;
#36062=CARTESIAN_POINT ( 'NONE',  ( -8.721998590732173540, -183.6283474603465606, -118.5089480183145128 ) ) ;
#36063=CARTESIAN_POINT ( 'NONE',  ( 71.15591247552653442, -177.1207230881787780, 36.22785377504035154 ) ) ;
#36064=VERTEX_POINT ( 'NONE', #1899 ) ;
#36065=ORIENTED_EDGE ( 'NONE', *, *, #4777, .F. ) ;
#36066=LINE ( 'NONE', #12407, #30810 ) ;
#36067=EDGE_CURVE ( 'NONE', #43082, #23765, #47776, .T. ) ;
#36068=AXIS2_PLACEMENT_3D ( 'NONE', #47738, #36401, #43773 ) ;
#36069=VECTOR ( 'NONE', #34510, 1000.000000000000000 ) ;
#36070=DIRECTION ( 'NONE',  ( 0.9374196611341231167, 0.000000000000000000, -0.3482016354343928088 ) ) ;
#36072=ORIENTED_EDGE ( 'NONE', *, *, #39775, .F. ) ;
#36073=ORIENTED_EDGE ( 'NONE', *, *, #29096, .F. ) ;
#36074=CARTESIAN_POINT ( 'NONE',  ( -138.3664773286546108, -193.5000000000000000, -85.41934182508015283 ) ) ;
#36075=CARTESIAN_POINT ( 'NONE',  ( -158.3442440847886985, -175.3837268820161057, -59.62093586438118109 ) ) ;
#36076=CARTESIAN_POINT ( 'NONE',  ( -65.47874029382337824, -183.6283474603465606, 122.8300162461137006 ) ) ;
#36077=DIRECTION ( 'NONE',  ( -0.5085311186492094127, 0.000000000000000000, -0.8610436117673619938 ) ) ;
#36079=ORIENTED_EDGE ( 'NONE', *, *, #644, .F. ) ;
#36080=EDGE_LOOP ( 'NONE', ( #30, #31620, #40349, #11397 ) ) ;
#36082=DIRECTION ( 'NONE',  ( -0.000000000000000000, 1.000000000000000000, -0.000000000000000000 ) ) ;
#36083=CARTESIAN_POINT ( 'NONE',  ( 76.47090317495664635, -189.7472609257535510, -3.534122433557455256 ) ) ;
#36084=CARTESIAN_POINT ( 'NONE',  ( -16.77927958806650821, -183.6283474603465606, -120.9136869416130082 ) ) ;
#36085=AXIS2_PLACEMENT_3D ( 'NONE', #790, #17096, #20492 ) ;
#36087=LINE ( 'NONE', #27686, #6298 ) ;
#36088=ORIENTED_EDGE ( 'NONE', *, *, #46549, .F. ) ;
#36090=EDGE_CURVE ( 'NONE', #2653, #22822, #50265, .T. ) ;
#36092=CARTESIAN_POINT ( 'NONE',  ( -91.49662025983745650, -189.7472609257535510, -116.2991637277475547 ) ) ;
#36094=EDGE_LOOP ( 'NONE', ( #20920, #37228, #15607, #38735 ) ) ;
#36097=ORIENTED_EDGE ( 'NONE', *, *, #2230, .F. ) ;
#36098=DIRECTION ( 'NONE',  ( -0.000000000000000000, 1.000000000000000000, 0.000000000000000000 ) ) ;
#36100=ORIENTED_EDGE ( 'NONE', *, *, #42312, .F. ) ;
#36101=PLANE ( 'NONE',  #5590 ) ;
#36102=CARTESIAN_POINT ( 'NONE',  ( -30.31202594373734627, -193.5000000000000000, -123.6727797384705809 ) ) ;
#36104=FACE_OUTER_BOUND ( 'NONE', #15865, .T. ) ;
#36106=FACE_OUTER_BOUND ( 'NONE', #8162, .T. ) ;
#36107=CIRCLE ( 'NONE', #3364, 125.0000000000000000 ) ;
#36109=VERTEX_POINT ( 'NONE', #19230 ) ;
#36110=LINE ( 'NONE', #31909, #46701 ) ;
#36112=PLANE ( 'NONE',  #12841 ) ;
#36113=DIRECTION ( 'NONE',  ( 0.000000000000000000, 0.000000000000000000, 1.000000000000000000 ) ) ;
#36114=ADVANCED_FACE ( 'NONE', ( #22907 ), #38415, .T. ) ;
#36115=ORIENTED_EDGE ( 'NONE', *, *, #36067, .T. ) ;
#36116=DIRECTION ( 'NONE',  ( -0.9266896074318317078, 0.000000000000000000, -0.3758275821142421647 ) ) ;
#36119=DIRECTION ( 'NONE',  ( -0.000000000000000000, 1.000000000000000000, -0.000000000000000000 ) ) ;
#36120=ORIENTED_EDGE ( 'NONE', *, *, #635, .F. ) ;
#36121=CARTESIAN_POINT ( 'NONE',  ( 65.38692482895591240, -193.5000000000000000, -51.57055649762701677 ) ) ;
#36122=EDGE_LOOP ( 'NONE', ( #20928, #48107, #22298, #46376 ) ) ;
#36123=ORIENTED_EDGE ( 'NONE', *, *, #50415, .F. ) ;
#36124=VECTOR ( 'NONE', #18320, 999.9999999999998863 ) ;
#36126=FACE_OUTER_BOUND ( 'NONE', #15606, .T. ) ;
#36129=PLANE ( 'NONE',  #43889 ) ;
#36130=DIRECTION ( 'NONE',  ( 0.000000000000000000, 0.000000000000000000, 1.000000000000000000 ) ) ;
#36131=ORIENTED_EDGE ( 'NONE', *, *, #633, .F. ) ;
#36133=FACE_OUTER_BOUND ( 'NONE', #50556, .T. ) ;
#36138=EDGE_CURVE ( 'NONE', #39416, #29039, #26839, .T. ) ;
#36139=EDGE_CURVE ( 'NONE', #4082, #17420, #38664, .T. ) ;
#36143=VERTEX_POINT ( 'NONE', #42618 ) ;
#36144=VECTOR ( 'NONE', #21626, 1000.000000000000000 ) ;
#36145=VECTOR ( 'NONE', #15794, 1000.000000000000000 ) ;
#36146=VERTEX_POINT ( 'NONE', #6633 ) ;
#36147=CARTESIAN_POINT ( 'NONE',  ( -144.2430459457361280, -193.5000000000000000, 78.77358243914957825 ) ) ;
#36149=PLANE ( 'NONE',  #27616 ) ;
#36152=ORIENTED_EDGE ( 'NONE', *, *, #1884, .F. ) ;
#36153=EDGE_CURVE ( 'NONE', #3854, #1503, #30179, .T. ) ;
#36154=EDGE_CURVE ( 'NONE', #50970, #12506, #18708, .T. ) ;
#36155=DIRECTION ( 'NONE',  ( 0.9995608365087946812, 0.000000000000000000, -0.02963332782254913048 ) ) ;
#36156=ORIENTED_EDGE ( 'NONE', *, *, #47006, .T. ) ;
#36157=PLANE ( 'NONE',  #45798 ) ;
#36158=VERTEX_POINT ( 'NONE', #34990 ) ;
#36159=ORIENTED_EDGE ( 'NONE', *, *, #11834, .T. ) ;
#36161=CIRCLE ( 'NONE', #30277, 125.0000000000000000 ) ;
#36164=LINE ( 'NONE', #27508, #49003 ) ;
#36166=EDGE_LOOP ( 'NONE', ( #35762, #37078, #39822, #47878 ) ) ;
#36167=CARTESIAN_POINT ( 'NONE',  ( -149.1282321233094876, -189.7472609257535510, -72.42760398749013007 ) ) ;
#36170=DIRECTION ( 'NONE',  ( 0.8124868780056825335, 0.000000000000000000, -0.5829794791144703447 ) ) ;
#36171=DIRECTION ( 'NONE',  ( -0.000000000000000000, 1.000000000000000000, -0.000000000000000000 ) ) ;
#36172=DIRECTION ( 'NONE',  ( 0.000000000000000000, 0.000000000000000000, -1.000000000000000000 ) ) ;
#36173=CIRCLE ( 'NONE', #32803, 125.0000000000000000 ) ;
#36174=CARTESIAN_POINT ( 'NONE',  ( -48.47912675150885065, -175.3837268820161057, 6.938893903907228378E-15 ) ) ;
#36175=LINE ( 'NONE', #32232, #19501 ) ;
#36177=PLANE ( 'NONE',  #13753 ) ;
#36178=DIRECTION ( 'NONE',  ( -0.000000000000000000, 1.000000000000000000, 0.000000000000000000 ) ) ;
#36179=CIRCLE ( 'NONE', #37045, 125.0000000000000000 ) ;
#36180=FACE_BOUND ( 'NONE', #22644, .T. ) ;
#36182=LINE ( 'NONE', #8077, #23943 ) ;
#36183=CARTESIAN_POINT ( 'NONE',  ( -48.47912675150885065, -189.7472609257535510, 6.938893903907228378E-15 ) ) ;
#36184=CARTESIAN_POINT ( 'NONE',  ( 60.58466639580034041, -193.5000000000000000, -61.07445476073405644 ) ) ;
#36185=EDGE_LOOP ( 'NONE', ( #31735, #46204, #26538, #11011 ) ) ;
#36186=DIRECTION ( 'NONE',  ( 0.4827922027307490205, 0.000000000000000000, -0.8757349421956345248 ) ) ;
#36188=CYLINDRICAL_SURFACE ( 'NONE', #13342, 125.0000000000000000 ) ;
#36190=EDGE_LOOP ( 'NONE', ( #23935, #13855, #50737, #4165, #48391 ) ) ;
#36195=EDGE_LOOP ( 'NONE', ( #10024, #40238, #42789, #16056 ) ) ;
#36196=EDGE_CURVE ( 'NONE', #51929, #39115, #38575, .T. ) ;
#36197=EDGE_LOOP ( 'NONE', ( #35169, #9863, #6201, #41112 ) ) ;
#36198=CARTESIAN_POINT ( 'NONE',  ( -112.1919339979530150, -193.5000000000000000, 107.5438431188761683 ) ) ;
#36199=ORIENTED_EDGE ( 'NONE', *, *, #26364, .T. ) ;
#36200=EDGE_CURVE ( 'NONE', #26846, #17445, #43403, .T. ) ;
#36201=PLANE ( 'NONE',  #11640 ) ;
#36202=EDGE_CURVE ( 'NONE', #9658, #8712, #43597, .T. ) ;
#36204=CIRCLE ( 'NONE', #15254, 125.0000000000000000 ) ;
#36205=ADVANCED_FACE ( 'NONE', ( #34469 ), #46572, .T. ) ;
#36206=VECTOR ( 'NONE', #9619, 1000.000000000000000 ) ;
#36207=ADVANCED_FACE ( 'NONE', ( #15538 ), #31553, .T. ) ;
#36209=PLANE ( 'NONE',  #34297 ) ;
#36211=EDGE_LOOP ( 'NONE', ( #11465, #14142, #4196, #7493 ) ) ;
#36212=DIRECTION ( 'NONE',  ( 0.000000000000000000, -1.000000000000000000, 0.000000000000000000 ) ) ;
#36213=CARTESIAN_POINT ( 'NONE',  ( 50.08808042611238420, -177.1207230881787780, -76.87330921200083367 ) ) ;
#36214=VERTEX_POINT ( 'NONE', #47863 ) ;
#36215=ORIENTED_EDGE ( 'NONE', *, *, #29162, .F. ) ;
#36216=ADVANCED_FACE ( 'NONE', ( #3970 ), #12359, .T. ) ;
#36219=DIRECTION ( 'NONE',  ( -0.2059786187410953262, 0.000000000000000000, -0.9785564922995046988 ) ) ;
#36220=ORIENTED_EDGE ( 'NONE', *, *, #6812, .T. ) ;
#36222=LINE ( 'NONE', #9167, #49423 ) ;
#36223=ORIENTED_EDGE ( 'NONE', *, *, #44298, .T. ) ;
#36224=LINE ( 'NONE', #23618, #14041 ) ;
#36225=DIRECTION ( 'NONE',  ( -0.000000000000000000, 1.000000000000000000, -0.000000000000000000 ) ) ;
#36228=ORIENTED_EDGE ( 'NONE', *, *, #51954, .T. ) ;
#36230=FACE_OUTER_BOUND ( 'NONE', #27998, .T. ) ;
#36232=DIRECTION ( 'NONE',  ( -0.000000000000000000, 1.000000000000000000, -0.000000000000000000 ) ) ;
#36234=DIRECTION ( 'NONE',  ( 0.000000000000000000, -1.000000000000000000, 0.000000000000000000 ) ) ;
#36235=CARTESIAN_POINT ( 'NONE',  ( -159.5526844214375615, -177.1207230881787780, 57.33816169485226055 ) ) ;
#36237=SHAPE_DEFINITION_REPRESENTATION ( #6300, #2890 ) ;
#36239=EDGE_CURVE ( 'NONE', #47580, #28774, #24201, .T. ) ;
#36243=LINE ( 'NONE', #20474, #4708 ) ;
#36244=AXIS2_PLACEMENT_3D ( 'NONE', #19740, #27640, #8437 ) ;
#36245=CARTESIAN_POINT ( 'NONE',  ( -14.52059121095390992, -183.6283474603465606, 119.2602935412682399 ) ) ;
#36247=ORIENTED_EDGE ( 'NONE', *, *, #48285, .F. ) ;
#36248=EDGE_LOOP ( 'NONE', ( #13542, #33893, #21743, #48278 ) ) ;
#36249=CIRCLE ( 'NONE', #49703, 125.0000000000000000 ) ;
#36253=PLANE ( 'NONE',  #44399 ) ;
#36254=CARTESIAN_POINT ( 'NONE',  ( 71.35177504360963496, -175.3837268820161057, 31.88354567335082024 ) ) ;
#36255=CARTESIAN_POINT ( 'NONE',  ( -112.1919339979530150, -175.3837268820161057, 107.5438431188761683 ) ) ;
#36257=EDGE_CURVE ( 'NONE', #32445, #37251, #1556, .T. ) ;
#36258=EDGE_CURVE ( 'NONE', #4155, #32314, #43898, .T. ) ;
#36262=ORIENTED_EDGE ( 'NONE', *, *, #46422, .T. ) ;
#36265=VECTOR ( 'NONE', #21617, 1000.000000000000000 ) ;
#36266=AXIS2_PLACEMENT_3D ( 'NONE', #10113, #29559, #25617 ) ;
#36268=CARTESIAN_POINT ( 'NONE',  ( -164.2529447963538871, -193.5000000000000000, 44.41421852208715393 ) ) ;
#36269=EDGE_CURVE ( 'NONE', #26701, #34028, #47702, .T. ) ;
#36274=DIRECTION ( 'NONE',  ( 0.000000000000000000, -1.000000000000000000, 0.000000000000000000 ) ) ;
#36275=ORIENTED_EDGE ( 'NONE', *, *, #16236, .F. ) ;
#36276=EDGE_CURVE ( 'NONE', #17499, #40613, #7645, .T. ) ;
#36277=PLANE ( 'NONE',  #39877 ) ;
#36279=CARTESIAN_POINT ( 'NONE',  ( -5.732832253866452454, -189.7472609257535510, -117.4638425504666799 ) ) ;
#36281=VERTEX_POINT ( 'NONE', #7895 ) ;
#36282=EDGE_CURVE ( 'NONE', #21757, #6199, #15928, .T. ) ;
#36284=CARTESIAN_POINT ( 'NONE',  ( 69.99104047056317768, -175.3837268820161057, -39.87254040532513244 ) ) ;
#36285=DIRECTION ( 'NONE',  ( 0.000000000000000000, -0.000000000000000000, -1.000000000000000000 ) ) ;
#36287=ORIENTED_EDGE ( 'NONE', *, *, #27452, .F. ) ;
#36288=EDGE_CURVE ( 'NONE', #50756, #19096, #48647, .T. ) ;
#36289=AXIS2_PLACEMENT_3D ( 'NONE', #32054, #48359, #8152 ) ;
#36290=LINE ( 'NONE', #12102, #28148 ) ;
#36291=DIRECTION ( 'NONE',  ( -0.000000000000000000, 1.000000000000000000, -0.000000000000000000 ) ) ;
#36293=ORIENTED_EDGE ( 'NONE', *, *, #6800, .T. ) ;
#36294=PLANE ( 'NONE',  #25806 ) ;
#36296=DIRECTION ( 'NONE',  ( 0.000000000000000000, -1.000000000000000000, -0.000000000000000000 ) ) ;
#36297=VERTEX_POINT ( 'NONE', #8421 ) ;
#36299=CIRCLE ( 'NONE', #29588, 125.0000000000000000 ) ;
#36301=VECTOR ( 'NONE', #35577, 1000.000000000000227 ) ;
#36302=ADVANCED_FACE ( 'NONE', ( #24448 ), #19720, .F. ) ;
#36304=DIRECTION ( 'NONE',  ( 0.000000000000000000, 0.000000000000000000, -1.000000000000000000 ) ) ;
#36305=ORIENTED_EDGE ( 'NONE', *, *, #22522, .T. ) ;
#36306=VECTOR ( 'NONE', #5771, 1000.000000000000000 ) ;
#36307=VECTOR ( 'NONE', #11816, 1000.000000000000000 ) ;
#36310=DIRECTION ( 'NONE',  ( 0.9842305779475980509, 0.000000000000000000, -0.1768902751225666647 ) ) ;
#36312=DIRECTION ( 'NONE',  ( -0.000000000000000000, 1.000000000000000000, -0.000000000000000000 ) ) ;
#36314=DIRECTION ( 'NONE',  ( -0.000000000000000000, 1.000000000000000000, 0.000000000000000000 ) ) ;
#36315=DIRECTION ( 'NONE',  ( 0.000000000000000000, -0.000000000000000000, -1.000000000000000000 ) ) ;
#36318=ORIENTED_EDGE ( 'NONE', *, *, #51160, .T. ) ;
#36320=VECTOR ( 'NONE', #10386, 1000.000000000000114 ) ;
#36321=ORIENTED_EDGE ( 'NONE', *, *, #48139, .T. ) ;
#36322=ADVANCED_FACE ( 'NONE', ( #25491 ), #28639, .T. ) ;
#36325=AXIS2_PLACEMENT_3D ( 'NONE', #35812, #15861, #19517 ) ;
#36326=CARTESIAN_POINT ( 'NONE',  ( -91.84482189527193441, -193.5000000000000000, -117.2365833888816695 ) ) ;
#36327=ORIENTED_EDGE ( 'NONE', *, *, #30508, .T. ) ;
#36328=ORIENTED_EDGE ( 'NONE', *, *, #49284, .F. ) ;
#36329=EDGE_LOOP ( 'NONE', ( #3340, #26201, #3700, #4375 ) ) ;
#36330=CARTESIAN_POINT ( 'NONE',  ( -112.2501518587238962, -189.7472609257535510, -106.3450133598699807 ) ) ;
#36332=CARTESIAN_POINT ( 'NONE',  ( -48.59739992243020623, -189.7472609257535510, -0.9929810960135115883 ) ) ;
#36334=ORIENTED_EDGE ( 'NONE', *, *, #45210, .T. ) ;
#36335=VECTOR ( 'NONE', #41434, 1000.000000000000000 ) ;
#36336=VERTEX_POINT ( 'NONE', #33111 ) ;
#36341=ORIENTED_EDGE ( 'NONE', *, *, #41916, .F. ) ;
#36342=AXIS2_PLACEMENT_3D ( 'NONE', #37268, #41201, #33335 ) ;
#36343=EDGE_CURVE ( 'NONE', #48288, #49251, #801, .T. ) ;
#36344=LINE ( 'NONE', #12430, #32889 ) ;
#36345=CARTESIAN_POINT ( 'NONE',  ( -140.5933766095837427, -175.3837268820161057, -84.49831343337066869 ) ) ;
#36349=CARTESIAN_POINT ( 'NONE',  ( -154.2693405752510500, -193.5000000000000000, 66.58401203837830451 ) ) ;
#36350=DIRECTION ( 'NONE',  ( 0.000000000000000000, 0.000000000000000000, 1.000000000000000000 ) ) ;
#36351=CARTESIAN_POINT ( 'NONE',  ( -138.3664773286545824, -183.6283474603465606, -85.41934182508016704 ) ) ;
#36353=VERTEX_POINT ( 'NONE', #37590 ) ;
#36355=ORIENTED_EDGE ( 'NONE', *, *, #32057, .T. ) ;
#36356=DIRECTION ( 'NONE',  ( 0.000000000000000000, 1.000000000000000000, 0.000000000000000000 ) ) ;
#36358=ORIENTED_EDGE ( 'NONE', *, *, #44666, .T. ) ;
#36359=FACE_OUTER_BOUND ( 'NONE', #7855, .T. ) ;
#36361=FACE_OUTER_BOUND ( 'NONE', #35720, .T. ) ;
#36363=CARTESIAN_POINT ( 'NONE',  ( -49.17567778057184569, -183.6283474603465606, -0.7175072570443327136 ) ) ;
#36364=AXIS2_PLACEMENT_3D ( 'NONE', #49486, #25807, #12925 ) ;
#36365=ORIENTED_EDGE ( 'NONE', *, *, #32659, .F. ) ;
#36366=CARTESIAN_POINT ( 'NONE',  ( -48.64924157374595381, -175.3837268820161057, 123.9998842437354227 ) ) ;
#36367=ORIENTED_EDGE ( 'NONE', *, *, #9704, .T. ) ;
#36368=FACE_BOUND ( 'NONE', #14615, .T. ) ;
#36371=CARTESIAN_POINT ( 'NONE',  ( 50.88012955800437709, -183.6283474603465606, 74.18852968774250201 ) ) ;
#36374=AXIS2_PLACEMENT_3D ( 'NONE', #5600, #2665, #49735 ) ;
#36378=ORIENTED_EDGE ( 'NONE', *, *, #21509, .T. ) ;
#36380=AXIS2_PLACEMENT_3D ( 'NONE', #45369, #20392, #13298 ) ;
#36381=CARTESIAN_POINT ( 'NONE',  ( 73.50869128264331209, -177.1207230881787780, -22.25084316132035056 ) ) ;
#36382=LINE ( 'NONE', #32185, #12699 ) ;
#36383=ORIENTED_EDGE ( 'NONE', *, *, #42322, .T. ) ;
#36385=CARTESIAN_POINT ( 'NONE',  ( 36.10886851198521441, -193.5000000000000000, 92.03190238880813467 ) ) ;
#36386=ADVANCED_FACE ( 'NONE', ( #1830 ), #49160, .F. ) ;
#36390=ORIENTED_EDGE ( 'NONE', *, *, #10517, .T. ) ;
#36392=DIRECTION ( 'NONE',  ( -0.000000000000000000, 1.000000000000000000, -0.000000000000000000 ) ) ;
#36396=ORIENTED_EDGE ( 'NONE', *, *, #25292, .F. ) ;
#36397=VERTEX_POINT ( 'NONE', #13409 ) ;
#36398=VECTOR ( 'NONE', #14415, 1000.000000000000000 ) ;
#36399=ORIENTED_EDGE ( 'NONE', *, *, #9184, .F. ) ;
#36400=CARTESIAN_POINT ( 'NONE',  ( -49.47868758801764955, -193.5000000000000000, -0.02963332782256313663 ) ) ;
#36401=DIRECTION ( 'NONE',  ( -0.000000000000000000, 1.000000000000000000, -0.000000000000000000 ) ) ;
#36402=EDGE_CURVE ( 'NONE', #7460, #5112, #13927, .T. ) ;
#36408=ORIENTED_EDGE ( 'NONE', *, *, #568, .T. ) ;
#36409=CARTESIAN_POINT ( 'NONE',  ( 47.28479244271901649, -193.5000000000000000, -78.77358243914883928 ) ) ;
#36410=EDGE_LOOP ( 'NONE', ( #14391, #48179, #19927, #33895 ) ) ;
#36411=ORIENTED_EDGE ( 'NONE', *, *, #15645, .F. ) ;
#36412=FACE_OUTER_BOUND ( 'NONE', #15837, .T. ) ;
#36413=DIRECTION ( 'NONE',  ( 0.000000000000000000, 0.000000000000000000, 1.000000000000000000 ) ) ;
#36414=CARTESIAN_POINT ( 'NONE',  ( -77.77032474405882567, -175.3837268820161057, 120.4907712303052989 ) ) ;
#36417=CARTESIAN_POINT ( 'NONE',  ( 18.00181100848372040, -183.6283474603465606, -105.8550183720733742 ) ) ;
#36420=CARTESIAN_POINT ( 'NONE',  ( 62.13187335169531877, -177.1207230881787780, -58.22548115875871844 ) ) ;
#36421=DIRECTION ( 'NONE',  ( -0.9995608365087946812, 0.000000000000000000, 0.02963332782254913048 ) ) ;
#36422=CARTESIAN_POINT ( 'NONE',  ( -99.02518858244150124, -193.5000000000000000, 114.3245189510261497 ) ) ;
#36423=CIRCLE ( 'NONE', #42323, 125.0000000000000000 ) ;
#36424=CARTESIAN_POINT ( 'NONE',  ( -48.47912675150885065, -177.1207230881787780, 6.938893903907228378E-15 ) ) ;
#36425=VECTOR ( 'NONE', #33594, 1000.000000000000000 ) ;
#36426=EDGE_CURVE ( 'NONE', #3068, #27986, #691, .T. ) ;
#36427=DIRECTION ( 'NONE',  ( 0.000000000000000000, -1.000000000000000000, -0.000000000000000000 ) ) ;
#36428=DIRECTION ( 'NONE',  ( 0.000000000000000000, 1.000000000000000000, 0.000000000000000000 ) ) ;
#36431=CARTESIAN_POINT ( 'NONE',  ( -18.95304271317703382, -193.5000000000000000, -121.4627941443854837 ) ) ;
#36433=EDGE_CURVE ( 'NONE', #1427, #30234, #17106, .T. ) ;
#36434=CARTESIAN_POINT ( 'NONE',  ( 41.41233698655026529, -193.5000000000000000, 86.85922373029363541 ) ) ;
#36435=FACE_BOUND ( 'NONE', #3255, .T. ) ;
#36436=ORIENTED_EDGE ( 'NONE', *, *, #47218, .T. ) ;
#36437=DIRECTION ( 'NONE',  ( 0.000000000000000000, 0.000000000000000000, -1.000000000000000000 ) ) ;
#36438=CARTESIAN_POINT ( 'NONE',  ( 74.31448861501728231, -183.6283474603465606, -23.38221600314289361 ) ) ;
#36439=ORIENTED_EDGE ( 'NONE', *, *, #24708, .T. ) ;
#36440=DIRECTION ( 'NONE',  ( -0.8610436117673548884, 0.000000000000000000, -0.5085311186492216251 ) ) ;
#36442=CIRCLE ( 'NONE', #38130, 124.9999999999999858 ) ;
#36447=FACE_BOUND ( 'NONE', #30229, .T. ) ;
#36448=DIRECTION ( 'NONE',  ( 0.000000000000000000, -1.000000000000000000, 0.000000000000000000 ) ) ;
#36449=EDGE_LOOP ( 'NONE', ( #7090, #43557, #4744, #45304 ) ) ;
#36450=LINE ( 'NONE', #20171, #7580 ) ;
#36451=VERTEX_POINT ( 'NONE', #20776 ) ;
#36452=ORIENTED_EDGE ( 'NONE', *, *, #3815, .F. ) ;
#36454=EDGE_LOOP ( 'NONE', ( #46122, #44464, #50983, #35701 ) ) ;
#36455=EDGE_CURVE ( 'NONE', #35554, #1331, #29175, .T. ) ;
#36457=VECTOR ( 'NONE', #35500, 1000.000000000000000 ) ;
#36460=AXIS2_PLACEMENT_3D ( 'NONE', #27455, #3800, #47953 ) ;
#36461=CYLINDRICAL_SURFACE ( 'NONE', #44072, 125.0000000000000000 ) ;
#36465=ORIENTED_EDGE ( 'NONE', *, *, #41443, .T. ) ;
#36466=ORIENTED_EDGE ( 'NONE', *, *, #6643, .T. ) ;
#36467=VECTOR ( 'NONE', #51747, 1000.000000000000114 ) ;
#36468=FACE_OUTER_BOUND ( 'NONE', #44545, .T. ) ;
#36469=ORIENTED_EDGE ( 'NONE', *, *, #19193, .F. ) ;
#36471=ORIENTED_EDGE ( 'NONE', *, *, #23861, .F. ) ;
#36472=PLANE ( 'NONE',  #49797 ) ;
#36473=LINE ( 'NONE', #12574, #14154 ) ;
#36474=ORIENTED_EDGE ( 'NONE', *, *, #11504, .T. ) ;
#36476=CARTESIAN_POINT ( 'NONE',  ( -145.0195698084541505, -189.7472609257535510, 79.40367028273126948 ) ) ;
#36478=EDGE_LOOP ( 'NONE', ( #30046, #20018, #14543, #19719, #35199 ) ) ;
#36480=DIRECTION ( 'NONE',  ( 0.000000000000000000, 0.000000000000000000, 1.000000000000000000 ) ) ;
#36482=CARTESIAN_POINT ( 'NONE',  ( -47.97059563285962724, -183.6283474603465606, -0.8610436117673480050 ) ) ;
#36485=DIRECTION ( 'NONE',  ( -0.000000000000000000, 1.000000000000000000, -0.000000000000000000 ) ) ;
#36486=EDGE_CURVE ( 'NONE', #27201, #20876, #7521, .T. ) ;
#36487=EDGE_CURVE ( 'NONE', #21200, #38380, #42807, .T. ) ;
#36491=DIRECTION ( 'NONE',  ( 0.2920567706369628924, 0.000000000000000000, 0.9564009842765264224 ) ) ;
#36492=DIRECTION ( 'NONE',  ( 0.000000000000000000, -0.000000000000000000, -1.000000000000000000 ) ) ;
#36493=ORIENTED_EDGE ( 'NONE', *, *, #11898, .T. ) ;
#36494=ORIENTED_EDGE ( 'NONE', *, *, #42927, .F. ) ;
#36496=CARTESIAN_POINT ( 'NONE',  ( 35.67816836544800907, -177.1207230881787780, -92.42591454022745268 ) ) ;
#36498=VECTOR ( 'NONE', #7483, 1000.000000000000000 ) ;
#36499=VECTOR ( 'NONE', #16752, 1000.000000000000000 ) ;
#36502=ORIENTED_EDGE ( 'NONE', *, *, #27401, .T. ) ;
#36503=ORIENTED_EDGE ( 'NONE', *, *, #21336, .T. ) ;
#36504=ADVANCED_FACE ( 'NONE', ( #22840 ), #31231, .T. ) ;
#36507=EDGE_CURVE ( 'NONE', #34352, #38645, #10486, .T. ) ;
#36509=EDGE_CURVE ( 'NONE', #40230, #41523, #28389, .T. ) ;
#36511=VECTOR ( 'NONE', #42286, 1000.000000000000000 ) ;
#36513=DIRECTION ( 'NONE',  ( 0.000000000000000000, 0.000000000000000000, 1.000000000000000000 ) ) ;
#36515=EDGE_CURVE ( 'NONE', #16210, #20990, #2609, .T. ) ;
#36516=ORIENTED_EDGE ( 'NONE', *, *, #25967, .T. ) ;
#36518=CIRCLE ( 'NONE', #30664, 125.0000000000000000 ) ;
#36519=LINE ( 'NONE', #8671, #31061 ) ;
#36521=CARTESIAN_POINT ( 'NONE',  ( -63.96873441216509093, -175.3837268820161057, -123.0287672223651612 ) ) ;
#36523=VECTOR ( 'NONE', #13410, 1000.000000000000000 ) ;
#36524=EDGE_LOOP ( 'NONE', ( #15028, #18791, #27672, #33720 ) ) ;
#36527=FACE_OUTER_BOUND ( 'NONE', #27331, .T. ) ;
#36528=EDGE_CURVE ( 'NONE', #4350, #39566, #20881, .T. ) ;
#36529=DIRECTION ( 'NONE',  ( 0.7378332790417239107, 0.000000000000000000, 0.6749830015182142207 ) ) ;
#36531=ORIENTED_EDGE ( 'NONE', *, *, #13166, .T. ) ;
#36533=CARTESIAN_POINT ( 'NONE',  ( -47.60339180931321579, -189.7472609257535510, -0.4827922027307358088 ) ) ;
#36534=CIRCLE ( 'NONE', #29830, 125.0000000000000568 ) ;
#36535=ORIENTED_EDGE ( 'NONE', *, *, #43712, .T. ) ;
#36538=ORIENTED_EDGE ( 'NONE', *, *, #43975, .F. ) ;
#36539=AXIS2_PLACEMENT_3D ( 'NONE', #32363, #12392, #28416 ) ;
#36540=PLANE ( 'NONE',  #45101 ) ;
#36541=DIRECTION ( 'NONE',  ( 0.000000000000000000, -1.000000000000000000, 0.000000000000000000 ) ) ;
#36543=DIRECTION ( 'NONE',  ( 0.000000000000000000, 1.000000000000000000, 0.000000000000000000 ) ) ;
#36544=ORIENTED_EDGE ( 'NONE', *, *, #4412, .T. ) ;
#36545=ADVANCED_FACE ( 'NONE', ( #34152 ), #2082, .T. ) ;
#36547=CARTESIAN_POINT ( 'NONE',  ( -59.16959496120699669, -183.6283474603465606, 123.5388265266452379 ) ) ;
#36548=CARTESIAN_POINT ( 'NONE',  ( -48.47912675150885065, -177.1207230881787780, 6.938893903907228378E-15 ) ) ;
#36549=ORIENTED_EDGE ( 'NONE', *, *, #51338, .T. ) ;
#36551=DIRECTION ( 'NONE',  ( 0.000000000000000000, 0.000000000000000000, -1.000000000000000000 ) ) ;
#36554=CARTESIAN_POINT ( 'NONE',  ( 15.80042947435468470, -189.7472609257535510, 107.2060569716377927 ) ) ;
#36556=EDGE_CURVE ( 'NONE', #44074, #33733, #15219, .T. ) ;
#36559=ADVANCED_FACE ( 'NONE', ( #22064 ), #38606, .T. ) ;
#36560=CARTESIAN_POINT ( 'NONE',  ( -44.48323084606168720, -193.5000000000000000, 124.9361149384469769 ) ) ;
#36561=VECTOR ( 'NONE', #30091, 1000.000000000000000 ) ;
#36562=DIRECTION ( 'NONE',  ( -0.3482016354343866471, 0.000000000000000000, -0.9374196611341253371 ) ) ;
#36565=LINE ( 'NONE', #13186, #20738 ) ;
#36568=ADVANCED_FACE ( 'NONE', ( #7073 ), #30978, .F. ) ;
#36574=EDGE_CURVE ( 'NONE', #21083, #40342, #6299, .T. ) ;
#36575=DIRECTION ( 'NONE',  ( -0.9374196611341206742, 0.000000000000000000, -0.3482016354343996367 ) ) ;
#36576=VECTOR ( 'NONE', #40188, 1000.000000000000114 ) ;
#36577=EDGE_CURVE ( 'NONE', #42139, #7207, #31491, .T. ) ;
#36580=LINE ( 'NONE', #4799, #43807 ) ;
#36581=ORIENTED_EDGE ( 'NONE', *, *, #40156, .F. ) ;
#36583=VECTOR ( 'NONE', #10017, 1000.000000000000000 ) ;
#36584=AXIS2_PLACEMENT_3D ( 'NONE', #27834, #8141, #4718 ) ;
#36586=ORIENTED_EDGE ( 'NONE', *, *, #50725, .F. ) ;
#36589=CARTESIAN_POINT ( 'NONE',  ( -47.64924157374594671, -193.5000000000000000, 123.9972451320097377 ) ) ;
#36590=ORIENTED_EDGE ( 'NONE', *, *, #5437, .T. ) ;
#36592=VECTOR ( 'NONE', #5031, 1000.000000000000114 ) ;
#36596=CARTESIAN_POINT ( 'NONE',  ( -48.82732838694325750, -183.6283474603465606, 0.9374196611341252261 ) ) ;
#36597=VECTOR ( 'NONE', #29703, 1000.000000000000114 ) ;
#36600=ORIENTED_EDGE ( 'NONE', *, *, #8636, .F. ) ;
#36603=AXIS2_PLACEMENT_3D ( 'NONE', #17305, #4685, #44627 ) ;
#36605=DIRECTION ( 'NONE',  ( -0.8455960035018311727, 0.000000000000000000, 0.5338233779647826305 ) ) ;
#36607=ORIENTED_EDGE ( 'NONE', *, *, #22408, .F. ) ;
#36609=FACE_OUTER_BOUND ( 'NONE', #33495, .T. ) ;
#36610=ORIENTED_EDGE ( 'NONE', *, *, #51350, .T. ) ;
#36611=CARTESIAN_POINT ( 'NONE',  ( 29.27398957514434130, -183.6283474603465606, -97.87467957287998388 ) ) ;
#36612=ORIENTED_EDGE ( 'NONE', *, *, #14700, .T. ) ;
#36613=DIRECTION ( 'NONE',  ( 0.9995608365087944591, 0.000000000000000000, -0.02963332782255633305 ) ) ;
#36614=DIRECTION ( 'NONE',  ( -0.000000000000000000, 1.000000000000000000, -0.000000000000000000 ) ) ;
#36615=FACE_OUTER_BOUND ( 'NONE', #23817, .T. ) ;
#36616=ORIENTED_EDGE ( 'NONE', *, *, #44663, .T. ) ;
#36620=VECTOR ( 'NONE', #26995, 1000.000000000000114 ) ;
#36621=CARTESIAN_POINT ( 'NONE',  ( -4.794493649713349015, -189.7472609257535510, -117.1181148702518726 ) ) ;
#36622=ORIENTED_EDGE ( 'NONE', *, *, #31824, .T. ) ;
#36624=AXIS2_PLACEMENT_3D ( 'NONE', #50736, #14479, #2634 ) ;
#36630=DIRECTION ( 'NONE',  ( 0.000000000000000000, 0.000000000000000000, -1.000000000000000000 ) ) ;
#36633=VERTEX_POINT ( 'NONE', #52013 ) ;
#36634=DIRECTION ( 'NONE',  ( 0.000000000000000000, 0.000000000000000000, 1.000000000000000000 ) ) ;
#36635=VERTEX_POINT ( 'NONE', #23604 ) ;
#36636=AXIS2_PLACEMENT_3D ( 'NONE', #12693, #32927, #20591 ) ;
#36637=DIRECTION ( 'NONE',  ( 0.2059786187411021818, 0.000000000000000000, -0.9785564922995032555 ) ) ;
#36639=AXIS2_PLACEMENT_3D ( 'NONE', #7560, #7049, #3609 ) ;
#36640=AXIS2_PLACEMENT_3D ( 'NONE', #3791, #6532, #22559 ) ;
#36641=DIRECTION ( 'NONE',  ( -0.5586467658036594619, 0.000000000000000000, 0.8294056854501971054 ) ) ;
#36642=CARTESIAN_POINT ( 'NONE',  ( 141.7825277784304205, -193.5000000000000000, 10.00000000000000178 ) ) ;
#36648=CIRCLE ( 'NONE', #31608, 125.0000000000000000 ) ;
#36649=ORIENTED_EDGE ( 'NONE', *, *, #22045, .T. ) ;
#36650=VERTEX_POINT ( 'NONE', #39621 ) ;
#36653=CARTESIAN_POINT ( 'NONE',  ( 75.17589904515342880, -175.3837268820161057, -18.28755301364250130 ) ) ;
#36655=ORIENTED_EDGE ( 'NONE', *, *, #6032, .T. ) ;
#36657=EDGE_CURVE ( 'NONE', #38881, #44484, #48568, .T. ) ;
#36658=DIRECTION ( 'NONE',  ( 0.000000000000000000, 1.000000000000000000, -0.000000000000000000 ) ) ;
#36660=VECTOR ( 'NONE', #15318, 1000.000000000000000 ) ;
#36665=DIRECTION ( 'NONE',  ( 0.000000000000000000, -0.000000000000000000, -1.000000000000000000 ) ) ;
#36667=CARTESIAN_POINT ( 'NONE',  ( -48.47912675150885065, -177.1207230881787780, 6.938893903907228378E-15 ) ) ;
#36668=DIRECTION ( 'NONE',  ( -0.000000000000000000, 1.000000000000000000, -0.000000000000000000 ) ) ;
#36670=ORIENTED_EDGE ( 'NONE', *, *, #15475, .T. ) ;
#36671=ORIENTED_EDGE ( 'NONE', *, *, #48461, .F. ) ;
#36672=DIRECTION ( 'NONE',  ( -0.000000000000000000, 1.000000000000000000, -0.000000000000000000 ) ) ;
#36673=DIRECTION ( 'NONE',  ( 0.7765238627180437447, 0.000000000000000000, -0.6300878435817094392 ) ) ;
#36674=VECTOR ( 'NONE', #51559, 1000.000000000000000 ) ;
#36676=CARTESIAN_POINT ( 'NONE',  ( -170.0502155641509319, -177.1207230881787780, -29.07697310430878090 ) ) ;
#36679=VECTOR ( 'NONE', #11350, 1000.000000000000000 ) ;
#36680=FACE_OUTER_BOUND ( 'NONE', #44111, .T. ) ;
#36683=AXIS2_PLACEMENT_3D ( 'NONE', #18659, #10767, #11012 ) ;
#36684=ORIENTED_EDGE ( 'NONE', *, *, #24591, .T. ) ;
#36686=ORIENTED_EDGE ( 'NONE', *, *, #36756, .T. ) ;
#36687=DIRECTION ( 'NONE',  ( -0.000000000000000000, 1.000000000000000000, -0.000000000000000000 ) ) ;
#36688=EDGE_LOOP ( 'NONE', ( #36493, #21326, #666, #39356 ) ) ;
#36689=DIRECTION ( 'NONE',  ( -0.000000000000000000, 1.000000000000000000, -0.000000000000000000 ) ) ;
#36690=DIRECTION ( 'NONE',  ( -0.000000000000000000, 1.000000000000000000, -0.000000000000000000 ) ) ;
#36691=LINE ( 'NONE', #48785, #24636 ) ;
#36692=ADVANCED_FACE ( 'NONE', ( #20441 ), #36209, .T. ) ;
#36694=ORIENTED_EDGE ( 'NONE', *, *, #20036, .T. ) ;
#36697=ORIENTED_EDGE ( 'NONE', *, *, #28496, .T. ) ;
#36699=AXIS2_PLACEMENT_3D ( 'NONE', #19366, #23561, #51186 ) ;
#36701=LINE ( 'NONE', #20402, #4334 ) ;
#36702=DIRECTION ( 'NONE',  ( 0.9027978299657387629, 0.000000000000000000, 0.4300652022765304450 ) ) ;
#36705=DIRECTION ( 'NONE',  ( 0.7765238627180437447, 0.000000000000000000, -0.6300878435817094392 ) ) ;
#36706=DIRECTION ( 'NONE',  ( 0.000000000000000000, 0.000000000000000000, -1.000000000000000000 ) ) ;
#36707=DIRECTION ( 'NONE',  ( 0.000000000000000000, 0.000000000000000000, 1.000000000000000000 ) ) ;
#36710=CARTESIAN_POINT ( 'NONE',  ( -48.47912675150885065, -175.3837268820161057, 6.938893903907228378E-15 ) ) ;
#36711=DIRECTION ( 'NONE',  ( -0.000000000000000000, 1.000000000000000000, -0.000000000000000000 ) ) ;
#36712=FACE_BOUND ( 'NONE', #10241, .T. ) ;
#36713=EDGE_LOOP ( 'NONE', ( #27290, #43411, #1491, #1415 ) ) ;
#36714=VECTOR ( 'NONE', #44235, 1000.000000000000114 ) ;
#36715=AXIS2_PLACEMENT_3D ( 'NONE', #28449, #41315, #24512 ) ;
#36716=EDGE_CURVE ( 'NONE', #11672, #15110, #9153, .T. ) ;
#36717=DIRECTION ( 'NONE',  ( -0.000000000000000000, 1.000000000000000000, -0.000000000000000000 ) ) ;
#36718=ORIENTED_EDGE ( 'NONE', *, *, #43369, .T. ) ;
#36719=VECTOR ( 'NONE', #2031, 1000.000000000000000 ) ;
#36720=LINE ( 'NONE', #8848, #17748 ) ;
#36728=ADVANCED_FACE ( 'NONE', ( #40658 ), #36995, .F. ) ;
#36729=DIRECTION ( 'NONE',  ( 0.000000000000000000, -1.000000000000000000, 0.000000000000000000 ) ) ;
#36734=AXIS2_PLACEMENT_3D ( 'NONE', #28461, #44508, #8495 ) ;
#36735=DIRECTION ( 'NONE',  ( -0.000000000000000000, 1.000000000000000000, -0.000000000000000000 ) ) ;
#36739=LINE ( 'NONE', #33313, #729 ) ;
#36740=DIRECTION ( 'NONE',  ( -0.000000000000000000, 1.000000000000000000, -0.000000000000000000 ) ) ;
#36741=DIRECTION ( 'NONE',  ( 0.9473263538541923934, 0.000000000000000000, -0.3202698538628350744 ) ) ;
#36742=VECTOR ( 'NONE', #21681, 1000.000000000000114 ) ;
#36743=ADVANCED_FACE ( 'NONE', ( #40933 ), #8614, .T. ) ;
#36744=LINE ( 'NONE', #20708, #25084 ) ;
#36745=CARTESIAN_POINT ( 'NONE',  ( 7.403327498934737960, -175.3837268820161057, -110.6939782313521192 ) ) ;
#36750=ORIENTED_EDGE ( 'NONE', *, *, #50117, .T. ) ;
#36751=DIRECTION ( 'NONE',  ( 0.000000000000000000, 1.000000000000000000, 0.000000000000000000 ) ) ;
#36752=VERTEX_POINT ( 'NONE', #41716 ) ;
#36755=DIRECTION ( 'NONE',  ( 0.000000000000000000, 1.000000000000000000, 0.000000000000000000 ) ) ;
#36756=EDGE_CURVE ( 'NONE', #13900, #17812, #17044, .T. ) ;
#36757=DIRECTION ( 'NONE',  ( -0.000000000000000000, 1.000000000000000000, -0.000000000000000000 ) ) ;
#36758=ORIENTED_EDGE ( 'NONE', *, *, #4156, .F. ) ;
#36762=EDGE_CURVE ( 'NONE', #46453, #19312, #3244, .T. ) ;
#36765=DIRECTION ( 'NONE',  ( -0.1476465640024918202, 0.000000000000000000, 0.9890401873221624784 ) ) ;
#36766=EDGE_CURVE ( 'NONE', #48486, #30945, #36744, .T. ) ;
#36770=ORIENTED_EDGE ( 'NONE', *, *, #44513, .T. ) ;
#36774=DIRECTION ( 'NONE',  ( 0.8124868780056825335, 0.000000000000000000, -0.5829794791144703447 ) ) ;
#36775=DIRECTION ( 'NONE',  ( 0.000000000000000000, 0.000000000000000000, -1.000000000000000000 ) ) ;
#36776=DIRECTION ( 'NONE',  ( 0.000000000000000000, -1.000000000000000000, -0.000000000000000000 ) ) ;
#36777=ORIENTED_EDGE ( 'NONE', *, *, #30622, .T. ) ;
#36779=AXIS2_PLACEMENT_3D ( 'NONE', #19372, #34864, #35385 ) ;
#36780=CARTESIAN_POINT ( 'NONE',  ( -48.71401279728982558, -193.5000000000000000, -0.9720229140804069745 ) ) ;
#36781=VECTOR ( 'NONE', #22654, 1000.000000000000000 ) ;
#36782=ADVANCED_FACE ( 'NONE', ( #17302 ), #25179, .T. ) ;
#36784=DIRECTION ( 'NONE',  ( 0.000000000000000000, -1.000000000000000000, 0.000000000000000000 ) ) ;
#36785=LINE ( 'NONE', #24429, #25789 ) ;
#36787=ORIENTED_EDGE ( 'NONE', *, *, #10249, .F. ) ;
#36788=VERTEX_POINT ( 'NONE', #37770 ) ;
#36790=CYLINDRICAL_SURFACE ( 'NONE', #46099, 125.0000000000000000 ) ;
#36792=CARTESIAN_POINT ( 'NONE',  ( 20.65191334053706029, -189.7472609257535510, 102.9412430821799802 ) ) ;
#36794=ORIENTED_EDGE ( 'NONE', *, *, #51209, .F. ) ;
#36795=DIRECTION ( 'NONE',  ( 0.9960498426152171181, 0.000000000000000000, -0.08879589532293157006 ) ) ;
#36796=CARTESIAN_POINT ( 'NONE',  ( -92.43312097795266880, -189.7472609257535510, -115.9484881370935483 ) ) ;
#36797=VERTEX_POINT ( 'NONE', #37517 ) ;
#36798=AXIS2_PLACEMENT_3D ( 'NONE', #47555, #12039, #15491 ) ;
#36799=CARTESIAN_POINT ( 'NONE',  ( 74.60098876342244978, -177.1207230881787780, 21.82395850507349522 ) ) ;
#36801=EDGE_LOOP ( 'NONE', ( #45392, #16032, #2213, #42540 ) ) ;
#36802=DIRECTION ( 'NONE',  ( -0.6300878435817094392, 0.000000000000000000, -0.7765238627180437447 ) ) ;
#36806=CARTESIAN_POINT ( 'NONE',  ( -134.9506378406916838, -189.7472609257535510, 90.26448786734087548 ) ) ;
#36807=DIRECTION ( 'NONE',  ( 0.000000000000000000, -0.000000000000000000, 1.000000000000000000 ) ) ;
#36808=CARTESIAN_POINT ( 'NONE',  ( 64.44365795514079309, -189.7472609257535510, -53.60452120946192878 ) ) ;
#36809=EDGE_LOOP ( 'NONE', ( #26, #49790, #27809, #39172 ) ) ;
#36810=VECTOR ( 'NONE', #12958, 1000.000000000000000 ) ;
#36811=AXIS2_PLACEMENT_3D ( 'NONE', #6570, #18644, #23104 ) ;
#36812=DIRECTION ( 'NONE',  ( 0.4300652022765245608, 0.000000000000000000, -0.9027978299657416494 ) ) ;
#36813=ADVANCED_BREP_SHAPE_REPRESENTATION ( '', ( #35805, #31742 ), #46023 ) ;
#36814=ORIENTED_EDGE ( 'NONE', *, *, #5015, .F. ) ;
#36815=LINE ( 'NONE', #13674, #40652 ) ;
#36816=CARTESIAN_POINT ( 'NONE',  ( -126.2322430781613605, -183.6283474603465606, 97.87467957288053810 ) ) ;
#36818=EDGE_LOOP ( 'NONE', ( #14641, #21823, #39898, #42224 ) ) ;
#36822=DIRECTION ( 'NONE',  ( -0.000000000000000000, 1.000000000000000000, -0.000000000000000000 ) ) ;
#36823=ORIENTED_EDGE ( 'NONE', *, *, #3234, .F. ) ;
#36825=VECTOR ( 'NONE', #3901, 1000.000000000000000 ) ;
#36826=CARTESIAN_POINT ( 'NONE',  ( -5.113431607746562690, -189.7472609257535510, 117.2365833888819537 ) ) ;
#36828=EDGE_CURVE ( 'NONE', #9325, #21275, #44623, .T. ) ;
#36829=CARTESIAN_POINT ( 'NONE',  ( -43.48323084606168720, -183.6283474603465606, 124.9001241957026167 ) ) ;
#36830=VERTEX_POINT ( 'NONE', #9408 ) ;
#36831=LINE ( 'NONE', #17125, #48428 ) ;
#36832=DIRECTION ( 'NONE',  ( 0.000000000000000000, 1.000000000000000000, 0.000000000000000000 ) ) ;
#36833=CARTESIAN_POINT ( 'NONE',  ( -49.32472275501068282, -193.5000000000000000, 0.5338233779647895139 ) ) ;
#36836=DIRECTION ( 'NONE',  ( -0.9960498426152177842, 0.000000000000000000, 0.08879589532292482545 ) ) ;
#36838=CARTESIAN_POINT ( 'NONE',  ( -48.47912675150885065, -189.7472609257535510, 6.938893903907228378E-15 ) ) ;
#36839=ORIENTED_EDGE ( 'NONE', *, *, #46548, .F. ) ;
#36841=DIRECTION ( 'NONE',  ( -0.8124868780056825335, 0.000000000000000000, 0.5829794791144703447 ) ) ;
#36843=CARTESIAN_POINT ( 'NONE',  ( -48.47912675150885065, -189.7472609257535510, 6.938893903907228378E-15 ) ) ;
#36846=AXIS2_PLACEMENT_3D ( 'NONE', #7318, #3618, #31743 ) ;
#36848=CARTESIAN_POINT ( 'NONE',  ( -135.6699833737243353, -175.3837268820161057, 89.56983042009326823 ) ) ;
#36849=DIRECTION ( 'NONE',  ( 0.000000000000000000, -1.000000000000000000, 0.000000000000000000 ) ) ;
#36850=ORIENTED_EDGE ( 'NONE', *, *, #568, .F. ) ;
#36852=VERTEX_POINT ( 'NONE', #43167 ) ;
#36853=DIRECTION ( 'NONE',  ( 0.000000000000000000, -1.000000000000000000, 0.000000000000000000 ) ) ;
#36854=DIRECTION ( 'NONE',  ( 0.1182731709213592358, 0.000000000000000000, 0.9929810960135178055 ) ) ;
#36855=EDGE_LOOP ( 'NONE', ( #21642, #24918, #15664, #35059 ) ) ;
#36856=CIRCLE ( 'NONE', #49452, 125.0000000000000000 ) ;
#36857=VERTEX_POINT ( 'NONE', #7172 ) ;
#36858=ORIENTED_EDGE ( 'NONE', *, *, #16951, .T. ) ;
#36859=ADVANCED_FACE ( 'NONE', ( #39231 ), #48095, .T. ) ;
#36860=DIRECTION ( 'NONE',  ( 0.000000000000000000, 1.000000000000000000, 0.000000000000000000 ) ) ;
#36861=ADVANCED_FACE ( 'NONE', ( #20483 ), #1031, .T. ) ;
#36863=EDGE_CURVE ( 'NONE', #18649, #51271, #508, .T. ) ;
#36865=FACE_OUTER_BOUND ( 'NONE', #32872, .T. ) ;
#36866=ORIENTED_EDGE ( 'NONE', *, *, #18900, .F. ) ;
#36868=EDGE_CURVE ( 'NONE', #49664, #36451, #15029, .T. ) ;
#36869=AXIS2_PLACEMENT_3D ( 'NONE', #43210, #27700, #7222 ) ;
#36871=CARTESIAN_POINT ( 'NONE',  ( -163.3245969606054473, -193.5000000000000000, -46.76022031560622594 ) ) ;
#36874=DIRECTION ( 'NONE',  ( 0.000000000000000000, -1.000000000000000000, 0.000000000000000000 ) ) ;
#36876=DIRECTION ( 'NONE',  ( 0.1182731709213660498, 0.000000000000000000, -0.9929810960135169173 ) ) ;
#36881=PLANE ( 'NONE',  #47536 ) ;
#36882=ADVANCED_FACE ( 'NONE', ( #8406 ), #36253, .T. ) ;
#36883=EDGE_LOOP ( 'NONE', ( #28524, #4299, #22528, #33693 ) ) ;
#36884=ORIENTED_EDGE ( 'NONE', *, *, #33903, .T. ) ;
#36886=ADVANCED_FACE ( 'NONE', ( #48630 ), #40449, .T. ) ;
#36887=DIRECTION ( 'NONE',  ( 0.000000000000000000, 0.000000000000000000, 1.000000000000000000 ) ) ;
#36891=AXIS2_PLACEMENT_3D ( 'NONE', #41250, #42549, #30711 ) ;
#36893=CYLINDRICAL_SURFACE ( 'NONE', #13654, 125.0000000000000000 ) ;
#36894=EDGE_LOOP ( 'NONE', ( #30353, #28337, #25599, #21826 ) ) ;
#36895=CARTESIAN_POINT ( 'NONE',  ( -120.2975302769383177, -183.6283474603465606, 102.3089288139533863 ) ) ;
#36896=EDGE_CURVE ( 'NONE', #22006, #32508, #251, .T. ) ;
#36897=CYLINDRICAL_SURFACE ( 'NONE', #14681, 125.0000000000000000 ) ;
#36898=ORIENTED_EDGE ( 'NONE', *, *, #29540, .T. ) ;
#36899=DIRECTION ( 'NONE',  ( 0.000000000000000000, 0.000000000000000000, -1.000000000000000000 ) ) ;
#36901=DIRECTION ( 'NONE',  ( -0.000000000000000000, -1.000000000000000000, 0.000000000000000000 ) ) ;
#36902=ORIENTED_EDGE ( 'NONE', *, *, #29744, .F. ) ;
#36903=DIRECTION ( 'NONE',  ( -0.000000000000000000, -1.000000000000000000, 0.000000000000000000 ) ) ;
#36904=PLANE ( 'NONE',  #20494 ) ;
#36907=ADVANCED_FACE ( 'NONE', ( #44145 ), #36790, .T. ) ;
#36908=VECTOR ( 'NONE', #25425, 1000.000000000000000 ) ;
#36911=EDGE_LOOP ( 'NONE', ( #20102, #24978, #48730, #3312 ) ) ;
#36915=ORIENTED_EDGE ( 'NONE', *, *, #7964, .T. ) ;
#36916=ORIENTED_EDGE ( 'NONE', *, *, #32113, .T. ) ;
#36917=LINE ( 'NONE', #5654, #23215 ) ;
#36920=ORIENTED_EDGE ( 'NONE', *, *, #48473, .T. ) ;
#36921=VECTOR ( 'NONE', #21145, 999.9999999999998863 ) ;
#36922=CARTESIAN_POINT ( 'NONE',  ( 12.12533326292403935, -177.1207230881787780, 109.3256576763158847 ) ) ;
#36924=CARTESIAN_POINT ( 'NONE',  ( 51.05451324771861010, -183.6283474603465606, 75.61781872352699452 ) ) ;
#36927=ADVANCED_FACE ( 'NONE', ( #24965 ), #32051, .T. ) ;
#36928=ADVANCED_FACE ( 'NONE', ( #45213 ), #9199, .T. ) ;
#36930=DIRECTION ( 'NONE',  ( -0.5085311186492273983, 0.000000000000000000, 0.8610436117673514467 ) ) ;
#36931=EDGE_LOOP ( 'NONE', ( #9780, #28556, #20811, #18611 ) ) ;
#36932=ORIENTED_EDGE ( 'NONE', *, *, #28552, .F. ) ;
#36933=EDGE_CURVE ( 'NONE', #35575, #27476, #50293, .T. ) ;
#36935=DIRECTION ( 'NONE',  ( 0.9266896074318370369, 0.000000000000000000, -0.3758275821142292306 ) ) ;
#36940=EDGE_LOOP ( 'NONE', ( #22930, #10416, #34975, #15593 ) ) ;
#36943=ORIENTED_EDGE ( 'NONE', *, *, #7419, .T. ) ;
#36946=ORIENTED_EDGE ( 'NONE', *, *, #48225, .F. ) ;
#36948=CARTESIAN_POINT ( 'NONE',  ( -172.4195137048758397, -175.3837268820161057, -3.844569333772413611 ) ) ;
#36949=LINE ( 'NONE', #5160, #32512 ) ;
#36950=EDGE_CURVE ( 'NONE', #51223, #5652, #1294, .T. ) ;
#36951=LINE ( 'NONE', #32487, #24561 ) ;
#36952=DIRECTION ( 'NONE',  ( 0.000000000000000000, -1.000000000000000000, 0.000000000000000000 ) ) ;
#36953=ORIENTED_EDGE ( 'NONE', *, *, #45317, .F. ) ;
#36955=ORIENTED_EDGE ( 'NONE', *, *, #8275, .F. ) ;
#36956=EDGE_CURVE ( 'NONE', #12493, #23734, #50441, .T. ) ;
#36957=VERTEX_POINT ( 'NONE', #29933 ) ;
#36960=DIRECTION ( 'NONE',  ( -0.000000000000000000, 1.000000000000000000, -0.000000000000000000 ) ) ;
#36962=DIRECTION ( 'NONE',  ( 0.000000000000000000, -0.000000000000000000, 1.000000000000000000 ) ) ;
#36963=LINE ( 'NONE', #427, #1045 ) ;
#36964=ORIENTED_EDGE ( 'NONE', *, *, #22414, .F. ) ;
#36965=CARTESIAN_POINT ( 'NONE',  ( -145.4373324222573842, -189.7472609257535510, -78.89300572996837957 ) ) ;
#36967=LINE ( 'NONE', #28549, #6850 ) ;
#36968=FACE_BOUND ( 'NONE', #41335, .T. ) ;
#36969=ORIENTED_EDGE ( 'NONE', *, *, #51732, .F. ) ;
#36970=DIRECTION ( 'NONE',  ( -0.000000000000000000, 1.000000000000000000, -0.000000000000000000 ) ) ;
#36971=ORIENTED_EDGE ( 'NONE', *, *, #3848, .F. ) ;
#36973=ORIENTED_EDGE ( 'NONE', *, *, #40743, .T. ) ;
#36974=DIRECTION ( 'NONE',  ( -0.7575112421616284619, 0.000000000000000000, 0.6528221181905119463 ) ) ;
#36975=VERTEX_POINT ( 'NONE', #25473 ) ;
#36978=FACE_OUTER_BOUND ( 'NONE', #51420, .T. ) ;
#36981=ORIENTED_EDGE ( 'NONE', *, *, #22934, .F. ) ;
#36983=EDGE_CURVE ( 'NONE', #19289, #10180, #17353, .T. ) ;
#36984=CARTESIAN_POINT ( 'NONE',  ( -132.6364218684650211, -183.6283474603465606, 92.42591454022807795 ) ) ;
#36985=VERTEX_POINT ( 'NONE', #41230 ) ;
#36986=ORIENTED_EDGE ( 'NONE', *, *, #34838, .F. ) ;
#36987=VERTEX_POINT ( 'NONE', #37814 ) ;
#36989=LINE ( 'NONE', #13857, #23478 ) ;
#36990=VECTOR ( 'NONE', #29807, 1000.000000000000000 ) ;
#36991=ORIENTED_EDGE ( 'NONE', *, *, #17167, .T. ) ;
#36992=LINE ( 'NONE', #49083, #10813 ) ;
#36993=DIRECTION ( 'NONE',  ( 0.000000000000000000, 0.000000000000000000, -1.000000000000000000 ) ) ;
#36994=DIRECTION ( 'NONE',  ( -0.9960498426152158968, 0.000000000000000000, -0.08879589532294571153 ) ) ;
#36995=PLANE ( 'NONE',  #10810 ) ;
#36997=VERTEX_POINT ( 'NONE', #41490 ) ;
#37000=ORIENTED_EDGE ( 'NONE', *, *, #1739, .F. ) ;
#37002=ADVANCED_FACE ( 'NONE', ( #50188 ), #45457, .T. ) ;
#37003=DIRECTION ( 'NONE',  ( 0.05924062789370748011, 0.000000000000000000, 0.9982437317643217956 ) ) ;
#37004=ORIENTED_EDGE ( 'NONE', *, *, #38929, .T. ) ;
#37006=ORIENTED_EDGE ( 'NONE', *, *, #17882, .T. ) ;
#37007=CARTESIAN_POINT ( 'NONE',  ( -48.47912675150885065, -189.7472609257535510, 6.938893903907228378E-15 ) ) ;
#37009=EDGE_LOOP ( 'NONE', ( #49709, #32576, #48943, #15977 ) ) ;
#37012=ADVANCED_FACE ( 'NONE', ( #22047 ), #17853, .T. ) ;
#37013=AXIS2_PLACEMENT_3D ( 'NONE', #32299, #16285, #28362 ) ;
#37015=DIRECTION ( 'NONE',  ( 0.9473263538541876194, 0.000000000000000000, 0.3202698538628486746 ) ) ;
#37016=DIRECTION ( 'NONE',  ( 0.9027978299657477557, 0.000000000000000000, -0.4300652022765115712 ) ) ;
#37018=PLANE ( 'NONE',  #39952 ) ;
#37021=DIRECTION ( 'NONE',  ( 0.000000000000000000, 0.000000000000000000, -1.000000000000000000 ) ) ;
#37024=DIRECTION ( 'NONE',  ( 0.000000000000000000, 0.000000000000000000, 1.000000000000000000 ) ) ;
#37025=LINE ( 'NONE', #32292, #44749 ) ;
#37028=LINE ( 'NONE', #8401, #41172 ) ;
#37030=ORIENTED_EDGE ( 'NONE', *, *, #113, .F. ) ;
#37031=VERTEX_POINT ( 'NONE', #33367 ) ;
#37032=EDGE_LOOP ( 'NONE', ( #26687, #41121, #5660, #28763 ) ) ;
#37033=EDGE_CURVE ( 'NONE', #50002, #14153, #1565, .T. ) ;
#37034=CARTESIAN_POINT ( 'NONE',  ( 76.37123734610607073, -183.6283474603465606, 6.114457023561876703 ) ) ;
#37035=PLANE ( 'NONE',  #3544 ) ;
#37036=LINE ( 'NONE', #32835, #13645 ) ;
#37039=ORIENTED_EDGE ( 'NONE', *, *, #2683, .T. ) ;
#37042=CIRCLE ( 'NONE', #2647, 125.0000000000000000 ) ;
#37043=FACE_OUTER_BOUND ( 'NONE', #10710, .T. ) ;
#37044=ORIENTED_EDGE ( 'NONE', *, *, #7346, .F. ) ;
#37045=AXIS2_PLACEMENT_3D ( 'NONE', #36183, #21205, #44076 ) ;
#37047=ORIENTED_EDGE ( 'NONE', *, *, #30108, .T. ) ;
#37048=CARTESIAN_POINT ( 'NONE',  ( -58.29063029684667185, -177.1207230881787780, 124.6143426664034877 ) ) ;
#37049=ADVANCED_FACE ( 'NONE', ( #49411 ), #22301, .T. ) ;
#37050=ORIENTED_EDGE ( 'NONE', *, *, #45549, .T. ) ;
#37053=CIRCLE ( 'NONE', #27815, 125.0000000000000000 ) ;
#37057=LINE ( 'NONE', #48905, #2324 ) ;
#37060=DIRECTION ( 'NONE',  ( 0.000000000000000000, -1.000000000000000000, 0.000000000000000000 ) ) ;
#37061=ORIENTED_EDGE ( 'NONE', *, *, #9116, .T. ) ;
#37062=LINE ( 'NONE', #28910, #30575 ) ;
#37063=PLANE ( 'NONE',  #45947 ) ;
#37064=EDGE_LOOP ( 'NONE', ( #7251, #20207, #33591, #28517 ) ) ;
#37066=CARTESIAN_POINT ( 'NONE',  ( 52.75081385575904136, -189.7472609257535510, 71.61357856150601719 ) ) ;
#37067=CARTESIAN_POINT ( 'NONE',  ( -50.89116676070555911, -177.1207230881787780, 124.9767260852757147 ) ) ;
#37069=PLANE ( 'NONE',  #8093 ) ;
#37071=CARTESIAN_POINT ( 'NONE',  ( -161.4019114581580823, -175.3837268820161057, 53.60452120946281696 ) ) ;
#37072=ORIENTED_EDGE ( 'NONE', *, *, #9568, .F. ) ;
#37073=DIRECTION ( 'NONE',  ( 0.000000000000000000, 0.000000000000000000, -1.000000000000000000 ) ) ;
#37075=DIRECTION ( 'NONE',  ( 0.000000000000000000, -1.000000000000000000, 0.000000000000000000 ) ) ;
#37076=AXIS2_PLACEMENT_3D ( 'NONE', #29443, #45495, #49692 ) ;
#37077=PLANE ( 'NONE',  #20683 ) ;
#37078=ORIENTED_EDGE ( 'NONE', *, *, #7396, .F. ) ;
#37079=VECTOR ( 'NONE', #30419, 1000.000000000000114 ) ;
#37080=LINE ( 'NONE', #17130, #21259 ) ;
#37081=DIRECTION ( 'NONE',  ( 0.8858462335218260097, 0.000000000000000000, 0.4639789333096864810 ) ) ;
#37082=AXIS2_PLACEMENT_3D ( 'NONE', #45774, #26564, #30001 ) ;
#37085=LINE ( 'NONE', #29209, #40739 ) ;
#37086=LINE ( 'NONE', #12647, #46253 ) ;
#37087=LINE ( 'NONE', #41036, #20166 ) ;
#37088=EDGE_CURVE ( 'NONE', #19748, #21876, #28424, .T. ) ;
#37089=CARTESIAN_POINT ( 'NONE',  ( -49.35486169370448550, -175.3837268820161057, -0.4827922027307481878 ) ) ;
#37090=CIRCLE ( 'NONE', #50540, 125.0000000000000000 ) ;
#37093=CIRCLE ( 'NONE', #14457, 125.0000000000000000 ) ;
#37095=DIRECTION ( 'NONE',  ( -0.000000000000000000, 1.000000000000000000, -0.000000000000000000 ) ) ;
#37096=DIRECTION ( 'NONE',  ( -0.000000000000000000, 1.000000000000000000, -0.000000000000000000 ) ) ;
#37098=EDGE_LOOP ( 'NONE', ( #27568, #49235, #18, #11394 ) ) ;
#37099=ORIENTED_EDGE ( 'NONE', *, *, #12168, .F. ) ;
#37100=DIRECTION ( 'NONE',  ( 0.9151456172430153524, 0.000000000000000000, 0.4031234292879792847 ) ) ;
#37102=ADVANCED_FACE ( 'NONE', ( #18869 ), #23351, .T. ) ;
#37107=ORIENTED_EDGE ( 'NONE', *, *, #29452, .T. ) ;
#37108=ADVANCED_FACE ( 'NONE', ( #39362 ), #14957, .T. ) ;
#37109=ORIENTED_EDGE ( 'NONE', *, *, #22993, .F. ) ;
#37110=PLANE ( 'NONE',  #30889 ) ;
#37111=AXIS2_PLACEMENT_3D ( 'NONE', #49887, #33341, #28858 ) ;
#37112=CARTESIAN_POINT ( 'NONE',  ( -48.41988612361515010, -183.6283474603465606, 0.9982437317643287900 ) ) ;
#37113=CARTESIAN_POINT ( 'NONE',  ( -105.7090724259147976, -189.7472609257535510, 111.1293539894142839 ) ) ;
#37116=DIRECTION ( 'NONE',  ( -0.05924062789371441901, 0.000000000000000000, 0.9982437317643214625 ) ) ;
#37120=ORIENTED_EDGE ( 'NONE', *, *, #38093, .T. ) ;
#37122=ORIENTED_EDGE ( 'NONE', *, *, #51347, .F. ) ;
#37123=PLANE ( 'NONE',  #16549 ) ;
#37124=FACE_OUTER_BOUND ( 'NONE', #520, .T. ) ;
#37125=CARTESIAN_POINT ( 'NONE',  ( 44.30815888362531041, -189.7472609257535510, 83.75869879877569701 ) ) ;
#37126=AXIS2_PLACEMENT_3D ( 'NONE', #7391, #23415, #39170 ) ;
#37130=ORIENTED_EDGE ( 'NONE', *, *, #45143, .F. ) ;
#37132=CARTESIAN_POINT ( 'NONE',  ( 63.82222181224018698, -189.7472609257535510, 52.57768177182521896 ) ) ;
#37133=CARTESIAN_POINT ( 'NONE',  ( 68.72094416275764672, -189.7472609257535510, -40.49875167738976955 ) ) ;
#37134=ORIENTED_EDGE ( 'NONE', *, *, #10525, .F. ) ;
#37135=CARTESIAN_POINT ( 'NONE',  ( 18.82962626094778003, -193.5000000000000000, 104.1428419024404519 ) ) ;
#37136=CARTESIAN_POINT ( 'NONE',  ( -48.07600332222088468, -189.7472609257535510, 0.9151456172430280089 ) ) ;
#37142=CARTESIAN_POINT ( 'NONE',  ( -47.60339180931321579, -177.1207230881787780, 0.4827922027307559594 ) ) ;
#37143=EDGE_LOOP ( 'NONE', ( #29084, #4087, #31325, #31145 ) ) ;
#37144=DIRECTION ( 'NONE',  ( 0.000000000000000000, -0.000000000000000000, 1.000000000000000000 ) ) ;
#37145=LINE ( 'NONE', #12455, #6786 ) ;
#37146=ORIENTED_EDGE ( 'NONE', *, *, #31701, .T. ) ;
#37147=AXIS2_PLACEMENT_3D ( 'NONE', #4134, #11478, #166 ) ;
#37148=ADVANCED_FACE ( 'NONE', ( #39093 ), #30966, .T. ) ;
#37149=CARTESIAN_POINT ( 'NONE',  ( -48.47912675150885065, -183.6283474603465606, 6.938893903907228378E-15 ) ) ;
#37151=DIRECTION ( 'NONE',  ( 0.000000000000000000, 0.000000000000000000, -1.000000000000000000 ) ) ;
#37155=VECTOR ( 'NONE', #4470, 1000.000000000000114 ) ;
#37156=ORIENTED_EDGE ( 'NONE', *, *, #47689, .T. ) ;
#37157=DIRECTION ( 'NONE',  ( 0.000000000000000000, 1.000000000000000000, 0.000000000000000000 ) ) ;
#37159=ORIENTED_EDGE ( 'NONE', *, *, #46441, .T. ) ;
#37160=FACE_OUTER_BOUND ( 'NONE', #42420, .T. ) ;
#37161=CYLINDRICAL_SURFACE ( 'NONE', #51447, 125.0000000000000000 ) ;
#37163=ADVANCED_FACE ( 'NONE', ( #47010 ), #27012, .T. ) ;
#37164=EDGE_LOOP ( 'NONE', ( #23918, #39286, #48363, #33293 ) ) ;
#37171=CARTESIAN_POINT ( 'NONE',  ( 73.66680038934278230, -175.3837268820161057, -26.55884942729568365 ) ) ;
#37174=ORIENTED_EDGE ( 'NONE', *, *, #41769, .T. ) ;
#37177=ORIENTED_EDGE ( 'NONE', *, *, #15329, .F. ) ;
#37178=CYLINDRICAL_SURFACE ( 'NONE', #46815, 125.0000000000000000 ) ;
#37182=FACE_OUTER_BOUND ( 'NONE', #29238, .T. ) ;
#37183=VERTEX_POINT ( 'NONE', #35413 ) ;
#37184=EDGE_LOOP ( 'NONE', ( #33308, #16982, #50712, #29546 ) ) ;
#37185=ORIENTED_EDGE ( 'NONE', *, *, #27223, .F. ) ;
#37187=FACE_OUTER_BOUND ( 'NONE', #9332, .T. ) ;
#37189=LINE ( 'NONE', #37716, #4571 ) ;
#37191=ORIENTED_EDGE ( 'NONE', *, *, #21809, .T. ) ;
#37192=ADVANCED_FACE ( 'NONE', ( #35163 ), #38592, .T. ) ;
#37193=CIRCLE ( 'NONE', #36325, 15.00000000000000000 ) ;
#37194=EDGE_LOOP ( 'NONE', ( #19656, #14621, #12369, #29003 ) ) ;
#37195=DIRECTION ( 'NONE',  ( 0.000000000000000000, 0.000000000000000000, -1.000000000000000000 ) ) ;
#37197=EDGE_LOOP ( 'NONE', ( #45960, #20228, #35444, #22149 ) ) ;
#37198=LINE ( 'NONE', #1186, #23318 ) ;
#37199=CARTESIAN_POINT ( 'NONE',  ( -85.77912150413021664, -189.7472609257535510, -119.3051146910911768 ) ) ;
#37201=LINE ( 'NONE', #40609, #46081 ) ;
#37202=EDGE_LOOP ( 'NONE', ( #13219, #40935, #41435, #22960 ) ) ;
#37203=DIRECTION ( 'NONE',  ( 0.000000000000000000, 1.000000000000000000, -0.000000000000000000 ) ) ;
#37205=ORIENTED_EDGE ( 'NONE', *, *, #23780, .F. ) ;
#37206=EDGE_CURVE ( 'NONE', #21292, #16634, #15736, .T. ) ;
#37208=FACE_OUTER_BOUND ( 'NONE', #28747, .T. ) ;
#37211=EDGE_LOOP ( 'NONE', ( #40234, #13321, #13372, #11941 ) ) ;
#37213=ADVANCED_FACE ( 'NONE', ( #31470 ), #34641, .T. ) ;
#37214=PLANE ( 'NONE',  #23145 ) ;
#37218=ADVANCED_FACE ( 'NONE', ( #36978 ), #39859, .T. ) ;
#37219=CIRCLE ( 'NONE', #258, 125.0000000000000000 ) ;
#37222=ADVANCED_FACE ( 'NONE', ( #19914 ), #44865, .T. ) ;
#37223=DIRECTION ( 'NONE',  ( -0.000000000000000000, 1.000000000000000000, -0.000000000000000000 ) ) ;
#37224=DIRECTION ( 'NONE',  ( -0.000000000000000000, 1.000000000000000000, -0.000000000000000000 ) ) ;
#37225=EDGE_LOOP ( 'NONE', ( #4554, #41360, #44153, #29129 ) ) ;
#37227=DIRECTION ( 'NONE',  ( -0.6965510290630033685, 0.000000000000000000, 0.7175072570443249420 ) ) ;
#37228=ORIENTED_EDGE ( 'NONE', *, *, #13687, .F. ) ;
#37229=VECTOR ( 'NONE', #32235, 1000.000000000000000 ) ;
#37230=CARTESIAN_POINT ( 'NONE',  ( -111.8989814360438828, -193.5000000000000000, -107.7168604805787027 ) ) ;
#37233=EDGE_CURVE ( 'NONE', #8838, #13900, #26784, .T. ) ;
#37235=CIRCLE ( 'NONE', #25490, 125.0000000000000000 ) ;
#37237=LINE ( 'NONE', #29863, #25968 ) ;
#37241=ORIENTED_EDGE ( 'NONE', *, *, #8275, .T. ) ;
#37242=EDGE_CURVE ( 'NONE', #3706, #33563, #8593, .T. ) ;
#37243=PLANE ( 'NONE',  #10099 ) ;
#37245=ORIENTED_EDGE ( 'NONE', *, *, #21094, .T. ) ;
#37247=EDGE_CURVE ( 'NONE', #16129, #37529, #15980, .T. ) ;
#37248=EDGE_LOOP ( 'NONE', ( #14523, #34959, #21808, #51282 ) ) ;
#37249=DIRECTION ( 'NONE',  ( 0.6528221181905227155, 0.000000000000000000, -0.7575112421616191360 ) ) ;
#37250=CARTESIAN_POINT ( 'NONE',  ( -147.6585554144535593, -183.6283474603465606, 76.08180419845380982 ) ) ;
#37251=VERTEX_POINT ( 'NONE', #28310 ) ;
#37253=FACE_OUTER_BOUND ( 'NONE', #32316, .T. ) ;
#37254=ORIENTED_EDGE ( 'NONE', *, *, #20543, .F. ) ;
#37255=ADVANCED_FACE ( 'NONE', ( #11758 ), #8085, .T. ) ;
#37256=DIRECTION ( 'NONE',  ( 0.9027978299657477557, 0.000000000000000000, -0.4300652022765115712 ) ) ;
#37258=ORIENTED_EDGE ( 'NONE', *, *, #12487, .F. ) ;
#37260=CARTESIAN_POINT ( 'NONE',  ( -47.55243714407701816, -175.3837268820161057, -0.3758275821142288420 ) ) ;
#37261=ORIENTED_EDGE ( 'NONE', *, *, #25384, .T. ) ;
#37264=LINE ( 'NONE', #44899, #40694 ) ;
#37265=AXIS2_PLACEMENT_3D ( 'NONE', #40020, #16390, #4045 ) ;
#37266=ORIENTED_EDGE ( 'NONE', *, *, #8611, .T. ) ;
#37267=VECTOR ( 'NONE', #36232, 1000.000000000000000 ) ;
#37268=CARTESIAN_POINT ( 'NONE',  ( -101.9736325116273576, -193.5000000000000000, 112.9749434763330811 ) ) ;
#37270=ORIENTED_EDGE ( 'NONE', *, *, #25723, .F. ) ;
#37271=DIRECTION ( 'NONE',  ( 0.000000000000000000, -0.000000000000000000, -1.000000000000000000 ) ) ;
#37272=EDGE_LOOP ( 'NONE', ( #15197, #14719, #33880, #25826 ) ) ;
#37273=VECTOR ( 'NONE', #952, 1000.000000000000000 ) ;
#37276=CARTESIAN_POINT ( 'NONE',  ( -123.5870580700902366, -189.7472609257535510, -98.66508442481458019 ) ) ;
#37278=FACE_OUTER_BOUND ( 'NONE', #29568, .T. ) ;
#37279=VERTEX_POINT ( 'NONE', #23849 ) ;
#37280=DIRECTION ( 'NONE',  ( 0.000000000000000000, 0.000000000000000000, 1.000000000000000000 ) ) ;
#37281=EDGE_CURVE ( 'NONE', #4055, #20290, #442, .T. ) ;
#37282=ADVANCED_FACE ( 'NONE', ( #27783 ), #32519, .T. ) ;
#37285=CARTESIAN_POINT ( 'NONE',  ( 4.558749771216725755, -183.6283474603465606, -112.0852863853379233 ) ) ;
#37287=FACE_OUTER_BOUND ( 'NONE', #27804, .T. ) ;
#37288=ADVANCED_FACE ( 'NONE', ( #7820 ), #4157, .T. ) ;
#37290=VERTEX_POINT ( 'NONE', #187 ) ;
#37291=CARTESIAN_POINT ( 'NONE',  ( -52.47502265695602119, -177.1207230881787780, -124.9361149384469485 ) ) ;
#37294=ORIENTED_EDGE ( 'NONE', *, *, #51649, .T. ) ;
#37297=EDGE_CURVE ( 'NONE', #30367, #37834, #16235, .T. ) ;
#37298=DIRECTION ( 'NONE',  ( 0.000000000000000000, 0.000000000000000000, -1.000000000000000000 ) ) ;
#37299=DIRECTION ( 'NONE',  ( 0.000000000000000000, 1.000000000000000000, 0.000000000000000000 ) ) ;
#37300=CIRCLE ( 'NONE', #49084, 125.0000000000000000 ) ;
#37302=AXIS2_PLACEMENT_3D ( 'NONE', #51096, #27136, #35286 ) ;
#37306=CIRCLE ( 'NONE', #32261, 125.0000000000000000 ) ;
#37307=EDGE_CURVE ( 'NONE', #5856, #13819, #41910, .T. ) ;
#37310=CARTESIAN_POINT ( 'NONE',  ( -47.47956591500005885, -189.7472609257535510, 0.02963332782257025594 ) ) ;
#37312=CARTESIAN_POINT ( 'NONE',  ( 50.08808042611238420, -183.6283474603465606, -76.87330921200083367 ) ) ;
#37315=CARTESIAN_POINT ( 'NONE',  ( -87.28630321566649286, -183.6283474603465606, 118.8234112238818341 ) ) ;
#37317=DIRECTION ( 'NONE',  ( -0.2920567706369628924, 0.000000000000000000, -0.9564009842765264224 ) ) ;
#37321=ORIENTED_EDGE ( 'NONE', *, *, #40974, .T. ) ;
#37323=ORIENTED_EDGE ( 'NONE', *, *, #35138, .F. ) ;
#37324=CARTESIAN_POINT ( 'NONE',  ( -173.3294908491238004, -177.1207230881787780, -6.114457023560984972 ) ) ;
#37325=VERTEX_POINT ( 'NONE', #32779 ) ;
#37326=CARTESIAN_POINT ( 'NONE',  ( -70.42295845586433245, -175.3837268820161057, -123.0587999703024877 ) ) ;
#37328=DIRECTION ( 'NONE',  ( -0.000000000000000000, 1.000000000000000000, -0.000000000000000000 ) ) ;
#37330=ORIENTED_EDGE ( 'NONE', *, *, #861, .T. ) ;
#37331=DIRECTION ( 'NONE',  ( 0.000000000000000000, -0.000000000000000000, -1.000000000000000000 ) ) ;
#37335=CARTESIAN_POINT ( 'NONE',  ( -171.1451123608488274, -175.3837268820161057, 18.13990644964088972 ) ) ;
#37336=CARTESIAN_POINT ( 'NONE',  ( -47.66663987350317910, -175.3837268820161057, 0.5829794791144832233 ) ) ;
#37337=FACE_OUTER_BOUND ( 'NONE', #13587, .T. ) ;
#37339=CARTESIAN_POINT ( 'NONE',  ( -173.4724443937511467, -177.1207230881787780, 1.292495564989519785 ) ) ;
#37340=VECTOR ( 'NONE', #22284, 1000.000000000000000 ) ;
#37341=ORIENTED_EDGE ( 'NONE', *, *, #44767, .F. ) ;
#37345=AXIS2_PLACEMENT_3D ( 'NONE', #49904, #13902, #32635 ) ;
#37346=PLANE ( 'NONE',  #48955 ) ;
#37350=CIRCLE ( 'NONE', #6296, 125.0000000000000000 ) ;
#37351=CIRCLE ( 'NONE', #12157, 125.0000000000000000 ) ;
#37353=DIRECTION ( 'NONE',  ( 0.7948544414133481562, 0.000000000000000000, 0.6068001458186002006 ) ) ;
#37354=AXIS2_PLACEMENT_3D ( 'NONE', #14520, #37653, #42100 ) ;
#37356=VECTOR ( 'NONE', #50708, 1000.000000000000114 ) ;
#37357=CARTESIAN_POINT ( 'NONE',  ( -154.5708152632604993, -183.6283474603465606, 64.19309449102807719 ) ) ;
#37358=EDGE_CURVE ( 'NONE', #30881, #32314, #41432, .T. ) ;
#37361=EDGE_LOOP ( 'NONE', ( #42528, #29665, #5624, #9280 ) ) ;
#37362=ORIENTED_EDGE ( 'NONE', *, *, #17620, .F. ) ;
#37363=DIRECTION ( 'NONE',  ( 0.000000000000000000, -1.000000000000000000, 0.000000000000000000 ) ) ;
#37365=CARTESIAN_POINT ( 'NONE',  ( -12.76653800058364574, -175.3837268820161057, -119.7898618611244927 ) ) ;
#37366=VERTEX_POINT ( 'NONE', #25413 ) ;
#37368=CIRCLE ( 'NONE', #14723, 125.0000000000000000 ) ;
#37369=ORIENTED_EDGE ( 'NONE', *, *, #9225, .F. ) ;
#37370=DIRECTION ( 'NONE',  ( 0.4566292373937077542, 0.000000000000000000, 0.8896570909947499883 ) ) ;
#37373=ADVANCED_FACE ( 'NONE', ( #9388 ), #10151, .T. ) ;
#37374=CARTESIAN_POINT ( 'NONE',  ( 74.49773146996551532, -183.6283474603465606, -22.39848972532281834 ) ) ;
#37375=DIRECTION ( 'NONE',  ( -0.000000000000000000, 1.000000000000000000, -0.000000000000000000 ) ) ;
#37377=CARTESIAN_POINT ( 'NONE',  ( 75.48400724637754422, -193.5000000000000000, -16.06677968424457248 ) ) ;
#37379=ORIENTED_EDGE ( 'NONE', *, *, #1622, .T. ) ;
#37380=AXIS2_PLACEMENT_3D ( 'NONE', #38797, #2805, #51434 ) ;
#37381=AXIS2_PLACEMENT_3D ( 'NONE', #12610, #1305, #21552 ) ;
#37382=CARTESIAN_POINT ( 'NONE',  ( -47.57632892154311577, -183.6283474603465606, 0.4300652022765314997 ) ) ;
#37383=VERTEX_POINT ( 'NONE', #17275 ) ;
#37386=PLANE ( 'NONE',  #21569 ) ;
#37387=AXIS2_PLACEMENT_3D ( 'NONE', #39122, #14710, #47548 ) ;
#37388=LINE ( 'NONE', #12946, #11384 ) ;
#37390=EDGE_CURVE ( 'NONE', #28294, #29691, #22237, .T. ) ;
#37391=AXIS2_PLACEMENT_3D ( 'NONE', #48459, #23752, #35834 ) ;
#37392=EDGE_LOOP ( 'NONE', ( #28582, #31113, #7011, #5075 ) ) ;
#37393=VERTEX_POINT ( 'NONE', #25161 ) ;
#37394=DIRECTION ( 'NONE',  ( 0.000000000000000000, 0.000000000000000000, -1.000000000000000000 ) ) ;
#37395=CARTESIAN_POINT ( 'NONE',  ( 67.29303306501925874, -189.7472609257535510, 47.13604789772128356 ) ) ;
#37396=ORIENTED_EDGE ( 'NONE', *, *, #7918, .F. ) ;
#37399=EDGE_CURVE ( 'NONE', #25303, #18124, #37237, .T. ) ;
#37400=CYLINDRICAL_SURFACE ( 'NONE', #11633, 125.0000000000000000 ) ;
#37401=ADVANCED_FACE ( 'NONE', ( #21983 ), #38003, .T. ) ;
#37403=ORIENTED_EDGE ( 'NONE', *, *, #29858, .T. ) ;
#37404=DIRECTION ( 'NONE',  ( 0.000000000000000000, 1.000000000000000000, 0.000000000000000000 ) ) ;
#37405=VERTEX_POINT ( 'NONE', #45654 ) ;
#37407=CARTESIAN_POINT ( 'NONE',  ( -22.62315034598912789, -177.1207230881787780, 121.2748789083720737 ) ) ;
#37408=LINE ( 'NONE', #48732, #8564 ) ;
#37410=VECTOR ( 'NONE', #37866, 999.9999999999998863 ) ;
#37411=DIRECTION ( 'NONE',  ( 0.000000000000000000, 0.000000000000000000, -1.000000000000000000 ) ) ;
#37414=LINE ( 'NONE', #1422, #7293 ) ;
#37415=ORIENTED_EDGE ( 'NONE', *, *, #13011, .F. ) ;
#37416=DIRECTION ( 'NONE',  ( 0.000000000000000000, -0.000000000000000000, -1.000000000000000000 ) ) ;
#37418=ORIENTED_EDGE ( 'NONE', *, *, #31778, .F. ) ;
#37419=CIRCLE ( 'NONE', #50004, 125.0000000000000000 ) ;
#37420=EDGE_CURVE ( 'NONE', #43188, #42645, #41173, .T. ) ;
#37423=ORIENTED_EDGE ( 'NONE', *, *, #4534, .T. ) ;
#37425=VERTEX_POINT ( 'NONE', #17789 ) ;
#37427=AXIS2_PLACEMENT_3D ( 'NONE', #27562, #52022, #468 ) ;
#37428=CIRCLE ( 'NONE', #26509, 125.0000000000000000 ) ;
#37430=ORIENTED_EDGE ( 'NONE', *, *, #11850, .T. ) ;
#37433=DIRECTION ( 'NONE',  ( 0.000000000000000000, -1.000000000000000000, -0.000000000000000000 ) ) ;
#37435=DIRECTION ( 'NONE',  ( 0.000000000000000000, 0.000000000000000000, 1.000000000000000000 ) ) ;
#37437=VERTEX_POINT ( 'NONE', #29079 ) ;
#37441=DIRECTION ( 'NONE',  ( 0.4031234292879792847, 0.000000000000000000, -0.9151456172430153524 ) ) ;
#37442=VECTOR ( 'NONE', #39851, 1000.000000000000000 ) ;
#37443=CIRCLE ( 'NONE', #16488, 125.0000000000000000 ) ;
#37444=CIRCLE ( 'NONE', #13936, 125.0000000000000000 ) ;
#37445=FACE_OUTER_BOUND ( 'NONE', #40942, .T. ) ;
#37446=DIRECTION ( 'NONE',  ( 0.000000000000000000, -0.000000000000000000, 1.000000000000000000 ) ) ;
#37447=EDGE_LOOP ( 'NONE', ( #43680, #16578, #20191, #42038 ) ) ;
#37448=AXIS2_PLACEMENT_3D ( 'NONE', #39407, #22362, #2398 ) ;
#37449=ADVANCED_FACE ( 'NONE', ( #33808 ), #49852, .T. ) ;
#37450=EDGE_CURVE ( 'NONE', #38808, #30367, #19265, .T. ) ;
#37453=ORIENTED_EDGE ( 'NONE', *, *, #25301, .T. ) ;
#37454=FACE_OUTER_BOUND ( 'NONE', #5688, .T. ) ;
#37455=ORIENTED_EDGE ( 'NONE', *, *, #47868, .F. ) ;
#37456=CIRCLE ( 'NONE', #19007, 125.0000000000000000 ) ;
#37457=CARTESIAN_POINT ( 'NONE',  ( 1.755575411425465360, -193.5000000000000000, 114.4616734920527392 ) ) ;
#37461=CIRCLE ( 'NONE', #10644, 125.0000000000000000 ) ;
#37462=LINE ( 'NONE', #13815, #35428 ) ;
#37464=ORIENTED_EDGE ( 'NONE', *, *, #10235, .T. ) ;
#37466=PLANE ( 'NONE',  #19148 ) ;
#37467=AXIS2_PLACEMENT_3D ( 'NONE', #14629, #46432, #26960 ) ;
#37469=ADVANCED_FACE ( 'NONE', ( #1496 ), #2277, .T. ) ;
#37470=AXIS2_PLACEMENT_3D ( 'NONE', #34481, #2939, #46586 ) ;
#37474=CARTESIAN_POINT ( 'NONE',  ( -213.8817838414232426, -213.5000000000000000, -10.00000000000000000 ) ) ;
#37475=VERTEX_POINT ( 'NONE', #45148 ) ;
#37477=LINE ( 'NONE', #13828, #8873 ) ;
#37479=PLANE ( 'NONE',  #48356 ) ;
#37480=DIRECTION ( 'NONE',  ( 0.000000000000000000, -1.000000000000000000, 0.000000000000000000 ) ) ;
#37482=FACE_BOUND ( 'NONE', #15573, .T. ) ;
#37486=DIRECTION ( 'NONE',  ( 0.000000000000000000, -1.000000000000000000, 0.000000000000000000 ) ) ;
#37488=VERTEX_POINT ( 'NONE', #49070 ) ;
#37490=VERTEX_POINT ( 'NONE', #13052 ) ;
#37492=AXIS2_PLACEMENT_3D ( 'NONE', #34740, #31846, #35263 ) ;
#37494=CIRCLE ( 'NONE', #3097, 125.0000000000000000 ) ;
#37495=DIRECTION ( 'NONE',  ( 0.000000000000000000, 0.000000000000000000, -1.000000000000000000 ) ) ;
#37496=EDGE_LOOP ( 'NONE', ( #27081, #27466, #32951, #6566 ) ) ;
#37500=DIRECTION ( 'NONE',  ( 0.000000000000000000, 0.000000000000000000, -1.000000000000000000 ) ) ;
#37501=ORIENTED_EDGE ( 'NONE', *, *, #31771, .F. ) ;
#37503=EDGE_LOOP ( 'NONE', ( #7075, #25839, #25583, #36718 ) ) ;
#37504=AXIS2_PLACEMENT_3D ( 'NONE', #34422, #2620, #46517 ) ;
#37505=EDGE_CURVE ( 'NONE', #22971, #20552, #22763, .T. ) ;
#37507=LINE ( 'NONE', #49080, #10909 ) ;
#37509=CARTESIAN_POINT ( 'NONE',  ( -48.64924157374596092, -189.7472609257535510, 124.9998842437354227 ) ) ;
#37511=LINE ( 'NONE', #20974, #15464 ) ;
#37512=ORIENTED_EDGE ( 'NONE', *, *, #3057, .T. ) ;
#37513=EDGE_CURVE ( 'NONE', #28039, #28978, #11431, .T. ) ;
#37514=EDGE_CURVE ( 'NONE', #22576, #7887, #19084, .T. ) ;
#37515=EDGE_CURVE ( 'NONE', #650, #45883, #23016, .T. ) ;
#37516=ADVANCED_FACE ( 'NONE', ( #11180 ), #3038, .F. ) ;
#37517=CARTESIAN_POINT ( 'NONE',  ( 18.49541618049842384, -183.6283474603465606, 105.5434062319798016 ) ) ;
#37518=LINE ( 'NONE', #6951, #461 ) ;
#37519=ORIENTED_EDGE ( 'NONE', *, *, #29564, .F. ) ;
#37521=VERTEX_POINT ( 'NONE', #34827 ) ;
#37522=AXIS2_PLACEMENT_3D ( 'NONE', #19879, #23819, #408 ) ;
#37525=EDGE_CURVE ( 'NONE', #7546, #18880, #25152, .T. ) ;
#37526=ORIENTED_EDGE ( 'NONE', *, *, #50958, .F. ) ;
#37527=DIRECTION ( 'NONE',  ( 0.000000000000000000, 0.000000000000000000, 1.000000000000000000 ) ) ;
#37528=DIRECTION ( 'NONE',  ( 0.000000000000000000, -1.000000000000000000, 0.000000000000000000 ) ) ;
#37529=VERTEX_POINT ( 'NONE', #51161 ) ;
#37531=CARTESIAN_POINT ( 'NONE',  ( -49.32472275501067571, -175.3837268820161057, -0.5338233779647935107 ) ) ;
#37532=CARTESIAN_POINT ( 'NONE',  ( -48.13092511607445090, -175.3837268820161057, -0.9374196611341135688 ) ) ;
#37535=FACE_OUTER_BOUND ( 'NONE', #12312, .T. ) ;
#37536=ORIENTED_EDGE ( 'NONE', *, *, #394, .T. ) ;
#37540=VECTOR ( 'NONE', #19033, 1000.000000000000000 ) ;
#37542=ADVANCED_FACE ( 'NONE', ( #22516 ), #46423, .T. ) ;
#37544=PLANE ( 'NONE',  #49879 ) ;
#37545=DIRECTION ( 'NONE',  ( 0.000000000000000000, -1.000000000000000000, 0.000000000000000000 ) ) ;
#37546=ORIENTED_EDGE ( 'NONE', *, *, #16170, .T. ) ;
#37547=AXIS2_PLACEMENT_3D ( 'NONE', #22548, #22011, #38031 ) ;
#37549=DIRECTION ( 'NONE',  ( -0.000000000000000000, 1.000000000000000000, 0.000000000000000000 ) ) ;
#37550=EDGE_CURVE ( 'NONE', #28018, #14212, #18809, .T. ) ;
#37551=CARTESIAN_POINT ( 'NONE',  ( -114.9600645115007040, -177.1207230881787780, 105.8550183720738573 ) ) ;
#37553=AXIS2_PLACEMENT_3D ( 'NONE', #32903, #41055, #25049 ) ;
#37554=ORIENTED_EDGE ( 'NONE', *, *, #51138, .T. ) ;
#37555=CARTESIAN_POINT ( 'NONE',  ( -166.6807411098556031, -183.6283474603465606, 37.47770156625504256 ) ) ;
#37556=DIRECTION ( 'NONE',  ( 0.000000000000000000, 1.000000000000000000, -0.000000000000000000 ) ) ;
#37557=EDGE_CURVE ( 'NONE', #5101, #17733, #46678, .T. ) ;
#37559=CARTESIAN_POINT ( 'NONE',  ( -164.2512865680372727, -193.5000000000000000, -47.13604789772046644 ) ) ;
#37562=DIRECTION ( 'NONE',  ( 0.9995608365087942371, 0.000000000000000000, 0.02963332782256331357 ) ) ;
#37563=ORIENTED_EDGE ( 'NONE', *, *, #25655, .T. ) ;
#37565=ORIENTED_EDGE ( 'NONE', *, *, #51891, .F. ) ;
#37568=DIRECTION ( 'NONE',  ( -0.000000000000000000, 1.000000000000000000, -0.000000000000000000 ) ) ;
#37569=AXIS2_PLACEMENT_3D ( 'NONE', #10498, #13421, #29968 ) ;
#37570=DIRECTION ( 'NONE',  ( -0.000000000000000000, 1.000000000000000000, -0.000000000000000000 ) ) ;
#37573=AXIS2_PLACEMENT_3D ( 'NONE', #40583, #20630, #36665 ) ;
#37575=CARTESIAN_POINT ( 'NONE',  ( 63.31225588004632243, -183.6283474603465606, 55.92572546981597981 ) ) ;
#37576=VERTEX_POINT ( 'NONE', #26431 ) ;
#37577=LINE ( 'NONE', #33627, #24823 ) ;
#37581=EDGE_LOOP ( 'NONE', ( #30777, #8172, #28216, #51377 ) ) ;
#37582=DIRECTION ( 'NONE',  ( -0.000000000000000000, 1.000000000000000000, -0.000000000000000000 ) ) ;
#37586=EDGE_CURVE ( 'NONE', #3837, #21231, #47455, .T. ) ;
#37589=EDGE_CURVE ( 'NONE', #19021, #29776, #38571, .T. ) ;
#37590=CARTESIAN_POINT ( 'NONE',  ( 57.31108707223381060, -175.3837268820161057, -66.58401203837753712 ) ) ;
#37591=DIRECTION ( 'NONE',  ( -0.000000000000000000, 1.000000000000000000, 0.000000000000000000 ) ) ;
#37593=DIRECTION ( 'NONE',  ( 0.000000000000000000, -0.000000000000000000, -1.000000000000000000 ) ) ;
#37594=CARTESIAN_POINT ( 'NONE',  ( -238.7407812814481076, -213.5000000000000000, 41.45482488023466772 ) ) ;
#37596=CARTESIAN_POINT ( 'NONE',  ( -31.30262293407085039, -193.5000000000000000, -123.8142468240611294 ) ) ;
#37599=VERTEX_POINT ( 'NONE', #24312 ) ;
#37601=DIRECTION ( 'NONE',  ( -0.000000000000000000, 1.000000000000000000, -0.000000000000000000 ) ) ;
#37602=DIRECTION ( 'NONE',  ( -0.4566292373937200777, 0.000000000000000000, 0.8896570909947436601 ) ) ;
#37603=ORIENTED_EDGE ( 'NONE', *, *, #6699, .T. ) ;
#37604=EDGE_LOOP ( 'NONE', ( #33990, #23760, #24557, #41598 ) ) ;
#37605=PLANE ( 'NONE',  #45023 ) ;
#37607=AXIS2_PLACEMENT_3D ( 'NONE', #43546, #14654, #23566 ) ;
#37608=LINE ( 'NONE', #21052, #8078 ) ;
#37610=EDGE_LOOP ( 'NONE', ( #21908, #32804, #28907, #34638 ) ) ;
#37611=DIRECTION ( 'NONE',  ( -0.9785564922995032555, 0.000000000000000000, -0.2059786187411021818 ) ) ;
#37612=CARTESIAN_POINT ( 'NONE',  ( -48.47912675150885065, -177.1207230881787780, 6.938893903907228378E-15 ) ) ;
#37614=AXIS2_PLACEMENT_3D ( 'NONE', #8224, #8471, #4277 ) ;
#37616=ORIENTED_EDGE ( 'NONE', *, *, #15846, .T. ) ;
#37619=EDGE_CURVE ( 'NONE', #39147, #12949, #44544, .T. ) ;
#37625=CARTESIAN_POINT ( 'NONE',  ( -149.5539421794694022, -189.7472609257535510, 73.54509967498655953 ) ) ;
#37627=LINE ( 'NONE', #13968, #38855 ) ;
#37628=AXIS2_PLACEMENT_3D ( 'NONE', #20724, #16261, #24660 ) ;
#37629=CARTESIAN_POINT ( 'NONE',  ( 21.49274850782854074, -189.7472609257535510, -103.5805805771126415 ) ) ;
#37630=DIRECTION ( 'NONE',  ( 0.000000000000000000, 0.000000000000000000, 1.000000000000000000 ) ) ;
#37631=CARTESIAN_POINT ( 'NONE',  ( 75.37518750349086361, -177.1207230881787780, 6.025661128238926523 ) ) ;
#37632=ORIENTED_EDGE ( 'NONE', *, *, #44097, .T. ) ;
#37633=ORIENTED_EDGE ( 'NONE', *, *, #41356, .T. ) ;
#37635=EDGE_CURVE ( 'NONE', #29101, #34495, #42776, .T. ) ;
#37636=DIRECTION ( 'NONE',  ( -0.000000000000000000, 1.000000000000000000, -0.000000000000000000 ) ) ;
#37637=LINE ( 'NONE', #13717, #26170 ) ;
#37641=AXIS2_PLACEMENT_3D ( 'NONE', #46259, #10755, #22593 ) ;
#37642=ORIENTED_EDGE ( 'NONE', *, *, #11551, .F. ) ;
#37643=FACE_OUTER_BOUND ( 'NONE', #10966, .T. ) ;
#37644=EDGE_CURVE ( 'NONE', #49035, #1773, #20107, .T. ) ;
#37646=CARTESIAN_POINT ( 'NONE',  ( -83.89965873179625078, -189.7472609257535510, 118.8334608768482354 ) ) ;
#37647=DIRECTION ( 'NONE',  ( 0.05924062789370748011, 0.000000000000000000, 0.9982437317643217956 ) ) ;
#37648=EDGE_LOOP ( 'NONE', ( #29076, #7643, #36262, #11332 ) ) ;
#37649=DIRECTION ( 'NONE',  ( 0.000000000000000000, 0.000000000000000000, 1.000000000000000000 ) ) ;
#37650=CIRCLE ( 'NONE', #31803, 125.0000000000000000 ) ;
#37651=CYLINDRICAL_SURFACE ( 'NONE', #43436, 125.0000000000000000 ) ;
#37652=ORIENTED_EDGE ( 'NONE', *, *, #32952, .F. ) ;
#37653=DIRECTION ( 'NONE',  ( -0.000000000000000000, 1.000000000000000000, -0.000000000000000000 ) ) ;
#37655=FACE_OUTER_BOUND ( 'NONE', #26125, .T. ) ;
#37656=VERTEX_POINT ( 'NONE', #128 ) ;
#37657=DIRECTION ( 'NONE',  ( 0.000000000000000000, 1.000000000000000000, 0.000000000000000000 ) ) ;
#37658=DIRECTION ( 'NONE',  ( -0.7948544414133523750, 0.000000000000000000, -0.6068001458185945385 ) ) ;
#37659=DIRECTION ( 'NONE',  ( -0.9982437317643222396, 0.000000000000000000, 0.05924062789370006937 ) ) ;
#37660=AXIS2_PLACEMENT_3D ( 'NONE', #47239, #7792, #35917 ) ;
#37663=DIRECTION ( 'NONE',  ( -0.9266896074318317078, 0.000000000000000000, -0.3758275821142421647 ) ) ;
#37664=CARTESIAN_POINT ( 'NONE',  ( -170.7514454179067513, -177.1207230881787780, -20.63201007055403480 ) ) ;
#37665=ORIENTED_EDGE ( 'NONE', *, *, #18568, .F. ) ;
#37667=FACE_OUTER_BOUND ( 'NONE', #36410, .T. ) ;
#37670=CARTESIAN_POINT ( 'NONE',  ( -165.8930023212105596, -193.5000000000000000, -39.87457906003682950 ) ) ;
#37675=AXIS2_PLACEMENT_3D ( 'NONE', #20272, #44194, #36047 ) ;
#37676=DIRECTION ( 'NONE',  ( 0.000000000000000000, 1.000000000000000000, -0.000000000000000000 ) ) ;
#37677=AXIS2_PLACEMENT_3D ( 'NONE', #3953, #19977, #36010 ) ;
#37678=LINE ( 'NONE', #49774, #8000 ) ;
#37680=EDGE_LOOP ( 'NONE', ( #41425, #27088, #14981, #31106 ) ) ;
#37681=CIRCLE ( 'NONE', #41006, 125.0000000000000000 ) ;
#37685=EDGE_CURVE ( 'NONE', #16176, #44109, #23791, .T. ) ;
#37686=CARTESIAN_POINT ( 'NONE',  ( -213.8817838414232426, -193.5000000000000000, -10.00000000000000000 ) ) ;
#37687=ORIENTED_EDGE ( 'NONE', *, *, #45900, .F. ) ;
#37690=AXIS2_PLACEMENT_3D ( 'NONE', #29865, #13581, #29603 ) ;
#37691=DIRECTION ( 'NONE',  ( 0.000000000000000000, -1.000000000000000000, 0.000000000000000000 ) ) ;
#37692=PLANE ( 'NONE',  #16134 ) ;
#37695=CARTESIAN_POINT ( 'NONE',  ( 47.28479244271900939, -189.7472609257535510, -78.77358243914883928 ) ) ;
#37696=AXIS2_PLACEMENT_3D ( 'NONE', #34545, #50598, #46656 ) ;
#37697=EDGE_CURVE ( 'NONE', #4360, #9774, #17623, .T. ) ;
#37700=DIRECTION ( 'NONE',  ( 0.000000000000000000, 0.000000000000000000, 1.000000000000000000 ) ) ;
#37702=FACE_OUTER_BOUND ( 'NONE', #43023, .T. ) ;
#37706=CARTESIAN_POINT ( 'NONE',  ( 76.28370911321322012, -193.5000000000000000, -7.696413904697510411 ) ) ;
#37707=PLANE ( 'NONE',  #46749 ) ;
#37708=ORIENTED_EDGE ( 'NONE', *, *, #26891, .T. ) ;
#37709=ORIENTED_EDGE ( 'NONE', *, *, #9888, .F. ) ;
#37710=ORIENTED_EDGE ( 'NONE', *, *, #14268, .F. ) ;
#37712=LINE ( 'NONE', #45354, #25990 ) ;
#37715=DIRECTION ( 'NONE',  ( -0.000000000000000000, 1.000000000000000000, -0.000000000000000000 ) ) ;
#37716=CARTESIAN_POINT ( 'NONE',  ( -77.67449977936060179, -189.7472609257535510, -121.5427093402339267 ) ) ;
#37717=ORIENTED_EDGE ( 'NONE', *, *, #44513, .F. ) ;
#37718=VECTOR ( 'NONE', #9923, 1000.000000000000000 ) ;
#37719=VERTEX_POINT ( 'NONE', #12480 ) ;
#37721=ORIENTED_EDGE ( 'NONE', *, *, #9872, .F. ) ;
#37727=CARTESIAN_POINT ( 'NONE',  ( -159.5526844214375899, -183.6283474603465606, 57.33816169485221081 ) ) ;
#37728=ORIENTED_EDGE ( 'NONE', *, *, #8929, .T. ) ;
#37729=CARTESIAN_POINT ( 'NONE',  ( 50.08808042611237710, -193.5000000000000000, -76.87330921200083367 ) ) ;
#37731=VECTOR ( 'NONE', #50135, 1000.000000000000227 ) ;
#37732=VERTEX_POINT ( 'NONE', #3823 ) ;
#37733=CYLINDRICAL_SURFACE ( 'NONE', #2750, 125.0000000000000000 ) ;
#37734=DIRECTION ( 'NONE',  ( 0.000000000000000000, 0.000000000000000000, -1.000000000000000000 ) ) ;
#37736=CARTESIAN_POINT ( 'NONE',  ( -37.08895481556041318, -177.1207230881787780, 124.4799742258550310 ) ) ;
#37740=DIRECTION ( 'NONE',  ( 0.000000000000000000, -1.000000000000000000, 0.000000000000000000 ) ) ;
#37741=FACE_BOUND ( 'NONE', #45053, .T. ) ;
#37743=VECTOR ( 'NONE', #21731, 1000.000000000000000 ) ;
#37746=ADVANCED_FACE ( 'NONE', ( #19846 ), #35879, .F. ) ;
#37747=EDGE_LOOP ( 'NONE', ( #28444, #10757, #9345, #51862 ) ) ;
#37748=ADVANCED_FACE ( 'NONE', ( #40071 ), #20105, .T. ) ;
#37749=DIRECTION ( 'NONE',  ( 0.2348860457809775482, 0.000000000000000000, 0.9720229140804121926 ) ) ;
#37750=VERTEX_POINT ( 'NONE', #15661 ) ;
#37751=CARTESIAN_POINT ( 'NONE',  ( 59.00260725618640123, -177.1207230881787780, -63.81752780152988436 ) ) ;
#37753=DIRECTION ( 'NONE',  ( 0.6965510290629932655, 0.000000000000000000, 0.7175072570443347120 ) ) ;
#37754=ORIENTED_EDGE ( 'NONE', *, *, #22522, .F. ) ;
#37755=EDGE_CURVE ( 'NONE', #3016, #37183, #51932, .T. ) ;
#37757=VERTEX_POINT ( 'NONE', #38652 ) ;
#37758=VERTEX_POINT ( 'NONE', #42339 ) ;
#37762=EDGE_LOOP ( 'NONE', ( #1397, #14672, #6584, #3076 ) ) ;
#37765=EDGE_CURVE ( 'NONE', #3689, #29108, #10290, .T. ) ;
#37766=LINE ( 'NONE', #46698, #15076 ) ;
#37768=DIRECTION ( 'NONE',  ( 0.2059786187410889424, 0.000000000000000000, 0.9785564922995060311 ) ) ;
#37770=CARTESIAN_POINT ( 'NONE',  ( -165.8930023212105596, -175.3837268820161057, -39.87457906003687214 ) ) ;
#37771=PLANE ( 'NONE',  #9717 ) ;
#37773=CARTESIAN_POINT ( 'NONE',  ( -159.3947744408687868, -183.6283474603465606, -55.44293326708444880 ) ) ;
#37775=EDGE_LOOP ( 'NONE', ( #46356, #5908, #38399, #24070 ) ) ;
#37777=ORIENTED_EDGE ( 'NONE', *, *, #24305, .F. ) ;
#37780=ORIENTED_EDGE ( 'NONE', *, *, #6379, .F. ) ;
#37782=DIRECTION ( 'NONE',  ( 0.000000000000000000, 0.000000000000000000, -1.000000000000000000 ) ) ;
#37783=ORIENTED_EDGE ( 'NONE', *, *, #10514, .F. ) ;
#37784=CARTESIAN_POINT ( 'NONE',  ( 1.755575411425465360, -175.3837268820161057, 114.4616734920527392 ) ) ;
#37786=ORIENTED_EDGE ( 'NONE', *, *, #2656, .F. ) ;
#37790=CARTESIAN_POINT ( 'NONE',  ( 73.87536152799695799, -175.3837268820161057, -25.58083653558413317 ) ) ;
#37791=ORIENTED_EDGE ( 'NONE', *, *, #28771, .F. ) ;
#37793=DIRECTION ( 'NONE',  ( -0.000000000000000000, 1.000000000000000000, -0.000000000000000000 ) ) ;
#37794=DIRECTION ( 'NONE',  ( 0.000000000000000000, -0.000000000000000000, 1.000000000000000000 ) ) ;
#37795=CARTESIAN_POINT ( 'NONE',  ( 75.12566530717464275, -189.7472609257535510, 18.62405380494842433 ) ) ;
#37798=CARTESIAN_POINT ( 'NONE',  ( 73.80528149577284580, -175.3837268820161057, 25.91377046305969145 ) ) ;
#37799=AXIS2_PLACEMENT_3D ( 'NONE', #13730, #13997, #37649 ) ;
#37800=AXIS2_PLACEMENT_3D ( 'NONE', #16626, #49471, #32634 ) ;
#37801=LINE ( 'NONE', #22290, #530 ) ;
#37804=LINE ( 'NONE', #50179, #1243 ) ;
#37807=CARTESIAN_POINT ( 'NONE',  ( -136.5246168469702468, -183.6283474603465606, 87.31661597576147926 ) ) ;
#37808=ADVANCED_FACE ( 'NONE', ( #41117 ), #38403, .T. ) ;
#37809=ORIENTED_EDGE ( 'NONE', *, *, #37297, .T. ) ;
#37810=EDGE_CURVE ( 'NONE', #7741, #12493, #22641, .T. ) ;
#37811=ORIENTED_EDGE ( 'NONE', *, *, #45245, .T. ) ;
#37812=ORIENTED_EDGE ( 'NONE', *, *, #48467, .F. ) ;
#37813=EDGE_CURVE ( 'NONE', #27207, #29743, #49011, .T. ) ;
#37814=CARTESIAN_POINT ( 'NONE',  ( 22.73247662810271308, -183.6283474603465606, -101.5140743725395254 ) ) ;
#37815=AXIS2_PLACEMENT_3D ( 'NONE', #24631, #48037, #24379 ) ;
#37816=EDGE_CURVE ( 'NONE', #10170, #29823, #42804, .T. ) ;
#37818=DIRECTION ( 'NONE',  ( 0.000000000000000000, 0.000000000000000000, 1.000000000000000000 ) ) ;
#37819=EDGE_CURVE ( 'NONE', #2485, #34006, #34709, .T. ) ;
#37820=CARTESIAN_POINT ( 'NONE',  ( -170.6250538923603131, -175.3837268820161057, 26.55884942729648657 ) ) ;
#37821=EDGE_CURVE ( 'NONE', #7849, #46212, #1162, .T. ) ;
#37824=EDGE_CURVE ( 'NONE', #2312, #32293, #20903, .T. ) ;
#37827=EDGE_CURVE ( 'NONE', #6051, #14309, #33229, .T. ) ;
#37828=DIRECTION ( 'NONE',  ( 0.2348860457809842095, 0.000000000000000000, -0.9720229140804107493 ) ) ;
#37829=EDGE_CURVE ( 'NONE', #17151, #27986, #26569, .T. ) ;
#37830=ORIENTED_EDGE ( 'NONE', *, *, #32708, .F. ) ;
#37831=PLANE ( 'NONE',  #47706 ) ;
#37834=VERTEX_POINT ( 'NONE', #10043 ) ;
#37835=VECTOR ( 'NONE', #33087, 1000.000000000000000 ) ;
#37836=DIRECTION ( 'NONE',  ( -0.7378332790417189146, 0.000000000000000000, -0.6749830015182196608 ) ) ;
#37837=DIRECTION ( 'NONE',  ( -0.000000000000000000, -1.000000000000000000, 0.000000000000000000 ) ) ;
#37838=VERTEX_POINT ( 'NONE', #50760 ) ;
#37844=CARTESIAN_POINT ( 'NONE',  ( -48.47912675150885065, -175.3837268820161057, 6.938893903907228378E-15 ) ) ;
#37847=DIRECTION ( 'NONE',  ( -0.000000000000000000, 1.000000000000000000, -0.000000000000000000 ) ) ;
#37850=ORIENTED_EDGE ( 'NONE', *, *, #13204, .T. ) ;
#37852=CARTESIAN_POINT ( 'NONE',  ( -49.35486169370449971, -183.6283474603465606, 0.4827922027307437469 ) ) ;
#37853=CARTESIAN_POINT ( 'NONE',  ( -150.5816505765687907, -183.6283474603465606, 70.36529243996407956 ) ) ;
#37854=AXIS2_PLACEMENT_3D ( 'NONE', #25359, #26122, #41124 ) ;
#37856=DIRECTION ( 'NONE',  ( 0.000000000000000000, 0.000000000000000000, -1.000000000000000000 ) ) ;
#37857=DIRECTION ( 'NONE',  ( -0.000000000000000000, 1.000000000000000000, 0.000000000000000000 ) ) ;
#37859=DIRECTION ( 'NONE',  ( 0.000000000000000000, 0.000000000000000000, 1.000000000000000000 ) ) ;
#37860=ORIENTED_EDGE ( 'NONE', *, *, #11232, .T. ) ;
#37862=CARTESIAN_POINT ( 'NONE',  ( 69.88207517204678254, -175.3837268820161057, 40.19484891390058579 ) ) ;
#37864=CARTESIAN_POINT ( 'NONE',  ( 5.542374969221969039, -177.1207230881787780, 112.7238987608088365 ) ) ;
#37865=VERTEX_POINT ( 'NONE', #22121 ) ;
#37866=DIRECTION ( 'NONE',  ( -0.9646355819083614058, 0.000000000000000000, 0.2635871660690581320 ) ) ;
#37867=DIRECTION ( 'NONE',  ( 0.4639789333096864810, 0.000000000000000000, 0.8858462335218260097 ) ) ;
#37868=AXIS2_PLACEMENT_3D ( 'NONE', #20815, #28935, #29210 ) ;
#37869=EDGE_CURVE ( 'NONE', #5856, #20143, #26826, .T. ) ;
#37872=DIRECTION ( 'NONE',  ( -0.000000000000000000, 1.000000000000000000, -0.000000000000000000 ) ) ;
#37875=EDGE_CURVE ( 'NONE', #47506, #26396, #33581, .T. ) ;
#37877=FACE_OUTER_BOUND ( 'NONE', #47266, .T. ) ;
#37878=AXIS2_PLACEMENT_3D ( 'NONE', #51333, #2712, #19279 ) ;
#37879=EDGE_CURVE ( 'NONE', #22697, #51897, #42857, .T. ) ;
#37881=CARTESIAN_POINT ( 'NONE',  ( -62.43888699632653783, -193.5000000000000000, 124.2180546213279371 ) ) ;
#37882=PLANE ( 'NONE',  #37958 ) ;
#37886=ADVANCED_FACE ( 'NONE', ( #38910 ), #47598, .T. ) ;
#37887=LINE ( 'NONE', #33688, #29655 ) ;
#37888=CARTESIAN_POINT ( 'NONE',  ( -30.48891621885992365, -193.5000000000000000, -122.6885491605229959 ) ) ;
#37889=VERTEX_POINT ( 'NONE', #11306 ) ;
#37890=ORIENTED_EDGE ( 'NONE', *, *, #48074, .F. ) ;
#37893=EDGE_LOOP ( 'NONE', ( #30366, #51663, #5720, #25315 ) ) ;
#37894=DIRECTION ( 'NONE',  ( 0.000000000000000000, 1.000000000000000000, 0.000000000000000000 ) ) ;
#37896=CARTESIAN_POINT ( 'NONE',  ( 65.38692482895591240, -183.6283474603465606, -51.57055649762701677 ) ) ;
#37897=PLANE ( 'NONE',  #32177 ) ;
#37899=ADVANCED_FACE ( 'NONE', ( #32313 ), #28376, .F. ) ;
#37902=CARTESIAN_POINT ( 'NONE',  ( 70.19984492582109681, -189.7472609257535510, 39.24667733211968823 ) ) ;
#37903=ORIENTED_EDGE ( 'NONE', *, *, #22420, .F. ) ;
#37904=CARTESIAN_POINT ( 'NONE',  ( -47.48307690889363641, -183.6283474603465606, -0.08879589532292464504 ) ) ;
#37905=ORIENTED_EDGE ( 'NONE', *, *, #43337, .T. ) ;
#37906=DIRECTION ( 'NONE',  ( 0.000000000000000000, 0.000000000000000000, 1.000000000000000000 ) ) ;
#37907=CIRCLE ( 'NONE', #47964, 125.0000000000000000 ) ;
#37908=EDGE_LOOP ( 'NONE', ( #19885, #13921, #28635, #47278 ) ) ;
#37909=CARTESIAN_POINT ( 'NONE',  ( -172.7479958471414250, -183.6283474603465606, -13.49993235881364129 ) ) ;
#37910=DIRECTION ( 'NONE',  ( -0.4031234292879792847, 0.000000000000000000, 0.9151456172430153524 ) ) ;
#37911=CIRCLE ( 'NONE', #49662, 125.0000000000000000 ) ;
#37912=CARTESIAN_POINT ( 'NONE',  ( -173.3968853974275817, -175.3837268820161057, 4.533605064404172325 ) ) ;
#37913=VECTOR ( 'NONE', #46818, 1000.000000000000000 ) ;
#37914=EDGE_CURVE ( 'NONE', #33217, #49349, #8156, .T. ) ;
#37915=ORIENTED_EDGE ( 'NONE', *, *, #9534, .F. ) ;
#37918=CARTESIAN_POINT ( 'NONE',  ( 22.03849146056077757, -189.7472609257535510, 103.2098131075567409 ) ) ;
#37920=CARTESIAN_POINT ( 'NONE',  ( -131.8938452225253855, -193.5000000000000000, 93.09664195018558530 ) ) ;
#37924=CARTESIAN_POINT ( 'NONE',  ( 56.81546028627040101, -193.5000000000000000, 65.49088066501711580 ) ) ;
#37925=ORIENTED_EDGE ( 'NONE', *, *, #36716, .T. ) ;
#37926=DIRECTION ( 'NONE',  ( -0.000000000000000000, 1.000000000000000000, -0.000000000000000000 ) ) ;
#37927=ORIENTED_EDGE ( 'NONE', *, *, #10537, .F. ) ;
#37928=CIRCLE ( 'NONE', #37965, 125.0000000000000000 ) ;
#37929=VECTOR ( 'NONE', #45938, 999.9999999999998863 ) ;
#37930=LINE ( 'NONE', #1139, #11952 ) ;
#37931=DIRECTION ( 'NONE',  ( 0.7378332790417239107, 0.000000000000000000, 0.6749830015182142207 ) ) ;
#37933=VERTEX_POINT ( 'NONE', #40988 ) ;
#37935=CARTESIAN_POINT ( 'NONE',  ( -84.85683048652069260, -189.7472609257535510, 118.5439281552633446 ) ) ;
#37936=FACE_OUTER_BOUND ( 'NONE', #19393, .T. ) ;
#37937=LINE ( 'NONE', #13768, #17365 ) ;
#37939=LINE ( 'NONE', #19203, #22410 ) ;
#37944=DIRECTION ( 'NONE',  ( 0.9960498426152158968, 0.000000000000000000, 0.08879589532294571153 ) ) ;
#37945=ORIENTED_EDGE ( 'NONE', *, *, #31115, .T. ) ;
#37947=AXIS2_PLACEMENT_3D ( 'NONE', #16930, #32938, #16688 ) ;
#37952=ORIENTED_EDGE ( 'NONE', *, *, #42081, .F. ) ;
#37953=LINE ( 'NONE', #18508, #22509 ) ;
#37955=PLANE ( 'NONE',  #37854 ) ;
#37957=ORIENTED_EDGE ( 'NONE', *, *, #44534, .F. ) ;
#37958=AXIS2_PLACEMENT_3D ( 'NONE', #1882, #33928, #30003 ) ;
#37959=EDGE_LOOP ( 'NONE', ( #46477, #37109, #45571, #165 ) ) ;
#37960=AXIS2_PLACEMENT_3D ( 'NONE', #2751, #47420, #18787 ) ;
#37962=ORIENTED_EDGE ( 'NONE', *, *, #14675, .F. ) ;
#37963=PLANE ( 'NONE',  #39179 ) ;
#37964=DIRECTION ( 'NONE',  ( 0.000000000000000000, -1.000000000000000000, 0.000000000000000000 ) ) ;
#37965=AXIS2_PLACEMENT_3D ( 'NONE', #770, #25461, #15569 ) ;
#37966=AXIS2_PLACEMENT_3D ( 'NONE', #51363, #22975, #31625 ) ;
#37972=VERTEX_POINT ( 'NONE', #1303 ) ;
#37973=CYLINDRICAL_SURFACE ( 'NONE', #25818, 125.0000000000000000 ) ;
#37974=CARTESIAN_POINT ( 'NONE',  ( 50.08808042611237710, -183.6283474603465606, -76.87330921200083367 ) ) ;
#37977=CARTESIAN_POINT ( 'NONE',  ( 76.09804998693969935, -189.7472609257535510, 10.27263529369908746 ) ) ;
#37978=ORIENTED_EDGE ( 'NONE', *, *, #30753, .F. ) ;
#37979=CARTESIAN_POINT ( 'NONE',  ( -55.65514169787633847, -189.7472609257535510, -123.7921848946937331 ) ) ;
#37980=EDGE_LOOP ( 'NONE', ( #50213, #8791, #36072, #37546 ) ) ;
#37981=VECTOR ( 'NONE', #14239, 1000.000000000000000 ) ;
#37983=DIRECTION ( 'NONE',  ( 0.8124868780056783146, 0.000000000000000000, 0.5829794791144762289 ) ) ;
#37986=DIRECTION ( 'NONE',  ( 0.000000000000000000, -1.000000000000000000, 0.000000000000000000 ) ) ;
#37987=DIRECTION ( 'NONE',  ( 0.000000000000000000, -0.000000000000000000, -1.000000000000000000 ) ) ;
#37988=CARTESIAN_POINT ( 'NONE',  ( -48.47912675150885065, -189.7472609257535510, 6.938893903907228378E-15 ) ) ;
#37989=ADVANCED_FACE ( 'NONE', ( #37043 ), #24975, .T. ) ;
#37990=FACE_OUTER_BOUND ( 'NONE', #32983, .T. ) ;
#37991=CIRCLE ( 'NONE', #6130, 125.0000000000000000 ) ;
#37992=DIRECTION ( 'NONE',  ( 0.000000000000000000, 0.000000000000000000, 1.000000000000000000 ) ) ;
#37995=CIRCLE ( 'NONE', #45027, 125.0000000000000000 ) ;
#37997=PLANE ( 'NONE',  #26349 ) ;
#37998=ORIENTED_EDGE ( 'NONE', *, *, #16338, .F. ) ;
#37999=ORIENTED_EDGE ( 'NONE', *, *, #41933, .F. ) ;
#38002=ORIENTED_EDGE ( 'NONE', *, *, #35486, .T. ) ;
#38003=CYLINDRICAL_SURFACE ( 'NONE', #51163, 125.0000000000000000 ) ;
#38004=CARTESIAN_POINT ( 'NONE',  ( 60.58466639580034041, -175.3837268820161057, -61.07445476073405644 ) ) ;
#38007=ADVANCED_FACE ( 'NONE', ( #40716 ), #12870, .T. ) ;
#38008=AXIS2_PLACEMENT_3D ( 'NONE', #50866, #14088, #26683 ) ;
#38012=ORIENTED_EDGE ( 'NONE', *, *, #50589, .T. ) ;
#38013=AXIS2_PLACEMENT_3D ( 'NONE', #26114, #32960, #45594 ) ;
#38019=DIRECTION ( 'NONE',  ( 0.000000000000000000, -1.000000000000000000, 0.000000000000000000 ) ) ;
#38021=AXIS2_PLACEMENT_3D ( 'NONE', #16819, #35998, #3943 ) ;
#38023=FACE_OUTER_BOUND ( 'NONE', #6575, .T. ) ;
#38024=EDGE_LOOP ( 'NONE', ( #12518, #13755, #38238, #28304 ) ) ;
#38025=DIRECTION ( 'NONE',  ( -0.9720229140804107493, 0.000000000000000000, -0.2348860457809842095 ) ) ;
#38027=AXIS2_PLACEMENT_3D ( 'NONE', #42908, #47381, #51090 ) ;
#38029=CARTESIAN_POINT ( 'NONE',  ( -8.169009709621407822, -183.6283474603465606, 118.3219948448695504 ) ) ;
#38030=ORIENTED_EDGE ( 'NONE', *, *, #13150, .T. ) ;
#38031=DIRECTION ( 'NONE',  ( 0.000000000000000000, -0.000000000000000000, -1.000000000000000000 ) ) ;
#38032=VERTEX_POINT ( 'NONE', #28890 ) ;
#38035=VECTOR ( 'NONE', #48289, 1000.000000000000114 ) ;
#38036=LINE ( 'NONE', #5752, #21722 ) ;
#38037=VERTEX_POINT ( 'NONE', #36796 ) ;
#38038=CARTESIAN_POINT ( 'NONE',  ( 66.03142248012328253, -177.1207230881787780, 50.12318939044040889 ) ) ;
#38039=EDGE_LOOP ( 'NONE', ( #9990, #49370, #22938, #29140 ) ) ;
#38040=EDGE_CURVE ( 'NONE', #33847, #728, #49149, .T. ) ;
#38041=ORIENTED_EDGE ( 'NONE', *, *, #11714, .T. ) ;
#38044=PLANE ( 'NONE',  #4556 ) ;
#38047=LINE ( 'NONE', #42512, #12266 ) ;
#38048=LINE ( 'NONE', #35144, #28092 ) ;
#38049=DIRECTION ( 'NONE',  ( 0.000000000000000000, -1.000000000000000000, 0.000000000000000000 ) ) ;
#38051=EDGE_CURVE ( 'NONE', #21480, #13363, #10070, .T. ) ;
#38052=EDGE_LOOP ( 'NONE', ( #14918, #16670, #3749, #5583 ) ) ;
#38054=CARTESIAN_POINT ( 'NONE',  ( -173.1763543514842070, -183.6283474603465606, 8.694908215728892387 ) ) ;
#38055=EDGE_CURVE ( 'NONE', #7798, #41514, #44680, .T. ) ;
#38059=EDGE_LOOP ( 'NONE', ( #24262, #28326, #24778, #18661 ) ) ;
#38060=EDGE_CURVE ( 'NONE', #34311, #23737, #36519, .T. ) ;
#38061=DIRECTION ( 'NONE',  ( 0.000000000000000000, -1.000000000000000000, 0.000000000000000000 ) ) ;
#38062=FACE_OUTER_BOUND ( 'NONE', #50919, .T. ) ;
#38063=ORIENTED_EDGE ( 'NONE', *, *, #47787, .T. ) ;
#38064=ORIENTED_EDGE ( 'NONE', *, *, #33618, .F. ) ;
#38066=ORIENTED_EDGE ( 'NONE', *, *, #23584, .T. ) ;
#38069=LINE ( 'NONE', #6805, #10272 ) ;
#38074=ORIENTED_EDGE ( 'NONE', *, *, #35255, .T. ) ;
#38075=CARTESIAN_POINT ( 'NONE',  ( 52.59568867645217694, -189.7472609257535510, -73.54509967498590584 ) ) ;
#38077=DIRECTION ( 'NONE',  ( -0.000000000000000000, 1.000000000000000000, -0.000000000000000000 ) ) ;
#38078=VERTEX_POINT ( 'NONE', #33378 ) ;
#38079=CARTESIAN_POINT ( 'NONE',  ( -18.31235070009513421, -189.7472609257535510, 121.3052580173829966 ) ) ;
#38081=CIRCLE ( 'NONE', #4527, 125.0000000000000000 ) ;
#38084=EDGE_LOOP ( 'NONE', ( #18583, #31437, #11237, #2276 ) ) ;
#38085=DIRECTION ( 'NONE',  ( 0.000000000000000000, 0.000000000000000000, 1.000000000000000000 ) ) ;
#38086=CARTESIAN_POINT ( 'NONE',  ( -48.47912675150885065, -183.6283474603465606, 6.938893903907228378E-15 ) ) ;
#38087=VERTEX_POINT ( 'NONE', #24701 ) ;
#38089=VERTEX_POINT ( 'NONE', #26242 ) ;
#38090=DIRECTION ( 'NONE',  ( -0.000000000000000000, 1.000000000000000000, -0.000000000000000000 ) ) ;
#38091=ORIENTED_EDGE ( 'NONE', *, *, #19669, .T. ) ;
#38092=EDGE_CURVE ( 'NONE', #27177, #7546, #6034, .T. ) ;
#38093=EDGE_CURVE ( 'NONE', #4695, #12964, #22585, .T. ) ;
#38097=VERTEX_POINT ( 'NONE', #46245 ) ;
#38098=VECTOR ( 'NONE', #18705, 1000.000000000000000 ) ;
#38100=CARTESIAN_POINT ( 'NONE',  ( 73.80528149577284580, -193.5000000000000000, 25.91377046305969145 ) ) ;
#38103=DIRECTION ( 'NONE',  ( -0.000000000000000000, 1.000000000000000000, -0.000000000000000000 ) ) ;
#38105=CARTESIAN_POINT ( 'NONE',  ( -167.1580984288391107, -175.3837268820161057, -39.24667733211878584 ) ) ;
#38106=PLANE ( 'NONE',  #9043 ) ;
#38110=EDGE_CURVE ( 'NONE', #21416, #37933, #19303, .T. ) ;
#38111=PLANE ( 'NONE',  #6998 ) ;
#38113=EDGE_CURVE ( 'NONE', #30709, #5333, #15139, .T. ) ;
#38114=DIRECTION ( 'NONE',  ( 0.000000000000000000, -0.000000000000000000, -1.000000000000000000 ) ) ;
#38118=LINE ( 'NONE', #41823, #39509 ) ;
#38119=AXIS2_PLACEMENT_3D ( 'NONE', #33464, #49504, #16907 ) ;
#38122=CARTESIAN_POINT ( 'NONE',  ( -132.6364218684650211, -177.1207230881787780, 92.42591454022807795 ) ) ;
#38123=FACE_OUTER_BOUND ( 'NONE', #33215, .T. ) ;
#38124=AXIS2_PLACEMENT_3D ( 'NONE', #39782, #48488, #32173 ) ;
#38126=CARTESIAN_POINT ( 'NONE',  ( 30.67449672666758431, -183.6283474603465606, 95.45105364470144593 ) ) ;
#38127=LINE ( 'NONE', #14499, #32947 ) ;
#38130=AXIS2_PLACEMENT_3D ( 'NONE', #7779, #3845, #8307 ) ;
#38131=DIRECTION ( 'NONE',  ( 0.6965510290629982615, 0.000000000000000000, -0.7175072570443298270 ) ) ;
#38132=DIRECTION ( 'NONE',  ( 0.000000000000000000, 0.000000000000000000, 1.000000000000000000 ) ) ;
#38133=PLANE ( 'NONE',  #22846 ) ;
#38135=EDGE_LOOP ( 'NONE', ( #22663, #13099, #33034, #5810 ) ) ;
#38136=VERTEX_POINT ( 'NONE', #50194 ) ;
#38137=CARTESIAN_POINT ( 'NONE',  ( -26.37732090265851070, -193.5000000000000000, -122.0143860769387203 ) ) ;
#38138=DIRECTION ( 'NONE',  ( 0.000000000000000000, -1.000000000000000000, 0.000000000000000000 ) ) ;
#38139=LINE ( 'NONE', #38412, #22170 ) ;
#38141=ADVANCED_FACE ( 'NONE', ( #38596 ), #5527, .T. ) ;
#38143=DIRECTION ( 'NONE',  ( -0.000000000000000000, 1.000000000000000000, -0.000000000000000000 ) ) ;
#38144=DIRECTION ( 'NONE',  ( -0.9960498426152158968, 0.000000000000000000, -0.08879589532294571153 ) ) ;
#38145=DIRECTION ( 'NONE',  ( 0.000000000000000000, 0.000000000000000000, -1.000000000000000000 ) ) ;
#38148=AXIS2_PLACEMENT_3D ( 'NONE', #46842, #3206, #15288 ) ;
#38149=VERTEX_POINT ( 'NONE', #38336 ) ;
#38150=CARTESIAN_POINT ( 'NONE',  ( -81.70897914701302511, -183.6283474603465606, -120.5021863277716676 ) ) ;
#38151=ORIENTED_EDGE ( 'NONE', *, *, #22408, .T. ) ;
#38152=AXIS2_PLACEMENT_3D ( 'NONE', #12585, #40429, #43862 ) ;
#38153=EDGE_CURVE ( 'NONE', #9556, #49683, #41777, .T. ) ;
#38156=DIRECTION ( 'NONE',  ( 0.000000000000000000, 1.000000000000000000, 0.000000000000000000 ) ) ;
#38159=AXIS2_PLACEMENT_3D ( 'NONE', #12126, #39718, #43685 ) ;
#38160=ADVANCED_FACE ( 'NONE', ( #42537 ), #22308, .F. ) ;
#38163=LINE ( 'NONE', #14533, #38456 ) ;
#38164=ORIENTED_EDGE ( 'NONE', *, *, #10466, .T. ) ;
#38166=CARTESIAN_POINT ( 'NONE',  ( 12.12533326292402514, -183.6283474603465606, 109.3256576763158847 ) ) ;
#38167=ORIENTED_EDGE ( 'NONE', *, *, #19315, .T. ) ;
#38170=VECTOR ( 'NONE', #2433, 1000.000000000000114 ) ;
#38171=CARTESIAN_POINT ( 'NONE',  ( -170.5806857741408180, -183.6283474603465606, -21.61797988633148648 ) ) ;
#38172=ADVANCED_FACE ( 'NONE', ( #21807 ), #17858, .F. ) ;
#38174=VERTEX_POINT ( 'NONE', #6559 ) ;
#38175=CARTESIAN_POINT ( 'NONE',  ( -134.7293151056888973, -175.3837268820161057, -89.08931047202572984 ) ) ;
#38177=EDGE_CURVE ( 'NONE', #6993, #31627, #31922, .T. ) ;
#38178=DIRECTION ( 'NONE',  ( -0.000000000000000000, 1.000000000000000000, -0.000000000000000000 ) ) ;
#38180=VERTEX_POINT ( 'NONE', #45464 ) ;
#38182=CARTESIAN_POINT ( 'NONE',  ( -126.2322430781613889, -183.6283474603465606, 97.87467957288052389 ) ) ;
#38183=CARTESIAN_POINT ( 'NONE',  ( -150.1390659022305840, -189.7472609257535510, 72.73415134496008250 ) ) ;
#38184=DIRECTION ( 'NONE',  ( -0.000000000000000000, 1.000000000000000000, -0.000000000000000000 ) ) ;
#38185=ADVANCED_FACE ( 'NONE', ( #15208 ), #26768, .F. ) ;
#38187=DIRECTION ( 'NONE',  ( -0.000000000000000000, 1.000000000000000000, -0.000000000000000000 ) ) ;
#38188=ORIENTED_EDGE ( 'NONE', *, *, #48940, .T. ) ;
#38190=LINE ( 'NONE', #9383, #21937 ) ;
#38192=DIRECTION ( 'NONE',  ( -0.000000000000000000, 1.000000000000000000, -0.000000000000000000 ) ) ;
#38196=ORIENTED_EDGE ( 'NONE', *, *, #30478, .F. ) ;
#38197=CARTESIAN_POINT ( 'NONE',  ( -156.2577088867455473, -193.5000000000000000, -63.31490529818420754 ) ) ;
#38198=EDGE_CURVE ( 'NONE', #4562, #3, #23852, .T. ) ;
#38199=AXIS2_PLACEMENT_3D ( 'NONE', #13572, #29339, #33801 ) ;
#38202=CARTESIAN_POINT ( 'NONE',  ( -47.60339180931321579, -183.6283474603465606, 0.4827922027307559594 ) ) ;
#38204=VERTEX_POINT ( 'NONE', #31222 ) ;
#38206=CARTESIAN_POINT ( 'NONE',  ( -47.66663987350317200, -189.7472609257535510, -0.5829794791144634614 ) ) ;
#38207=CIRCLE ( 'NONE', #14699, 125.0000000000000000 ) ;
#38208=DIRECTION ( 'NONE',  ( 0.000000000000000000, 1.000000000000000000, 0.000000000000000000 ) ) ;
#38209=AXIS2_PLACEMENT_3D ( 'NONE', #19236, #35243, #51294 ) ;
#38210=CARTESIAN_POINT ( 'NONE',  ( 39.18328161278952138, -175.3837268820161057, 89.10837311819237527 ) ) ;
#38211=ORIENTED_EDGE ( 'NONE', *, *, #13327, .F. ) ;
#38213=ORIENTED_EDGE ( 'NONE', *, *, #24342, .F. ) ;
#38214=CIRCLE ( 'NONE', #21545, 125.0000000000000000 ) ;
#38215=DIRECTION ( 'NONE',  ( 0.000000000000000000, 1.000000000000000000, -0.000000000000000000 ) ) ;
#38216=LINE ( 'NONE', #22716, #9264 ) ;
#38219=ORIENTED_EDGE ( 'NONE', *, *, #2099, .T. ) ;
#38220=ADVANCED_FACE ( 'NONE', ( #42799 ), #18879, .T. ) ;
#38223=EDGE_CURVE ( 'NONE', #44250, #16764, #10744, .T. ) ;
#38225=EDGE_LOOP ( 'NONE', ( #51610, #33900, #43584, #30455 ) ) ;
#38227=ORIENTED_EDGE ( 'NONE', *, *, #32422, .T. ) ;
#38228=VECTOR ( 'NONE', #49463, 1000.000000000000227 ) ;
#38229=CARTESIAN_POINT ( 'NONE',  ( -45.06671089634843952, -177.1207230881787780, -124.9534129907280402 ) ) ;
#38230=LINE ( 'NONE', #46652, #17421 ) ;
#38231=AXIS2_PLACEMENT_3D ( 'NONE', #6136, #17705, #29762 ) ;
#38235=ORIENTED_EDGE ( 'NONE', *, *, #14542, .F. ) ;
#38236=DIRECTION ( 'NONE',  ( 0.000000000000000000, 0.000000000000000000, -1.000000000000000000 ) ) ;
#38237=VERTEX_POINT ( 'NONE', #30969 ) ;
#38238=ORIENTED_EDGE ( 'NONE', *, *, #30513, .F. ) ;
#38239=PLANE ( 'NONE',  #17027 ) ;
#38240=EDGE_CURVE ( 'NONE', #34311, #18605, #48707, .T. ) ;
#38242=CARTESIAN_POINT ( 'NONE',  ( -55.05561436132770581, -189.7472609257535510, 124.8268793598474105 ) ) ;
#38244=VECTOR ( 'NONE', #38245, 1000.000000000000114 ) ;
#38245=DIRECTION ( 'NONE',  ( -0.5085311186492094127, 0.000000000000000000, -0.8610436117673619938 ) ) ;
#38250=EDGE_CURVE ( 'NONE', #27224, #51897, #12602, .T. ) ;
#38251=FACE_OUTER_BOUND ( 'NONE', #28387, .T. ) ;
#38252=AXIS2_PLACEMENT_3D ( 'NONE', #39511, #16393, #31632 ) ;
#38253=ORIENTED_EDGE ( 'NONE', *, *, #12827, .F. ) ;
#38254=DIRECTION ( 'NONE',  ( -0.000000000000000000, 1.000000000000000000, -0.000000000000000000 ) ) ;
#38256=ORIENTED_EDGE ( 'NONE', *, *, #25017, .F. ) ;
#38258=ORIENTED_EDGE ( 'NONE', *, *, #27828, .F. ) ;
#38261=VECTOR ( 'NONE', #50420, 1000.000000000000000 ) ;
#38263=DIRECTION ( 'NONE',  ( 0.000000000000000000, -1.000000000000000000, 0.000000000000000000 ) ) ;
#38265=PLANE ( 'NONE',  #39221 ) ;
#38266=CIRCLE ( 'NONE', #45008, 125.0000000000000000 ) ;
#38267=AXIS2_PLACEMENT_3D ( 'NONE', #36780, #24682, #36001 ) ;
#38268=DIRECTION ( 'NONE',  ( 0.4827922027307490205, 0.000000000000000000, -0.8757349421956345248 ) ) ;
#38269=DIRECTION ( 'NONE',  ( -0.4031234292879792847, 0.000000000000000000, 0.9151456172430153524 ) ) ;
#38270=EDGE_LOOP ( 'NONE', ( #2797, #19579, #35734, #13924 ) ) ;
#38271=ORIENTED_EDGE ( 'NONE', *, *, #11888, .T. ) ;
#38273=CARTESIAN_POINT ( 'NONE',  ( -7.223120065443615623, -177.1207230881787780, 117.9955164924470523 ) ) ;
#38274=DIRECTION ( 'NONE',  ( 0.000000000000000000, -1.000000000000000000, -0.000000000000000000 ) ) ;
#38276=FILL_AREA_STYLE ('',( #6234 ) ) ;
#38277=AXIS2_PLACEMENT_3D ( 'NONE', #9826, #42389, #22434 ) ;
#38278=CARTESIAN_POINT ( 'NONE',  ( -165.8930023212105596, -189.7472609257535510, -39.87457906003690766 ) ) ;
#38281=ORIENTED_EDGE ( 'NONE', *, *, #13687, .T. ) ;
#38282=EDGE_CURVE ( 'NONE', #25951, #51005, #41975, .T. ) ;
#38285=FACE_OUTER_BOUND ( 'NONE', #7913, .T. ) ;
#38286=VERTEX_POINT ( 'NONE', #39609 ) ;
#38287=CARTESIAN_POINT ( 'NONE',  ( -48.47912675150885065, -183.6283474603465606, 6.938893903907228378E-15 ) ) ;
#38288=VERTEX_POINT ( 'NONE', #43056 ) ;
#38289=ORIENTED_EDGE ( 'NONE', *, *, #28231, .T. ) ;
#38290=DIRECTION ( 'NONE',  ( 0.000000000000000000, -0.000000000000000000, 1.000000000000000000 ) ) ;
#38292=PLANE ( 'NONE',  #37547 ) ;
#38293=ORIENTED_EDGE ( 'NONE', *, *, #37513, .F. ) ;
#38295=CARTESIAN_POINT ( 'NONE',  ( -47.60339180931321579, -193.5000000000000000, -0.4827922027307358088 ) ) ;
#38296=ORIENTED_EDGE ( 'NONE', *, *, #11614, .F. ) ;
#38297=FACE_OUTER_BOUND ( 'NONE', #3651, .T. ) ;
#38298=ORIENTED_EDGE ( 'NONE', *, *, #19282, .F. ) ;
#38301=CARTESIAN_POINT ( 'NONE',  ( 70.98542830588607444, -183.6283474603465606, -36.78613984829962646 ) ) ;
#38302=AXIS2_PLACEMENT_3D ( 'NONE', #39349, #36178, #51206 ) ;
#38304=CIRCLE ( 'NONE', #49239, 125.0000000000000000 ) ;
#38305=EDGE_CURVE ( 'NONE', #48694, #16051, #3622, .T. ) ;
#38306=DIRECTION ( 'NONE',  ( -0.9473263538541946138, 0.000000000000000000, 0.3202698538628279690 ) ) ;
#38307=DIRECTION ( 'NONE',  ( 0.000000000000000000, 0.000000000000000000, 1.000000000000000000 ) ) ;
#38309=DIRECTION ( 'NONE',  ( 1.000000000000000000, 0.000000000000000000, -0.000000000000000000 ) ) ;
#38310=LINE ( 'NONE', #50421, #5472 ) ;
#38311=VECTOR ( 'NONE', #42490, 1000.000000000000000 ) ;
#38316=CARTESIAN_POINT ( 'NONE',  ( -160.9694636715425702, -193.5000000000000000, 54.50618404931040573 ) ) ;
#38317=LINE ( 'NONE', #18097, #35787 ) ;
#38320=AXIS2_PLACEMENT_3D ( 'NONE', #7775, #3838, #7527 ) ;
#38321=AXIS2_PLACEMENT_3D ( 'NONE', #23888, #36234, #32561 ) ;
#38323=AXIS2_PLACEMENT_3D ( 'NONE', #16910, #8238, #31891 ) ;
#38324=VECTOR ( 'NONE', #46726, 1000.000000000000000 ) ;
#38326=VERTEX_POINT ( 'NONE', #35680 ) ;
#38327=CARTESIAN_POINT ( 'NONE',  ( -48.53836737940257251, -193.5000000000000000, 0.9982437317643279018 ) ) ;
#38330=ORIENTED_EDGE ( 'NONE', *, *, #5070, .F. ) ;
#38331=VECTOR ( 'NONE', #35768, 1000.000000000000000 ) ;
#38333=DIRECTION ( 'NONE',  ( 0.1768902751225733261, 0.000000000000000000, -0.9842305779475966077 ) ) ;
#38334=CARTESIAN_POINT ( 'NONE',  ( 75.21854001195777073, -183.6283474603465606, -8.665274887905439982 ) ) ;
#38336=CARTESIAN_POINT ( 'NONE',  ( -159.8192355313504720, -177.1207230881787780, -56.81883646197830018 ) ) ;
#38338=CARTESIAN_POINT ( 'NONE',  ( 59.70893145360469845, -193.5000000000000000, -60.59166255800332124 ) ) ;
#38340=ORIENTED_EDGE ( 'NONE', *, *, #51713, .T. ) ;
#38342=VECTOR ( 'NONE', #5116, 1000.000000000000227 ) ;
#38345=CARTESIAN_POINT ( 'NONE',  ( 44.30815888362531041, -193.5000000000000000, 83.75869879877569701 ) ) ;
#38346=VECTOR ( 'NONE', #39727, 1000.000000000000114 ) ;
#38347=ADVANCED_FACE ( 'NONE', ( #7326 ), #3113, .T. ) ;
#38349=DIRECTION ( 'NONE',  ( 0.3482016354343928088, 0.000000000000000000, 0.9374196611341231167 ) ) ;
#38350=EDGE_LOOP ( 'NONE', ( #10447, #35325, #36215, #4210 ) ) ;
#38352=DIRECTION ( 'NONE',  ( 0.000000000000000000, 1.000000000000000000, -0.000000000000000000 ) ) ;
#38354=VECTOR ( 'NONE', #50578, 1000.000000000000000 ) ;
#38356=VECTOR ( 'NONE', #33707, 1000.000000000000114 ) ;
#38357=CARTESIAN_POINT ( 'NONE',  ( 59.29945538372744807, -193.5000000000000000, 63.31490529818492519 ) ) ;
#38358=CIRCLE ( 'NONE', #23261, 125.0000000000000000 ) ;
#38359=ORIENTED_EDGE ( 'NONE', *, *, #46613, .T. ) ;
#38360=CARTESIAN_POINT ( 'NONE',  ( -154.2693405752510500, -175.3837268820161057, 66.58401203837831872 ) ) ;
#38361=EDGE_LOOP ( 'NONE', ( #6949, #50090, #50017, #41970 ) ) ;
#38363=CARTESIAN_POINT ( 'NONE',  ( 67.29469129333651267, -193.5000000000000000, -44.41421852208627286 ) ) ;
#38365=FACE_OUTER_BOUND ( 'NONE', #38361, .T. ) ;
#38366=EDGE_LOOP ( 'NONE', ( #38537, #34856, #1896, #46059 ) ) ;
#38369=CARTESIAN_POINT ( 'NONE',  ( -144.6608085595393902, -175.3837268820161057, -78.26291788638665992 ) ) ;
#38372=CARTESIAN_POINT ( 'NONE',  ( -52.47502265695602119, -193.5000000000000000, -123.9361149384469485 ) ) ;
#38374=EDGE_CURVE ( 'NONE', #15492, #37383, #47275, .T. ) ;
#38376=DIRECTION ( 'NONE',  ( -0.000000000000000000, 1.000000000000000000, -0.000000000000000000 ) ) ;
#38377=DIRECTION ( 'NONE',  ( 0.6300878435817038881, 0.000000000000000000, 0.7765238627180482966 ) ) ;
#38379=FACE_OUTER_BOUND ( 'NONE', #1943, .T. ) ;
#38380=VERTEX_POINT ( 'NONE', #20428 ) ;
#38382=PLANE ( 'NONE',  #11187 ) ;
#38384=DIRECTION ( 'NONE',  ( 0.000000000000000000, -1.000000000000000000, 0.000000000000000000 ) ) ;
#38385=EDGE_LOOP ( 'NONE', ( #50283, #19636, #51562, #49806 ) ) ;
#38386=AXIS2_PLACEMENT_3D ( 'NONE', #40877, #4900, #12750 ) ;
#38387=VECTOR ( 'NONE', #37872, 1000.000000000000000 ) ;
#38390=VECTOR ( 'NONE', #40323, 1000.000000000000000 ) ;
#38391=DIRECTION ( 'NONE',  ( -0.000000000000000000, 1.000000000000000000, -0.000000000000000000 ) ) ;
#38392=DIRECTION ( 'NONE',  ( -0.000000000000000000, 1.000000000000000000, -0.000000000000000000 ) ) ;
#38394=CARTESIAN_POINT ( 'NONE',  ( 43.18784210722336070, -189.7472609257535510, -84.98333260264753619 ) ) ;
#38395=AXIS2_PLACEMENT_3D ( 'NONE', #7255, #10680, #50124 ) ;
#38398=DIRECTION ( 'NONE',  ( -0.4566292373937140270, 0.000000000000000000, 0.8896570909947467687 ) ) ;
#38399=ORIENTED_EDGE ( 'NONE', *, *, #31335, .F. ) ;
#38400=EDGE_CURVE ( 'NONE', #30050, #38380, #40644, .T. ) ;
#38402=AXIS2_PLACEMENT_3D ( 'NONE', #21845, #38376, #5831 ) ;
#38403=CYLINDRICAL_SURFACE ( 'NONE', #1698, 125.0000000000000000 ) ;
#38404=VECTOR ( 'NONE', #36529, 1000.000000000000000 ) ;
#38408=ORIENTED_EDGE ( 'NONE', *, *, #51229, .F. ) ;
#38409=PLANE ( 'NONE',  #18335 ) ;
#38410=EDGE_CURVE ( 'NONE', #41514, #21292, #33619, .T. ) ;
#38411=DIRECTION ( 'NONE',  ( 0.4300652022765115712, 0.000000000000000000, 0.9027978299657477557 ) ) ;
#38412=CARTESIAN_POINT ( 'NONE',  ( -148.6149069237406195, -193.5000000000000000, -74.81861753132355375 ) ) ;
#38415=PLANE ( 'NONE',  #20834 ) ;
#38417=LINE ( 'NONE', #50000, #36144 ) ;
#38418=AXIS2_PLACEMENT_3D ( 'NONE', #11145, #22487, #3278 ) ;
#38419=CARTESIAN_POINT ( 'NONE',  ( 69.88207517204678254, -193.5000000000000000, 40.19484891390058579 ) ) ;
#38421=EDGE_LOOP ( 'NONE', ( #20614, #17755, #12697, #7130 ) ) ;
#38422=CIRCLE ( 'NONE', #15790, 125.0000000000000000 ) ;
#38424=LINE ( 'NONE', #34228, #11305 ) ;
#38425=ORIENTED_EDGE ( 'NONE', *, *, #36090, .F. ) ;
#38426=DIRECTION ( 'NONE',  ( 0.000000000000000000, 0.000000000000000000, 1.000000000000000000 ) ) ;
#38427=VECTOR ( 'NONE', #18509, 1000.000000000000000 ) ;
#38428=EDGE_CURVE ( 'NONE', #14578, #16046, #36450, .T. ) ;
#38429=ORIENTED_EDGE ( 'NONE', *, *, #38055, .T. ) ;
#38430=FACE_OUTER_BOUND ( 'NONE', #41399, .T. ) ;
#38431=DIRECTION ( 'NONE',  ( -0.000000000000000000, 1.000000000000000000, -0.000000000000000000 ) ) ;
#38432=PLANE ( 'NONE',  #23225 ) ;
#38433=AXIS2_PLACEMENT_3D ( 'NONE', #1166, #37433, #13784 ) ;
#38434=VERTEX_POINT ( 'NONE', #44367 ) ;
#38435=LINE ( 'NONE', #31058, #23972 ) ;
#38436=CARTESIAN_POINT ( 'NONE',  ( -11.47118876952528765, -175.3837268820161057, 118.3487137068149053 ) ) ;
#38440=ORIENTED_EDGE ( 'NONE', *, *, #27890, .F. ) ;
#38442=CARTESIAN_POINT ( 'NONE',  ( 45.66222513722992460, -177.1207230881787780, 80.70646587903453906 ) ) ;
#38443=AXIS2_PLACEMENT_3D ( 'NONE', #42045, #5820, #46017 ) ;
#38444=EDGE_LOOP ( 'NONE', ( #37721, #43393, #16379, #41404 ) ) ;
#38445=DIRECTION ( 'NONE',  ( 0.000000000000000000, 0.000000000000000000, 1.000000000000000000 ) ) ;
#38447=DIRECTION ( 'NONE',  ( 0.000000000000000000, 0.000000000000000000, 1.000000000000000000 ) ) ;
#38449=ORIENTED_EDGE ( 'NONE', *, *, #34946, .F. ) ;
#38451=DIRECTION ( 'NONE',  ( 0.000000000000000000, 1.000000000000000000, 0.000000000000000000 ) ) ;
#38453=VERTEX_POINT ( 'NONE', #36984 ) ;
#38454=CARTESIAN_POINT ( 'NONE',  ( -102.5006284722404502, -193.5000000000000000, -112.7238987608084386 ) ) ;
#38456=VECTOR ( 'NONE', #31060, 1000.000000000000000 ) ;
#38457=AXIS2_PLACEMENT_3D ( 'NONE', #16744, #944, #31717 ) ;
#38464=EDGE_CURVE ( 'NONE', #45486, #34708, #5080, .T. ) ;
#38465=VERTEX_POINT ( 'NONE', #8355 ) ;
#38466=EDGE_CURVE ( 'NONE', #46293, #4438, #32523, .T. ) ;
#38467=ADVANCED_FACE ( 'NONE', ( #193 ), #9140, .T. ) ;
#38468=CARTESIAN_POINT ( 'NONE',  ( -47.49008656418669005, -183.6283474603465606, -0.1476465640024710591 ) ) ;
#38469=EDGE_CURVE ( 'NONE', #38948, #6177, #51999, .T. ) ;
#38471=AXIS2_PLACEMENT_3D ( 'NONE', #14967, #22590, #47537 ) ;
#38473=CARTESIAN_POINT ( 'NONE',  ( -99.62791064391784346, -189.7472609257535510, -114.0561348912352173 ) ) ;
#38475=EDGE_LOOP ( 'NONE', ( #6487, #17536, #4885, #39139 ) ) ;
#38480=DIRECTION ( 'NONE',  ( -0.4300652022765304450, 0.000000000000000000, 0.9027978299657387629 ) ) ;
#38484=EDGE_CURVE ( 'NONE', #18044, #33115, #51265, .T. ) ;
#38485=EDGE_LOOP ( 'NONE', ( #6399, #33362, #10860, #30516 ) ) ;
#38486=AXIS2_PLACEMENT_3D ( 'NONE', #47815, #50987, #2873 ) ;
#38490=PLANE ( 'NONE',  #25369 ) ;
#38492=ORIENTED_EDGE ( 'NONE', *, *, #26836, .F. ) ;
#38493=EDGE_CURVE ( 'NONE', #40406, #9307, #976, .T. ) ;
#38495=LINE ( 'NONE', #32150, #40793 ) ;
#38498=ORIENTED_EDGE ( 'NONE', *, *, #9284, .F. ) ;
#38500=AXIS2_PLACEMENT_3D ( 'NONE', #19319, #35330, #43488 ) ;
#38502=PLANE ( 'NONE',  #40925 ) ;
#38503=LINE ( 'NONE', #33530, #22475 ) ;
#38506=FACE_OUTER_BOUND ( 'NONE', #6216, .T. ) ;
#38508=CARTESIAN_POINT ( 'NONE',  ( -59.86929868745821182, -193.5000000000000000, -124.4799742258549600 ) ) ;
#38511=PLANE ( 'NONE',  #38008 ) ;
#38512=AXIS2_PLACEMENT_3D ( 'NONE', #17799, #25934, #41710 ) ;
#38513=DIRECTION ( 'NONE',  ( 0.000000000000000000, 0.000000000000000000, 1.000000000000000000 ) ) ;
#38515=LINE ( 'NONE', #10657, #13119 ) ;
#38517=PLANE ( 'NONE',  #7238 ) ;
#38518=DIRECTION ( 'NONE',  ( 0.000000000000000000, 0.000000000000000000, -1.000000000000000000 ) ) ;
#38519=CIRCLE ( 'NONE', #48584, 125.0000000000000000 ) ;
#38522=ORIENTED_EDGE ( 'NONE', *, *, #29205, .T. ) ;
#38524=ORIENTED_EDGE ( 'NONE', *, *, #38040, .T. ) ;
#38526=ORIENTED_EDGE ( 'NONE', *, *, #10421, .T. ) ;
#38527=ADVANCED_FACE ( 'NONE', ( #45403 ), #33564, .T. ) ;
#38528=LINE ( 'NONE', #18557, #40538 ) ;
#38529=EDGE_CURVE ( 'NONE', #51567, #30637, #29870, .T. ) ;
#38531=EDGE_CURVE ( 'NONE', #138, #26111, #14121, .T. ) ;
#38532=DIRECTION ( 'NONE',  ( 0.7378332790417333475, 0.000000000000000000, -0.6749830015182038956 ) ) ;
#38533=ORIENTED_EDGE ( 'NONE', *, *, #29837, .F. ) ;
#38534=AXIS2_PLACEMENT_3D ( 'NONE', #16041, #49657, #9449 ) ;
#38535=CYLINDRICAL_SURFACE ( 'NONE', #42719, 125.0000000000000000 ) ;
#38536=CARTESIAN_POINT ( 'NONE',  ( -44.48323084606168720, -193.5000000000000000, 124.9361149384469769 ) ) ;
#38537=ORIENTED_EDGE ( 'NONE', *, *, #48165, .F. ) ;
#38538=CARTESIAN_POINT ( 'NONE',  ( -124.4642912599203584, -189.7472609257535510, 99.25348746834863789 ) ) ;
#38541=DIRECTION ( 'NONE',  ( 0.000000000000000000, -1.000000000000000000, 0.000000000000000000 ) ) ;
#38542=ORIENTED_EDGE ( 'NONE', *, *, #3446, .T. ) ;
#38543=ORIENTED_EDGE ( 'NONE', *, *, #245, .F. ) ;
#38544=ORIENTED_EDGE ( 'NONE', *, *, #32751, .T. ) ;
#38546=CARTESIAN_POINT ( 'NONE',  ( -50.89116676070551648, -183.6283474603465606, 124.9767260852757147 ) ) ;
#38547=ADVANCED_FACE ( 'NONE', ( #30135 ), #42473, .T. ) ;
#38548=CARTESIAN_POINT ( 'NONE',  ( -114.4014177456970458, -193.5000000000000000, 105.0256126866236457 ) ) ;
#38549=CARTESIAN_POINT ( 'NONE',  ( -8.721998590732194856, -177.1207230881787780, -118.5089480183145270 ) ) ;
#38552=EDGE_CURVE ( 'NONE', #43478, #12206, #40311, .T. ) ;
#38553=EDGE_CURVE ( 'NONE', #19199, #30881, #5946, .T. ) ;
#38555=LINE ( 'NONE', #30926, #50076 ) ;
#38556=EDGE_LOOP ( 'NONE', ( #15070, #17673, #21220, #6899 ) ) ;
#38558=ORIENTED_EDGE ( 'NONE', *, *, #48747, .T. ) ;
#38559=ORIENTED_EDGE ( 'NONE', *, *, #14771, .T. ) ;
#38560=DIRECTION ( 'NONE',  ( 0.000000000000000000, 0.000000000000000000, 1.000000000000000000 ) ) ;
#38564=LINE ( 'NONE', #34607, #18385 ) ;
#38566=DIRECTION ( 'NONE',  ( -0.000000000000000000, 1.000000000000000000, -0.000000000000000000 ) ) ;
#38568=ORIENTED_EDGE ( 'NONE', *, *, #45312, .F. ) ;
#38570=LINE ( 'NONE', #41988, #30604 ) ;
#38571=CIRCLE ( 'NONE', #13405, 125.0000000000000000 ) ;
#38572=DIRECTION ( 'NONE',  ( -0.000000000000000000, 1.000000000000000000, -0.000000000000000000 ) ) ;
#38573=VERTEX_POINT ( 'NONE', #21990 ) ;
#38574=CARTESIAN_POINT ( 'NONE',  ( 69.25251857196690253, -189.7472609257535510, 38.92640747825683434 ) ) ;
#38575=CIRCLE ( 'NONE', #18440, 125.0000000000000000 ) ;
#38576=PLANE ( 'NONE',  #18063 ) ;
#38577=CARTESIAN_POINT ( 'NONE',  ( 53.62339707355158680, -183.6283474603465606, -70.36529243996334060 ) ) ;
#38586=ORIENTED_EDGE ( 'NONE', *, *, #21026, .T. ) ;
#38587=EDGE_CURVE ( 'NONE', #33386, #16397, #35260, .T. ) ;
#38588=ADVANCED_FACE ( 'NONE', ( #1502 ), #37243, .T. ) ;
#38589=FACE_OUTER_BOUND ( 'NONE', #10711, .T. ) ;
#38590=VERTEX_POINT ( 'NONE', #42208 ) ;
#38591=VECTOR ( 'NONE', #23029, 1000.000000000000000 ) ;
#38592=PLANE ( 'NONE',  #31819 ) ;
#38594=CARTESIAN_POINT ( 'NONE',  ( 53.56330073376472001, -189.7472609257535510, 72.19655804062048787 ) ) ;
#38596=FACE_OUTER_BOUND ( 'NONE', #25694, .T. ) ;
#38597=ORIENTED_EDGE ( 'NONE', *, *, #44786, .T. ) ;
#38603=EDGE_CURVE ( 'NONE', #24136, #41591, #22242, .T. ) ;
#38604=LINE ( 'NONE', #38345, #29271 ) ;
#38605=ADVANCED_FACE ( 'NONE', ( #5721 ), #29607, .T. ) ;
#38606=PLANE ( 'NONE',  #27578 ) ;
#38607=CARTESIAN_POINT ( 'NONE',  ( -48.47912675150885065, -177.1207230881787780, 6.938893903907228378E-15 ) ) ;
#38608=ORIENTED_EDGE ( 'NONE', *, *, #3369, .F. ) ;
#38610=CARTESIAN_POINT ( 'NONE',  ( -26.37732090265849294, -189.7472609257535510, -122.0143860769386919 ) ) ;
#38611=ORIENTED_EDGE ( 'NONE', *, *, #30104, .F. ) ;
#38612=PLANE ( 'NONE',  #23101 ) ;
#38613=ORIENTED_EDGE ( 'NONE', *, *, #40633, .F. ) ;
#38615=ORIENTED_EDGE ( 'NONE', *, *, #42202, .T. ) ;
#38617=DIRECTION ( 'NONE',  ( 0.000000000000000000, 0.000000000000000000, -1.000000000000000000 ) ) ;
#38618=LINE ( 'NONE', #30994, #40927 ) ;
#38621=VECTOR ( 'NONE', #18516, 1000.000000000000000 ) ;
#38622=AXIS2_PLACEMENT_3D ( 'NONE', #47121, #3235, #3730 ) ;
#38623=PLANE ( 'NONE',  #43314 ) ;
#38625=DIRECTION ( 'NONE',  ( 0.000000000000000000, 0.000000000000000000, 1.000000000000000000 ) ) ;
#38626=CARTESIAN_POINT ( 'NONE',  ( -31.30262293407085039, -177.1207230881787780, -123.8142468240611294 ) ) ;
#38627=VERTEX_POINT ( 'NONE', #50378 ) ;
#38630=DIRECTION ( 'NONE',  ( 0.7765238627180482966, 0.000000000000000000, -0.6300878435817038881 ) ) ;
#38631=FACE_OUTER_BOUND ( 'NONE', #24397, .T. ) ;
#38632=DIRECTION ( 'NONE',  ( 0.000000000000000000, 1.000000000000000000, 0.000000000000000000 ) ) ;
#38633=VERTEX_POINT ( 'NONE', #14366 ) ;
#38634=DIRECTION ( 'NONE',  ( -0.000000000000000000, 1.000000000000000000, -0.000000000000000000 ) ) ;
#38635=CARTESIAN_POINT ( 'NONE',  ( -33.86391487983341619, -175.3837268820161057, 124.1426420773540542 ) ) ;
#38637=CARTESIAN_POINT ( 'NONE',  ( -46.06708674231131084, -193.5000000000000000, -124.9767260852756863 ) ) ;
#38638=VERTEX_POINT ( 'NONE', #33813 ) ;
#38639=AXIS2_PLACEMENT_3D ( 'NONE', #3370, #51471, #34900 ) ;
#38640=PLANE ( 'NONE',  #47474 ) ;
#38642=LINE ( 'NONE', #34699, #8457 ) ;
#38645=VERTEX_POINT ( 'NONE', #10938 ) ;
#38647=CYLINDRICAL_SURFACE ( 'NONE', #49665, 125.0000000000000000 ) ;
#38650=EDGE_CURVE ( 'NONE', #44477, #7058, #35359, .T. ) ;
#38651=ORIENTED_EDGE ( 'NONE', *, *, #51660, .F. ) ;
#38652=CARTESIAN_POINT ( 'NONE',  ( -153.4237445717492392, -175.3837268820161057, 66.05018866041349668 ) ) ;
#38654=VECTOR ( 'NONE', #7112, 1000.000000000000000 ) ;
#38655=CARTESIAN_POINT ( 'NONE',  ( -47.87232660569025455, -193.5000000000000000, -0.7948544414133454916 ) ) ;
#38659=EDGE_CURVE ( 'NONE', #36957, #16290, #51671, .T. ) ;
#38660=CARTESIAN_POINT ( 'NONE',  ( -23.25236516653336594, -183.6283474603465606, -121.4073237908566654 ) ) ;
#38661=DIRECTION ( 'NONE',  ( -0.000000000000000000, 1.000000000000000000, -0.000000000000000000 ) ) ;
#38662=CARTESIAN_POINT ( 'NONE',  ( 141.7825277784304205, -213.5000000000000000, -41.45482488023466061 ) ) ;
#38663=ORIENTED_EDGE ( 'NONE', *, *, #6087, .T. ) ;
#38664=LINE ( 'NONE', #34221, #5014 ) ;
#38666=CARTESIAN_POINT ( 'NONE',  ( 76.01188277843577623, -189.7472609257535510, 11.26891947860283061 ) ) ;
#38667=DIRECTION ( 'NONE',  ( -0.000000000000000000, 1.000000000000000000, -0.000000000000000000 ) ) ;
#38668=VERTEX_POINT ( 'NONE', #11189 ) ;
#38669=VECTOR ( 'NONE', #48765, 1000.000000000000000 ) ;
#38671=PLANE ( 'NONE',  #44028 ) ;
#38672=EDGE_LOOP ( 'NONE', ( #4063, #4751, #51921, #32948 ) ) ;
#38679=ORIENTED_EDGE ( 'NONE', *, *, #29092, .T. ) ;
#38680=DIRECTION ( 'NONE',  ( 0.8757349421956379665, 0.000000000000000000, -0.4827922027307427477 ) ) ;
#38681=CARTESIAN_POINT ( 'NONE',  ( -48.47912675150885065, -189.7472609257535510, 6.938893903907228378E-15 ) ) ;
#38682=ORIENTED_EDGE ( 'NONE', *, *, #1875, .T. ) ;
#38683=DIRECTION ( 'NONE',  ( -0.000000000000000000, 1.000000000000000000, 0.000000000000000000 ) ) ;
#38684=VECTOR ( 'NONE', #7379, 1000.000000000000227 ) ;
#38685=DIRECTION ( 'NONE',  ( -0.000000000000000000, 1.000000000000000000, -0.000000000000000000 ) ) ;
#38687=ORIENTED_EDGE ( 'NONE', *, *, #35291, .T. ) ;
#38689=CARTESIAN_POINT ( 'NONE',  ( -159.0901268547125653, -183.6283474603465606, 58.22548115875958530 ) ) ;
#38691=EDGE_CURVE ( 'NONE', #45141, #26421, #14902, .T. ) ;
#38695=CARTESIAN_POINT ( 'NONE',  ( 71.97629403264902237, -177.1207230881787780, -29.43839964798648623 ) ) ;
#38698=LINE ( 'NONE', #2704, #47042 ) ;
#38703=EDGE_CURVE ( 'NONE', #34512, #47944, #6748, .T. ) ;
#38704=EDGE_LOOP ( 'NONE', ( #41056, #16792, #31152, #30779 ) ) ;
#38705=DIRECTION ( 'NONE',  ( 0.6965510290629882695, 0.000000000000000000, 0.7175072570443395970 ) ) ;
#38706=EDGE_CURVE ( 'NONE', #31601, #42139, #39311, .T. ) ;
#38707=CIRCLE ( 'NONE', #11020, 125.0000000000000000 ) ;
#38708=LINE ( 'NONE', #42664, #42074 ) ;
#38709=CARTESIAN_POINT ( 'NONE',  ( -48.47912675150885065, -183.6283474603465606, 6.938893903907228378E-15 ) ) ;
#38710=CARTESIAN_POINT ( 'NONE',  ( -48.47912675150885065, -189.7472609257535510, 6.938893903907228378E-15 ) ) ;
#38714=DIRECTION ( 'NONE',  ( 0.000000000000000000, 0.000000000000000000, -1.000000000000000000 ) ) ;
#38715=ORIENTED_EDGE ( 'NONE', *, *, #44227, .T. ) ;
#38719=DIRECTION ( 'NONE',  ( -0.000000000000000000, 1.000000000000000000, -0.000000000000000000 ) ) ;
#38720=CYLINDRICAL_SURFACE ( 'NONE', #19430, 125.0000000000000000 ) ;
#38722=VECTOR ( 'NONE', #43552, 1000.000000000000227 ) ;
#38723=VERTEX_POINT ( 'NONE', #27733 ) ;
#38724=ORIENTED_EDGE ( 'NONE', *, *, #45313, .F. ) ;
#38725=CIRCLE ( 'NONE', #16089, 125.0000000000000000 ) ;
#38726=ORIENTED_EDGE ( 'NONE', *, *, #20996, .T. ) ;
#38727=CARTESIAN_POINT ( 'NONE',  ( -238.7407812814481076, -213.5000000000000000, -9.999999999999987566 ) ) ;
#38728=CARTESIAN_POINT ( 'NONE',  ( -122.3978016498073345, -183.6283474603465606, -100.8019320314827070 ) ) ;
#38729=LINE ( 'NONE', #47160, #27034 ) ;
#38730=DIRECTION ( 'NONE',  ( 0.000000000000000000, -1.000000000000000000, 0.000000000000000000 ) ) ;
#38734=ORIENTED_EDGE ( 'NONE', *, *, #27907, .F. ) ;
#38735=ORIENTED_EDGE ( 'NONE', *, *, #633, .T. ) ;
#38737=AXIS2_PLACEMENT_3D ( 'NONE', #22903, #38138, #2146 ) ;
#38738=CARTESIAN_POINT ( 'NONE',  ( -26.20043062753592977, -175.3837268820161057, -122.9986166548863196 ) ) ;
#38739=CARTESIAN_POINT ( 'NONE',  ( -48.47912675150885065, -189.7472609257535510, 6.938893903907228378E-15 ) ) ;
#38741=EDGE_CURVE ( 'NONE', #4396, #13063, #2538, .T. ) ;
#38742=LINE ( 'NONE', #50860, #12777 ) ;
#38745=CARTESIAN_POINT ( 'NONE',  ( 15.80042947435468470, -189.7472609257535510, 107.2060569716377927 ) ) ;
#38746=VERTEX_POINT ( 'NONE', #18817 ) ;
#38748=ORIENTED_EDGE ( 'NONE', *, *, #40051, .T. ) ;
#38749=DIRECTION ( 'NONE',  ( 0.000000000000000000, -0.000000000000000000, 1.000000000000000000 ) ) ;
#38750=DIRECTION ( 'NONE',  ( 0.000000000000000000, -1.000000000000000000, 0.000000000000000000 ) ) ;
#38755=CARTESIAN_POINT ( 'NONE',  ( -48.47912675150885065, -183.6283474603465606, 6.938893903907228378E-15 ) ) ;
#38756=CYLINDRICAL_SURFACE ( 'NONE', #3866, 125.0000000000000000 ) ;
#38757=EDGE_CURVE ( 'NONE', #14148, #3147, #50898, .T. ) ;
#38759=EDGE_CURVE ( 'NONE', #3318, #43850, #42994, .T. ) ;
#38761=CARTESIAN_POINT ( 'NONE',  ( 71.15591247552653442, -183.6283474603465606, 36.22785377504035154 ) ) ;
#38763=ADVANCED_FACE ( 'NONE', ( #51169 ), #3564, .T. ) ;
#38764=CARTESIAN_POINT ( 'NONE',  ( -48.59739992243022755, -183.6283474603465606, 0.9929810960135230236 ) ) ;
#38765=DIRECTION ( 'NONE',  ( 0.000000000000000000, 1.000000000000000000, 0.000000000000000000 ) ) ;
#38767=EDGE_CURVE ( 'NONE', #27923, #32981, #36161, .T. ) ;
#38769=CARTESIAN_POINT ( 'NONE',  ( -172.2424017797220870, -193.5000000000000000, 7.666780576875859232 ) ) ;
#38771=VECTOR ( 'NONE', #26109, 999.9999999999998863 ) ;
#38772=CARTESIAN_POINT ( 'NONE',  ( -172.9089226952081617, -193.5000000000000000, 11.92584929509620117 ) ) ;
#38773=AXIS2_PLACEMENT_3D ( 'NONE', #12586, #40961, #5245 ) ;
#38774=CIRCLE ( 'NONE', #37966, 125.0000000000000000 ) ;
#38778=VERTEX_POINT ( 'NONE', #24320 ) ;
#38781=CARTESIAN_POINT ( 'NONE',  ( -172.1341525481709880, -189.7472609257535510, 18.28755301364335750 ) ) ;
#38782=EDGE_CURVE ( 'NONE', #14631, #34611, #8295, .T. ) ;
#38783=ORIENTED_EDGE ( 'NONE', *, *, #22816, .F. ) ;
#38785=EDGE_LOOP ( 'NONE', ( #38542, #26440, #17732, #36358 ) ) ;
#38786=DIRECTION ( 'NONE',  ( 0.000000000000000000, -0.000000000000000000, -1.000000000000000000 ) ) ;
#38787=LINE ( 'NONE', #10420, #51180 ) ;
#38788=LINE ( 'NONE', #38548, #37718 ) ;
#38789=CARTESIAN_POINT ( 'NONE',  ( -48.47912675150885065, -189.7472609257535510, 6.938893903907228378E-15 ) ) ;
#38790=PLANE ( 'NONE',  #1181 ) ;
#38792=VERTEX_POINT ( 'NONE', #47978 ) ;
#38793=AXIS2_PLACEMENT_3D ( 'NONE', #19216, #27603, #17091 ) ;
#38795=EDGE_CURVE ( 'NONE', #4839, #24818, #39807, .T. ) ;
#38796=ORIENTED_EDGE ( 'NONE', *, *, #42271, .F. ) ;
#38797=CARTESIAN_POINT ( 'NONE',  ( -84.82349129030166068, -193.5000000000000000, -119.5996955107802222 ) ) ;
#38798=ORIENTED_EDGE ( 'NONE', *, *, #35262, .T. ) ;
#38799=VERTEX_POINT ( 'NONE', #669 ) ;
#38801=CARTESIAN_POINT ( 'NONE',  ( -94.78385179329471555, -177.1207230881787780, 115.0304316645283080 ) ) ;
#38802=EDGE_CURVE ( 'NONE', #46508, #29853, #44812, .T. ) ;
#38804=DIRECTION ( 'NONE',  ( -0.000000000000000000, 1.000000000000000000, -0.000000000000000000 ) ) ;
#38807=CARTESIAN_POINT ( 'NONE',  ( 20.65191334053708161, -193.5000000000000000, 102.9412430821799802 ) ) ;
#38808=VERTEX_POINT ( 'NONE', #40325 ) ;
#38810=ORIENTED_EDGE ( 'NONE', *, *, #41764, .F. ) ;
#38814=DIRECTION ( 'NONE',  ( -0.000000000000000000, 1.000000000000000000, -0.000000000000000000 ) ) ;
#38815=VECTOR ( 'NONE', #27520, 1000.000000000000114 ) ;
#38817=AXIS2_PLACEMENT_3D ( 'NONE', #16659, #44759, #39750 ) ;
#38819=DIRECTION ( 'NONE',  ( 0.000000000000000000, -1.000000000000000000, 0.000000000000000000 ) ) ;
#38820=DIRECTION ( 'NONE',  ( 0.000000000000000000, 0.000000000000000000, 1.000000000000000000 ) ) ;
#38822=FACE_OUTER_BOUND ( 'NONE', #31966, .T. ) ;
#38824=CARTESIAN_POINT ( 'NONE',  ( -21.46839590530488451, -193.5000000000000000, 122.0467960216650738 ) ) ;
#38825=CARTESIAN_POINT ( 'NONE',  ( -149.9407190013151592, -189.7472609257535510, -73.01058346660460074 ) ) ;
#38826=VECTOR ( 'NONE', #47520, 1000.000000000000000 ) ;
#38827=EDGE_CURVE ( 'NONE', #10779, #18318, #8797, .T. ) ;
#38829=CARTESIAN_POINT ( 'NONE',  ( -65.65563056894596627, -193.5000000000000000, 123.8142468240612999 ) ) ;
#38830=DIRECTION ( 'NONE',  ( -0.000000000000000000, 1.000000000000000000, -0.000000000000000000 ) ) ;
#38831=EDGE_CURVE ( 'NONE', #21117, #664, #19857, .T. ) ;
#38832=LINE ( 'NONE', #15456, #39144 ) ;
#38833=ORIENTED_EDGE ( 'NONE', *, *, #17776, .F. ) ;
#38840=CARTESIAN_POINT ( 'NONE',  ( 40.71578595748727736, -177.1207230881787780, 86.14171647324927505 ) ) ;
#38843=CIRCLE ( 'NONE', #7782, 125.0000000000000000 ) ;
#38845=FACE_BOUND ( 'NONE', #39315, .T. ) ;
#38846=DIRECTION ( 'NONE',  ( 0.05924062789371441901, 0.000000000000000000, -0.9982437317643214625 ) ) ;
#38848=AXIS2_PLACEMENT_3D ( 'NONE', #20747, #36776, #20472 ) ;
#38851=ORIENTED_EDGE ( 'NONE', *, *, #47245, .T. ) ;
#38852=ADVANCED_FACE ( 'NONE', ( #20113 ), #48242, .T. ) ;
#38853=EDGE_LOOP ( 'NONE', ( #36607, #46494, #44116, #38877 ) ) ;
#38854=DIRECTION ( 'NONE',  ( 0.000000000000000000, 0.000000000000000000, 1.000000000000000000 ) ) ;
#38855=VECTOR ( 'NONE', #10281, 1000.000000000000000 ) ;
#38858=AXIS2_PLACEMENT_3D ( 'NONE', #25159, #4932, #21209 ) ;
#38860=DIRECTION ( 'NONE',  ( 0.000000000000000000, 0.000000000000000000, -1.000000000000000000 ) ) ;
#38862=DIRECTION ( 'NONE',  ( 0.000000000000000000, -0.000000000000000000, 1.000000000000000000 ) ) ;
#38864=ORIENTED_EDGE ( 'NONE', *, *, #38529, .F. ) ;
#38865=DIRECTION ( 'NONE',  ( 0.6068001458185945385, 0.000000000000000000, -0.7948544414133523750 ) ) ;
#38866=VERTEX_POINT ( 'NONE', #45605 ) ;
#38867=LINE ( 'NONE', #6579, #42401 ) ;
#38868=VECTOR ( 'NONE', #19195, 999.9999999999998863 ) ;
#38869=ORIENTED_EDGE ( 'NONE', *, *, #10172, .F. ) ;
#38871=EDGE_CURVE ( 'NONE', #46522, #1772, #41902, .T. ) ;
#38874=CARTESIAN_POINT ( 'NONE',  ( -171.5592422664403216, -177.1207230881787780, -21.82395850507255375 ) ) ;
#38876=ORIENTED_EDGE ( 'NONE', *, *, #3598, .F. ) ;
#38877=ORIENTED_EDGE ( 'NONE', *, *, #48303, .F. ) ;
#38878=VECTOR ( 'NONE', #31347, 1000.000000000000114 ) ;
#38881=VERTEX_POINT ( 'NONE', #33756 ) ;
#38882=LINE ( 'NONE', #34679, #1854 ) ;
#38883=CARTESIAN_POINT ( 'NONE',  ( 32.99469856375238663, -175.3837268820161057, 94.79987230212020677 ) ) ;
#38885=CARTESIAN_POINT ( 'NONE',  ( -238.7407812814481076, -193.5000000000000000, -9.999999999999987566 ) ) ;
#38887=DIRECTION ( 'NONE',  ( 0.000000000000000000, 1.000000000000000000, 0.000000000000000000 ) ) ;
#38888=FACE_OUTER_BOUND ( 'NONE', #37762, .T. ) ;
#38890=AXIS2_PLACEMENT_3D ( 'NONE', #25547, #30016, #41570 ) ;
#38891=FACE_OUTER_BOUND ( 'NONE', #14329, .T. ) ;
#38892=DIRECTION ( 'NONE',  ( 0.8124868780056825335, 0.000000000000000000, -0.5829794791144703447 ) ) ;
#38893=CARTESIAN_POINT ( 'NONE',  ( 20.66186849114819069, -193.5000000000000000, -104.1370384486465070 ) ) ;
#38895=VECTOR ( 'NONE', #41402, 1000.000000000000114 ) ;
#38896=DIRECTION ( 'NONE',  ( 0.000000000000000000, 0.000000000000000000, -1.000000000000000000 ) ) ;
#38898=DIRECTION ( 'NONE',  ( 0.000000000000000000, 1.000000000000000000, 0.000000000000000000 ) ) ;
#38901=ORIENTED_EDGE ( 'NONE', *, *, #28532, .F. ) ;
#38904=DIRECTION ( 'NONE',  ( 0.000000000000000000, 0.000000000000000000, -1.000000000000000000 ) ) ;
#38906=CARTESIAN_POINT ( 'NONE',  ( -48.07600332222087758, -189.7472609257535510, -0.9151456172430111335 ) ) ;
#38908=AXIS2_PLACEMENT_3D ( 'NONE', #5773, #41997, #29916 ) ;
#38909=EDGE_LOOP ( 'NONE', ( #47131, #28472, #2979, #25679 ) ) ;
#38910=FACE_OUTER_BOUND ( 'NONE', #27529, .T. ) ;
#38911=VECTOR ( 'NONE', #50507, 999.9999999999998863 ) ;
#38912=DIRECTION ( 'NONE',  ( 0.000000000000000000, -1.000000000000000000, -0.000000000000000000 ) ) ;
#38913=VERTEX_POINT ( 'NONE', #22191 ) ;
#38914=ORIENTED_EDGE ( 'NONE', *, *, #21395, .F. ) ;
#38917=CARTESIAN_POINT ( 'NONE',  ( -107.6930423737362190, -183.6283474603465606, 110.0850225811110761 ) ) ;
#38919=ORIENTED_EDGE ( 'NONE', *, *, #28771, .T. ) ;
#38920=CARTESIAN_POINT ( 'NONE',  ( 24.15597040328004752, -193.5000000000000000, -101.7307360698543874 ) ) ;
#38921=CARTESIAN_POINT ( 'NONE',  ( -48.47912675150885065, -177.1207230881787780, 6.938893903907228378E-15 ) ) ;
#38922=CARTESIAN_POINT ( 'NONE',  ( -43.48323084606168720, -177.1207230881787780, 124.9001241957026167 ) ) ;
#38923=DIRECTION ( 'NONE',  ( -0.2348860457809707758, 0.000000000000000000, -0.9720229140804138579 ) ) ;
#38925=CARTESIAN_POINT ( 'NONE',  ( -26.71218532227686637, -175.3837268820161057, 122.0745693923550732 ) ) ;
#38926=ORIENTED_EDGE ( 'NONE', *, *, #24791, .T. ) ;
#38927=DIRECTION ( 'NONE',  ( 0.000000000000000000, 0.000000000000000000, -1.000000000000000000 ) ) ;
#38929=EDGE_CURVE ( 'NONE', #20567, #33538, #41183, .T. ) ;
#38932=CARTESIAN_POINT ( 'NONE',  ( -156.9880281022168163, -189.7472609257535510, -60.01515274640939879 ) ) ;
#38933=EDGE_LOOP ( 'NONE', ( #24907, #26220, #29628, #42226 ) ) ;
#38934=VERTEX_POINT ( 'NONE', #29297 ) ;
#38935=DIRECTION ( 'NONE',  ( -0.000000000000000000, 1.000000000000000000, -0.000000000000000000 ) ) ;
#38939=AXIS2_PLACEMENT_3D ( 'NONE', #4291, #28705, #40275 ) ;
#38940=PLANE ( 'NONE',  #2190 ) ;
#38942=ORIENTED_EDGE ( 'NONE', *, *, #35247, .T. ) ;
#38944=CARTESIAN_POINT ( 'NONE',  ( 50.70030191143631271, -193.5000000000000000, -76.08180419845318454 ) ) ;
#38945=AXIS2_PLACEMENT_3D ( 'NONE', #23273, #35088, #26415 ) ;
#38946=ORIENTED_EDGE ( 'NONE', *, *, #39617, .T. ) ;
#38947=DIRECTION ( 'NONE',  ( 0.8124868780056742068, 0.000000000000000000, 0.5829794791144820021 ) ) ;
#38948=VERTEX_POINT ( 'NONE', #45857 ) ;
#38949=CYLINDRICAL_SURFACE ( 'NONE', #39865, 125.0000000000000000 ) ;
#38951=EDGE_CURVE ( 'NONE', #4337, #34100, #5664, .T. ) ;
#38952=ORIENTED_EDGE ( 'NONE', *, *, #36956, .F. ) ;
#38956=VECTOR ( 'NONE', #35631, 1000.000000000000000 ) ;
#38958=CARTESIAN_POINT ( 'NONE',  ( 76.31829002442924548, -183.6283474603465606, 7.113702696402428138 ) ) ;
#38959=ADVANCED_FACE ( 'NONE', ( #17220 ), #1703, .T. ) ;
#38960=CARTESIAN_POINT ( 'NONE',  ( -48.47912675150885065, -175.3837268820161057, 6.938893903907228378E-15 ) ) ;
#38965=DIRECTION ( 'NONE',  ( 0.9842305779475980509, 0.000000000000000000, -0.1768902751225666647 ) ) ;
#38966=EDGE_CURVE ( 'NONE', #40042, #5249, #1763, .T. ) ;
#38967=DIRECTION ( 'NONE',  ( 0.7948544414133565938, 0.000000000000000000, -0.6068001458185890984 ) ) ;
#38971=ORIENTED_EDGE ( 'NONE', *, *, #24358, .F. ) ;
#38972=CARTESIAN_POINT ( 'NONE',  ( -130.7087404384255080, -175.3837268820161057, -94.14505102712755047 ) ) ;
#38973=CARTESIAN_POINT ( 'NONE',  ( -68.21229068036655008, -183.6283474603465606, -123.4325817657429809 ) ) ;
#38977=DIRECTION ( 'NONE',  ( -0.000000000000000000, 1.000000000000000000, -0.000000000000000000 ) ) ;
#38978=VERTEX_POINT ( 'NONE', #42149 ) ;
#38981=ORIENTED_EDGE ( 'NONE', *, *, #32331, .T. ) ;
#38983=CARTESIAN_POINT ( 'NONE',  ( -108.5723883981723930, -177.1207230881787780, 109.6074810615846360 ) ) ;
#38984=FACE_OUTER_BOUND ( 'NONE', #4616, .T. ) ;
#38986=CARTESIAN_POINT ( 'NONE',  ( -157.4685091425930636, -175.3837268820161057, -59.13814366165043168 ) ) ;
#38987=DIRECTION ( 'NONE',  ( 0.000000000000000000, 0.000000000000000000, 1.000000000000000000 ) ) ;
#38988=ORIENTED_EDGE ( 'NONE', *, *, #43380, .T. ) ;
#38990=ADVANCED_FACE ( 'NONE', ( #49285 ), #37955, .T. ) ;
#38992=CARTESIAN_POINT ( 'NONE',  ( -48.65601702663141737, -193.5000000000000000, -0.9842305779475923888 ) ) ;
#38995=ORIENTED_EDGE ( 'NONE', *, *, #41730, .T. ) ;
#38996=EDGE_CURVE ( 'NONE', #33019, #34940, #50062, .T. ) ;
#38998=DIRECTION ( 'NONE',  ( -0.8757349421956412971, 0.000000000000000000, 0.4827922027307366970 ) ) ;
#39000=FACE_OUTER_BOUND ( 'NONE', #30286, .T. ) ;
#39002=ORIENTED_EDGE ( 'NONE', *, *, #27130, .T. ) ;
#39003=PLANE ( 'NONE',  #38500 ) ;
#39005=DIRECTION ( 'NONE',  ( 0.000000000000000000, 0.000000000000000000, 1.000000000000000000 ) ) ;
#39011=VECTOR ( 'NONE', #21656, 1000.000000000000000 ) ;
#39012=DIRECTION ( 'NONE',  ( 0.000000000000000000, -0.000000000000000000, -1.000000000000000000 ) ) ;
#39013=DIRECTION ( 'NONE',  ( 0.000000000000000000, 0.000000000000000000, 1.000000000000000000 ) ) ;
#39016=VECTOR ( 'NONE', #43440, 1000.000000000000000 ) ;
#39020=DIRECTION ( 'NONE',  ( 0.3202698538628416247, 0.000000000000000000, -0.9473263538541900619 ) ) ;
#39021=DIRECTION ( 'NONE',  ( -0.000000000000000000, 1.000000000000000000, -0.000000000000000000 ) ) ;
#39022=ORIENTED_EDGE ( 'NONE', *, *, #19277, .F. ) ;
#39025=DIRECTION ( 'NONE',  ( -0.000000000000000000, 1.000000000000000000, -0.000000000000000000 ) ) ;
#39029=DIRECTION ( 'NONE',  ( -0.9266896074318370369, 0.000000000000000000, 0.3758275821142292306 ) ) ;
#39030=ORIENTED_EDGE ( 'NONE', *, *, #17473, .F. ) ;
#39032=CARTESIAN_POINT ( 'NONE',  ( -48.47912675150885065, -175.3837268820161057, 6.938893903907228378E-15 ) ) ;
#39035=EDGE_CURVE ( 'NONE', #40551, #23392, #5977, .T. ) ;
#39036=ADVANCED_FACE ( 'NONE', ( #29549 ), #47399, .T. ) ;
#39037=CARTESIAN_POINT ( 'NONE',  ( -69.77312546433407192, -193.5000000000000000, 123.1729094355500109 ) ) ;
#39040=ORIENTED_EDGE ( 'NONE', *, *, #35269, .T. ) ;
#39042=CARTESIAN_POINT ( 'NONE',  ( -147.2362428880188077, -193.5000000000000000, -74.98773087994455011 ) ) ;
#39045=PLANE ( 'NONE',  #20921 ) ;
#39046=AXIS2_PLACEMENT_3D ( 'NONE', #20323, #36356, #20588 ) ;
#39048=DIRECTION ( 'NONE',  ( 0.000000000000000000, 0.000000000000000000, 1.000000000000000000 ) ) ;
#39049=ORIENTED_EDGE ( 'NONE', *, *, #38466, .F. ) ;
#39052=ADVANCED_FACE ( 'NONE', ( #14839 ), #11378, .T. ) ;
#39053=CARTESIAN_POINT ( 'NONE',  ( -88.23625491228469286, -177.1207230881787780, 118.5089480183148254 ) ) ;
#39054=ORIENTED_EDGE ( 'NONE', *, *, #23639, .T. ) ;
#39055=LINE ( 'NONE', #43265, #39060 ) ;
#39058=EDGE_CURVE ( 'NONE', #34403, #45844, #35333, .T. ) ;
#39059=CARTESIAN_POINT ( 'NONE',  ( 73.87536152799695799, -193.5000000000000000, -25.58083653558413317 ) ) ;
#39060=VECTOR ( 'NONE', #23316, 1000.000000000000000 ) ;
#39062=AXIS2_PLACEMENT_3D ( 'NONE', #22310, #10227, #6038 ) ;
#39063=EDGE_CURVE ( 'NONE', #12404, #19021, #11125, .T. ) ;
#39064=CARTESIAN_POINT ( 'NONE',  ( 74.61260187273140332, -183.6283474603465606, -14.98512977653174794 ) ) ;
#39065=CARTESIAN_POINT ( 'NONE',  ( -148.6149069237406195, -193.5000000000000000, -74.81861753132355375 ) ) ;
#39069=EDGE_LOOP ( 'NONE', ( #49332, #9520, #43389, #27038 ) ) ;
#39070=CIRCLE ( 'NONE', #38252, 125.0000000000000000 ) ;
#39072=LINE ( 'NONE', #2044, #34589 ) ;
#39073=FACE_OUTER_BOUND ( 'NONE', #30197, .T. ) ;
#39074=ORIENTED_EDGE ( 'NONE', *, *, #31100, .T. ) ;
#39075=CARTESIAN_POINT ( 'NONE',  ( -49.30901192927175458, -193.5000000000000000, -123.9972451320097093 ) ) ;
#39076=LINE ( 'NONE', #3087, #12144 ) ;
#39078=DIRECTION ( 'NONE',  ( 0.000000000000000000, 0.000000000000000000, 1.000000000000000000 ) ) ;
#39079=ORIENTED_EDGE ( 'NONE', *, *, #10466, .F. ) ;
#39080=LINE ( 'NONE', #3092, #48152 ) ;
#39081=DIRECTION ( 'NONE',  ( 0.000000000000000000, 0.000000000000000000, -1.000000000000000000 ) ) ;
#39082=PLANE ( 'NONE',  #2247 ) ;
#39083=ORIENTED_EDGE ( 'NONE', *, *, #16740, .T. ) ;
#39084=AXIS2_PLACEMENT_3D ( 'NONE', #234, #40434, #48080 ) ;
#39085=CARTESIAN_POINT ( 'NONE',  ( -19.51863976943889867, -175.3837268820161057, 120.5706864261537277 ) ) ;
#39086=VECTOR ( 'NONE', #38103, 1000.000000000000000 ) ;
#39087=VECTOR ( 'NONE', #48877, 1000.000000000000114 ) ;
#39088=DIRECTION ( 'NONE',  ( 0.9374196611341231167, 0.000000000000000000, -0.3482016354343928088 ) ) ;
#39091=VERTEX_POINT ( 'NONE', #10620 ) ;
#39092=EDGE_CURVE ( 'NONE', #1503, #22453, #23234, .T. ) ;
#39093=FACE_OUTER_BOUND ( 'NONE', #20993, .T. ) ;
#39094=FACE_BOUND ( 'NONE', #3208, .T. ) ;
#39096=CARTESIAN_POINT ( 'NONE',  ( 57.31108707223382481, -175.3837268820161057, -66.58401203837755133 ) ) ;
#39098=EDGE_CURVE ( 'NONE', #51600, #18514, #19294, .T. ) ;
#39099=EDGE_CURVE ( 'NONE', #27859, #11977, #30577, .T. ) ;
#39101=AXIS2_PLACEMENT_3D ( 'NONE', #43350, #11791, #50994 ) ;
#39103=ORIENTED_EDGE ( 'NONE', *, *, #21450, .F. ) ;
#39104=EDGE_CURVE ( 'NONE', #26723, #41529, #26652, .T. ) ;
#39105=ORIENTED_EDGE ( 'NONE', *, *, #48032, .F. ) ;
#39107=DIRECTION ( 'NONE',  ( 0.000000000000000000, -0.000000000000000000, 1.000000000000000000 ) ) ;
#39109=EDGE_CURVE ( 'NONE', #25612, #602, #42416, .T. ) ;
#39115=VERTEX_POINT ( 'NONE', #2725 ) ;
#39118=ORIENTED_EDGE ( 'NONE', *, *, #30111, .T. ) ;
#39120=VECTOR ( 'NONE', #12255, 1000.000000000000000 ) ;
#39121=EDGE_CURVE ( 'NONE', #14481, #38037, #20253, .T. ) ;
#39122=CARTESIAN_POINT ( 'NONE',  ( -49.13194886969936448, -183.6283474603465606, -0.7575112421616214675 ) ) ;
#39123=EDGE_LOOP ( 'NONE', ( #7969, #3440, #4845, #45179 ) ) ;
#39127=ADVANCED_FACE ( 'NONE', ( #10360 ), #38720, .T. ) ;
#39128=DIRECTION ( 'NONE',  ( 0.000000000000000000, 1.000000000000000000, 0.000000000000000000 ) ) ;
#39129=VERTEX_POINT ( 'NONE', #46899 ) ;
#39130=FACE_OUTER_BOUND ( 'NONE', #15246, .T. ) ;
#39132=EDGE_LOOP ( 'NONE', ( #41398, #48518, #25486, #32250 ) ) ;
#39133=EDGE_CURVE ( 'NONE', #26117, #13237, #10880, .T. ) ;
#39135=ORIENTED_EDGE ( 'NONE', *, *, #31656, .F. ) ;
#39136=CARTESIAN_POINT ( 'NONE',  ( 8.750818922897904528, -189.7472609257535510, -111.1293539894138434 ) ) ;
#39137=VECTOR ( 'NONE', #9297, 1000.000000000000000 ) ;
#39139=ORIENTED_EDGE ( 'NONE', *, *, #48140, .T. ) ;
#39141=DIRECTION ( 'NONE',  ( -0.000000000000000000, 1.000000000000000000, -0.000000000000000000 ) ) ;
#39142=DIRECTION ( 'NONE',  ( -0.000000000000000000, 1.000000000000000000, -0.000000000000000000 ) ) ;
#39144=VECTOR ( 'NONE', #27259, 1000.000000000000114 ) ;
#39145=AXIS2_PLACEMENT_3D ( 'NONE', #10194, #9684, #29907 ) ;
#39147=VERTEX_POINT ( 'NONE', #23486 ) ;
#39149=AXIS2_PLACEMENT_3D ( 'NONE', #46126, #26123, #22192 ) ;
#39150=LINE ( 'NONE', #26806, #9513 ) ;
#39151=EDGE_CURVE ( 'NONE', #24942, #21292, #46374, .T. ) ;
#39154=FACE_OUTER_BOUND ( 'NONE', #47141, .T. ) ;
#39155=VERTEX_POINT ( 'NONE', #11893 ) ;
#39157=CIRCLE ( 'NONE', #15570, 125.0000000000000000 ) ;
#39158=CARTESIAN_POINT ( 'NONE',  ( 60.51025563957495024, -193.5000000000000000, 59.13814366165116354 ) ) ;
#39160=DIRECTION ( 'NONE',  ( -0.000000000000000000, 1.000000000000000000, -0.000000000000000000 ) ) ;
#39161=ORIENTED_EDGE ( 'NONE', *, *, #17231, .T. ) ;
#39162=ORIENTED_EDGE ( 'NONE', *, *, #11242, .T. ) ;
#39163=EDGE_CURVE ( 'NONE', #9746, #15667, #31989, .T. ) ;
#39164=VECTOR ( 'NONE', #15909, 1000.000000000000000 ) ;
#39165=CARTESIAN_POINT ( 'NONE',  ( -48.47912675150885065, -183.6283474603465606, 6.938893903907228378E-15 ) ) ;
#39167=CARTESIAN_POINT ( 'NONE',  ( -112.7586829773731267, -175.3837268820161057, -107.2060569716373379 ) ) ;
#39168=DIRECTION ( 'NONE',  ( -0.6068001458185890984, 0.000000000000000000, -0.7948544414133565938 ) ) ;
#39169=LINE ( 'NONE', #3424, #6927 ) ;
#39170=DIRECTION ( 'NONE',  ( 0.000000000000000000, -0.000000000000000000, 1.000000000000000000 ) ) ;
#39171=VECTOR ( 'NONE', #23223, 1000.000000000000114 ) ;
#39172=ORIENTED_EDGE ( 'NONE', *, *, #44089, .T. ) ;
#39173=EDGE_CURVE ( 'NONE', #43321, #17649, #46278, .T. ) ;
#39174=EDGE_CURVE ( 'NONE', #30367, #19842, #3756, .T. ) ;
#39176=ADVANCED_FACE ( 'NONE', ( #4033 ), #12145, .T. ) ;
#39177=EDGE_CURVE ( 'NONE', #17406, #10047, #20050, .T. ) ;
#39178=ORIENTED_EDGE ( 'NONE', *, *, #7529, .T. ) ;
#39179=AXIS2_PLACEMENT_3D ( 'NONE', #17502, #18004, #4888 ) ;
#39180=ORIENTED_EDGE ( 'NONE', *, *, #49938, .F. ) ;
#39181=CIRCLE ( 'NONE', #49254, 125.0000000000000000 ) ;
#39182=VERTEX_POINT ( 'NONE', #32131 ) ;
#39184=AXIS2_PLACEMENT_3D ( 'NONE', #23959, #51568, #19263 ) ;
#39185=CARTESIAN_POINT ( 'NONE',  ( -60.86541030502398542, -177.1207230881787780, -124.3848060646151623 ) ) ;
#39186=CIRCLE ( 'NONE', #46780, 125.0000000000000000 ) ;
#39188=CIRCLE ( 'NONE', #34173, 125.0000000000000000 ) ;
#39192=DIRECTION ( 'NONE',  ( -0.2348860457809707758, 0.000000000000000000, -0.9720229140804138579 ) ) ;
#39193=VERTEX_POINT ( 'NONE', #36076 ) ;
#39195=CARTESIAN_POINT ( 'NONE',  ( -238.7407812814481076, -213.5000000000000000, -9.999999999999987566 ) ) ;
#39196=ORIENTED_EDGE ( 'NONE', *, *, #8288, .T. ) ;
#39197=CARTESIAN_POINT ( 'NONE',  ( -73.70588833648349691, -183.6283474603465606, 121.4073237908568359 ) ) ;
#39202=CARTESIAN_POINT ( 'NONE',  ( -16.10442403432823255, -193.5000000000000000, -119.6996507684850286 ) ) ;
#39203=ORIENTED_EDGE ( 'NONE', *, *, #17373, .T. ) ;
#39204=EDGE_CURVE ( 'NONE', #39548, #12962, #38707, .T. ) ;
#39205=FACE_OUTER_BOUND ( 'NONE', #12336, .T. ) ;
#39207=VERTEX_POINT ( 'NONE', #74 ) ;
#39208=CARTESIAN_POINT ( 'NONE',  ( -48.47912675150885065, -189.7472609257535510, 6.938893903907228378E-15 ) ) ;
#39209=CIRCLE ( 'NONE', #35008, 125.0000000000000000 ) ;
#39211=EDGE_LOOP ( 'NONE', ( #42623, #27611, #39022, #28061 ) ) ;
#39213=AXIS2_PLACEMENT_3D ( 'NONE', #5587, #21614, #33686 ) ;
#39215=EDGE_LOOP ( 'NONE', ( #15177, #12821, #48330, #5279 ) ) ;
#39218=EDGE_LOOP ( 'NONE', ( #8901, #23815, #17767, #37403 ) ) ;
#39219=CARTESIAN_POINT ( 'NONE',  ( -48.47912675150885065, -177.1207230881787780, 6.938893903907228378E-15 ) ) ;
#39220=VERTEX_POINT ( 'NONE', #44229 ) ;
#39221=AXIS2_PLACEMENT_3D ( 'NONE', #34832, #10156, #50377 ) ;
#39222=CARTESIAN_POINT ( 'NONE',  ( 27.50603775690334274, -189.7472609257535510, -99.25348746834811209 ) ) ;
#39223=CIRCLE ( 'NONE', #32510, 125.0000000000000000 ) ;
#39224=CARTESIAN_POINT ( 'NONE',  ( -48.41988612361514299, -189.7472609257535510, -0.9982437317643144681 ) ) ;
#39225=ORIENTED_EDGE ( 'NONE', *, *, #28066, .T. ) ;
#39229=LINE ( 'NONE', #19507, #36660 ) ;
#39230=VECTOR ( 'NONE', #16547, 1000.000000000000000 ) ;
#39231=FACE_OUTER_BOUND ( 'NONE', #47699, .T. ) ;
#39232=FACE_OUTER_BOUND ( 'NONE', #34778, .T. ) ;
#39233=VECTOR ( 'NONE', #47817, 999.9999999999998863 ) ;
#39234=DIRECTION ( 'NONE',  ( -0.6749830015182196608, 0.000000000000000000, 0.7378332790417189146 ) ) ;
#39236=CARTESIAN_POINT ( 'NONE',  ( -48.47912675150885065, -177.1207230881787780, 6.938893903907228378E-15 ) ) ;
#39239=ADVANCED_FACE ( 'NONE', ( #43708 ), #4542, .T. ) ;
#39240=EDGE_CURVE ( 'NONE', #48318, #18389, #47916, .T. ) ;
#39242=LINE ( 'NONE', #23226, #25464 ) ;
#39243=VERTEX_POINT ( 'NONE', #8226 ) ;
#39244=VECTOR ( 'NONE', #32414, 999.9999999999998863 ) ;
#39245=CIRCLE ( 'NONE', #8187, 125.0000000000000000 ) ;
#39247=CARTESIAN_POINT ( 'NONE',  ( -99.22478721462985618, -189.7472609257535510, -113.1409892739921901 ) ) ;
#39248=ORIENTED_EDGE ( 'NONE', *, *, #7511, .F. ) ;
#39250=LINE ( 'NONE', #30322, #7380 ) ;
#39252=DIRECTION ( 'NONE',  ( 0.6528221181905174975, 0.000000000000000000, 0.7575112421616236880 ) ) ;
#39253=DIRECTION ( 'NONE',  ( 0.000000000000000000, 1.000000000000000000, 0.000000000000000000 ) ) ;
#39255=ORIENTED_EDGE ( 'NONE', *, *, #40966, .F. ) ;
#39257=DIRECTION ( 'NONE',  ( 0.000000000000000000, 0.000000000000000000, -1.000000000000000000 ) ) ;
#39258=CARTESIAN_POINT ( 'NONE',  ( 43.63512310656540905, -175.3837268820161057, 84.49831343337136502 ) ) ;
#39259=CIRCLE ( 'NONE', #7387, 125.0000000000000000 ) ;
#39261=EDGE_CURVE ( 'NONE', #23501, #5804, #47125, .T. ) ;
#39262=VECTOR ( 'NONE', #28980, 1000.000000000000000 ) ;
#39263=CARTESIAN_POINT ( 'NONE',  ( -73.94077438226447896, -177.1207230881787780, 122.3793467049372481 ) ) ;
#39264=CARTESIAN_POINT ( 'NONE',  ( -43.48323084606168720, -193.5000000000000000, 124.9001241957026167 ) ) ;
#39267=CARTESIAN_POINT ( 'NONE',  ( -145.6517069852673103, -189.7472609257535510, 78.62880929222940551 ) ) ;
#39268=EDGE_CURVE ( 'NONE', #33217, #14253, #2628, .T. ) ;
#39270=ORIENTED_EDGE ( 'NONE', *, *, #16947, .T. ) ;
#39271=ORIENTED_EDGE ( 'NONE', *, *, #30897, .T. ) ;
#39272=DIRECTION ( 'NONE',  ( 0.9982437317643217956, 0.000000000000000000, -0.05924062789370748011 ) ) ;
#39274=ORIENTED_EDGE ( 'NONE', *, *, #43847, .T. ) ;
#39275=DIRECTION ( 'NONE',  ( 0.000000000000000000, -1.000000000000000000, 0.000000000000000000 ) ) ;
#39279=FACE_OUTER_BOUND ( 'NONE', #33556, .T. ) ;
#39281=ORIENTED_EDGE ( 'NONE', *, *, #46193, .T. ) ;
#39282=CARTESIAN_POINT ( 'NONE',  ( -48.93575598890257794, -193.5000000000000000, 0.8896570909947506545 ) ) ;
#39283=CIRCLE ( 'NONE', #46881, 125.0000000000000000 ) ;
#39284=AXIS2_PLACEMENT_3D ( 'NONE', #42502, #2566, #7288 ) ;
#39285=CARTESIAN_POINT ( 'NONE',  ( -133.8011377042516301, -193.5000000000000000, -91.35181687837437892 ) ) ;
#39286=ORIENTED_EDGE ( 'NONE', *, *, #45916, .F. ) ;
#39287=VECTOR ( 'NONE', #37582, 1000.000000000000000 ) ;
#39288=CARTESIAN_POINT ( 'NONE',  ( -168.4003408533108086, -183.6283474603465606, -35.26900067126612726 ) ) ;
#39290=PLANE ( 'NONE',  #22359 ) ;
#39291=DIRECTION ( 'NONE',  ( 0.000000000000000000, -0.000000000000000000, -1.000000000000000000 ) ) ;
#39292=EDGE_CURVE ( 'NONE', #26252, #41591, #16065, .T. ) ;
#39293=DIRECTION ( 'NONE',  ( 0.000000000000000000, -1.000000000000000000, -0.000000000000000000 ) ) ;
#39294=ORIENTED_EDGE ( 'NONE', *, *, #31937, .F. ) ;
#39296=AXIS2_PLACEMENT_3D ( 'NONE', #7579, #34407, #42803 ) ;
#39297=LINE ( 'NONE', #3301, #10910 ) ;
#39298=PLANE ( 'NONE',  #19536 ) ;
#39300=ORIENTED_EDGE ( 'NONE', *, *, #16049, .T. ) ;
#39301=CARTESIAN_POINT ( 'NONE',  ( -126.2322430781613605, -183.6283474603465606, 97.87467957288053810 ) ) ;
#39302=EDGE_CURVE ( 'NONE', #6939, #13237, #41223, .T. ) ;
#39303=VECTOR ( 'NONE', #24404, 1000.000000000000000 ) ;
#39305=EDGE_CURVE ( 'NONE', #19975, #14630, #28693, .T. ) ;
#39306=VERTEX_POINT ( 'NONE', #4814 ) ;
#39307=LINE ( 'NONE', #3309, #27285 ) ;
#39309=ORIENTED_EDGE ( 'NONE', *, *, #49274, .F. ) ;
#39310=LINE ( 'NONE', #25604, #25020 ) ;
#39311=LINE ( 'NONE', #47732, #31135 ) ;
#39313=ORIENTED_EDGE ( 'NONE', *, *, #24913, .F. ) ;
#39314=VERTEX_POINT ( 'NONE', #31616 ) ;
#39315=EDGE_LOOP ( 'NONE', ( #18973, #9141, #36770, #5187 ) ) ;
#39316=CARTESIAN_POINT ( 'NONE',  ( -48.47912675150885065, -189.7472609257535510, 6.938893903907228378E-15 ) ) ;
#39319=AXIS2_PLACEMENT_3D ( 'NONE', #45884, #9878, #25901 ) ;
#39320=VECTOR ( 'NONE', #34661, 1000.000000000000000 ) ;
#39325=AXIS2_PLACEMENT_3D ( 'NONE', #27552, #35425, #7830 ) ;
#39326=DIRECTION ( 'NONE',  ( 0.000000000000000000, -1.000000000000000000, 0.000000000000000000 ) ) ;
#39328=CARTESIAN_POINT ( 'NONE',  ( -12.10142301649613827, -189.7472609257535510, -118.5439281552630746 ) ) ;
#39329=ORIENTED_EDGE ( 'NONE', *, *, #11898, .F. ) ;
#39332=DIRECTION ( 'NONE',  ( 0.000000000000000000, 0.000000000000000000, -1.000000000000000000 ) ) ;
#39333=CARTESIAN_POINT ( 'NONE',  ( 37.99238433767461487, -175.3837268820161057, -90.26448786734026442 ) ) ;
#39335=ORIENTED_EDGE ( 'NONE', *, *, #9573, .F. ) ;
#39338=CIRCLE ( 'NONE', #29288, 125.0000000000000000 ) ;
#39340=LINE ( 'NONE', #3594, #19558 ) ;
#39341=DIRECTION ( 'NONE',  ( -0.9374196611341206742, 0.000000000000000000, -0.3482016354343996367 ) ) ;
#39342=CARTESIAN_POINT ( 'NONE',  ( -37.08895481556041318, -183.6283474603465606, 124.4799742258550452 ) ) ;
#39343=FACE_OUTER_BOUND ( 'NONE', #40328, .T. ) ;
#39345=DIRECTION ( 'NONE',  ( 0.1768902751225592818, 0.000000000000000000, 0.9842305779475992722 ) ) ;
#39348=DIRECTION ( 'NONE',  ( 0.000000000000000000, 1.000000000000000000, -0.000000000000000000 ) ) ;
#39349=CARTESIAN_POINT ( 'NONE',  ( -167.6453766917639427, -183.6283474603465606, 37.74128873232411507 ) ) ;
#39351=VERTEX_POINT ( 'NONE', #49494 ) ;
#39352=AXIS2_PLACEMENT_3D ( 'NONE', #24434, #28098, #783 ) ;
#39353=LINE ( 'NONE', #3359, #9659 ) ;
#39356=ORIENTED_EDGE ( 'NONE', *, *, #23642, .T. ) ;
#39357=DIRECTION ( 'NONE',  ( -0.000000000000000000, 1.000000000000000000, -0.000000000000000000 ) ) ;
#39358=EDGE_CURVE ( 'NONE', #42195, #43059, #1648, .T. ) ;
#39359=ORIENTED_EDGE ( 'NONE', *, *, #33020, .F. ) ;
#39360=ADVANCED_FACE ( 'NONE', ( #5072 ), #21086, .T. ) ;
#39361=VECTOR ( 'NONE', #18811, 1000.000000000000000 ) ;
#39362=FACE_OUTER_BOUND ( 'NONE', #6336, .T. ) ;
#39363=EDGE_CURVE ( 'NONE', #20713, #39399, #49734, .T. ) ;
#39364=FACE_BOUND ( 'NONE', #46273, .T. ) ;
#39366=CARTESIAN_POINT ( 'NONE',  ( -123.5870580700902508, -193.5000000000000000, -98.66508442481455177 ) ) ;
#39367=ORIENTED_EDGE ( 'NONE', *, *, #41095, .T. ) ;
#39369=DIRECTION ( 'NONE',  ( 0.000000000000000000, 0.000000000000000000, 1.000000000000000000 ) ) ;
#39370=VERTEX_POINT ( 'NONE', #37646 ) ;
#39371=DIRECTION ( 'NONE',  ( -0.9473263538541899509, 0.000000000000000000, -0.3202698538628415692 ) ) ;
#39373=DIRECTION ( 'NONE',  ( 0.9785564922995060311, 0.000000000000000000, -0.2059786187410889424 ) ) ;
#39374=ORIENTED_EDGE ( 'NONE', *, *, #27765, .T. ) ;
#39376=FACE_OUTER_BOUND ( 'NONE', #44878, .T. ) ;
#39378=VECTOR ( 'NONE', #42984, 1000.000000000000227 ) ;
#39379=PLANE ( 'NONE',  #47493 ) ;
#39380=VERTEX_POINT ( 'NONE', #5862 ) ;
#39381=FACE_OUTER_BOUND ( 'NONE', #24610, .T. ) ;
#39382=AXIS2_PLACEMENT_3D ( 'NONE', #24845, #30018, #28265 ) ;
#39386=CARTESIAN_POINT ( 'NONE',  ( -85.77912150413021664, -175.3837268820161057, -119.3051146910911768 ) ) ;
#39391=DIRECTION ( 'NONE',  ( -0.02963332782255633305, 0.000000000000000000, -0.9995608365087944591 ) ) ;
#39392=CARTESIAN_POINT ( 'NONE',  ( -91.84482189527193441, -175.3837268820161057, -117.2365833888816695 ) ) ;
#39394=DIRECTION ( 'NONE',  ( -0.000000000000000000, 1.000000000000000000, -0.000000000000000000 ) ) ;
#39395=CARTESIAN_POINT ( 'NONE',  ( 24.88090138098523241, -183.6283474603465606, 99.97252634603304955 ) ) ;
#39397=EDGE_CURVE ( 'NONE', #20913, #36158, #47949, .T. ) ;
#39398=EDGE_CURVE ( 'NONE', #32761, #49503, #9787, .T. ) ;
#39399=VERTEX_POINT ( 'NONE', #6113 ) ;
#39400=ADVANCED_FACE ( 'NONE', ( #21879 ), #21351, .T. ) ;
#39403=FACE_OUTER_BOUND ( 'NONE', #11257, .T. ) ;
#39407=CARTESIAN_POINT ( 'NONE',  ( 57.12946453413545100, -175.3837268820161057, 66.87170886602000053 ) ) ;
#39410=EDGE_CURVE ( 'NONE', #19952, #19715, #853, .T. ) ;
#39411=DIRECTION ( 'NONE',  ( 0.000000000000000000, 0.000000000000000000, 1.000000000000000000 ) ) ;
#39412=DIRECTION ( 'NONE',  ( -0.000000000000000000, 1.000000000000000000, -0.000000000000000000 ) ) ;
#39413=VERTEX_POINT ( 'NONE', #49220 ) ;
#39414=VERTEX_POINT ( 'NONE', #17433 ) ;
#39415=ADVANCED_FACE ( 'NONE', ( #1894 ), #17931, .T. ) ;
#39416=VERTEX_POINT ( 'NONE', #26065 ) ;
#39418=CARTESIAN_POINT ( 'NONE',  ( -171.7589556598192360, -183.6283474603465606, -13.35228579481114863 ) ) ;
#39420=VECTOR ( 'NONE', #45081, 1000.000000000000000 ) ;
#39422=CARTESIAN_POINT ( 'NONE',  ( -127.0132498732365889, -193.5000000000000000, 97.24912084693261249 ) ) ;
#39424=EDGE_CURVE ( 'NONE', #14713, #8278, #45534, .T. ) ;
#39426=DIRECTION ( 'NONE',  ( -0.000000000000000000, 1.000000000000000000, -0.000000000000000000 ) ) ;
#39427=VERTEX_POINT ( 'NONE', #25294 ) ;
#39428=ORIENTED_EDGE ( 'NONE', *, *, #34013, .T. ) ;
#39429=VERTEX_POINT ( 'NONE', #51043 ) ;
#39430=FACE_OUTER_BOUND ( 'NONE', #26080, .T. ) ;
#39431=CARTESIAN_POINT ( 'NONE',  ( -173.3968853974275817, -193.5000000000000000, 4.533605064404221174 ) ) ;
#39433=EDGE_CURVE ( 'NONE', #33166, #20294, #10817, .T. ) ;
#39434=CIRCLE ( 'NONE', #31078, 125.0000000000000000 ) ;
#39435=VECTOR ( 'NONE', #19010, 1000.000000000000000 ) ;
#39436=DIRECTION ( 'NONE',  ( -0.000000000000000000, 1.000000000000000000, 0.000000000000000000 ) ) ;
#39440=ORIENTED_EDGE ( 'NONE', *, *, #41298, .F. ) ;
#39441=CARTESIAN_POINT ( 'NONE',  ( -49.13194886969938580, -189.7472609257535510, 0.7575112421616214675 ) ) ;
#39444=VERTEX_POINT ( 'NONE', #47340 ) ;
#39447=DIRECTION ( 'NONE',  ( 0.000000000000000000, -0.000000000000000000, 1.000000000000000000 ) ) ;
#39448=DIRECTION ( 'NONE',  ( 0.000000000000000000, 0.000000000000000000, 1.000000000000000000 ) ) ;
#39449=ORIENTED_EDGE ( 'NONE', *, *, #42726, .F. ) ;
#39451=CARTESIAN_POINT ( 'NONE',  ( 61.98524708613674505, -177.1207230881787780, 56.33604425924833237 ) ) ;
#39452=DIRECTION ( 'NONE',  ( -0.000000000000000000, 1.000000000000000000, 0.000000000000000000 ) ) ;
#39453=( NAMED_UNIT ( * ) PLANE_ANGLE_UNIT ( ) SI_UNIT ( $, .RADIAN. ) );
#39454=VECTOR ( 'NONE', #450, 1000.000000000000000 ) ;
#39455=EDGE_LOOP ( 'NONE', ( #16168, #40603, #37122, #14796 ) ) ;
#39456=DIRECTION ( 'NONE',  ( -0.000000000000000000, 1.000000000000000000, -0.000000000000000000 ) ) ;
#39457=DIRECTION ( 'NONE',  ( 0.000000000000000000, 0.000000000000000000, -1.000000000000000000 ) ) ;
#39459=ADVANCED_FACE ( 'NONE', ( #26579 ), #15033, .T. ) ;
#39460=ADVANCED_FACE ( 'NONE', ( #34718 ), #31293, .T. ) ;
#39461=ORIENTED_EDGE ( 'NONE', *, *, #31463, .F. ) ;
#39462=ADVANCED_FACE ( 'NONE', ( #18192 ), #22130, .F. ) ;
#39463=FACE_OUTER_BOUND ( 'NONE', #44947, .T. ) ;
#39464=DIRECTION ( 'NONE',  ( 0.000000000000000000, 0.000000000000000000, -1.000000000000000000 ) ) ;
#39465=EDGE_CURVE ( 'NONE', #7505, #14417, #50768, .T. ) ;
#39468=EDGE_LOOP ( 'NONE', ( #31361, #48780, #51876, #30156 ) ) ;
#39469=DIRECTION ( 'NONE',  ( 0.4031234292879665171, 0.000000000000000000, 0.9151456172430210145 ) ) ;
#39471=FACE_OUTER_BOUND ( 'NONE', #27748, .T. ) ;
#39472=CARTESIAN_POINT ( 'NONE',  ( -91.22542124915045747, -175.3837268820161057, 117.4638425504669925 ) ) ;
#39474=CARTESIAN_POINT ( 'NONE',  ( -41.90263914168912152, -193.5000000000000000, -124.8268793598473536 ) ) ;
#39475=EDGE_CURVE ( 'NONE', #1228, #38434, #22649, .T. ) ;
#39476=VECTOR ( 'NONE', #31554, 1000.000000000000000 ) ;
#39478=VECTOR ( 'NONE', #573, 1000.000000000000000 ) ;
#39479=PLANE ( 'NONE',  #33003 ) ;
#39481=LINE ( 'NONE', #15853, #31194 ) ;
#39482=DIRECTION ( 'NONE',  ( 0.8858462335218260097, -0.000000000000000000, -0.4639789333096864810 ) ) ;
#39484=ORIENTED_EDGE ( 'NONE', *, *, #47204, .T. ) ;
#39485=EDGE_CURVE ( 'NONE', #13511, #30309, #26171, .T. ) ;
#39488=EDGE_CURVE ( 'NONE', #34611, #9242, #34985, .T. ) ;
#39489=DIRECTION ( 'NONE',  ( 0.000000000000000000, 1.000000000000000000, -0.000000000000000000 ) ) ;
#39491=ORIENTED_EDGE ( 'NONE', *, *, #23200, .T. ) ;
#39495=DIRECTION ( 'NONE',  ( -0.000000000000000000, 1.000000000000000000, -0.000000000000000000 ) ) ;
#39497=CARTESIAN_POINT ( 'NONE',  ( 69.14211578623219623, -183.6283474603465606, 42.31126686685117733 ) ) ;
#39500=ORIENTED_EDGE ( 'NONE', *, *, #17686, .F. ) ;
#39501=ORIENTED_EDGE ( 'NONE', *, *, #16517, .F. ) ;
#39502=ADVANCED_FACE ( 'NONE', ( #50262 ), #2664, .F. ) ;
#39504=DIRECTION ( 'NONE',  ( 0.4566292373937077542, 0.000000000000000000, 0.8896570909947499883 ) ) ;
#39505=DIRECTION ( 'NONE',  ( 0.9564009842765202052, 0.000000000000000000, 0.2920567706369833760 ) ) ;
#39506=CARTESIAN_POINT ( 'NONE',  ( -156.6671849566219805, -193.5000000000000000, 60.59166255800406731 ) ) ;
#39508=ORIENTED_EDGE ( 'NONE', *, *, #7612, .F. ) ;
#39509=VECTOR ( 'NONE', #42070, 1000.000000000000000 ) ;
#39511=CARTESIAN_POINT ( 'NONE',  ( -49.03777351731250889, -183.6283474603465606, 0.8294056854502042109 ) ) ;
#39512=AXIS2_PLACEMENT_3D ( 'NONE', #26493, #41483, #6278 ) ;
#39515=ORIENTED_EDGE ( 'NONE', *, *, #9225, .T. ) ;
#39516=DIRECTION ( 'NONE',  ( -0.000000000000000000, 1.000000000000000000, -0.000000000000000000 ) ) ;
#39517=DIRECTION ( 'NONE',  ( -0.3482016354343866471, 0.000000000000000000, -0.9374196611341253371 ) ) ;
#39519=FACE_OUTER_BOUND ( 'NONE', #21469, .T. ) ;
#39520=DIRECTION ( 'NONE',  ( 0.6965510290630033685, 0.000000000000000000, -0.7175072570443249420 ) ) ;
#39521=EDGE_CURVE ( 'NONE', #41796, #24186, #11057, .T. ) ;
#39523=ADVANCED_FACE ( 'NONE', ( #14511 ), #18704, .T. ) ;
#39524=ORIENTED_EDGE ( 'NONE', *, *, #46138, .F. ) ;
#39526=ORIENTED_EDGE ( 'NONE', *, *, #41242, .T. ) ;
#39528=VECTOR ( 'NONE', #23989, 1000.000000000000000 ) ;
#39529=PLANE ( 'NONE',  #27842 ) ;
#39531=DIRECTION ( 'NONE',  ( -0.000000000000000000, 1.000000000000000000, -0.000000000000000000 ) ) ;
#39532=DIRECTION ( 'NONE',  ( 0.000000000000000000, 1.000000000000000000, 0.000000000000000000 ) ) ;
#39534=FACE_OUTER_BOUND ( 'NONE', #17552, .T. ) ;
#39536=ORIENTED_EDGE ( 'NONE', *, *, #39397, .F. ) ;
#39537=ORIENTED_EDGE ( 'NONE', *, *, #36896, .F. ) ;
#39538=EDGE_CURVE ( 'NONE', #48929, #9685, #49085, .T. ) ;
#39539=DIRECTION ( 'NONE',  ( -0.000000000000000000, 1.000000000000000000, -0.000000000000000000 ) ) ;
#39541=ORIENTED_EDGE ( 'NONE', *, *, #42248, .F. ) ;
#39542=VECTOR ( 'NONE', #29849, 999.9999999999998863 ) ;
#39543=ORIENTED_EDGE ( 'NONE', *, *, #30282, .T. ) ;
#39544=CARTESIAN_POINT ( 'NONE',  ( 52.36832552120769435, -175.3837268820161057, -72.15117186584490128 ) ) ;
#39547=CARTESIAN_POINT ( 'NONE',  ( 67.42090074966655777, -175.3837268820161057, -46.82076062204441058 ) ) ;
#39548=VERTEX_POINT ( 'NONE', #28830 ) ;
#39554=CARTESIAN_POINT ( 'NONE',  ( 43.12693905415815010, -193.5000000000000000, -83.57229767764155781 ) ) ;
#39555=CARTESIAN_POINT ( 'NONE',  ( -70.75782287548088334, -189.7472609257535510, 122.9986166548864901 ) ) ;
#39557=CIRCLE ( 'NONE', #9387, 124.9999999999999858 ) ;
#39558=EDGE_LOOP ( 'NONE', ( #27614, #15888, #29614, #39501 ) ) ;
#39560=DIRECTION ( 'NONE',  ( -0.000000000000000000, 1.000000000000000000, -0.000000000000000000 ) ) ;
#39561=CARTESIAN_POINT ( 'NONE',  ( 38.48673058372652633, -189.7472609257535510, 88.39086586114804334 ) ) ;
#39564=DIRECTION ( 'NONE',  ( 0.000000000000000000, -0.000000000000000000, -1.000000000000000000 ) ) ;
#39565=CARTESIAN_POINT ( 'NONE',  ( 17.15229921100054611, -193.5000000000000000, -106.3838142112212921 ) ) ;
#39566=VERTEX_POINT ( 'NONE', #48836 ) ;
#39567=DIRECTION ( 'NONE',  ( 0.9890401873221644768, 0.000000000000000000, -0.1476465640024779702 ) ) ;
#39569=LINE ( 'NONE', #28775, #1296 ) ;
#39570=ORIENTED_EDGE ( 'NONE', *, *, #45282, .T. ) ;
#39572=DIRECTION ( 'NONE',  ( -0.000000000000000000, 1.000000000000000000, 0.000000000000000000 ) ) ;
#39573=CARTESIAN_POINT ( 'NONE',  ( 75.32224018181403835, -177.1207230881787780, 7.024906801079477958 ) ) ;
#39574=VECTOR ( 'NONE', #4768, 1000.000000000000000 ) ;
#39575=CARTESIAN_POINT ( 'NONE',  ( 50.88012955800436998, -193.5000000000000000, 74.18852968774250201 ) ) ;
#39577=LINE ( 'NONE', #3588, #28412 ) ;
#39581=ORIENTED_EDGE ( 'NONE', *, *, #24054, .T. ) ;
#39582=AXIS2_PLACEMENT_3D ( 'NONE', #14755, #41830, #23906 ) ;
#39583=EDGE_LOOP ( 'NONE', ( #43904, #31752, #42068, #41428 ) ) ;
#39584=LINE ( 'NONE', #48270, #42207 ) ;
#39587=FACE_OUTER_BOUND ( 'NONE', #2137, .T. ) ;
#39588=LINE ( 'NONE', #44585, #5402 ) ;
#39589=CYLINDRICAL_SURFACE ( 'NONE', #46383, 125.0000000000000000 ) ;
#39590=ORIENTED_EDGE ( 'NONE', *, *, #32052, .F. ) ;
#39591=LINE ( 'NONE', #31461, #37229 ) ;
#39593=AXIS2_PLACEMENT_3D ( 'NONE', #36063, #12659, #12402 ) ;
#39594=CARTESIAN_POINT ( 'NONE',  ( -48.47912675150885065, -189.7472609257535510, 6.938893903907228378E-15 ) ) ;
#39595=ORIENTED_EDGE ( 'NONE', *, *, #35602, .T. ) ;
#39596=VECTOR ( 'NONE', #44656, 1000.000000000000000 ) ;
#39600=DIRECTION ( 'NONE',  ( -0.3482016354343928088, 0.000000000000000000, -0.9374196611341231167 ) ) ;
#39601=VERTEX_POINT ( 'NONE', #40653 ) ;
#39602=FACE_OUTER_BOUND ( 'NONE', #37009, .T. ) ;
#39603=ORIENTED_EDGE ( 'NONE', *, *, #20750, .T. ) ;
#39605=FACE_BOUND ( 'NONE', #5126, .T. ) ;
#39607=VERTEX_POINT ( 'NONE', #17293 ) ;
#39608=AXIS2_PLACEMENT_3D ( 'NONE', #34932, #23123, #14992 ) ;
#39609=CARTESIAN_POINT ( 'NONE',  ( -88.78924379339714790, -177.1207230881787780, -118.3219948448692520 ) ) ;
#39611=VECTOR ( 'NONE', #35473, 1000.000000000000000 ) ;
#39612=EDGE_LOOP ( 'NONE', ( #25507, #25339, #25685, #31820 ) ) ;
#39614=ORIENTED_EDGE ( 'NONE', *, *, #17776, .T. ) ;
#39615=PLANE ( 'NONE',  #34300 ) ;
#39616=DIRECTION ( 'NONE',  ( -0.4031234292879600778, 0.000000000000000000, -0.9151456172430237901 ) ) ;
#39617=EDGE_CURVE ( 'NONE', #37719, #3202, #8545, .T. ) ;
#39620=ADVANCED_FACE ( 'NONE', ( #12807 ), #1239, .T. ) ;
#39621=CARTESIAN_POINT ( 'NONE',  ( -162.4844509910036265, -183.6283474603465606, -48.77484799213895172 ) ) ;
#39622=ORIENTED_EDGE ( 'NONE', *, *, #15048, .F. ) ;
#39624=DIRECTION ( 'NONE',  ( 0.000000000000000000, 0.000000000000000000, 1.000000000000000000 ) ) ;
#39625=VERTEX_POINT ( 'NONE', #8874 ) ;
#39626=VECTOR ( 'NONE', #9049, 1000.000000000000000 ) ;
#39629=VERTEX_POINT ( 'NONE', #13347 ) ;
#39630=CARTESIAN_POINT ( 'NONE',  ( 75.27070168362158142, -175.3837268820161057, 17.63462396184792524 ) ) ;
#39631=ORIENTED_EDGE ( 'NONE', *, *, #32240, .T. ) ;
#39634=VERTEX_POINT ( 'NONE', #3434 ) ;
#39635=DIRECTION ( 'NONE',  ( 0.000000000000000000, 0.000000000000000000, 1.000000000000000000 ) ) ;
#39636=CARTESIAN_POINT ( 'NONE',  ( -169.9131040279660283, -193.5000000000000000, 29.64437826672835996 ) ) ;
#39638=ADVANCED_FACE ( 'NONE', ( #24387 ), #41185, .T. ) ;
#39640=VERTEX_POINT ( 'NONE', #45164 ) ;
#39641=CARTESIAN_POINT ( 'NONE',  ( -47.47956591500005885, -183.6283474603465606, 0.02963332782257025594 ) ) ;
#39642=EDGE_CURVE ( 'NONE', #34518, #16239, #5209, .T. ) ;
#39643=DIRECTION ( 'NONE',  ( 0.000000000000000000, 1.000000000000000000, 0.000000000000000000 ) ) ;
#39644=DIRECTION ( 'NONE',  ( -0.8455960035018199594, 0.000000000000000000, -0.5338233779648003940 ) ) ;
#39648=FACE_OUTER_BOUND ( 'NONE', #48197, .T. ) ;
#39649=EDGE_LOOP ( 'NONE', ( #36159, #32542, #11185, #30089 ) ) ;
#39652=AXIS2_PLACEMENT_3D ( 'NONE', #2912, #34967, #51031 ) ;
#39653=PLANE ( 'NONE',  #28785 ) ;
#39657=DIRECTION ( 'NONE',  ( 0.000000000000000000, -1.000000000000000000, 0.000000000000000000 ) ) ;
#39659=ORIENTED_EDGE ( 'NONE', *, *, #34013, .F. ) ;
#39660=ORIENTED_EDGE ( 'NONE', *, *, #48027, .F. ) ;
#39661=AXIS2_PLACEMENT_3D ( 'NONE', #31264, #27059, #47057 ) ;
#39663=AXIS2_PLACEMENT_3D ( 'NONE', #48294, #39862, #24378 ) ;
#39664=AXIS2_PLACEMENT_3D ( 'NONE', #19972, #24684, #7874 ) ;
#39665=CARTESIAN_POINT ( 'NONE',  ( 72.05536924052414349, -193.5000000000000000, 33.11246405730899056 ) ) ;
#39668=DIRECTION ( 'NONE',  ( 0.5085311186492094127, 0.000000000000000000, 0.8610436117673619938 ) ) ;
#39669=LINE ( 'NONE', #2913, #40456 ) ;
#39670=ORIENTED_EDGE ( 'NONE', *, *, #38113, .T. ) ;
#39673=ORIENTED_EDGE ( 'NONE', *, *, #38110, .F. ) ;
#39675=CARTESIAN_POINT ( 'NONE',  ( -133.0671220150036334, -193.5000000000000000, -92.03190238880748097 ) ) ;
#39677=EDGE_CURVE ( 'NONE', #26704, #23694, #3523, .T. ) ;
#39679=VERTEX_POINT ( 'NONE', #4953 ) ;
#39682=CYLINDRICAL_SURFACE ( 'NONE', #41999, 125.0000000000000000 ) ;
#39685=ORIENTED_EDGE ( 'NONE', *, *, #23595, .F. ) ;
#39687=VERTEX_POINT ( 'NONE', #20973 ) ;
#39692=DIRECTION ( 'NONE',  ( -0.9473263538541946138, 0.000000000000000000, 0.3202698538628279690 ) ) ;
#39694=DIRECTION ( 'NONE',  ( 0.000000000000000000, 0.000000000000000000, 1.000000000000000000 ) ) ;
#39699=CIRCLE ( 'NONE', #16212, 125.0000000000000000 ) ;
#39700=FACE_OUTER_BOUND ( 'NONE', #33596, .T. ) ;
#39701=EDGE_CURVE ( 'NONE', #22526, #42721, #35406, .T. ) ;
#39702=ORIENTED_EDGE ( 'NONE', *, *, #28713, .T. ) ;
#39703=DIRECTION ( 'NONE',  ( -0.000000000000000000, 1.000000000000000000, -0.000000000000000000 ) ) ;
#39705=CARTESIAN_POINT ( 'NONE',  ( -162.9896759831412965, -183.6283474603465606, -50.12318939043964861 ) ) ;
#39706=EDGE_CURVE ( 'NONE', #31601, #4103, #34088, .T. ) ;
#39708=DIRECTION ( 'NONE',  ( 0.000000000000000000, 1.000000000000000000, 0.000000000000000000 ) ) ;
#39710=CARTESIAN_POINT ( 'NONE',  ( -172.9089226952081617, -193.5000000000000000, 11.92584929509620117 ) ) ;
#39714=CARTESIAN_POINT ( 'NONE',  ( -7.223120065443619175, -183.6283474603465606, 117.9955164924470523 ) ) ;
#39716=AXIS2_PLACEMENT_3D ( 'NONE', #3940, #23634, #12056 ) ;
#39717=CARTESIAN_POINT ( 'NONE',  ( -159.8192355313504152, -183.6283474603465606, -56.81883646197837834 ) ) ;
#39718=DIRECTION ( 'NONE',  ( 0.000000000000000000, 1.000000000000000000, 0.000000000000000000 ) ) ;
#39721=DIRECTION ( 'NONE',  ( -0.9960498426152158968, 0.000000000000000000, -0.08879589532294571153 ) ) ;
#39722=DIRECTION ( 'NONE',  ( -0.000000000000000000, 1.000000000000000000, -0.000000000000000000 ) ) ;
#39723=DIRECTION ( 'NONE',  ( 0.000000000000000000, 0.000000000000000000, -1.000000000000000000 ) ) ;
#39724=DIRECTION ( 'NONE',  ( -0.000000000000000000, 1.000000000000000000, -0.000000000000000000 ) ) ;
#39727=DIRECTION ( 'NONE',  ( 0.2348860457809775482, 0.000000000000000000, 0.9720229140804121926 ) ) ;
#39728=AXIS2_PLACEMENT_3D ( 'NONE', #3450, #43661, #23679 ) ;
#39730=PLANE ( 'NONE',  #27961 ) ;
#39731=EDGE_LOOP ( 'NONE', ( #4282, #21788, #18795, #18834 ) ) ;
#39733=DIRECTION ( 'NONE',  ( -0.9266896074318291543, 0.000000000000000000, -0.3758275821142488260 ) ) ;
#39734=ORIENTED_EDGE ( 'NONE', *, *, #51954, .F. ) ;
#39735=FACE_OUTER_BOUND ( 'NONE', #47391, .T. ) ;
#39739=EDGE_CURVE ( 'NONE', #6533, #46287, #49865, .T. ) ;
#39740=DIRECTION ( 'NONE',  ( 0.000000000000000000, -0.000000000000000000, -1.000000000000000000 ) ) ;
#39744=ADVANCED_FACE ( 'NONE', ( #50138 ), #6235, .T. ) ;
#39745=ORIENTED_EDGE ( 'NONE', *, *, #42340, .T. ) ;
#39746=DIRECTION ( 'NONE',  ( -0.000000000000000000, 1.000000000000000000, -0.000000000000000000 ) ) ;
#39750=DIRECTION ( 'NONE',  ( 0.000000000000000000, 0.000000000000000000, -1.000000000000000000 ) ) ;
#39753=ORIENTED_EDGE ( 'NONE', *, *, #3196, .T. ) ;
#39757=PLANE ( 'NONE',  #27403 ) ;
#39759=EDGE_CURVE ( 'NONE', #22186, #16764, #43774, .T. ) ;
#39761=ORIENTED_EDGE ( 'NONE', *, *, #1897, .F. ) ;
#39763=CARTESIAN_POINT ( 'NONE',  ( -89.44307666693794090, -183.6283474603465606, -117.0391155081702266 ) ) ;
#39764=EDGE_CURVE ( 'NONE', #51485, #51398, #41445, .T. ) ;
#39766=VERTEX_POINT ( 'NONE', #1513 ) ;
#39768=EDGE_CURVE ( 'NONE', #47058, #7135, #22252, .T. ) ;
#39769=CARTESIAN_POINT ( 'NONE',  ( -73.70588833648351113, -177.1207230881787780, 121.4073237908568359 ) ) ;
#39770=DIRECTION ( 'NONE',  ( 0.9374196611341231167, 0.000000000000000000, -0.3482016354343928088 ) ) ;
#39775=EDGE_CURVE ( 'NONE', #29802, #29776, #25428, .T. ) ;
#39776=VERTEX_POINT ( 'NONE', #18332 ) ;
#39777=LINE ( 'NONE', #12182, #38324 ) ;
#39778=CARTESIAN_POINT ( 'NONE',  ( -56.71246971489870958, -193.5000000000000000, -124.7285535218267682 ) ) ;
#39779=CARTESIAN_POINT ( 'NONE',  ( -48.47912675150885065, -189.7472609257535510, 6.938893903907228378E-15 ) ) ;
#39781=CARTESIAN_POINT ( 'NONE',  ( 74.80070215680143519, -177.1207230881787780, 13.35228579481199596 ) ) ;
#39782=CARTESIAN_POINT ( 'NONE',  ( 34.93559171950835918, -183.6283474603465606, -93.09664195018497423 ) ) ;
#39783=CARTESIAN_POINT ( 'NONE',  ( -71.22983192549011733, -175.3837268820161057, -121.8950816227732759 ) ) ;
#39784=CARTESIAN_POINT ( 'NONE',  ( 32.49319223169170812, -189.7472609257535510, -95.22858582633060109 ) ) ;
#39786=ORIENTED_EDGE ( 'NONE', *, *, #30191, .F. ) ;
#39787=CARTESIAN_POINT ( 'NONE',  ( -169.6719064342497632, -177.1207230881787780, 30.61552143554992256 ) ) ;
#39788=ORIENTED_EDGE ( 'NONE', *, *, #73, .F. ) ;
#39789=VERTEX_POINT ( 'NONE', #38278 ) ;
#39790=CARTESIAN_POINT ( 'NONE',  ( 24.88090138098524307, -193.5000000000000000, 99.97252634603304955 ) ) ;
#39791=DIRECTION ( 'NONE',  ( 0.000000000000000000, 0.000000000000000000, 1.000000000000000000 ) ) ;
#39792=EDGE_LOOP ( 'NONE', ( #22512, #5876, #36622, #39825 ) ) ;
#39793=CIRCLE ( 'NONE', #28022, 125.0000000000000000 ) ;
#39794=VECTOR ( 'NONE', #42304, 1000.000000000000000 ) ;
#39795=VERTEX_POINT ( 'NONE', #2020 ) ;
#39797=AXIS2_PLACEMENT_3D ( 'NONE', #5114, #33490, #37151 ) ;
#39799=EDGE_LOOP ( 'NONE', ( #43549, #50096, #744, #36247 ) ) ;
#39800=DIRECTION ( 'NONE',  ( -0.000000000000000000, 1.000000000000000000, -0.000000000000000000 ) ) ;
#39801=CARTESIAN_POINT ( 'NONE',  ( -49.42645310536304493, -193.5000000000000000, 0.3202698538628349079 ) ) ;
#39802=EDGE_LOOP ( 'NONE', ( #13576, #34293, #25281, #32629 ) ) ;
#39803=DIRECTION ( 'NONE',  ( -0.000000000000000000, 1.000000000000000000, -0.000000000000000000 ) ) ;
#39804=CARTESIAN_POINT ( 'NONE',  ( -117.8923552450419265, -189.7472609257535510, 102.7511748916629131 ) ) ;
#39805=EDGE_CURVE ( 'NONE', #47094, #4101, #2298, .T. ) ;
#39807=LINE ( 'NONE', #28760, #47092 ) ;
#39808=AXIS2_PLACEMENT_3D ( 'NONE', #148, #4356, #40094 ) ;
#39809=CARTESIAN_POINT ( 'NONE',  ( -47.57632892154310866, -193.5000000000000000, -0.4300652022765113491 ) ) ;
#39810=ORIENTED_EDGE ( 'NONE', *, *, #38553, .T. ) ;
#39811=VERTEX_POINT ( 'NONE', #50388 ) ;
#39814=EDGE_CURVE ( 'NONE', #840, #22277, #34541, .T. ) ;
#39815=DIRECTION ( 'NONE',  ( 0.5085311186492216251, 0.000000000000000000, -0.8610436117673548884 ) ) ;
#39816=CARTESIAN_POINT ( 'NONE',  ( -106.2948367055609964, -175.3837268820161057, -110.8257356506552327 ) ) ;
#39817=DIRECTION ( 'NONE',  ( 0.5586467658036415873, 0.000000000000000000, 0.8294056854502090959 ) ) ;
#39820=ORIENTED_EDGE ( 'NONE', *, *, #17657, .T. ) ;
#39822=ORIENTED_EDGE ( 'NONE', *, *, #46741, .T. ) ;
#39825=ORIENTED_EDGE ( 'NONE', *, *, #44293, .T. ) ;
#39826=VECTOR ( 'NONE', #30669, 1000.000000000000000 ) ;
#39828=DIRECTION ( 'NONE',  ( 0.4827922027307366970, 0.000000000000000000, 0.8757349421956412971 ) ) ;
#39830=AXIS2_PLACEMENT_3D ( 'NONE', #28393, #44442, #8428 ) ;
#39831=CIRCLE ( 'NONE', #17207, 125.0000000000000000 ) ;
#39832=CARTESIAN_POINT ( 'NONE',  ( 67.87295084395104539, -183.6283474603465606, 42.87565520599286373 ) ) ;
#39833=LINE ( 'NONE', #27509, #20055 ) ;
#39835=DIRECTION ( 'NONE',  ( -0.2920567706369833760, 0.000000000000000000, 0.9564009842765202052 ) ) ;
#39836=ORIENTED_EDGE ( 'NONE', *, *, #37635, .T. ) ;
#39837=VECTOR ( 'NONE', #51852, 1000.000000000000000 ) ;
#39838=ADVANCED_FACE ( 'NONE', ( #14911 ), #7531, .T. ) ;
#39840=LINE ( 'NONE', #4376, #11971 ) ;
#39844=CIRCLE ( 'NONE', #21411, 125.0000000000000000 ) ;
#39846=CARTESIAN_POINT ( 'NONE',  ( -47.70260288879080690, -175.3837268820161057, -0.6300878435817026668 ) ) ;
#39850=CARTESIAN_POINT ( 'NONE',  ( -81.70897914701313880, -177.1207230881787780, -120.5021863277716534 ) ) ;
#39851=DIRECTION ( 'NONE',  ( -0.000000000000000000, 1.000000000000000000, -0.000000000000000000 ) ) ;
#39852=FACE_BOUND ( 'NONE', #4492, .T. ) ;
#39853=VERTEX_POINT ( 'NONE', #31429 ) ;
#39855=DIRECTION ( 'NONE',  ( -0.000000000000000000, 1.000000000000000000, -0.000000000000000000 ) ) ;
#39856=ORIENTED_EDGE ( 'NONE', *, *, #46560, .T. ) ;
#39859=PLANE ( 'NONE',  #36019 ) ;
#39860=VECTOR ( 'NONE', #36562, 1000.000000000000114 ) ;
#39861=FACE_BOUND ( 'NONE', #52025, .T. ) ;
#39862=DIRECTION ( 'NONE',  ( 0.000000000000000000, -1.000000000000000000, 0.000000000000000000 ) ) ;
#39864=VECTOR ( 'NONE', #31637, 1000.000000000000227 ) ;
#39865=AXIS2_PLACEMENT_3D ( 'NONE', #10853, #51322, #7439 ) ;
#39868=EDGE_LOOP ( 'NONE', ( #21713, #43133, #8405, #22246 ) ) ;
#39870=ORIENTED_EDGE ( 'NONE', *, *, #5158, .T. ) ;
#39871=LINE ( 'NONE', #48302, #30930 ) ;
#39872=ORIENTED_EDGE ( 'NONE', *, *, #9348, .T. ) ;
#39873=CIRCLE ( 'NONE', #17254, 125.0000000000000000 ) ;
#39874=CARTESIAN_POINT ( 'NONE',  ( -171.7300019102062549, -183.6283474603465606, -20.83798868929510562 ) ) ;
#39876=CARTESIAN_POINT ( 'NONE',  ( -65.65563056894596627, -193.5000000000000000, 123.8142468240612999 ) ) ;
#39877=AXIS2_PLACEMENT_3D ( 'NONE', #4755, #48907, #16315 ) ;
#39878=VECTOR ( 'NONE', #42698, 1000.000000000000000 ) ;
#39880=LINE ( 'NONE', #43834, #40721 ) ;
#39883=CYLINDRICAL_SURFACE ( 'NONE', #42371, 125.0000000000000000 ) ;
#39887=CARTESIAN_POINT ( 'NONE',  ( -172.5669052183642123, -183.6283474603465606, 15.07392567185546994 ) ) ;
#39888=ORIENTED_EDGE ( 'NONE', *, *, #11162, .T. ) ;
#39889=DIRECTION ( 'NONE',  ( -0.7175072570443299380, 0.000000000000000000, -0.6965510290629983725 ) ) ;
#39890=VERTEX_POINT ( 'NONE', #31695 ) ;
#39892=EDGE_LOOP ( 'NONE', ( #20830, #15590, #4598, #35242 ) ) ;
#39893=CYLINDRICAL_SURFACE ( 'NONE', #42571, 15.00000000000000000 ) ;
#39894=DIRECTION ( 'NONE',  ( -0.000000000000000000, 1.000000000000000000, 0.000000000000000000 ) ) ;
#39895=ORIENTED_EDGE ( 'NONE', *, *, #33007, .F. ) ;
#39896=ADVANCED_FACE ( 'NONE', ( #6759 ), #11720, .T. ) ;
#39897=CARTESIAN_POINT ( 'NONE',  ( 26.52087324849106054, -173.5000000000000284, -70.00000000000002842 ) ) ;
#39898=ORIENTED_EDGE ( 'NONE', *, *, #32946, .T. ) ;
#39899=CARTESIAN_POINT ( 'NONE',  ( -49.38192458147459263, -193.5000000000000000, -0.4300652022765235616 ) ) ;
#39900=VECTOR ( 'NONE', #47833, 1000.000000000000000 ) ;
#39901=FACE_OUTER_BOUND ( 'NONE', #42388, .T. ) ;
#39902=CARTESIAN_POINT ( 'NONE',  ( 46.01898237923986557, -193.5000000000000000, -81.82363577055902226 ) ) ;
#39904=CARTESIAN_POINT ( 'NONE',  ( -101.0675409952200283, -183.6283474603465606, 113.3995532942340958 ) ) ;
#39906=FACE_OUTER_BOUND ( 'NONE', #24161, .T. ) ;
#39907=AXIS2_PLACEMENT_3D ( 'NONE', #32105, #48149, #12122 ) ;
#39908=ORIENTED_EDGE ( 'NONE', *, *, #20800, .T. ) ;
#39910=PLANE ( 'NONE',  #39716 ) ;
#39911=LINE ( 'NONE', #28085, #36576 ) ;
#39912=CARTESIAN_POINT ( 'NONE',  ( 19.33815737959698566, -177.1207230881787780, 105.0038855142078233 ) ) ;
#39913=EDGE_LOOP ( 'NONE', ( #44253, #45811, #43740, #42932 ) ) ;
#39915=AXIS2_PLACEMENT_3D ( 'NONE', #46141, #19481, #3710 ) ;
#39917=CARTESIAN_POINT ( 'NONE',  ( -172.6359455740846158, -183.6283474603465606, -14.49428645563797069 ) ) ;
#39920=VERTEX_POINT ( 'NONE', #46967 ) ;
#39921=AXIS2_PLACEMENT_3D ( 'NONE', #17392, #8699, #40745 ) ;
#39922=ORIENTED_EDGE ( 'NONE', *, *, #47437, .F. ) ;
#39924=CIRCLE ( 'NONE', #5569, 125.0000000000000000 ) ;
#39926=DIRECTION ( 'NONE',  ( 0.8896570909947499883, 0.000000000000000000, -0.4566292373937077542 ) ) ;
#39927=DIRECTION ( 'NONE',  ( -0.8610436117673621048, 0.000000000000000000, 0.5085311186492095237 ) ) ;
#39929=ORIENTED_EDGE ( 'NONE', *, *, #42856, .F. ) ;
#39933=ORIENTED_EDGE ( 'NONE', *, *, #27910, .T. ) ;
#39935=VECTOR ( 'NONE', #31462, 1000.000000000000000 ) ;
#39936=VECTOR ( 'NONE', #24605, 1000.000000000000000 ) ;
#39938=CARTESIAN_POINT ( 'NONE',  ( 34.93559171950835918, -177.1207230881787780, -93.09664195018497423 ) ) ;
#39940=AXIS2_PLACEMENT_3D ( 'NONE', #35778, #48669, #47632 ) ;
#39941=ORIENTED_EDGE ( 'NONE', *, *, #12778, .F. ) ;
#39942=CARTESIAN_POINT ( 'NONE',  ( -47.51449116960048968, -189.7472609257535510, 0.2635871660690785045 ) ) ;
#39947=VECTOR ( 'NONE', #48401, 1000.000000000000000 ) ;
#39948=ADVANCED_FACE ( 'NONE', ( #47471 ), #27219, .T. ) ;
#39949=VECTOR ( 'NONE', #45200, 1000.000000000000000 ) ;
#39952=AXIS2_PLACEMENT_3D ( 'NONE', #37790, #37545, #34871 ) ;
#39955=EDGE_LOOP ( 'NONE', ( #30397, #27963, #39670, #12199 ) ) ;
#39956=CARTESIAN_POINT ( 'NONE',  ( -123.0610352593084400, -189.7472609257535510, 99.06333546307732263 ) ) ;
#39960=DIRECTION ( 'NONE',  ( -0.000000000000000000, 1.000000000000000000, -0.000000000000000000 ) ) ;
#39963=DIRECTION ( 'NONE',  ( 0.6965510290629982615, 0.000000000000000000, -0.7175072570443298270 ) ) ;
#39964=PLANE ( 'NONE',  #16948 ) ;
#39965=CARTESIAN_POINT ( 'NONE',  ( -37.67038537088846084, -193.5000000000000000, -124.5318076226586470 ) ) ;
#39966=VERTEX_POINT ( 'NONE', #19357 ) ;
#39967=DIRECTION ( 'NONE',  ( 0.000000000000000000, 1.000000000000000000, 0.000000000000000000 ) ) ;
#39968=CARTESIAN_POINT ( 'NONE',  ( -151.4272465800706016, -183.6283474603465606, 70.89911581792887318 ) ) ;
#39973=DIRECTION ( 'NONE',  ( -0.8610436117673548884, 0.000000000000000000, -0.5085311186492216251 ) ) ;
#39974=ORIENTED_EDGE ( 'NONE', *, *, #13061, .F. ) ;
#39977=LINE ( 'NONE', #16624, #34040 ) ;
#39979=VECTOR ( 'NONE', #9927, 1000.000000000000000 ) ;
#39980=DIRECTION ( 'NONE',  ( 0.000000000000000000, -1.000000000000000000, -0.000000000000000000 ) ) ;
#39981=ADVANCED_FACE ( 'NONE', ( #43776 ), #35119, .T. ) ;
#39984=ADVANCED_FACE ( 'NONE', ( #3573 ), #7269, .F. ) ;
#39986=VECTOR ( 'NONE', #32205, 1000.000000000000114 ) ;
#39988=DIRECTION ( 'NONE',  ( -0.000000000000000000, 1.000000000000000000, -0.000000000000000000 ) ) ;
#39989=DIRECTION ( 'NONE',  ( 0.000000000000000000, -1.000000000000000000, 0.000000000000000000 ) ) ;
#39993=CIRCLE ( 'NONE', #22384, 125.0000000000000000 ) ;
#39994=EDGE_LOOP ( 'NONE', ( #27020, #23577, #28036, #33382 ) ) ;
#39995=CARTESIAN_POINT ( 'NONE',  ( -142.2007120195389405, -193.5000000000000000, 81.19354792697798473 ) ) ;
#39997=AXIS2_PLACEMENT_3D ( 'NONE', #18262, #46900, #5665 ) ;
#39998=EDGE_CURVE ( 'NONE', #12264, #47175, #33766, .T. ) ;
#40001=VERTEX_POINT ( 'NONE', #4891 ) ;
#40007=CARTESIAN_POINT ( 'NONE',  ( -48.47912675150885065, -189.7472609257535510, 6.938893903907228378E-15 ) ) ;
#40008=CARTESIAN_POINT ( 'NONE',  ( -41.30311180514221547, -175.3837268820161057, 123.7921848946937899 ) ) ;
#40009=ORIENTED_EDGE ( 'NONE', *, *, #43642, .T. ) ;
#40013=DIRECTION ( 'NONE',  ( -0.000000000000000000, 1.000000000000000000, -0.000000000000000000 ) ) ;
#40014=CIRCLE ( 'NONE', #5656, 125.0000000000000000 ) ;
#40015=LINE ( 'NONE', #50843, #577 ) ;
#40017=DIRECTION ( 'NONE',  ( -0.8757349421956412971, 0.000000000000000000, 0.4827922027307366970 ) ) ;
#40020=CARTESIAN_POINT ( 'NONE',  ( -114.9600645115007040, -193.5000000000000000, 105.8550183720738573 ) ) ;
#40021=VECTOR ( 'NONE', #28686, 1000.000000000000000 ) ;
#40024=DIRECTION ( 'NONE',  ( -0.000000000000000000, 1.000000000000000000, -0.000000000000000000 ) ) ;
#40026=EDGE_LOOP ( 'NONE', ( #6316, #5414, #14423, #48900 ) ) ;
#40027=VECTOR ( 'NONE', #39746, 1000.000000000000000 ) ;
#40028=VERTEX_POINT ( 'NONE', #10368 ) ;
#40030=LINE ( 'NONE', #16142, #42620 ) ;
#40031=ORIENTED_EDGE ( 'NONE', *, *, #39998, .T. ) ;
#40036=ORIENTED_EDGE ( 'NONE', *, *, #10104, .T. ) ;
#40039=AXIS2_PLACEMENT_3D ( 'NONE', #11786, #35706, #3392 ) ;
#40041=CARTESIAN_POINT ( 'NONE',  ( -48.47912675150885065, -183.6283474603465606, 6.938893903907228378E-15 ) ) ;
#40042=VERTEX_POINT ( 'NONE', #18006 ) ;
#40043=DIRECTION ( 'NONE',  ( 0.000000000000000000, 1.000000000000000000, 0.000000000000000000 ) ) ;
#40044=FACE_OUTER_BOUND ( 'NONE', #26336, .T. ) ;
#40045=ORIENTED_EDGE ( 'NONE', *, *, #45908, .F. ) ;
#40047=LINE ( 'NONE', #12458, #18158 ) ;
#40048=EDGE_CURVE ( 'NONE', #21919, #51603, #22476, .T. ) ;
#40049=DIRECTION ( 'NONE',  ( 0.5085311186492154079, 0.000000000000000000, 0.8610436117673585521 ) ) ;
#40050=CARTESIAN_POINT ( 'NONE',  ( -43.48323084606168720, -193.5000000000000000, 124.9001241957026167 ) ) ;
#40051=EDGE_CURVE ( 'NONE', #44024, #27852, #18273, .T. ) ;
#40052=DIRECTION ( 'NONE',  ( -0.000000000000000000, 1.000000000000000000, -0.000000000000000000 ) ) ;
#40053=EDGE_CURVE ( 'NONE', #10162, #50250, #30373, .T. ) ;
#40054=VERTEX_POINT ( 'NONE', #6445 ) ;
#40056=EDGE_CURVE ( 'NONE', #5333, #10177, #50331, .T. ) ;
#40057=ORIENTED_EDGE ( 'NONE', *, *, #17296, .T. ) ;
#40058=EDGE_LOOP ( 'NONE', ( #25754, #35057, #50274, #1175 ) ) ;
#40059=AXIS2_PLACEMENT_3D ( 'NONE', #22790, #15173, #27229 ) ;
#40063=FACE_OUTER_BOUND ( 'NONE', #12761, .T. ) ;
#40064=ORIENTED_EDGE ( 'NONE', *, *, #36239, .T. ) ;
#40065=EDGE_CURVE ( 'NONE', #39601, #33164, #14319, .T. ) ;
#40068=CARTESIAN_POINT ( 'NONE',  ( 27.23560471289042439, -189.7472609257535510, 99.45993886622848379 ) ) ;
#40069=ADVANCED_FACE ( 'NONE', ( #49559 ), #42161, .F. ) ;
#40070=ADVANCED_FACE ( 'NONE', ( #37445 ), #13285, .F. ) ;
#40071=FACE_OUTER_BOUND ( 'NONE', #43575, .T. ) ;
#40072=AXIS2_PLACEMENT_3D ( 'NONE', #47460, #4097, #20366 ) ;
#40073=ORIENTED_EDGE ( 'NONE', *, *, #24366, .F. ) ;
#40076=AXIS2_PLACEMENT_3D ( 'NONE', #8686, #12882, #17109 ) ;
#40077=CARTESIAN_POINT ( 'NONE',  ( -5.113431607746556473, -175.3837268820161057, 117.2365833888819537 ) ) ;
#40078=ORIENTED_EDGE ( 'NONE', *, *, #25723, .T. ) ;
#40079=LINE ( 'NONE', #20111, #48506 ) ;
#40080=FACE_OUTER_BOUND ( 'NONE', #42551, .T. ) ;
#40085=DIRECTION ( 'NONE',  ( 0.2920567706369694982, 0.000000000000000000, 0.9564009842765243130 ) ) ;
#40087=ORIENTED_EDGE ( 'NONE', *, *, #195, .T. ) ;
#40088=EDGE_LOOP ( 'NONE', ( #8815, #24310, #20246, #36439 ) ) ;
#40089=VECTOR ( 'NONE', #33638, 999.9999999999998863 ) ;
#40090=FACE_OUTER_BOUND ( 'NONE', #5408, .T. ) ;
#40091=FACE_OUTER_BOUND ( 'NONE', #37184, .T. ) ;
#40092=DIRECTION ( 'NONE',  ( 0.000000000000000000, 0.000000000000000000, 1.000000000000000000 ) ) ;
#40094=DIRECTION ( 'NONE',  ( 0.000000000000000000, 0.000000000000000000, 1.000000000000000000 ) ) ;
#40095=VERTEX_POINT ( 'NONE', #1178 ) ;
#40097=DIRECTION ( 'NONE',  ( -0.000000000000000000, 1.000000000000000000, -0.000000000000000000 ) ) ;
#40099=DIRECTION ( 'NONE',  ( 0.000000000000000000, -1.000000000000000000, 0.000000000000000000 ) ) ;
#40100=ORIENTED_EDGE ( 'NONE', *, *, #44337, .F. ) ;
#40101=VECTOR ( 'NONE', #874, 1000.000000000000000 ) ;
#40103=VECTOR ( 'NONE', #45373, 1000.000000000000000 ) ;
#40104=CARTESIAN_POINT ( 'NONE',  ( -158.9435005891548371, -193.5000000000000000, -56.33604425924755077 ) ) ;
#40105=DIRECTION ( 'NONE',  ( 0.000000000000000000, 0.000000000000000000, 1.000000000000000000 ) ) ;
#40106=CIRCLE ( 'NONE', #40932, 125.0000000000000000 ) ;
#40107=CARTESIAN_POINT ( 'NONE',  ( -49.13194886969938580, -193.5000000000000000, 0.7575112421616214675 ) ) ;
#40108=CARTESIAN_POINT ( 'NONE',  ( -49.47868758801764955, -175.3837268820161057, 0.02963332782255607284 ) ) ;
#40109=ORIENTED_EDGE ( 'NONE', *, *, #36515, .T. ) ;
#40112=EDGE_CURVE ( 'NONE', #34695, #32136, #14071, .T. ) ;
#40113=ORIENTED_EDGE ( 'NONE', *, *, #37088, .T. ) ;
#40114=DIRECTION ( 'NONE',  ( -0.000000000000000000, 1.000000000000000000, 0.000000000000000000 ) ) ;
#40115=AXIS2_PLACEMENT_3D ( 'NONE', #37310, #34147, #25748 ) ;
#40117=CARTESIAN_POINT ( 'NONE',  ( -48.47912675150885065, -183.6283474603465606, 6.938893903907228378E-15 ) ) ;
#40119=EDGE_CURVE ( 'NONE', #49227, #27750, #16973, .T. ) ;
#40121=CARTESIAN_POINT ( 'NONE',  ( -20.16057156355605784, -175.3837268820161057, -120.7230919990158782 ) ) ;
#40122=ADVANCED_FACE ( 'NONE', ( #6183 ), #33520, .F. ) ;
#40123=ORIENTED_EDGE ( 'NONE', *, *, #26750, .F. ) ;
#40126=EDGE_CURVE ( 'NONE', #34274, #39306, #5238, .T. ) ;
#40127=CIRCLE ( 'NONE', #7435, 125.0000000000000000 ) ;
#40128=FACE_BOUND ( 'NONE', #27701, .T. ) ;
#40129=EDGE_LOOP ( 'NONE', ( #48269, #48542, #3250, #45589 ) ) ;
#40130=CARTESIAN_POINT ( 'NONE',  ( -46.12632737020502560, -193.5000000000000000, -123.9784823535113532 ) ) ;
#40131=DIRECTION ( 'NONE',  ( 0.000000000000000000, 0.000000000000000000, -1.000000000000000000 ) ) ;
#40132=ORIENTED_EDGE ( 'NONE', *, *, #9604, .F. ) ;
#40135=ORIENTED_EDGE ( 'NONE', *, *, #26364, .F. ) ;
#40137=CARTESIAN_POINT ( 'NONE',  ( 27.42205759510523677, -193.5000000000000000, 98.05618656931996213 ) ) ;
#40138=VECTOR ( 'NONE', #41338, 1000.000000000000000 ) ;
#40139=ADVANCED_FACE ( 'NONE', ( #15356 ), #38490, .T. ) ;
#40141=FACE_BOUND ( 'NONE', #31756, .T. ) ;
#40143=ORIENTED_EDGE ( 'NONE', *, *, #39302, .T. ) ;
#40145=EDGE_CURVE ( 'NONE', #32545, #50673, #42693, .T. ) ;
#40147=ORIENTED_EDGE ( 'NONE', *, *, #49630, .F. ) ;
#40149=ORIENTED_EDGE ( 'NONE', *, *, #5396, .F. ) ;
#40150=DIRECTION ( 'NONE',  ( -0.000000000000000000, -1.000000000000000000, 0.000000000000000000 ) ) ;
#40151=VECTOR ( 'NONE', #22529, 1000.000000000000000 ) ;
#40152=ORIENTED_EDGE ( 'NONE', *, *, #7419, .F. ) ;
#40153=DIRECTION ( 'NONE',  ( 0.000000000000000000, 0.000000000000000000, -1.000000000000000000 ) ) ;
#40154=CARTESIAN_POINT ( 'NONE',  ( 67.04262753014327814, -189.7472609257535510, -47.74645837849745078 ) ) ;
#40156=EDGE_CURVE ( 'NONE', #48767, #30683, #38774, .T. ) ;
#40159=EDGE_LOOP ( 'NONE', ( #5605, #3114, #2716, #34891 ) ) ;
#40162=ORIENTED_EDGE ( 'NONE', *, *, #22600, .T. ) ;
#40163=EDGE_LOOP ( 'NONE', ( #24382, #44045, #9790, #19600 ) ) ;
#40166=PLANE ( 'NONE',  #7949 ) ;
#40167=ORIENTED_EDGE ( 'NONE', *, *, #37879, .T. ) ;
#40168=FACE_OUTER_BOUND ( 'NONE', #18427, .T. ) ;
#40169=EDGE_LOOP ( 'NONE', ( #10330, #2359, #23865, #17198 ) ) ;
#40170=CARTESIAN_POINT ( 'NONE',  ( -111.3295483157475445, -189.7472609257535510, 108.0501018472332504 ) ) ;
#40172=ORIENTED_EDGE ( 'NONE', *, *, #10991, .T. ) ;
#40174=FACE_OUTER_BOUND ( 'NONE', #48745, .T. ) ;
#40175=VECTOR ( 'NONE', #10582, 1000.000000000000000 ) ;
#40176=CARTESIAN_POINT ( 'NONE',  ( -72.96029774493611342, -193.5000000000000000, 122.5792489240759409 ) ) ;
#40179=LINE ( 'NONE', #48070, #39230 ) ;
#40180=CARTESIAN_POINT ( 'NONE',  ( -48.47912675150885065, -183.6283474603465606, 6.938893903907228378E-15 ) ) ;
#40182=AXIS2_PLACEMENT_3D ( 'NONE', #25752, #41785, #20773 ) ;
#40183=FACE_OUTER_BOUND ( 'NONE', #28985, .T. ) ;
#40184=ORIENTED_EDGE ( 'NONE', *, *, #29528, .F. ) ;
#40185=EDGE_CURVE ( 'NONE', #46675, #13353, #6701, .T. ) ;
#40187=CARTESIAN_POINT ( 'NONE',  ( -149.5539421794694022, -189.7472609257535510, 73.54509967498655953 ) ) ;
#40188=DIRECTION ( 'NONE',  ( -0.9995608365087946812, 0.000000000000000000, 0.02963332782254913048 ) ) ;
#40190=EDGE_LOOP ( 'NONE', ( #12737, #31715, #224, #38429 ) ) ;
#40191=VECTOR ( 'NONE', #2006, 1000.000000000000114 ) ;
#40192=DIRECTION ( 'NONE',  ( 0.000000000000000000, 0.000000000000000000, -1.000000000000000000 ) ) ;
#40193=DIRECTION ( 'NONE',  ( 0.000000000000000000, 0.000000000000000000, 1.000000000000000000 ) ) ;
#40195=ORIENTED_EDGE ( 'NONE', *, *, #5860, .T. ) ;
#40197=ORIENTED_EDGE ( 'NONE', *, *, #45212, .T. ) ;
#40199=CARTESIAN_POINT ( 'NONE',  ( -154.6193097927903182, -193.5000000000000000, -66.02470404298122730 ) ) ;
#40200=DIRECTION ( 'NONE',  ( 0.000000000000000000, -1.000000000000000000, -0.000000000000000000 ) ) ;
#40202=LINE ( 'NONE', #12341, #6117 ) ;
#40204=ORIENTED_EDGE ( 'NONE', *, *, #13541, .F. ) ;
#40205=DIRECTION ( 'NONE',  ( -0.7575112421616284619, 0.000000000000000000, 0.6528221181905119463 ) ) ;
#40206=EDGE_CURVE ( 'NONE', #14560, #5201, #38729, .T. ) ;
#40212=ORIENTED_EDGE ( 'NONE', *, *, #12754, .T. ) ;
#40213=DIRECTION ( 'NONE',  ( 0.000000000000000000, 0.000000000000000000, -1.000000000000000000 ) ) ;
#40218=DIRECTION ( 'NONE',  ( 0.000000000000000000, 0.000000000000000000, -1.000000000000000000 ) ) ;
#40219=EDGE_LOOP ( 'NONE', ( #33667, #36073, #2778, #28223 ) ) ;
#40221=VERTEX_POINT ( 'NONE', #23244 ) ;
#40222=CARTESIAN_POINT ( 'NONE',  ( -48.53836737940257251, -175.3837268820161057, 0.9982437317643279018 ) ) ;
#40223=LINE ( 'NONE', #4239, #51508 ) ;
#40224=CARTESIAN_POINT ( 'NONE',  ( 7.859956736328458149, -189.7472609257535510, -111.5836353223468649 ) ) ;
#40227=AXIS2_PLACEMENT_3D ( 'NONE', #22991, #35077, #23509 ) ;
#40230=VERTEX_POINT ( 'NONE', #7473 ) ;
#40231=DIRECTION ( 'NONE',  ( 0.8124868780056783146, 0.000000000000000000, 0.5829794791144762289 ) ) ;
#40234=ORIENTED_EDGE ( 'NONE', *, *, #13683, .F. ) ;
#40235=EDGE_CURVE ( 'NONE', #32301, #17165, #2736, .T. ) ;
#40236=DIRECTION ( 'NONE',  ( 0.6068001458186002006, 0.000000000000000000, -0.7948544414133481562 ) ) ;
#40237=CARTESIAN_POINT ( 'NONE',  ( -72.96029774493611342, -183.6283474603465606, 122.5792489240759409 ) ) ;
#40238=ORIENTED_EDGE ( 'NONE', *, *, #14684, .F. ) ;
#40239=PLANE ( 'NONE',  #29620 ) ;
#40240=ORIENTED_EDGE ( 'NONE', *, *, #25440, .F. ) ;
#40242=DIRECTION ( 'NONE',  ( 0.000000000000000000, -1.000000000000000000, 0.000000000000000000 ) ) ;
#40243=DIRECTION ( 'NONE',  ( 0.000000000000000000, -0.000000000000000000, 1.000000000000000000 ) ) ;
#40244=LINE ( 'NONE', #7169, #32777 ) ;
#40245=CARTESIAN_POINT ( 'NONE',  ( -48.30223647638628393, -189.7472609257535510, 0.9842305779476049343 ) ) ;
#40246=LINE ( 'NONE', #28939, #24924 ) ;
#40247=CARTESIAN_POINT ( 'NONE',  ( -15.81236726369127155, -183.6283474603465606, -120.6560517527615559 ) ) ;
#40248=CARTESIAN_POINT ( 'NONE',  ( -166.8403286750647680, -175.3837268820161057, -40.19484891389966918 ) ) ;
#40249=EDGE_CURVE ( 'NONE', #42721, #51264, #10630, .T. ) ;
#40252=ORIENTED_EDGE ( 'NONE', *, *, #28354, .T. ) ;
#40253=VERTEX_POINT ( 'NONE', #47679 ) ;
#40255=VECTOR ( 'NONE', #18824, 1000.000000000000000 ) ;
#40256=CIRCLE ( 'NONE', #47009, 125.0000000000000000 ) ;
#40258=ORIENTED_EDGE ( 'NONE', *, *, #19149, .F. ) ;
#40259=VERTEX_POINT ( 'NONE', #27159 ) ;
#40260=VERTEX_POINT ( 'NONE', #39263 ) ;
#40267=LINE ( 'NONE', #35306, #36714 ) ;
#40268=DIRECTION ( 'NONE',  ( 0.7378332790417333475, 0.000000000000000000, -0.6749830015182038956 ) ) ;
#40270=EDGE_LOOP ( 'NONE', ( #13759, #3485, #18564, #29981 ) ) ;
#40274=EDGE_LOOP ( 'NONE', ( #35780, #50651, #49099, #39933 ) ) ;
#40275=DIRECTION ( 'NONE',  ( 0.000000000000000000, -0.000000000000000000, 1.000000000000000000 ) ) ;
#40276=ADVANCED_FACE ( 'NONE', ( #43717 ), #18772, .T. ) ;
#40277=CARTESIAN_POINT ( 'NONE',  ( 33.09766481721657527, -193.5000000000000000, 93.38753978496653474 ) ) ;
#40278=LINE ( 'NONE', #47684, #20623 ) ;
#40279=DIRECTION ( 'NONE',  ( 0.9785564922995017012, 0.000000000000000000, 0.2059786187411094538 ) ) ;
#40280=EDGE_CURVE ( 'NONE', #31839, #41498, #6094, .T. ) ;
#40281=ORIENTED_EDGE ( 'NONE', *, *, #29075, .T. ) ;
#40282=VERTEX_POINT ( 'NONE', #26908 ) ;
#40283=ORIENTED_EDGE ( 'NONE', *, *, #3213, .T. ) ;
#40284=DIRECTION ( 'NONE',  ( 0.000000000000000000, -1.000000000000000000, 0.000000000000000000 ) ) ;
#40286=VERTEX_POINT ( 'NONE', #38986 ) ;
#40287=DIRECTION ( 'NONE',  ( 0.000000000000000000, 1.000000000000000000, -0.000000000000000000 ) ) ;
#40288=FACE_OUTER_BOUND ( 'NONE', #32713, .T. ) ;
#40289=ORIENTED_EDGE ( 'NONE', *, *, #32604, .F. ) ;
#40291=CARTESIAN_POINT ( 'NONE',  ( -14.52059121095390815, -193.5000000000000000, 119.2602935412682541 ) ) ;
#40292=ADVANCED_FACE ( 'NONE', ( #15108 ), #31111, .T. ) ;
#40295=EDGE_LOOP ( 'NONE', ( #14989, #49690, #12781, #35134 ) ) ;
#40296=DIRECTION ( 'NONE',  ( -0.9151456172430237901, 0.000000000000000000, 0.4031234292879600778 ) ) ;
#40301=CARTESIAN_POINT ( 'NONE',  ( 21.47984469475713354, -189.7472609257535510, 102.3804074221065292 ) ) ;
#40302=ORIENTED_EDGE ( 'NONE', *, *, #25153, .F. ) ;
#40304=DIRECTION ( 'NONE',  ( -0.9842305779475992722, 0.000000000000000000, 0.1768902751225592818 ) ) ;
#40309=ORIENTED_EDGE ( 'NONE', *, *, #28852, .F. ) ;
#40311=CIRCLE ( 'NONE', #28574, 125.0000000000000000 ) ;
#40312=CARTESIAN_POINT ( 'NONE',  ( -48.36085358058748795, -193.5000000000000000, 0.9929810960135245779 ) ) ;
#40313=DIRECTION ( 'NONE',  ( 0.000000000000000000, -0.000000000000000000, 1.000000000000000000 ) ) ;
#40315=ORIENTED_EDGE ( 'NONE', *, *, #35608, .F. ) ;
#40316=LINE ( 'NONE', #380, #11413 ) ;
#40318=ORIENTED_EDGE ( 'NONE', *, *, #30096, .T. ) ;
#40321=VERTEX_POINT ( 'NONE', #40797 ) ;
#40323=DIRECTION ( 'NONE',  ( -0.000000000000000000, 1.000000000000000000, -0.000000000000000000 ) ) ;
#40325=CARTESIAN_POINT ( 'NONE',  ( 2.066935079424590871, -189.7472609257535510, -114.3245189510257660 ) ) ;
#40326=DIRECTION ( 'NONE',  ( -0.000000000000000000, 1.000000000000000000, -0.000000000000000000 ) ) ;
#40328=EDGE_LOOP ( 'NONE', ( #13028, #25864, #4673, #50452 ) ) ;
#40329=VECTOR ( 'NONE', #22879, 1000.000000000000114 ) ;
#40330=ORIENTED_EDGE ( 'NONE', *, *, #22703, .F. ) ;
#40337=ADVANCED_FACE ( 'NONE', ( #16127 ), #51882, .T. ) ;
#40338=EDGE_CURVE ( 'NONE', #14481, #9782, #36344, .T. ) ;
#40339=VERTEX_POINT ( 'NONE', #32666 ) ;
#40340=DIRECTION ( 'NONE',  ( 0.000000000000000000, -0.000000000000000000, 1.000000000000000000 ) ) ;
#40342=VERTEX_POINT ( 'NONE', #3768 ) ;
#40344=CARTESIAN_POINT ( 'NONE',  ( 50.27798938500057346, -177.1207230881787780, 74.98773087994526065 ) ) ;
#40345=EDGE_CURVE ( 'NONE', #4350, #19912, #31887, .T. ) ;
#40349=ORIENTED_EDGE ( 'NONE', *, *, #22523, .T. ) ;
#40351=DIRECTION ( 'NONE',  ( -0.000000000000000000, 1.000000000000000000, -0.000000000000000000 ) ) ;
#40353=EDGE_CURVE ( 'NONE', #33115, #33038, #44498, .T. ) ;
#40355=CARTESIAN_POINT ( 'NONE',  ( -147.0463339291295881, -183.6283474603465606, 76.87330921200150158 ) ) ;
#40358=CARTESIAN_POINT ( 'NONE',  ( -172.9089226952081901, -189.7472609257535510, 11.92584929509617986 ) ) ;
#40360=VECTOR ( 'NONE', #34698, 1000.000000000000000 ) ;
#40362=CARTESIAN_POINT ( 'NONE',  ( -166.6265240196292439, -175.3837268820161057, 40.81902153125349031 ) ) ;
#40366=CARTESIAN_POINT ( 'NONE',  ( -67.22356632362124174, -193.5000000000000000, -123.5865930638409509 ) ) ;
#40368=DIRECTION ( 'NONE',  ( 0.000000000000000000, -1.000000000000000000, 0.000000000000000000 ) ) ;
#40369=FACE_BOUND ( 'NONE', #43177, .T. ) ;
#40374=EDGE_LOOP ( 'NONE', ( #2671, #43131, #10546, #47110 ) ) ;
#40375=LINE ( 'NONE', #4395, #11998 ) ;
#40376=ORIENTED_EDGE ( 'NONE', *, *, #32203, .T. ) ;
#40379=VECTOR ( 'NONE', #50834, 1000.000000000000000 ) ;
#40381=CARTESIAN_POINT ( 'NONE',  ( -127.4665351220365324, -183.6283474603465606, -96.88131563365297438 ) ) ;
#40383=DIRECTION ( 'NONE',  ( -0.000000000000000000, 1.000000000000000000, -0.000000000000000000 ) ) ;
#40386=EDGE_CURVE ( 'NONE', #31640, #20084, #35829, .T. ) ;
#40387=DIRECTION ( 'NONE',  ( 0.000000000000000000, -0.000000000000000000, -1.000000000000000000 ) ) ;
#40388=ORIENTED_EDGE ( 'NONE', *, *, #330, .F. ) ;
#40390=DIRECTION ( 'NONE',  ( 0.000000000000000000, -1.000000000000000000, 0.000000000000000000 ) ) ;
#40391=DIRECTION ( 'NONE',  ( 0.000000000000000000, -0.000000000000000000, -1.000000000000000000 ) ) ;
#40392=CIRCLE ( 'NONE', #26982, 125.0000000000000000 ) ;
#40393=EDGE_CURVE ( 'NONE', #23372, #3704, #82, .T. ) ;
#40395=ADVANCED_FACE ( 'NONE', ( #32397 ), #20575, .T. ) ;
#40399=VECTOR ( 'NONE', #48421, 1000.000000000000000 ) ;
#40403=DIRECTION ( 'NONE',  ( -0.000000000000000000, 1.000000000000000000, -0.000000000000000000 ) ) ;
#40404=PLANE ( 'NONE',  #48271 ) ;
#40406=VERTEX_POINT ( 'NONE', #39418 ) ;
#40407=EDGE_CURVE ( 'NONE', #885, #38237, #32104, .T. ) ;
#40408=DIRECTION ( 'NONE',  ( 0.000000000000000000, -0.000000000000000000, 1.000000000000000000 ) ) ;
#40409=ORIENTED_EDGE ( 'NONE', *, *, #47421, .T. ) ;
#40411=ORIENTED_EDGE ( 'NONE', *, *, #6815, .F. ) ;
#40413=CARTESIAN_POINT ( 'NONE',  ( 69.66827051661184100, -189.7472609257535510, -40.81902153125260213 ) ) ;
#40415=EDGE_CURVE ( 'NONE', #4396, #13513, #12818, .T. ) ;
#40416=FACE_OUTER_BOUND ( 'NONE', #50988, .T. ) ;
#40417=LINE ( 'NONE', #12310, #18293 ) ;
#40418=ORIENTED_EDGE ( 'NONE', *, *, #3817, .F. ) ;
#40419=VECTOR ( 'NONE', #14044, 1000.000000000000114 ) ;
#40420=ADVANCED_FACE ( 'NONE', ( #15800 ), #42849, .F. ) ;
#40423=DIRECTION ( 'NONE',  ( -0.000000000000000000, 1.000000000000000000, -0.000000000000000000 ) ) ;
#40425=EDGE_CURVE ( 'NONE', #20084, #26704, #31535, .T. ) ;
#40429=DIRECTION ( 'NONE',  ( 0.000000000000000000, -1.000000000000000000, 0.000000000000000000 ) ) ;
#40434=DIRECTION ( 'NONE',  ( -0.000000000000000000, -1.000000000000000000, 0.000000000000000000 ) ) ;
#40436=DIRECTION ( 'NONE',  ( 0.000000000000000000, 1.000000000000000000, -0.000000000000000000 ) ) ;
#40437=ORIENTED_EDGE ( 'NONE', *, *, #6366, .F. ) ;
#40440=CARTESIAN_POINT ( 'NONE',  ( -172.1341525481710164, -175.3837268820161057, 18.28755301364338237 ) ) ;
#40443=ORIENTED_EDGE ( 'NONE', *, *, #10403, .T. ) ;
#40444=VECTOR ( 'NONE', #43999, 1000.000000000000000 ) ;
#40447=VECTOR ( 'NONE', #43885, 1000.000000000000227 ) ;
#40448=ADVANCED_FACE ( 'NONE', ( #43108 ), #18942, .T. ) ;
#40449=PLANE ( 'NONE',  #25924 ) ;
#40451=CARTESIAN_POINT ( 'NONE',  ( -155.4121128832437364, -177.1207230881787780, -62.78108192021941392 ) ) ;
#40452=DIRECTION ( 'NONE',  ( 0.4031234292879665171, 0.000000000000000000, 0.9151456172430210145 ) ) ;
#40453=ORIENTED_EDGE ( 'NONE', *, *, #24963, .F. ) ;
#40455=DIRECTION ( 'NONE',  ( 0.000000000000000000, 1.000000000000000000, 0.000000000000000000 ) ) ;
#40456=VECTOR ( 'NONE', #18946, 1000.000000000000000 ) ;
#40458=VERTEX_POINT ( 'NONE', #43382 ) ;
#40459=AXIS2_PLACEMENT_3D ( 'NONE', #40077, #51666, #9266 ) ;
#40461=ORIENTED_EDGE ( 'NONE', *, *, #34906, .F. ) ;
#40462=DIRECTION ( 'NONE',  ( 0.6965510290629932655, 0.000000000000000000, 0.7175072570443347120 ) ) ;
#40463=EDGE_CURVE ( 'NONE', #24385, #34100, #50581, .T. ) ;
#40466=ADVANCED_FACE ( 'NONE', ( #27071 ), #7117, .F. ) ;
#40467=CARTESIAN_POINT ( 'NONE',  ( 75.60865171534658202, -193.5000000000000000, -15.07392567185468124 ) ) ;
#40468=PLANE ( 'NONE',  #50428 ) ;
#40469=DIRECTION ( 'NONE',  ( -0.4827922027307551267, 0.000000000000000000, 0.8757349421956311941 ) ) ;
#40470=DIRECTION ( 'NONE',  ( -0.000000000000000000, 1.000000000000000000, 0.000000000000000000 ) ) ;
#40471=ORIENTED_EDGE ( 'NONE', *, *, #32362, .F. ) ;
#40474=CARTESIAN_POINT ( 'NONE',  ( -11.80936624585914707, -175.3837268820161057, -119.5003291395395735 ) ) ;
#40475=VECTOR ( 'NONE', #32556, 1000.000000000000000 ) ;
#40477=ORIENTED_EDGE ( 'NONE', *, *, #48436, .T. ) ;
#40478=DIRECTION ( 'NONE',  ( 0.000000000000000000, -1.000000000000000000, 0.000000000000000000 ) ) ;
#40479=CARTESIAN_POINT ( 'NONE',  ( -140.0851925571752474, -175.3837268820161057, 83.57229767764225414 ) ) ;
#40481=CARTESIAN_POINT ( 'NONE',  ( 26.62880456707183896, -189.7472609257535510, 98.66508442481513441 ) ) ;
#40484=PLANE ( 'NONE',  #39921 ) ;
#40485=CARTESIAN_POINT ( 'NONE',  ( 60.90550954139435902, -193.5000000000000000, 60.49794494914085874 ) ) ;
#40486=LINE ( 'NONE', #11612, #20831 ) ;
#40487=ORIENTED_EDGE ( 'NONE', *, *, #17818, .F. ) ;
#40488=DIRECTION ( 'NONE',  ( 0.000000000000000000, -1.000000000000000000, 0.000000000000000000 ) ) ;
#40490=DIRECTION ( 'NONE',  ( 0.000000000000000000, 1.000000000000000000, 0.000000000000000000 ) ) ;
#40491=VERTEX_POINT ( 'NONE', #43883 ) ;
#40492=DIRECTION ( 'NONE',  ( 0.000000000000000000, -1.000000000000000000, 0.000000000000000000 ) ) ;
#40493=AXIS2_PLACEMENT_3D ( 'NONE', #19649, #20169, #3892 ) ;
#40494=DIRECTION ( 'NONE',  ( 0.000000000000000000, 0.000000000000000000, -1.000000000000000000 ) ) ;
#40497=ORIENTED_EDGE ( 'NONE', *, *, #43916, .T. ) ;
#40498=DIRECTION ( 'NONE',  ( 0.9960498426152171181, 0.000000000000000000, -0.08879589532293157006 ) ) ;
#40499=ORIENTED_EDGE ( 'NONE', *, *, #12417, .T. ) ;
#40500=CIRCLE ( 'NONE', #47248, 124.9999999999999858 ) ;
#40501=AXIS2_PLACEMENT_3D ( 'NONE', #38454, #14818, #50039 ) ;
#40502=DIRECTION ( 'NONE',  ( -0.000000000000000000, 1.000000000000000000, 0.000000000000000000 ) ) ;
#40506=DIRECTION ( 'NONE',  ( 0.000000000000000000, 1.000000000000000000, -0.000000000000000000 ) ) ;
#40507=DIRECTION ( 'NONE',  ( -0.000000000000000000, 1.000000000000000000, -0.000000000000000000 ) ) ;
#40510=LINE ( 'NONE', #62, #1829 ) ;
#40511=ORIENTED_EDGE ( 'NONE', *, *, #2099, .F. ) ;
#40512=VECTOR ( 'NONE', #36170, 1000.000000000000000 ) ;
#40513=ORIENTED_EDGE ( 'NONE', *, *, #16048, .F. ) ;
#40514=DIRECTION ( 'NONE',  ( -0.9027978299657477557, 0.000000000000000000, 0.4300652022765115712 ) ) ;
#40515=VECTOR ( 'NONE', #42143, 1000.000000000000000 ) ;
#40516=DIRECTION ( 'NONE',  ( 0.4031234292879665171, 0.000000000000000000, 0.9151456172430210145 ) ) ;
#40517=ORIENTED_EDGE ( 'NONE', *, *, #46422, .F. ) ;
#40520=DIRECTION ( 'NONE',  ( -0.8455960035018272869, 0.000000000000000000, 0.5338233779647886257 ) ) ;
#40521=EDGE_CURVE ( 'NONE', #42748, #50890, #30767, .T. ) ;
#40525=ORIENTED_EDGE ( 'NONE', *, *, #20358, .F. ) ;
#40526=VECTOR ( 'NONE', #42204, 1000.000000000000000 ) ;
#40527=EDGE_LOOP ( 'NONE', ( #38526, #5779, #3116, #24256 ) ) ;
#40529=LINE ( 'NONE', #20306, #19085 ) ;
#40530=LINE ( 'NONE', #20571, #26872 ) ;
#40533=AXIS2_PLACEMENT_3D ( 'NONE', #26049, #49717, #1876 ) ;
#40535=DIRECTION ( 'NONE',  ( 0.000000000000000000, 0.000000000000000000, -1.000000000000000000 ) ) ;
#40537=DIRECTION ( 'NONE',  ( 0.000000000000000000, 0.000000000000000000, -1.000000000000000000 ) ) ;
#40538=VECTOR ( 'NONE', #46676, 1000.000000000000114 ) ;
#40539=LINE ( 'NONE', #4557, #31642 ) ;
#40540=DIRECTION ( 'NONE',  ( -0.000000000000000000, 1.000000000000000000, -0.000000000000000000 ) ) ;
#40541=FACE_OUTER_BOUND ( 'NONE', #33630, .T. ) ;
#40542=ORIENTED_EDGE ( 'NONE', *, *, #40767, .T. ) ;
#40544=CARTESIAN_POINT ( 'NONE',  ( -127.0132498732365889, -177.1207230881787780, 97.24912084693261249 ) ) ;
#40545=DIRECTION ( 'NONE',  ( -0.000000000000000000, 1.000000000000000000, -0.000000000000000000 ) ) ;
#40546=ORIENTED_EDGE ( 'NONE', *, *, #44767, .T. ) ;
#40548=LINE ( 'NONE', #16144, #24029 ) ;
#40549=CIRCLE ( 'NONE', #32158, 125.0000000000000000 ) ;
#40550=CARTESIAN_POINT ( 'NONE',  ( -47.57632892154310866, -189.7472609257535510, -0.4300652022765113491 ) ) ;
#40551=VERTEX_POINT ( 'NONE', #13297 ) ;
#40554=AXIS2_PLACEMENT_3D ( 'NONE', #2134, #38912, #26570 ) ;
#40555=ORIENTED_EDGE ( 'NONE', *, *, #44788, .F. ) ;
#40556=CARTESIAN_POINT ( 'NONE',  ( 14.94072793302542124, -193.5000000000000000, 107.7168604805791574 ) ) ;
#40558=FACE_OUTER_BOUND ( 'NONE', #51162, .T. ) ;
#40559=EDGE_CURVE ( 'NONE', #34133, #19374, #5273, .T. ) ;
#40561=CARTESIAN_POINT ( 'NONE',  ( -48.59739992243022755, -177.1207230881787780, 0.9929810960135230236 ) ) ;
#40562=CARTESIAN_POINT ( 'NONE',  ( -95.18697522258266019, -177.1207230881787780, 115.9455772817713353 ) ) ;
#40563=DIRECTION ( 'NONE',  ( -0.000000000000000000, 1.000000000000000000, -0.000000000000000000 ) ) ;
#40565=CIRCLE ( 'NONE', #7012, 125.0000000000000000 ) ;
#40566=DIRECTION ( 'NONE',  ( 0.000000000000000000, -1.000000000000000000, -0.000000000000000000 ) ) ;
#40567=ORIENTED_EDGE ( 'NONE', *, *, #24891, .F. ) ;
#40568=CARTESIAN_POINT ( 'NONE',  ( -48.47912675150885065, -175.3837268820161057, 6.938893903907228378E-15 ) ) ;
#40569=EDGE_LOOP ( 'NONE', ( #29811, #30476, #16417, #18561 ) ) ;
#40570=ORIENTED_EDGE ( 'NONE', *, *, #26241, .F. ) ;
#40571=CIRCLE ( 'NONE', #45636, 125.0000000000000000 ) ;
#40572=LINE ( 'NONE', #12204, #8496 ) ;
#40573=CARTESIAN_POINT ( 'NONE',  ( 73.50869128264329788, -193.5000000000000000, -22.25084316132035056 ) ) ;
#40575=ORIENTED_EDGE ( 'NONE', *, *, #37755, .F. ) ;
#40576=CARTESIAN_POINT ( 'NONE',  ( -47.70260288879081401, -175.3837268820161057, 0.6300878435817218737 ) ) ;
#40577=ADVANCED_FACE ( 'NONE', ( #9357 ), #13023, .T. ) ;
#40578=DIRECTION ( 'NONE',  ( 0.7575112421616145841, 0.000000000000000000, 0.6528221181905280446 ) ) ;
#40580=CARTESIAN_POINT ( 'NONE',  ( -134.9734323446613189, -193.5000000000000000, 88.85232316304893629 ) ) ;
#40582=DIRECTION ( 'NONE',  ( -0.8455960035018199594, 0.000000000000000000, -0.5338233779648003940 ) ) ;
#40583=CARTESIAN_POINT ( 'NONE',  ( -172.0839188101925004, -175.3837268820161057, -18.62405380494756812 ) ) ;
#40584=CIRCLE ( 'NONE', #15448, 125.0000000000000000 ) ;
#40585=EDGE_CURVE ( 'NONE', #16507, #27859, #37930, .T. ) ;
#40587=DIRECTION ( 'NONE',  ( 0.000000000000000000, 0.000000000000000000, 1.000000000000000000 ) ) ;
#40588=EDGE_LOOP ( 'NONE', ( #40240, #11127, #43612, #40 ) ) ;
#40591=AXIS2_PLACEMENT_3D ( 'NONE', #6537, #30424, #46731 ) ;
#40594=CARTESIAN_POINT ( 'NONE',  ( -169.2746641285359317, -189.7472609257535510, -32.14713283941905786 ) ) ;
#40595=ADVANCED_FACE ( 'NONE', ( #1411 ), #25849, .T. ) ;
#40601=ORIENTED_EDGE ( 'NONE', *, *, #8613, .F. ) ;
#40603=ORIENTED_EDGE ( 'NONE', *, *, #30622, .F. ) ;
#40604=ORIENTED_EDGE ( 'NONE', *, *, #12465, .T. ) ;
#40605=DIRECTION ( 'NONE',  ( 0.000000000000000000, 0.000000000000000000, 1.000000000000000000 ) ) ;
#40607=LINE ( 'NONE', #8317, #19940 ) ;
#40609=CARTESIAN_POINT ( 'NONE',  ( -38.66762320617017679, -177.1207230881787780, -124.6143426664033740 ) ) ;
#40610=ORIENTED_EDGE ( 'NONE', *, *, #35090, .F. ) ;
#40612=EDGE_LOOP ( 'NONE', ( #46057, #16427, #33626, #41337 ) ) ;
#40613=VERTEX_POINT ( 'NONE', #25083 ) ;
#40614=DIRECTION ( 'NONE',  ( 0.000000000000000000, -1.000000000000000000, -0.000000000000000000 ) ) ;
#40615=CARTESIAN_POINT ( 'NONE',  ( -33.52607327456453135, -189.7472609257535510, -124.1024020384603119 ) ) ;
#40616=FACE_OUTER_BOUND ( 'NONE', #43391, .T. ) ;
#40620=LINE ( 'NONE', #4138, #50705 ) ;
#40622=ORIENTED_EDGE ( 'NONE', *, *, #48204, .F. ) ;
#40623=DIRECTION ( 'NONE',  ( 0.000000000000000000, -1.000000000000000000, 0.000000000000000000 ) ) ;
#40624=CARTESIAN_POINT ( 'NONE',  ( -48.47912675150885065, -177.1207230881787780, 6.938893903907228378E-15 ) ) ;
#40625=CIRCLE ( 'NONE', #21366, 125.0000000000000000 ) ;
#40626=EDGE_CURVE ( 'NONE', #48534, #18665, #28753, .T. ) ;
#40628=FACE_BOUND ( 'NONE', #24255, .T. ) ;
#40629=ORIENTED_EDGE ( 'NONE', *, *, #5972, .T. ) ;
#40630=LINE ( 'NONE', #8846, #5519 ) ;
#40632=CARTESIAN_POINT ( 'NONE',  ( -145.4373324222574126, -175.3837268820161057, -78.89300572996837957 ) ) ;
#40633=EDGE_CURVE ( 'NONE', #21155, #38288, #33485, .T. ) ;
#40634=ORIENTED_EDGE ( 'NONE', *, *, #22236, .F. ) ;
#40635=EDGE_CURVE ( 'NONE', #26640, #11081, #46098, .T. ) ;
#40637=AXIS2_PLACEMENT_3D ( 'NONE', #21166, #8548, #37446 ) ;
#40638=ORIENTED_EDGE ( 'NONE', *, *, #11245, .T. ) ;
#40639=DIRECTION ( 'NONE',  ( 0.000000000000000000, -0.000000000000000000, -1.000000000000000000 ) ) ;
#40640=DIRECTION ( 'NONE',  ( -0.000000000000000000, 1.000000000000000000, -0.000000000000000000 ) ) ;
#40644=LINE ( 'NONE', #4668, #39454 ) ;
#40645=ORIENTED_EDGE ( 'NONE', *, *, #31099, .F. ) ;
#40646=ADVANCED_FACE ( 'NONE', ( #9557 ), #28990, .T. ) ;
#40647=EDGE_LOOP ( 'NONE', ( #5489, #29682, #40622, #7960 ) ) ;
#40648=CARTESIAN_POINT ( 'NONE',  ( 59.70893145360470555, -175.3837268820161057, -60.59166255800331413 ) ) ;
#40649=ADVANCED_FACE ( 'NONE', ( #41602 ), #25329, .T. ) ;
#40650=ORIENTED_EDGE ( 'NONE', *, *, #26559, .F. ) ;
#40651=CARTESIAN_POINT ( 'NONE',  ( 62.13187335169531167, -183.6283474603465606, -58.22548115875872554 ) ) ;
#40652=VECTOR ( 'NONE', #17113, 1000.000000000000000 ) ;
#40653=CARTESIAN_POINT ( 'NONE',  ( -33.86391487983340909, -189.7472609257535510, 124.1426420773540684 ) ) ;
#40654=DIRECTION ( 'NONE',  ( 0.000000000000000000, 0.000000000000000000, -1.000000000000000000 ) ) ;
#40655=EDGE_CURVE ( 'NONE', #18230, #7739, #5365, .T. ) ;
#40656=CIRCLE ( 'NONE', #37302, 125.0000000000000000 ) ;
#40657=AXIS2_PLACEMENT_3D ( 'NONE', #19139, #51210, #7309 ) ;
#40658=FACE_OUTER_BOUND ( 'NONE', #43655, .T. ) ;
#40659=DIRECTION ( 'NONE',  ( 0.000000000000000000, 0.000000000000000000, -1.000000000000000000 ) ) ;
#40663=ORIENTED_EDGE ( 'NONE', *, *, #29590, .T. ) ;
#40665=AXIS2_PLACEMENT_3D ( 'NONE', #43332, #2613, #3382 ) ;
#40667=ORIENTED_EDGE ( 'NONE', *, *, #42031, .T. ) ;
#40669=ORIENTED_EDGE ( 'NONE', *, *, #10006, .F. ) ;
#40670=LINE ( 'NONE', #16799, #12022 ) ;
#40671=CARTESIAN_POINT ( 'NONE',  ( -49.08592689732745384, -183.6283474603465606, 0.7948544414133550395 ) ) ;
#40672=ORIENTED_EDGE ( 'NONE', *, *, #21997, .T. ) ;
#40674=CARTESIAN_POINT ( 'NONE',  ( -21.64528618042744412, -183.6283474603465606, 121.0625654437174887 ) ) ;
#40676=ORIENTED_EDGE ( 'NONE', *, *, #17202, .F. ) ;
#40677=ORIENTED_EDGE ( 'NONE', *, *, #27666, .T. ) ;
#40678=PLANE ( 'NONE',  #31257 ) ;
#40679=CARTESIAN_POINT ( 'NONE',  ( 73.03012110230136500, -175.3837268820161057, 24.72869175143112130 ) ) ;
#40680=FACE_OUTER_BOUND ( 'NONE', #40159, .T. ) ;
#40687=LINE ( 'NONE', #37798, #14765 ) ;
#40688=PLANE ( 'NONE',  #42221 ) ;
#40689=ORIENTED_EDGE ( 'NONE', *, *, #43507, .F. ) ;
#40690=VERTEX_POINT ( 'NONE', #37407 ) ;
#40691=AXIS2_PLACEMENT_3D ( 'NONE', #23570, #39341, #8504 ) ;
#40693=EDGE_CURVE ( 'NONE', #47251, #24620, #17467, .T. ) ;
#40694=VECTOR ( 'NONE', #29372, 1000.000000000000000 ) ;
#40695=AXIS2_PLACEMENT_3D ( 'NONE', #3601, #7803, #44342 ) ;
#40698=CARTESIAN_POINT ( 'NONE',  ( 66.11593792271145276, -175.3837268820161057, -47.37063079638321739 ) ) ;
#40699=ADVANCED_FACE ( 'NONE', ( #25858 ), #30560, .F. ) ;
#40700=VERTEX_POINT ( 'NONE', #6415 ) ;
#40703=ORIENTED_EDGE ( 'NONE', *, *, #27879, .F. ) ;
#40704=EDGE_CURVE ( 'NONE', #12031, #2659, #10342, .T. ) ;
#40705=CARTESIAN_POINT ( 'NONE',  ( 76.51419089073348800, -177.1207230881787780, -1.292495564988658030 ) ) ;
#40706=ADVANCED_FACE ( 'NONE', ( #18237 ), #22692, .F. ) ;
#40707=LINE ( 'NONE', #8408, #13598 ) ;
#40708=CIRCLE ( 'NONE', #8011, 125.0000000000000000 ) ;
#40709=LINE ( 'NONE', #28625, #37155 ) ;
#40710=DIRECTION ( 'NONE',  ( 0.000000000000000000, 0.000000000000000000, -1.000000000000000000 ) ) ;
#40711=VECTOR ( 'NONE', #11647, 1000.000000000000000 ) ;
#40713=DIRECTION ( 'NONE',  ( -0.000000000000000000, 1.000000000000000000, -0.000000000000000000 ) ) ;
#40714=EDGE_CURVE ( 'NONE', #49553, #17248, #6135, .T. ) ;
#40716=FACE_OUTER_BOUND ( 'NONE', #42778, .T. ) ;
#40719=CARTESIAN_POINT ( 'NONE',  ( 67.42090074966655777, -193.5000000000000000, -46.82076062204441058 ) ) ;
#40721=VECTOR ( 'NONE', #47541, 1000.000000000000000 ) ;
#40723=ORIENTED_EDGE ( 'NONE', *, *, #45278, .F. ) ;
#40725=EDGE_CURVE ( 'NONE', #2935, #22714, #1942, .T. ) ;
#40726=EDGE_CURVE ( 'NONE', #30974, #1806, #24565, .T. ) ;
#40729=CARTESIAN_POINT ( 'NONE',  ( -47.50057025920934706, -177.1207230881787780, -0.2059786187410884151 ) ) ;
#40730=DIRECTION ( 'NONE',  ( 0.4639789333096864810, 0.000000000000000000, -0.8858462335218260097 ) ) ;
#40733=CARTESIAN_POINT ( 'NONE',  ( -48.47912675150885065, -175.3837268820161057, 6.938893903907228378E-15 ) ) ;
#40735=ORIENTED_EDGE ( 'NONE', *, *, #22114, .F. ) ;
#40736=CARTESIAN_POINT ( 'NONE',  ( 62.59443091842027940, -177.1207230881787780, -57.33816169485140790 ) ) ;
#40737=DIRECTION ( 'NONE',  ( 0.000000000000000000, -0.000000000000000000, 1.000000000000000000 ) ) ;
#40739=VECTOR ( 'NONE', #13702, 999.9999999999998863 ) ;
#40741=CARTESIAN_POINT ( 'NONE',  ( 61.98524708613674505, -183.6283474603465606, 56.33604425924833237 ) ) ;
#40742=CARTESIAN_POINT ( 'NONE',  ( -166.8403286750647680, -189.7472609257535510, -40.19484891389974734 ) ) ;
#40743=EDGE_CURVE ( 'NONE', #49730, #7246, #48931, .T. ) ;
#40744=ORIENTED_EDGE ( 'NONE', *, *, #14766, .T. ) ;
#40745=DIRECTION ( 'NONE',  ( -0.9785564922995046988, 0.000000000000000000, 0.2059786187410953262 ) ) ;
#40746=DIRECTION ( 'NONE',  ( 0.000000000000000000, 0.000000000000000000, -1.000000000000000000 ) ) ;
#40748=ORIENTED_EDGE ( 'NONE', *, *, #8285, .T. ) ;
#40749=DIRECTION ( 'NONE',  ( -0.6749830015182091136, 0.000000000000000000, -0.7378332790417285736 ) ) ;
#40751=VECTOR ( 'NONE', #41156, 1000.000000000000114 ) ;
#40752=LINE ( 'NONE', #16615, #23209 ) ;
#40755=DIRECTION ( 'NONE',  ( 0.000000000000000000, 1.000000000000000000, 0.000000000000000000 ) ) ;
#40758=VERTEX_POINT ( 'NONE', #26633 ) ;
#40760=ORIENTED_EDGE ( 'NONE', *, *, #19596, .T. ) ;
#40762=CARTESIAN_POINT ( 'NONE',  ( -149.5539421794694022, -193.5000000000000000, 73.54509967498655953 ) ) ;
#40763=ADVANCED_FACE ( 'NONE', ( #14295 ), #13773, .T. ) ;
#40764=DIRECTION ( 'NONE',  ( -0.9266896074318343723, 0.000000000000000000, 0.3758275821142357809 ) ) ;
#40765=CARTESIAN_POINT ( 'NONE',  ( 33.25242634436024503, -175.3837268820161057, -94.57776286494160445 ) ) ;
#40767=EDGE_CURVE ( 'NONE', #32626, #47580, #17982, .T. ) ;
#40768=EDGE_CURVE ( 'NONE', #10121, #20252, #30834, .T. ) ;
#40769=CARTESIAN_POINT ( 'NONE',  ( -72.72541169915514558, -193.5000000000000000, 121.6072260099955287 ) ) ;
#40771=LINE ( 'NONE', #49202, #990 ) ;
#40772=DIRECTION ( 'NONE',  ( 0.000000000000000000, 0.000000000000000000, 1.000000000000000000 ) ) ;
#40773=FACE_OUTER_BOUND ( 'NONE', #496, .T. ) ;
#40775=CIRCLE ( 'NONE', #14811, 125.0000000000000000 ) ;
#40777=CARTESIAN_POINT ( 'NONE',  ( 61.22907552172956258, -193.5000000000000000, -57.79541595648221630 ) ) ;
#40782=VECTOR ( 'NONE', #1694, 1000.000000000000000 ) ;
#40783=ORIENTED_EDGE ( 'NONE', *, *, #30282, .F. ) ;
#40787=DIRECTION ( 'NONE',  ( -0.8124868780056863082, 0.000000000000000000, 0.5829794791144649047 ) ) ;
#40788=AXIS2_PLACEMENT_3D ( 'NONE', #38100, #9743, #22611 ) ;
#40789=DIRECTION ( 'NONE',  ( -0.000000000000000000, 1.000000000000000000, -0.000000000000000000 ) ) ;
#40790=VERTEX_POINT ( 'NONE', #50555 ) ;
#40791=EDGE_LOOP ( 'NONE', ( #42466, #26405, #44057, #44243 ) ) ;
#40793=VECTOR ( 'NONE', #40024, 1000.000000000000000 ) ;
#40794=DIRECTION ( 'NONE',  ( -0.9982437317643214625, 0.000000000000000000, -0.05924062789371441901 ) ) ;
#40795=PLANE ( 'NONE',  #20771 ) ;
#40797=CARTESIAN_POINT ( 'NONE',  ( 7.859956736328458149, -175.3837268820161057, -111.5836353223468649 ) ) ;
#40798=DIRECTION ( 'NONE',  ( 0.000000000000000000, 0.000000000000000000, 1.000000000000000000 ) ) ;
#40799=VERTEX_POINT ( 'NONE', #15850 ) ;
#40800=DIRECTION ( 'NONE',  ( -0.7378332790417239107, 0.000000000000000000, -0.6749830015182142207 ) ) ;
#40802=LINE ( 'NONE', #47930, #26577 ) ;
#40804=FACE_OUTER_BOUND ( 'NONE', #34915, .T. ) ;
#40805=ORIENTED_EDGE ( 'NONE', *, *, #9075, .F. ) ;
#40808=DIRECTION ( 'NONE',  ( 0.000000000000000000, 0.000000000000000000, -1.000000000000000000 ) ) ;
#40811=ORIENTED_EDGE ( 'NONE', *, *, #30340, .F. ) ;
#40812=CARTESIAN_POINT ( 'NONE',  ( -48.47912675150885065, -183.6283474603465606, 6.938893903907228378E-15 ) ) ;
#40814=DIRECTION ( 'NONE',  ( -0.000000000000000000, 1.000000000000000000, -0.000000000000000000 ) ) ;
#40815=VERTEX_POINT ( 'NONE', #2967 ) ;
#40816=FACE_OUTER_BOUND ( 'NONE', #4172, .T. ) ;
#40819=FACE_OUTER_BOUND ( 'NONE', #24048, .T. ) ;
#40821=FACE_BOUND ( 'NONE', #45264, .T. ) ;
#40823=VECTOR ( 'NONE', #42306, 1000.000000000000000 ) ;
#40825=ORIENTED_EDGE ( 'NONE', *, *, #42382, .F. ) ;
#40827=AXIS2_PLACEMENT_3D ( 'NONE', #9430, #45438, #5497 ) ;
#40828=DIRECTION ( 'NONE',  ( -0.9473263538541923934, 0.000000000000000000, 0.3202698538628350744 ) ) ;
#40829=DIRECTION ( 'NONE',  ( 0.9995608365087940150, 0.000000000000000000, 0.02963332782257007206 ) ) ;
#40830=PLANE ( 'NONE',  #13144 ) ;
#40831=EDGE_CURVE ( 'NONE', #7741, #3888, #34653, .T. ) ;
#40832=ADVANCED_FACE ( 'NONE', ( #11876 ), #31863, .T. ) ;
#40833=CIRCLE ( 'NONE', #39149, 125.0000000000000000 ) ;
#40835=EDGE_LOOP ( 'NONE', ( #12088, #17187, #17574, #31342 ) ) ;
#40836=CARTESIAN_POINT ( 'NONE',  ( -112.7586829773731267, -189.7472609257535510, -107.2060569716373379 ) ) ;
#40837=VECTOR ( 'NONE', #32406, 1000.000000000000000 ) ;
#40838=ORIENTED_EDGE ( 'NONE', *, *, #30331, .T. ) ;
#40840=DIRECTION ( 'NONE',  ( -0.8757349421956310831, 0.000000000000000000, -0.4827922027307550712 ) ) ;
#40841=CARTESIAN_POINT ( 'NONE',  ( -49.25565061422688728, -175.3837268820161057, -0.6300878435817132139 ) ) ;
#40842=ORIENTED_EDGE ( 'NONE', *, *, #24348, .T. ) ;
#40850=EDGE_CURVE ( 'NONE', #9326, #21927, #6918, .T. ) ;
#40852=CARTESIAN_POINT ( 'NONE',  ( 31.28129687248616619, -183.6283474603465606, 96.24590808611479531 ) ) ;
#40854=AXIS2_PLACEMENT_3D ( 'NONE', #14303, #38965, #6163 ) ;
#40855=DIRECTION ( 'NONE',  ( -0.000000000000000000, -1.000000000000000000, 0.000000000000000000 ) ) ;
#40856=DIRECTION ( 'NONE',  ( 0.000000000000000000, 0.000000000000000000, 1.000000000000000000 ) ) ;
#40857=VERTEX_POINT ( 'NONE', #32114 ) ;
#40862=DIRECTION ( 'NONE',  ( 0.9151456172430153524, 0.000000000000000000, 0.4031234292879792847 ) ) ;
#40864=VECTOR ( 'NONE', #15877, 1000.000000000000000 ) ;
#40866=VECTOR ( 'NONE', #31565, 1000.000000000000000 ) ;
#40868=VECTOR ( 'NONE', #5047, 1000.000000000000000 ) ;
#40872=AXIS2_PLACEMENT_3D ( 'NONE', #23680, #48660, #36285 ) ;
#40873=EDGE_LOOP ( 'NONE', ( #33026, #27036, #7659, #49844 ) ) ;
#40875=ORIENTED_EDGE ( 'NONE', *, *, #36139, .T. ) ;
#40877=CARTESIAN_POINT ( 'NONE',  ( -49.44376233341720450, -177.1207230881787780, -0.2635871660690713436 ) ) ;
#40878=DIRECTION ( 'NONE',  ( 0.000000000000000000, 0.000000000000000000, 1.000000000000000000 ) ) ;
#40880=DIRECTION ( 'NONE',  ( 0.000000000000000000, 1.000000000000000000, -0.000000000000000000 ) ) ;
#40882=PLANE ( 'NONE',  #38457 ) ;
#40883=ORIENTED_EDGE ( 'NONE', *, *, #13203, .F. ) ;
#40884=ADVANCED_FACE ( 'NONE', ( #15581 ), #39479, .T. ) ;
#40886=CARTESIAN_POINT ( 'NONE',  ( 51.65665342072240662, -193.5000000000000000, 74.81861753132422166 ) ) ;
#40887=CIRCLE ( 'NONE', #38386, 125.0000000000000000 ) ;
#40888=VECTOR ( 'NONE', #2645, 1000.000000000000000 ) ;
#40889=DIRECTION ( 'NONE',  ( 0.000000000000000000, 1.000000000000000000, 0.000000000000000000 ) ) ;
#40890=DIRECTION ( 'NONE',  ( 0.000000000000000000, 0.000000000000000000, -1.000000000000000000 ) ) ;
#40891=VECTOR ( 'NONE', #35616, 1000.000000000000227 ) ;
#40892=DIRECTION ( 'NONE',  ( 0.000000000000000000, 0.000000000000000000, 1.000000000000000000 ) ) ;
#40893=CARTESIAN_POINT ( 'NONE',  ( 8.448131207122532516, -175.3837268820161057, 111.2847127925100352 ) ) ;
#40894=CARTESIAN_POINT ( 'NONE',  ( -154.0877180371535360, -189.7472609257535510, -66.87170886601934683 ) ) ;
#40896=VERTEX_POINT ( 'NONE', #11358 ) ;
#40898=DIRECTION ( 'NONE',  ( 0.000000000000000000, 0.000000000000000000, -1.000000000000000000 ) ) ;
#40899=CARTESIAN_POINT ( 'NONE',  ( -129.5578577291867646, -189.7472609257535510, 93.82025162278060293 ) ) ;
#40900=FACE_BOUND ( 'NONE', #50287, .T. ) ;
#40901=ORIENTED_EDGE ( 'NONE', *, *, #18309, .F. ) ;
#40903=EDGE_CURVE ( 'NONE', #25927, #14590, #22950, .T. ) ;
#40904=VECTOR ( 'NONE', #15283, 1000.000000000000000 ) ;
#40906=VERTEX_POINT ( 'NONE', #11632 ) ;
#40909=ORIENTED_EDGE ( 'NONE', *, *, #50630, .T. ) ;
#40910=CARTESIAN_POINT ( 'NONE',  ( -238.7407812814481076, -213.5000000000000000, 10.00000000000000178 ) ) ;
#40911=VECTOR ( 'NONE', #39142, 1000.000000000000000 ) ;
#40914=DIRECTION ( 'NONE',  ( -0.8757349421956345248, 0.000000000000000000, -0.4827922027307490205 ) ) ;
#40915=DIRECTION ( 'NONE',  ( 0.000000000000000000, 0.000000000000000000, 1.000000000000000000 ) ) ;
#40917=EDGE_LOOP ( 'NONE', ( #22556, #36694, #28435, #39745 ) ) ;
#40919=EDGE_CURVE ( 'NONE', #50197, #12264, #27909, .T. ) ;
#40920=DIRECTION ( 'NONE',  ( 0.000000000000000000, 1.000000000000000000, 0.000000000000000000 ) ) ;
#40923=ORIENTED_EDGE ( 'NONE', *, *, #11762, .F. ) ;
#40924=DIRECTION ( 'NONE',  ( -0.000000000000000000, -1.000000000000000000, 0.000000000000000000 ) ) ;
#40925=AXIS2_PLACEMENT_3D ( 'NONE', #47171, #30346, #6458 ) ;
#40926=CARTESIAN_POINT ( 'NONE',  ( -18.54723674587610560, -189.7472609257535510, 120.3332351033025702 ) ) ;
#40927=VECTOR ( 'NONE', #27570, 999.9999999999998863 ) ;
#40929=PLANE ( 'NONE',  #46926 ) ;
#40931=CARTESIAN_POINT ( 'NONE',  ( 65.79610465833508215, -177.1207230881787780, -50.65739320401928580 ) ) ;
#40932=AXIS2_PLACEMENT_3D ( 'NONE', #51345, #11376, #27411 ) ;
#40933=FACE_OUTER_BOUND ( 'NONE', #45777, .T. ) ;
#40935=ORIENTED_EDGE ( 'NONE', *, *, #51638, .F. ) ;
#40936=CARTESIAN_POINT ( 'NONE',  ( -167.6453766917639427, -183.6283474603465606, 37.74128873232411507 ) ) ;
#40937=LINE ( 'NONE', #43837, #10482 ) ;
#40938=EDGE_LOOP ( 'NONE', ( #15673, #32125, #22215, #21204 ) ) ;
#40942=EDGE_LOOP ( 'NONE', ( #26095, #16798, #47843, #4400 ) ) ;
#40943=DIRECTION ( 'NONE',  ( 1.000000000000000000, 0.000000000000000000, -6.978251959525016136E-17 ) ) ;
#40944=EDGE_CURVE ( 'NONE', #10598, #42603, #23470, .T. ) ;
#40947=CARTESIAN_POINT ( 'NONE',  ( -33.86391487983341619, -175.3837268820161057, 124.1426420773540542 ) ) ;
#40948=DIRECTION ( 'NONE',  ( 0.000000000000000000, 0.000000000000000000, -1.000000000000000000 ) ) ;
#40950=CARTESIAN_POINT ( 'NONE',  ( -48.47912675150885065, -183.6283474603465606, 6.938893903907228378E-15 ) ) ;
#40952=VECTOR ( 'NONE', #45742, 1000.000000000000000 ) ;
#40956=PLANE ( 'NONE',  #24695 ) ;
#40961=DIRECTION ( 'NONE',  ( 0.000000000000000000, 1.000000000000000000, -0.000000000000000000 ) ) ;
#40963=DIRECTION ( 'NONE',  ( 0.7765238627180437447, 0.000000000000000000, -0.6300878435817094392 ) ) ;
#40965=ADVANCED_FACE ( 'NONE', ( #39232 ), #47900, .T. ) ;
#40966=EDGE_CURVE ( 'NONE', #16634, #15304, #39699, .T. ) ;
#40968=ORIENTED_EDGE ( 'NONE', *, *, #41678, .T. ) ;
#40969=ORIENTED_EDGE ( 'NONE', *, *, #7568, .T. ) ;
#40970=CIRCLE ( 'NONE', #18328, 125.0000000000000000 ) ;
#40973=VECTOR ( 'NONE', #2926, 1000.000000000000000 ) ;
#40974=EDGE_CURVE ( 'NONE', #19921, #43567, #13194, .T. ) ;
#40975=VECTOR ( 'NONE', #10298, 1000.000000000000000 ) ;
#40978=ORIENTED_EDGE ( 'NONE', *, *, #5411, .F. ) ;
#40979=ORIENTED_EDGE ( 'NONE', *, *, #12262, .F. ) ;
#40980=ORIENTED_EDGE ( 'NONE', *, *, #2532, .T. ) ;
#40981=VECTOR ( 'NONE', #31875, 1000.000000000000114 ) ;
#40982=CARTESIAN_POINT ( 'NONE',  ( 31.28129687248616619, -183.6283474603465606, 96.24590808611479531 ) ) ;
#40983=CARTESIAN_POINT ( 'NONE',  ( 64.86941505090324256, -177.1207230881787780, -50.28156562190505241 ) ) ;
#40985=CARTESIAN_POINT ( 'NONE',  ( -146.2338470511239450, -183.6283474603465606, 76.29032973288700248 ) ) ;
#40988=CARTESIAN_POINT ( 'NONE',  ( -91.22542124915045747, -189.7472609257535510, 117.4638425504669925 ) ) ;
#40989=ORIENTED_EDGE ( 'NONE', *, *, #33557, .F. ) ;
#40990=CIRCLE ( 'NONE', #44348, 124.9999999999999858 ) ;
#40992=ORIENTED_EDGE ( 'NONE', *, *, #12038, .F. ) ;
#40993=FACE_OUTER_BOUND ( 'NONE', #34726, .T. ) ;
#40994=ORIENTED_EDGE ( 'NONE', *, *, #30757, .T. ) ;
#40995=DIRECTION ( 'NONE',  ( -0.000000000000000000, -1.000000000000000000, 0.000000000000000000 ) ) ;
#40996=DIRECTION ( 'NONE',  ( -0.000000000000000000, 1.000000000000000000, -0.000000000000000000 ) ) ;
#40997=CARTESIAN_POINT ( 'NONE',  ( -65.65563056894595206, -183.6283474603465606, 123.8142468240612857 ) ) ;
#40998=CARTESIAN_POINT ( 'NONE',  ( -80.17897391495031911, -183.6283474603465606, 120.9136869416132498 ) ) ;
#40999=CARTESIAN_POINT ( 'NONE',  ( -49.46816693883101124, -183.6283474603465606, -0.1476465640024848536 ) ) ;
#41001=VECTOR ( 'NONE', #46091, 1000.000000000000000 ) ;
#41002=LINE ( 'NONE', #4494, #6346 ) ;
#41003=ORIENTED_EDGE ( 'NONE', *, *, #19143, .F. ) ;
#41004=CARTESIAN_POINT ( 'NONE',  ( -48.47912675150885065, -175.3837268820161057, 6.938893903907228378E-15 ) ) ;
#41005=LINE ( 'NONE', #18071, #25788 ) ;
#41006=AXIS2_PLACEMENT_3D ( 'NONE', #12024, #44094, #40153 ) ;
#41007=ORIENTED_EDGE ( 'NONE', *, *, #7337, .T. ) ;
#41008=ADVANCED_FACE ( 'NONE', ( #8993 ), #20285, .F. ) ;
#41012=CARTESIAN_POINT ( 'NONE',  ( 6.443011874827243801, -183.6283474603465606, 112.2878385610370771 ) ) ;
#41013=DIRECTION ( 'NONE',  ( -0.7765238627180482966, 0.000000000000000000, 0.6300878435817038881 ) ) ;
#41015=EDGE_CURVE ( 'NONE', #46251, #48376, #9502, .T. ) ;
#41016=VECTOR ( 'NONE', #32937, 1000.000000000000000 ) ;
#41020=EDGE_LOOP ( 'NONE', ( #24022, #26990, #10212, #16362 ) ) ;
#41022=EDGE_CURVE ( 'NONE', #13401, #46759, #19580, .T. ) ;
#41023=CARTESIAN_POINT ( 'NONE',  ( -112.2501518587239104, -193.5000000000000000, -106.3450133598699665 ) ) ;
#41024=CARTESIAN_POINT ( 'NONE',  ( -33.98218805075476467, -189.7472609257535510, 123.1496609813405456 ) ) ;
#41026=ADVANCED_FACE ( 'NONE', ( #49199 ), #17140, .T. ) ;
#41028=EDGE_CURVE ( 'NONE', #39766, #44661, #27938, .T. ) ;
#41030=DIRECTION ( 'NONE',  ( -0.5586467658036594619, 0.000000000000000000, 0.8294056854501971054 ) ) ;
#41033=DIRECTION ( 'NONE',  ( -0.5586467658036415873, 0.000000000000000000, -0.8294056854502090959 ) ) ;
#41036=CARTESIAN_POINT ( 'NONE',  ( -170.2790847791494855, -193.5000000000000000, -28.10285082451569494 ) ) ;
#41038=DIRECTION ( 'NONE',  ( 0.000000000000000000, 0.000000000000000000, 1.000000000000000000 ) ) ;
#41040=CARTESIAN_POINT ( 'NONE',  ( -167.4530144994566285, -177.1207230881787780, -34.94873081740328757 ) ) ;
#41042=DIRECTION ( 'NONE',  ( -0.000000000000000000, 1.000000000000000000, -0.000000000000000000 ) ) ;
#41046=FACE_OUTER_BOUND ( 'NONE', #15416, .T. ) ;
#41047=EDGE_CURVE ( 'NONE', #35050, #45987, #9256, .T. ) ;
#41048=CARTESIAN_POINT ( 'NONE',  ( -44.48323084606168720, -183.6283474603465606, 124.9361149384469769 ) ) ;
#41052=VERTEX_POINT ( 'NONE', #20546 ) ;
#41053=CARTESIAN_POINT ( 'NONE',  ( -106.4764934152196645, -193.5000000000000000, -110.7307791902282474 ) ) ;
#41054=DIRECTION ( 'NONE',  ( 0.000000000000000000, 0.000000000000000000, 1.000000000000000000 ) ) ;
#41055=DIRECTION ( 'NONE',  ( 0.000000000000000000, -1.000000000000000000, -0.000000000000000000 ) ) ;
#41056=ORIENTED_EDGE ( 'NONE', *, *, #39538, .F. ) ;
#41058=AXIS2_PLACEMENT_3D ( 'NONE', #48205, #21589, #12903 ) ;
#41059=EDGE_CURVE ( 'NONE', #50918, #36788, #7800, .T. ) ;
#41060=DIRECTION ( 'NONE',  ( 0.000000000000000000, -0.000000000000000000, -1.000000000000000000 ) ) ;
#41061=DIRECTION ( 'NONE',  ( -0.5338233779648003940, 0.000000000000000000, 0.8455960035018199594 ) ) ;
#41063=CARTESIAN_POINT ( 'NONE',  ( 74.13662511985246795, -193.5000000000000000, 18.47640724094592457 ) ) ;
#41064=ORIENTED_EDGE ( 'NONE', *, *, #1459, .F. ) ;
#41066=ORIENTED_EDGE ( 'NONE', *, *, #49818, .F. ) ;
#41067=ADVANCED_FACE ( 'NONE', ( #12918 ), #16629, .T. ) ;
#41070=EDGE_CURVE ( 'NONE', #1407, #34403, #20820, .T. ) ;
#41071=DIRECTION ( 'NONE',  ( 0.000000000000000000, -1.000000000000000000, 0.000000000000000000 ) ) ;
#41072=CARTESIAN_POINT ( 'NONE',  ( -4.176930889631405464, -175.3837268820161057, 116.8859077982279615 ) ) ;
#41073=PLANE ( 'NONE',  #34137 ) ;
#41074=EDGE_CURVE ( 'NONE', #13416, #12178, #16882, .T. ) ;
#41075=ORIENTED_EDGE ( 'NONE', *, *, #33944, .T. ) ;
#41076=VERTEX_POINT ( 'NONE', #8209 ) ;
#41077=LINE ( 'NONE', #17955, #14730 ) ;
#41078=DIRECTION ( 'NONE',  ( -0.4031234292879792847, 0.000000000000000000, 0.9151456172430153524 ) ) ;
#41079=AXIS2_PLACEMENT_3D ( 'NONE', #35101, #50886, #38532 ) ;
#41080=VERTEX_POINT ( 'NONE', #40247 ) ;
#41083=DIRECTION ( 'NONE',  ( 0.2348860457809775482, 0.000000000000000000, 0.9720229140804121926 ) ) ;
#41086=VERTEX_POINT ( 'NONE', #42075 ) ;
#41087=CARTESIAN_POINT ( 'NONE',  ( -81.14588623932559130, -193.5000000000000000, 120.6560517527618117 ) ) ;
#41093=ORIENTED_EDGE ( 'NONE', *, *, #37827, .T. ) ;
#41094=DIRECTION ( 'NONE',  ( -0.000000000000000000, 1.000000000000000000, -0.000000000000000000 ) ) ;
#41095=EDGE_CURVE ( 'NONE', #28776, #48767, #37627, .T. ) ;
#41096=CARTESIAN_POINT ( 'NONE',  ( 75.28414827670441412, -183.6283474603465606, -7.666780576874951514 ) ) ;
#41097=ORIENTED_EDGE ( 'NONE', *, *, #36950, .F. ) ;
#41100=DIRECTION ( 'NONE',  ( 0.000000000000000000, -1.000000000000000000, 0.000000000000000000 ) ) ;
#41102=FACE_OUTER_BOUND ( 'NONE', #27004, .T. ) ;
#41103=ADVANCED_FACE ( 'NONE', ( #37877 ), #26303, .T. ) ;
#41104=VECTOR ( 'NONE', #3570, 1000.000000000000000 ) ;
#41106=DIRECTION ( 'NONE',  ( 0.000000000000000000, 0.000000000000000000, 1.000000000000000000 ) ) ;
#41109=ORIENTED_EDGE ( 'NONE', *, *, #41799, .F. ) ;
#41110=LINE ( 'NONE', #17730, #31038 ) ;
#41111=CARTESIAN_POINT ( 'NONE',  ( -38.66762320617017679, -183.6283474603465606, -124.6143426664033740 ) ) ;
#41112=ORIENTED_EDGE ( 'NONE', *, *, #15400, .T. ) ;
#41113=ORIENTED_EDGE ( 'NONE', *, *, #7628, .F. ) ;
#41114=PLANE ( 'NONE',  #6418 ) ;
#41117=FACE_OUTER_BOUND ( 'NONE', #11099, .T. ) ;
#41118=ORIENTED_EDGE ( 'NONE', *, *, #5910, .F. ) ;
#41121=ORIENTED_EDGE ( 'NONE', *, *, #39092, .F. ) ;
#41122=FACE_OUTER_BOUND ( 'NONE', #3032, .T. ) ;
#41124=DIRECTION ( 'NONE',  ( -0.5586467658036476935, 0.000000000000000000, -0.8294056854502049880 ) ) ;
#41125=CARTESIAN_POINT ( 'NONE',  ( -48.47912675150885065, -177.1207230881787780, 6.938893903907228378E-15 ) ) ;
#41127=VERTEX_POINT ( 'NONE', #29466 ) ;
#41128=VERTEX_POINT ( 'NONE', #29997 ) ;
#41130=DIRECTION ( 'NONE',  ( 0.000000000000000000, 0.000000000000000000, -1.000000000000000000 ) ) ;
#41133=CARTESIAN_POINT ( 'NONE',  ( -48.47912675150885065, -193.5000000000000000, 125.0000000000000000 ) ) ;
#41134=ORIENTED_EDGE ( 'NONE', *, *, #50822, .T. ) ;
#41136=EDGE_CURVE ( 'NONE', #17733, #15597, #22104, .T. ) ;
#41137=VECTOR ( 'NONE', #2733, 999.9999999999998863 ) ;
#41140=DIRECTION ( 'NONE',  ( -0.000000000000000000, 1.000000000000000000, -0.000000000000000000 ) ) ;
#41142=ORIENTED_EDGE ( 'NONE', *, *, #26947, .T. ) ;
#41143=DIRECTION ( 'NONE',  ( 0.000000000000000000, 0.000000000000000000, -1.000000000000000000 ) ) ;
#41144=DIRECTION ( 'NONE',  ( -0.9646355819083556327, 0.000000000000000000, -0.2635871660690782825 ) ) ;
#41148=ORIENTED_EDGE ( 'NONE', *, *, #42039, .T. ) ;
#41149=LINE ( 'NONE', #45630, #29229 ) ;
#41150=VERTEX_POINT ( 'NONE', #38394 ) ;
#41151=ORIENTED_EDGE ( 'NONE', *, *, #38966, .F. ) ;
#41152=DIRECTION ( 'NONE',  ( 0.000000000000000000, 0.000000000000000000, -1.000000000000000000 ) ) ;
#41154=ADVANCED_FACE ( 'NONE', ( #18434 ), #34450, .T. ) ;
#41156=DIRECTION ( 'NONE',  ( -0.05924062789370006937, 0.000000000000000000, -0.9982437317643222396 ) ) ;
#41157=DIRECTION ( 'NONE',  ( -0.000000000000000000, 1.000000000000000000, 0.000000000000000000 ) ) ;
#41158=CARTESIAN_POINT ( 'NONE',  ( 71.18041382641611392, -193.5000000000000000, -32.52067927015754378 ) ) ;
#41160=DIRECTION ( 'NONE',  ( 0.9929810960135178055, 0.000000000000000000, -0.1182731709213592358 ) ) ;
#41161=CARTESIAN_POINT ( 'NONE',  ( -118.1688136093591908, -193.5000000000000000, -103.7706487676296661 ) ) ;
#41162=ADVANCED_FACE ( 'NONE', ( #49476 ), #9508, .F. ) ;
#41163=LINE ( 'NONE', #5183, #24470 ) ;
#41164=FACE_BOUND ( 'NONE', #22262, .T. ) ;
#41165=VERTEX_POINT ( 'NONE', #16532 ) ;
#41166=CARTESIAN_POINT ( 'NONE',  ( 72.82672500347334221, -175.3837268820161057, 25.70779184431858866 ) ) ;
#41169=PLANE ( 'NONE',  #38858 ) ;
#41172=VECTOR ( 'NONE', #20752, 1000.000000000000000 ) ;
#41173=LINE ( 'NONE', #33559, #37743 ) ;
#41176=VERTEX_POINT ( 'NONE', #48597 ) ;
#41178=VERTEX_POINT ( 'NONE', #8628 ) ;
#41183=CIRCLE ( 'NONE', #3413, 125.0000000000000000 ) ;
#41184=VERTEX_POINT ( 'NONE', #33586 ) ;
#41185=PLANE ( 'NONE',  #47169 ) ;
#41187=EDGE_LOOP ( 'NONE', ( #9419, #37565, #34363, #8095 ) ) ;
#41189=CARTESIAN_POINT ( 'NONE',  ( -47.57632892154311577, -193.5000000000000000, 0.4300652022765314997 ) ) ;
#41191=ORIENTED_EDGE ( 'NONE', *, *, #7214, .F. ) ;
#41192=FACE_OUTER_BOUND ( 'NONE', #33797, .T. ) ;
#41193=DIRECTION ( 'NONE',  ( -0.000000000000000000, 1.000000000000000000, -0.000000000000000000 ) ) ;
#41198=CARTESIAN_POINT ( 'NONE',  ( -152.8713435144644848, -183.6283474603465606, -68.75510947788595217 ) ) ;
#41199=CIRCLE ( 'NONE', #11821, 125.0000000000000000 ) ;
#41201=DIRECTION ( 'NONE',  ( -0.8896570909947467687, 0.000000000000000000, -0.4566292373937140270 ) ) ;
#41202=DIRECTION ( 'NONE',  ( 0.5338233779647826305, 0.000000000000000000, 0.8455960035018311727 ) ) ;
#41203=ORIENTED_EDGE ( 'NONE', *, *, #49630, .T. ) ;
#41204=DIRECTION ( 'NONE',  ( 0.000000000000000000, 0.000000000000000000, 1.000000000000000000 ) ) ;
#41206=CIRCLE ( 'NONE', #28598, 125.0000000000000000 ) ;
#41208=DIRECTION ( 'NONE',  ( -0.000000000000000000, 1.000000000000000000, -0.000000000000000000 ) ) ;
#41209=CARTESIAN_POINT ( 'NONE',  ( 64.01121016852529522, -193.5000000000000000, -54.50618404930953176 ) ) ;
#41210=EDGE_CURVE ( 'NONE', #5856, #20039, #33061, .T. ) ;
#41214=DIRECTION ( 'NONE',  ( 0.000000000000000000, 0.000000000000000000, 1.000000000000000000 ) ) ;
#41216=DIRECTION ( 'NONE',  ( 0.000000000000000000, 1.000000000000000000, 0.000000000000000000 ) ) ;
#41217=CARTESIAN_POINT ( 'NONE',  ( -48.47912675150885065, -173.5000000000000284, 15.00000000000000711 ) ) ;
#41220=CARTESIAN_POINT ( 'NONE',  ( 10.73478887071926202, -177.1207230881787780, -110.0850225811106924 ) ) ;
#41221=ADVANCED_FACE ( 'NONE', ( #44389 ), #13610, .T. ) ;
#41223=CIRCLE ( 'NONE', #11841, 125.0000000000000000 ) ;
#41228=ADVANCED_FACE ( 'NONE', ( #29375 ), #36472, .T. ) ;
#41230=CARTESIAN_POINT ( 'NONE',  ( 9.336583202542586335, -175.3837268820161057, 110.8257356506556164 ) ) ;
#41231=DIRECTION ( 'NONE',  ( 0.000000000000000000, -1.000000000000000000, -0.000000000000000000 ) ) ;
#41232=DIRECTION ( 'NONE',  ( -0.000000000000000000, 1.000000000000000000, -0.000000000000000000 ) ) ;
#41233=DIRECTION ( 'NONE',  ( -0.6965510290630033685, 0.000000000000000000, 0.7175072570443249420 ) ) ;
#41234=VECTOR ( 'NONE', #51646, 999.9999999999998863 ) ;
#41235=ORIENTED_EDGE ( 'NONE', *, *, #42022, .F. ) ;
#41237=DIRECTION ( 'NONE',  ( -0.000000000000000000, 1.000000000000000000, 0.000000000000000000 ) ) ;
#41239=DIRECTION ( 'NONE',  ( -0.000000000000000000, 1.000000000000000000, -0.000000000000000000 ) ) ;
#41240=AXIS2_PLACEMENT_3D ( 'NONE', #963, #17016, #47126 ) ;
#41241=PLANE ( 'NONE',  #7193 ) ;
#41242=EDGE_CURVE ( 'NONE', #16977, #14631, #27144, .T. ) ;
#41243=ORIENTED_EDGE ( 'NONE', *, *, #6112, .F. ) ;
#41245=ORIENTED_EDGE ( 'NONE', *, *, #1352, .F. ) ;
#41246=CARTESIAN_POINT ( 'NONE',  ( -49.21696003055057389, -177.1207230881787780, -0.6749830015182127774 ) ) ;
#41247=ADVANCED_FACE ( 'NONE', ( #49624 ), #21502, .T. ) ;
#41248=VECTOR ( 'NONE', #16824, 1000.000000000000000 ) ;
#41249=EDGE_CURVE ( 'NONE', #10587, #23438, #17057, .T. ) ;
#41250=CARTESIAN_POINT ( 'NONE',  ( -48.47912675150885065, -189.7472609257535510, 6.938893903907228378E-15 ) ) ;
#41251=CARTESIAN_POINT ( 'NONE',  ( -131.8938452225253855, -183.6283474603465606, 93.09664195018557109 ) ) ;
#41253=LINE ( 'NONE', #13412, #49341 ) ;
#41254=DIRECTION ( 'NONE',  ( 0.000000000000000000, -1.000000000000000000, 0.000000000000000000 ) ) ;
#41257=AXIS2_PLACEMENT_3D ( 'NONE', #14772, #30785, #46829 ) ;
#41260=DIRECTION ( 'NONE',  ( 0.000000000000000000, 0.000000000000000000, -1.000000000000000000 ) ) ;
#41262=VERTEX_POINT ( 'NONE', #45180 ) ;
#41264=DIRECTION ( 'NONE',  ( 0.000000000000000000, 1.000000000000000000, -0.000000000000000000 ) ) ;
#41266=EDGE_LOOP ( 'NONE', ( #28706, #4184, #18345, #27362 ) ) ;
#41268=CARTESIAN_POINT ( 'NONE',  ( -162.3451783319732442, -193.5000000000000000, 51.57055649762783389 ) ) ;
#41269=CARTESIAN_POINT ( 'NONE',  ( 51.78320179844650539, -193.5000000000000000, -72.96212019587142095 ) ) ;
#41271=ORIENTED_EDGE ( 'NONE', *, *, #6510, .T. ) ;
#41272=EDGE_CURVE ( 'NONE', #10210, #15063, #40670, .T. ) ;
#41275=DIRECTION ( 'NONE',  ( -0.3482016354343928088, 0.000000000000000000, -0.9374196611341231167 ) ) ;
#41276=CIRCLE ( 'NONE', #46326, 125.0000000000000000 ) ;
#41277=LINE ( 'NONE', #1616, #45048 ) ;
#41278=ORIENTED_EDGE ( 'NONE', *, *, #26121, .F. ) ;
#41280=CARTESIAN_POINT ( 'NONE',  ( -170.8336150310144887, -175.3837268820161057, 25.58083653558494319 ) ) ;
#41283=CARTESIAN_POINT ( 'NONE',  ( -48.47912675150885065, -193.5000000000000000, 124.0000000000000142 ) ) ;
#41284=EDGE_LOOP ( 'NONE', ( #36471, #40703, #2450, #48999 ) ) ;
#41285=DIRECTION ( 'NONE',  ( -0.000000000000000000, 1.000000000000000000, -0.000000000000000000 ) ) ;
#41286=FACE_OUTER_BOUND ( 'NONE', #34597, .T. ) ;
#41287=PLANE ( 'NONE',  #5106 ) ;
#41288=CARTESIAN_POINT ( 'NONE',  ( 26.70958190211001337, -193.5000000000000000, -99.85818990449013199 ) ) ;
#41290=DIRECTION ( 'NONE',  ( 0.000000000000000000, 1.000000000000000000, -0.000000000000000000 ) ) ;
#41292=VECTOR ( 'NONE', #7719, 1000.000000000000000 ) ;
#41293=DIRECTION ( 'NONE',  ( 0.000000000000000000, 0.000000000000000000, 1.000000000000000000 ) ) ;
#41294=CYLINDRICAL_SURFACE ( 'NONE', #48039, 125.0000000000000000 ) ;
#41296=VERTEX_POINT ( 'NONE', #48853 ) ;
#41297=VERTEX_POINT ( 'NONE', #20723 ) ;
#41298=EDGE_CURVE ( 'NONE', #13171, #39625, #40571, .T. ) ;
#41300=DIRECTION ( 'NONE',  ( -0.000000000000000000, 1.000000000000000000, -0.000000000000000000 ) ) ;
#41301=CARTESIAN_POINT ( 'NONE',  ( -64.08700758308647494, -175.3837268820161057, -124.0217483183786840 ) ) ;
#41302=CARTESIAN_POINT ( 'NONE',  ( -4.525132525065792777, -175.3837268820161057, 115.9484881370938325 ) ) ;
#41303=ORIENTED_EDGE ( 'NONE', *, *, #46863, .T. ) ;
#41305=ORIENTED_EDGE ( 'NONE', *, *, #21997, .F. ) ;
#41306=DIRECTION ( 'NONE',  ( 0.000000000000000000, -0.000000000000000000, 1.000000000000000000 ) ) ;
#41307=VECTOR ( 'NONE', #42774, 1000.000000000000000 ) ;
#41309=CARTESIAN_POINT ( 'NONE',  ( -238.7407812814481076, -193.5000000000000000, -41.45482488023466061 ) ) ;
#41311=VERTEX_POINT ( 'NONE', #50404 ) ;
#41313=VECTOR ( 'NONE', #19978, 1000.000000000000000 ) ;
#41315=DIRECTION ( 'NONE',  ( 0.7175072570443348230, 0.000000000000000000, -0.6965510290629933765 ) ) ;
#41316=EDGE_LOOP ( 'NONE', ( #18578, #48507, #18140, #31233 ) ) ;
#41317=ADVANCED_FACE ( 'NONE', ( #2314 ), #25957, .T. ) ;
#41318=CARTESIAN_POINT ( 'NONE',  ( -168.8371699641976704, -189.7472609257535510, 33.74820638215506108 ) ) ;
#41320=LINE ( 'NONE', #1388, #31404 ) ;
#41323=CARTESIAN_POINT ( 'NONE',  ( -163.3872488209693756, -183.6283474603465606, -49.20491319441543254 ) ) ;
#41324=CARTESIAN_POINT ( 'NONE',  ( 68.59638248015004081, -193.5000000000000000, -43.79868877201405297 ) ) ;
#41325=CARTESIAN_POINT ( 'NONE',  ( -128.2395503755045638, -177.1207230881787780, -96.24590808611419845 ) ) ;
#41327=VECTOR ( 'NONE', #20328, 1000.000000000000000 ) ;
#41328=VERTEX_POINT ( 'NONE', #18348 ) ;
#41330=CIRCLE ( 'NONE', #32103, 125.0000000000000000 ) ;
#41332=AXIS2_PLACEMENT_3D ( 'NONE', #45823, #49772, #14025 ) ;
#41333=CARTESIAN_POINT ( 'NONE',  ( -48.53836737940255119, -177.1207230881787780, -0.9982437317643153563 ) ) ;
#41334=LINE ( 'NONE', #37918, #40101 ) ;
#41335=EDGE_LOOP ( 'NONE', ( #6580, #9463, #39161, #43233 ) ) ;
#41336=DIRECTION ( 'NONE',  ( -0.6965510290629982615, 0.000000000000000000, 0.7175072570443298270 ) ) ;
#41337=ORIENTED_EDGE ( 'NONE', *, *, #9309, .T. ) ;
#41338=DIRECTION ( 'NONE',  ( -0.000000000000000000, 1.000000000000000000, -0.000000000000000000 ) ) ;
#41342=CARTESIAN_POINT ( 'NONE',  ( -23.01747912075237679, -183.6283474603465606, -122.3793467049370776 ) ) ;
#41343=EDGE_LOOP ( 'NONE', ( #15833, #29712, #30243, #22161 ) ) ;
#41344=DIRECTION ( 'NONE',  ( 0.000000000000000000, 0.000000000000000000, 1.000000000000000000 ) ) ;
#41345=DIRECTION ( 'NONE',  ( 0.000000000000000000, 0.000000000000000000, 1.000000000000000000 ) ) ;
#41348=CARTESIAN_POINT ( 'NONE',  ( -47.60339180931321579, -193.5000000000000000, 0.4827922027307559594 ) ) ;
#41352=AXIS2_PLACEMENT_3D ( 'NONE', #12604, #8667, #24691 ) ;
#41355=EDGE_LOOP ( 'NONE', ( #152, #26191, #19835, #34837 ) ) ;
#41356=EDGE_CURVE ( 'NONE', #36397, #4130, #29667, .T. ) ;
#41359=DIRECTION ( 'NONE',  ( 0.000000000000000000, -1.000000000000000000, 0.000000000000000000 ) ) ;
#41360=ORIENTED_EDGE ( 'NONE', *, *, #7959, .F. ) ;
#41361=EDGE_CURVE ( 'NONE', #27201, #29477, #26464, .T. ) ;
#41363=ADVANCED_FACE ( 'NONE', ( #14395 ), #46714, .T. ) ;
#41367=VECTOR ( 'NONE', #22582, 1000.000000000000000 ) ;
#41368=EDGE_CURVE ( 'NONE', #34268, #3435, #33761, .T. ) ;
#41369=PLANE ( 'NONE',  #43051 ) ;
#41371=ORIENTED_EDGE ( 'NONE', *, *, #15210, .F. ) ;
#41373=EDGE_CURVE ( 'NONE', #30848, #2316, #22549, .T. ) ;
#41374=ORIENTED_EDGE ( 'NONE', *, *, #3980, .T. ) ;
#41379=DIRECTION ( 'NONE',  ( -0.000000000000000000, 1.000000000000000000, -0.000000000000000000 ) ) ;
#41384=EDGE_LOOP ( 'NONE', ( #4609, #50662, #29702, #40087 ) ) ;
#41385=DIRECTION ( 'NONE',  ( 0.3758275821142292861, 0.000000000000000000, 0.9266896074318371479 ) ) ;
#41386=DIRECTION ( 'NONE',  ( -0.1476465640024779702, 0.000000000000000000, -0.9890401873221644768 ) ) ;
#41389=CARTESIAN_POINT ( 'NONE',  ( -114.1105527140175155, -183.6283474603465606, 106.3838142112217611 ) ) ;
#41390=AXIS2_PLACEMENT_3D ( 'NONE', #16152, #40043, #39005 ) ;
#41393=ADVANCED_FACE ( 'NONE', ( #2035 ), #50922, .T. ) ;
#41394=CIRCLE ( 'NONE', #11152, 125.0000000000000000 ) ;
#41395=EDGE_CURVE ( 'NONE', #46485, #47175, #18077, .T. ) ;
#41398=ORIENTED_EDGE ( 'NONE', *, *, #51304, .F. ) ;
#41399=EDGE_LOOP ( 'NONE', ( #26948, #6842, #19262, #29961 ) ) ;
#41400=DIRECTION ( 'NONE',  ( 0.000000000000000000, -1.000000000000000000, -0.000000000000000000 ) ) ;
#41402=DIRECTION ( 'NONE',  ( 0.7765238627180393038, 0.000000000000000000, 0.6300878435817147682 ) ) ;
#41403=DIRECTION ( 'NONE',  ( 0.9027978299657446470, 0.000000000000000000, -0.4300652022765183435 ) ) ;
#41404=ORIENTED_EDGE ( 'NONE', *, *, #6704, .T. ) ;
#41405=DIRECTION ( 'NONE',  ( -0.000000000000000000, 1.000000000000000000, -0.000000000000000000 ) ) ;
#41406=AXIS2_PLACEMENT_3D ( 'NONE', #50263, #41847, #5863 ) ;
#41407=ORIENTED_EDGE ( 'NONE', *, *, #12826, .F. ) ;
#41409=EDGE_LOOP ( 'NONE', ( #6512, #38946, #22163, #8672 ) ) ;
#41410=PLANE ( 'NONE',  #10299 ) ;
#41412=DIRECTION ( 'NONE',  ( -0.000000000000000000, 1.000000000000000000, -0.000000000000000000 ) ) ;
#41413=ORIENTED_EDGE ( 'NONE', *, *, #47195, .F. ) ;
#41414=LINE ( 'NONE', #1482, #30659 ) ;
#41415=CARTESIAN_POINT ( 'NONE',  ( -28.86423599357335590, -193.5000000000000000, 122.4396006697296002 ) ) ;
#41416=DIRECTION ( 'NONE',  ( 0.000000000000000000, 0.000000000000000000, -1.000000000000000000 ) ) ;
#41419=FACE_BOUND ( 'NONE', #3591, .T. ) ;
#41420=ORIENTED_EDGE ( 'NONE', *, *, #29783, .T. ) ;
#41421=CARTESIAN_POINT ( 'NONE',  ( -48.47912675150885065, -183.6283474603465606, 6.938893903907228378E-15 ) ) ;
#41424=EDGE_CURVE ( 'NONE', #17362, #34406, #43543, .T. ) ;
#41425=ORIENTED_EDGE ( 'NONE', *, *, #47873, .F. ) ;
#41426=ADVANCED_FACE ( 'NONE', ( #43789 ), #19368, .T. ) ;
#41428=ORIENTED_EDGE ( 'NONE', *, *, #15984, .T. ) ;
#41429=VECTOR ( 'NONE', #6787, 1000.000000000000000 ) ;
#41430=ADVANCED_FACE ( 'NONE', ( #51188 ), #26983, .T. ) ;
#41432=LINE ( 'NONE', #37751, #21775 ) ;
#41433=DIRECTION ( 'NONE',  ( 0.000000000000000000, 0.000000000000000000, 1.000000000000000000 ) ) ;
#41434=DIRECTION ( 'NONE',  ( -0.6965510290629882695, 0.000000000000000000, -0.7175072570443395970 ) ) ;
#41435=ORIENTED_EDGE ( 'NONE', *, *, #45786, .F. ) ;
#41436=DIRECTION ( 'NONE',  ( 0.000000000000000000, 1.000000000000000000, -0.000000000000000000 ) ) ;
#41442=CARTESIAN_POINT ( 'NONE',  ( 74.77174840718836890, -177.1207230881787780, 20.83798868929603998 ) ) ;
#41443=EDGE_CURVE ( 'NONE', #3937, #38180, #46980, .T. ) ;
#41444=ORIENTED_EDGE ( 'NONE', *, *, #13016, .F. ) ;
#41445=LINE ( 'NONE', #5731, #10207 ) ;
#41446=DIRECTION ( 'NONE',  ( -0.000000000000000000, 1.000000000000000000, -0.000000000000000000 ) ) ;
#41447=ORIENTED_EDGE ( 'NONE', *, *, #33949, .F. ) ;
#41448=ADVANCED_FACE ( 'NONE', ( #35382 ), #35644, .F. ) ;
#41450=DIRECTION ( 'NONE',  ( 0.4031234292879600778, 0.000000000000000000, 0.9151456172430237901 ) ) ;
#41451=DIRECTION ( 'NONE',  ( -0.000000000000000000, 1.000000000000000000, -0.000000000000000000 ) ) ;
#41454=VERTEX_POINT ( 'NONE', #39064 ) ;
#41455=CARTESIAN_POINT ( 'NONE',  ( -47.48307690889363641, -175.3837268820161057, -0.08879589532292464504 ) ) ;
#41456=CARTESIAN_POINT ( 'NONE',  ( -238.7407812814481076, -193.5000000000000000, 10.00000000000000178 ) ) ;
#41457=CIRCLE ( 'NONE', #30542, 125.0000000000000000 ) ;
#41458=EDGE_LOOP ( 'NONE', ( #40825, #27521, #19877, #11889 ) ) ;
#41459=AXIS2_PLACEMENT_3D ( 'NONE', #24415, #11552, #4445 ) ;
#41460=DIRECTION ( 'NONE',  ( 0.000000000000000000, -0.000000000000000000, -1.000000000000000000 ) ) ;
#41463=DIRECTION ( 'NONE',  ( 0.000000000000000000, 0.000000000000000000, 1.000000000000000000 ) ) ;
#41464=ORIENTED_EDGE ( 'NONE', *, *, #3448, .F. ) ;
#41465=AXIS2_PLACEMENT_3D ( 'NONE', #29845, #21966, #37987 ) ;
#41466=EDGE_LOOP ( 'NONE', ( #49949, #34285, #47959, #48353 ) ) ;
#41467=DIRECTION ( 'NONE',  ( 0.000000000000000000, 0.000000000000000000, 1.000000000000000000 ) ) ;
#41471=VERTEX_POINT ( 'NONE', #48000 ) ;
#41472=CARTESIAN_POINT ( 'NONE',  ( -238.7407812814481076, -213.5000000000000000, -41.45482488023466061 ) ) ;
#41473=DIRECTION ( 'NONE',  ( 0.000000000000000000, 0.000000000000000000, -1.000000000000000000 ) ) ;
#41475=EDGE_CURVE ( 'NONE', #30907, #34863, #7542, .T. ) ;
#41476=DIRECTION ( 'NONE',  ( -0.000000000000000000, 1.000000000000000000, -0.000000000000000000 ) ) ;
#41477=FACE_OUTER_BOUND ( 'NONE', #37610, .T. ) ;
#41480=DIRECTION ( 'NONE',  ( -0.000000000000000000, 1.000000000000000000, -0.000000000000000000 ) ) ;
#41481=FACE_OUTER_BOUND ( 'NONE', #30651, .T. ) ;
#41482=ORIENTED_EDGE ( 'NONE', *, *, #48303, .T. ) ;
#41483=DIRECTION ( 'NONE',  ( -0.02963332782257007553, 0.000000000000000000, 0.9995608365087941261 ) ) ;
#41484=CARTESIAN_POINT ( 'NONE',  ( -48.30223647638628393, -183.6283474603465606, 0.9842305779476049343 ) ) ;
#41486=EDGE_CURVE ( 'NONE', #4051, #47336, #36164, .T. ) ;
#41487=EDGE_CURVE ( 'NONE', #25456, #13663, #15438, .T. ) ;
#41488=EDGE_LOOP ( 'NONE', ( #8507, #32892, #19654, #33980 ) ) ;
#41490=CARTESIAN_POINT ( 'NONE',  ( -130.0559183202350084, -175.3837268820161057, -93.38753978496592367 ) ) ;
#41491=CARTESIAN_POINT ( 'NONE',  ( 18.00181100848376303, -177.1207230881787780, -105.8550183720733742 ) ) ;
#41495=AXIS2_PLACEMENT_3D ( 'NONE', #28351, #44404, #8389 ) ;
#41496=LINE ( 'NONE', #4737, #29992 ) ;
#41498=VERTEX_POINT ( 'NONE', #11470 ) ;
#41499=VECTOR ( 'NONE', #50809, 1000.000000000000227 ) ;
#41500=LINE ( 'NONE', #40719, #48307 ) ;
#41501=ORIENTED_EDGE ( 'NONE', *, *, #39701, .T. ) ;
#41502=DIRECTION ( 'NONE',  ( 0.000000000000000000, 0.000000000000000000, -1.000000000000000000 ) ) ;
#41503=VERTEX_POINT ( 'NONE', #43016 ) ;
#41507=AXIS2_PLACEMENT_3D ( 'NONE', #12680, #12938, #28966 ) ;
#41508=EDGE_CURVE ( 'NONE', #51805, #15063, #6203, .T. ) ;
#41514=VERTEX_POINT ( 'NONE', #39832 ) ;
#41516=ORIENTED_EDGE ( 'NONE', *, *, #33675, .T. ) ;
#41517=DIRECTION ( 'NONE',  ( 0.5586467658036476935, 0.000000000000000000, 0.8294056854502049880 ) ) ;
#41518=ORIENTED_EDGE ( 'NONE', *, *, #40768, .F. ) ;
#41519=EDGE_CURVE ( 'NONE', #51413, #46129, #25474, .T. ) ;
#41520=DIRECTION ( 'NONE',  ( 0.000000000000000000, 1.000000000000000000, 0.000000000000000000 ) ) ;
#41521=CARTESIAN_POINT ( 'NONE',  ( 71.73509643893275722, -177.1207230881787780, -30.40954281680804172 ) ) ;
#41522=CARTESIAN_POINT ( 'NONE',  ( 4.109287492203100634, -183.6283474603465606, -113.3995532942336979 ) ) ;
#41523=VERTEX_POINT ( 'NONE', #11981 ) ;
#41524=ORIENTED_EDGE ( 'NONE', *, *, #33684, .T. ) ;
#41527=AXIS2_PLACEMENT_3D ( 'NONE', #41209, #20995, #37016 ) ;
#41528=CARTESIAN_POINT ( 'NONE',  ( -58.29063029684667185, -183.6283474603465606, 124.6143426664034877 ) ) ;
#41529=VERTEX_POINT ( 'NONE', #28012 ) ;
#41531=PLANE ( 'NONE',  #25138 ) ;
#41532=AXIS2_PLACEMENT_3D ( 'NONE', #41198, #49372, #1529 ) ;
#41533=CARTESIAN_POINT ( 'NONE',  ( 21.49274850782853363, -189.7472609257535510, -103.5805805771126415 ) ) ;
#41534=AXIS2_PLACEMENT_3D ( 'NONE', #13893, #14940, #30947 ) ;
#41535=VERTEX_POINT ( 'NONE', #15175 ) ;
#41536=CARTESIAN_POINT ( 'NONE',  ( -41.24387117724851493, -193.5000000000000000, 124.7904286264581231 ) ) ;
#41538=CIRCLE ( 'NONE', #42365, 125.0000000000000000 ) ;
#41541=ORIENTED_EDGE ( 'NONE', *, *, #11888, .F. ) ;
#41544=AXIS2_PLACEMENT_3D ( 'NONE', #38086, #50460, #34156 ) ;
#41546=DIRECTION ( 'NONE',  ( -0.000000000000000000, 1.000000000000000000, -0.000000000000000000 ) ) ;
#41547=DIRECTION ( 'NONE',  ( -0.5338233779647887367, 0.000000000000000000, -0.8455960035018273979 ) ) ;
#41548=EDGE_CURVE ( 'NONE', #40230, #45352, #31187, .T. ) ;
#41549=CIRCLE ( 'NONE', #49974, 125.0000000000000000 ) ;
#41551=AXIS2_PLACEMENT_3D ( 'NONE', #42283, #17629, #45477 ) ;
#41554=CARTESIAN_POINT ( 'NONE',  ( -47.82630463331833681, -189.7472609257535510, 0.7575112421616305713 ) ) ;
#41555=CARTESIAN_POINT ( 'NONE',  ( 2.669657140899374337, -189.7472609257535510, 114.0561348912355868 ) ) ;
#41557=VERTEX_POINT ( 'NONE', #1189 ) ;
#41559=CARTESIAN_POINT ( 'NONE',  ( -166.9790462269951945, -177.1207230881787780, 36.52255268223134266 ) ) ;
#41560=CARTESIAN_POINT ( 'NONE',  ( -49.32472275501068282, -183.6283474603465606, 0.5338233779647895139 ) ) ;
#41562=EDGE_LOOP ( 'NONE', ( #35515, #40123, #15625, #22232 ) ) ;
#41563=AXIS2_PLACEMENT_3D ( 'NONE', #18929, #46800, #3158 ) ;
#41566=CARTESIAN_POINT ( 'NONE',  ( -123.4791267515088435, -173.5000000000000284, 70.00000000000000000 ) ) ;
#41567=AXIS2_PLACEMENT_3D ( 'NONE', #42112, #2172, #25834 ) ;
#41568=VECTOR ( 'NONE', #14231, 1000.000000000000000 ) ;
#41570=DIRECTION ( 'NONE',  ( 0.000000000000000000, 0.000000000000000000, -1.000000000000000000 ) ) ;
#41571=ORIENTED_EDGE ( 'NONE', *, *, #43586, .T. ) ;
#41574=CARTESIAN_POINT ( 'NONE',  ( -47.82630463331832971, -177.1207230881787780, -0.7575112421616121416 ) ) ;
#41575=ORIENTED_EDGE ( 'NONE', *, *, #21450, .T. ) ;
#41576=AXIS2_PLACEMENT_3D ( 'NONE', #31435, #22787, #34598 ) ;
#41577=AXIS2_PLACEMENT_3D ( 'NONE', #5008, #29163, #17618 ) ;
#41578=DIRECTION ( 'NONE',  ( -0.000000000000000000, 1.000000000000000000, -0.000000000000000000 ) ) ;
#41579=VERTEX_POINT ( 'NONE', #28279 ) ;
#41580=DIRECTION ( 'NONE',  ( 0.000000000000000000, 1.000000000000000000, 0.000000000000000000 ) ) ;
#41581=VERTEX_POINT ( 'NONE', #49309 ) ;
#41582=LINE ( 'NONE', #41323, #3966 ) ;
#41585=CARTESIAN_POINT ( 'NONE',  ( 37.99238433767461487, -189.7472609257535510, -90.26448786734026442 ) ) ;
#41586=AXIS2_PLACEMENT_3D ( 'NONE', #51125, #14855, #43200 ) ;
#41589=DIRECTION ( 'NONE',  ( 0.5338233779647826305, 0.000000000000000000, 0.8455960035018311727 ) ) ;
#41591=VERTEX_POINT ( 'NONE', #33266 ) ;
#41593=EDGE_CURVE ( 'NONE', #44250, #25303, #32745, .T. ) ;
#41594=ADVANCED_FACE ( 'NONE', ( #4905 ), #20931, .F. ) ;
#41595=ORIENTED_EDGE ( 'NONE', *, *, #1585, .F. ) ;
#41596=LINE ( 'NONE', #45566, #35948 ) ;
#41598=ORIENTED_EDGE ( 'NONE', *, *, #46138, .T. ) ;
#41601=CIRCLE ( 'NONE', #1319, 125.0000000000000000 ) ;
#41602=FACE_OUTER_BOUND ( 'NONE', #44444, .T. ) ;
#41604=DIRECTION ( 'NONE',  ( 0.000000000000000000, 0.000000000000000000, 1.000000000000000000 ) ) ;
#41605=VERTEX_POINT ( 'NONE', #36414 ) ;
#41606=VECTOR ( 'NONE', #47306, 1000.000000000000000 ) ;
#41609=LINE ( 'NONE', #10596, #7923 ) ;
#41612=CARTESIAN_POINT ( 'NONE',  ( -117.8923552450418981, -175.3837268820161057, 102.7511748916629415 ) ) ;
#41615=CARTESIAN_POINT ( 'NONE',  ( 61.38599058177057799, -193.5000000000000000, 59.62093586438192006 ) ) ;
#41618=AXIS2_PLACEMENT_3D ( 'NONE', #45620, #29040, #25621 ) ;
#41621=ORIENTED_EDGE ( 'NONE', *, *, #46537, .T. ) ;
#41622=VECTOR ( 'NONE', #22167, 1000.000000000000000 ) ;
#41623=ORIENTED_EDGE ( 'NONE', *, *, #14060, .F. ) ;
#41624=CARTESIAN_POINT ( 'NONE',  ( -48.47912675150885065, -177.1207230881787780, 6.938893903907228378E-15 ) ) ;
#41625=VECTOR ( 'NONE', #27044, 1000.000000000000000 ) ;
#41626=CIRCLE ( 'NONE', #16473, 15.00000000000000000 ) ;
#41628=ORIENTED_EDGE ( 'NONE', *, *, #49954, .F. ) ;
#41629=CARTESIAN_POINT ( 'NONE',  ( -1.230335819511603423, -193.5000000000000000, 115.7261930397108216 ) ) ;
#41630=ORIENTED_EDGE ( 'NONE', *, *, #14374, .F. ) ;
#41631=DIRECTION ( 'NONE',  ( -0.6528221181905119463, 0.000000000000000000, -0.7575112421616284619 ) ) ;
#41632=CARTESIAN_POINT ( 'NONE',  ( -16.77927958806651887, -193.5000000000000000, -120.9136869416130082 ) ) ;
#41633=CARTESIAN_POINT ( 'NONE',  ( -48.98765787015808115, -183.6283474603465606, 0.8610436117673582190 ) ) ;
#41634=ORIENTED_EDGE ( 'NONE', *, *, #41487, .T. ) ;
#41638=PLANE ( 'NONE',  #44517 ) ;
#41639=CIRCLE ( 'NONE', #43334, 125.0000000000000000 ) ;
#41641=VECTOR ( 'NONE', #21904, 1000.000000000000341 ) ;
#41643=LINE ( 'NONE', #25122, #47379 ) ;
#41644=ORIENTED_EDGE ( 'NONE', *, *, #23748, .T. ) ;
#41646=ORIENTED_EDGE ( 'NONE', *, *, #27334, .T. ) ;
#41648=ORIENTED_EDGE ( 'NONE', *, *, #24628, .F. ) ;
#41649=PLANE ( 'NONE',  #35539 ) ;
#41651=CIRCLE ( 'NONE', #27392, 125.0000000000000000 ) ;
#41652=DIRECTION ( 'NONE',  ( 0.000000000000000000, -0.000000000000000000, -1.000000000000000000 ) ) ;
#41653=AXIS2_PLACEMENT_3D ( 'NONE', #32869, #39967, #32093 ) ;
#41655=CIRCLE ( 'NONE', #1375, 125.0000000000000000 ) ;
#41657=EDGE_CURVE ( 'NONE', #22956, #3706, #36691, .T. ) ;
#41658=CARTESIAN_POINT ( 'NONE',  ( -48.47912675150885065, -189.7472609257535510, 6.938893903907228378E-15 ) ) ;
#41659=EDGE_CURVE ( 'NONE', #51892, #26963, #44571, .T. ) ;
#41661=DIRECTION ( 'NONE',  ( 0.000000000000000000, -0.000000000000000000, 1.000000000000000000 ) ) ;
#41664=AXIS2_PLACEMENT_3D ( 'NONE', #6176, #26386, #10361 ) ;
#41665=ORIENTED_EDGE ( 'NONE', *, *, #13677, .T. ) ;
#41667=AXIS2_PLACEMENT_3D ( 'NONE', #50785, #22407, #35252 ) ;
#41668=ORIENTED_EDGE ( 'NONE', *, *, #27435, .T. ) ;
#41669=CARTESIAN_POINT ( 'NONE',  ( -48.82732838694325750, -193.5000000000000000, 0.9374196611341252261 ) ) ;
#41670=EDGE_CURVE ( 'NONE', #50927, #38934, #29049, .T. ) ;
#41672=DIRECTION ( 'NONE',  ( -0.000000000000000000, -1.000000000000000000, 0.000000000000000000 ) ) ;
#41673=ORIENTED_EDGE ( 'NONE', *, *, #27600, .F. ) ;
#41674=EDGE_CURVE ( 'NONE', #19289, #28248, #32919, .T. ) ;
#41675=LINE ( 'NONE', #29060, #43273 ) ;
#41676=DIRECTION ( 'NONE',  ( 0.6528221181905227155, 0.000000000000000000, -0.7575112421616191360 ) ) ;
#41677=CARTESIAN_POINT ( 'NONE',  ( 76.09804998693969935, -175.3837268820161057, 10.27263529369908035 ) ) ;
#41678=EDGE_CURVE ( 'NONE', #41503, #29039, #9456, .T. ) ;
#41680=EDGE_CURVE ( 'NONE', #10587, #19788, #36951, .T. ) ;
#41681=CARTESIAN_POINT ( 'NONE',  ( -94.25732089370191602, -183.6283474603465606, 116.3157639405754935 ) ) ;
#41682=FACE_BOUND ( 'NONE', #39868, .T. ) ;
#41686=AXIS2_PLACEMENT_3D ( 'NONE', #26363, #17196, #5372 ) ;
#41688=LINE ( 'NONE', #45389, #3682 ) ;
#41690=AXIS2_PLACEMENT_3D ( 'NONE', #49725, #37100, #17423 ) ;
#41691=EDGE_CURVE ( 'NONE', #25127, #50038, #5686, .T. ) ;
#41692=ORIENTED_EDGE ( 'NONE', *, *, #16841, .F. ) ;
#41693=CARTESIAN_POINT ( 'NONE',  ( 74.00867759460086859, -175.3837268820161057, 24.93467037017223120 ) ) ;
#41694=ORIENTED_EDGE ( 'NONE', *, *, #10965, .F. ) ;
#41695=DIRECTION ( 'NONE',  ( -0.000000000000000000, 1.000000000000000000, -0.000000000000000000 ) ) ;
#41697=CARTESIAN_POINT ( 'NONE',  ( -47.55243714407702527, -177.1207230881787780, 0.3758275821142491591 ) ) ;
#41698=AXIS2_PLACEMENT_3D ( 'NONE', #15353, #3269, #7718 ) ;
#41699=CARTESIAN_POINT ( 'NONE',  ( 39.18328161278951427, -189.7472609257535510, 89.10837311819236106 ) ) ;
#41700=VERTEX_POINT ( 'NONE', #21708 ) ;
#41702=CIRCLE ( 'NONE', #16550, 125.0000000000000000 ) ;
#41704=CARTESIAN_POINT ( 'NONE',  ( 33.75048693540708911, -189.7472609257535510, 94.14505102712816154 ) ) ;
#41710=DIRECTION ( 'NONE',  ( 0.000000000000000000, 0.000000000000000000, 1.000000000000000000 ) ) ;
#41711=PLANE ( 'NONE',  #11723 ) ;
#41712=VERTEX_POINT ( 'NONE', #1723 ) ;
#41713=DIRECTION ( 'NONE',  ( 0.000000000000000000, 0.000000000000000000, 1.000000000000000000 ) ) ;
#41714=FACE_OUTER_BOUND ( 'NONE', #22366, .T. ) ;
#41715=ORIENTED_EDGE ( 'NONE', *, *, #48800, .F. ) ;
#41716=CARTESIAN_POINT ( 'NONE',  ( 36.19006208304271155, -177.1207230881787780, 90.59430563621340582 ) ) ;
#41720=CARTESIAN_POINT ( 'NONE',  ( -172.0839188101925004, -175.3837268820161057, -18.62405380494756812 ) ) ;
#41721=ORIENTED_EDGE ( 'NONE', *, *, #3112, .F. ) ;
#41722=VECTOR ( 'NONE', #24338, 1000.000000000000114 ) ;
#41724=AXIS2_PLACEMENT_3D ( 'NONE', #41288, #37353, #33151 ) ;
#41725=ORIENTED_EDGE ( 'NONE', *, *, #26229, .F. ) ;
#41727=DIRECTION ( 'NONE',  ( -0.9929810960135169173, 0.000000000000000000, -0.1182731709213660498 ) ) ;
#41728=ORIENTED_EDGE ( 'NONE', *, *, #6961, .F. ) ;
#41730=EDGE_CURVE ( 'NONE', #29042, #30411, #44683, .T. ) ;
#41733=EDGE_CURVE ( 'NONE', #13063, #7058, #29832, .T. ) ;
#41734=DIRECTION ( 'NONE',  ( 0.000000000000000000, 0.000000000000000000, -1.000000000000000000 ) ) ;
#41735=ORIENTED_EDGE ( 'NONE', *, *, #1569, .T. ) ;
#41740=FACE_OUTER_BOUND ( 'NONE', #20173, .T. ) ;
#41741=CIRCLE ( 'NONE', #35838, 125.0000000000000000 ) ;
#41742=CARTESIAN_POINT ( 'NONE',  ( -121.5885020763900712, -183.6283474603465606, -101.3904297239421197 ) ) ;
#41743=AXIS2_PLACEMENT_3D ( 'NONE', #30793, #46837, #26842 ) ;
#41750=CARTESIAN_POINT ( 'NONE',  ( -165.1736796818183564, -193.5000000000000000, -41.93543928473608418 ) ) ;
#41751=CARTESIAN_POINT ( 'NONE',  ( 72.71365293123227502, -183.6283474603465606, -30.61552143554913030 ) ) ;
#41753=CIRCLE ( 'NONE', #9830, 125.0000000000000000 ) ;
#41754=EDGE_CURVE ( 'NONE', #24430, #20725, #26208, .T. ) ;
#41755=ORIENTED_EDGE ( 'NONE', *, *, #14115, .T. ) ;
#41757=CARTESIAN_POINT ( 'NONE',  ( 74.18685885783125400, -193.5000000000000000, -18.13990644964002996 ) ) ;
#41759=LINE ( 'NONE', #1551, #39949 ) ;
#41760=ORIENTED_EDGE ( 'NONE', *, *, #36138, .F. ) ;
#41761=EDGE_CURVE ( 'NONE', #33090, #45648, #34042, .T. ) ;
#41762=CARTESIAN_POINT ( 'NONE',  ( -48.53836737940255119, -193.5000000000000000, -0.9982437317643153563 ) ) ;
#41764=EDGE_CURVE ( 'NONE', #19780, #9360, #10379, .T. ) ;
#41765=CARTESIAN_POINT ( 'NONE',  ( 76.09804998693969935, -175.3837268820161057, 10.27263529369908746 ) ) ;
#41766=ORIENTED_EDGE ( 'NONE', *, *, #24643, .F. ) ;
#41767=DIRECTION ( 'NONE',  ( -0.000000000000000000, 1.000000000000000000, -0.000000000000000000 ) ) ;
#41769=EDGE_CURVE ( 'NONE', #46929, #33918, #37462, .T. ) ;
#41771=DIRECTION ( 'NONE',  ( -0.000000000000000000, 1.000000000000000000, -0.000000000000000000 ) ) ;
#41777=LINE ( 'NONE', #45721, #21856 ) ;
#41778=ORIENTED_EDGE ( 'NONE', *, *, #1326, .T. ) ;
#41781=ORIENTED_EDGE ( 'NONE', *, *, #40626, .T. ) ;
#41782=FACE_OUTER_BOUND ( 'NONE', #29026, .T. ) ;
#41783=AXIS2_PLACEMENT_3D ( 'NONE', #7768, #51414, #19346 ) ;
#41784=ORIENTED_EDGE ( 'NONE', *, *, #24380, .F. ) ;
#41785=DIRECTION ( 'NONE',  ( -0.9842305779475967187, 0.000000000000000000, -0.1768902751225733538 ) ) ;
#41786=CIRCLE ( 'NONE', #11447, 125.0000000000000000 ) ;
#41787=ORIENTED_EDGE ( 'NONE', *, *, #31778, .T. ) ;
#41788=CIRCLE ( 'NONE', #38443, 125.0000000000000000 ) ;
#41793=DIRECTION ( 'NONE',  ( 0.000000000000000000, 0.000000000000000000, 1.000000000000000000 ) ) ;
#41794=EDGE_LOOP ( 'NONE', ( #32457, #20177, #4959, #18852 ) ) ;
#41795=DIRECTION ( 'NONE',  ( -0.8455960035018234011, 0.000000000000000000, -0.5338233779647948429 ) ) ;
#41796=VERTEX_POINT ( 'NONE', #42436 ) ;
#41797=DIRECTION ( 'NONE',  ( 0.000000000000000000, 1.000000000000000000, 0.000000000000000000 ) ) ;
#41798=VERTEX_POINT ( 'NONE', #18020 ) ;
#41799=EDGE_CURVE ( 'NONE', #41579, #16540, #34301, .T. ) ;
#41801=CARTESIAN_POINT ( 'NONE',  ( -77.43961373357963396, -175.3837268820161057, -120.5706864261535145 ) ) ;
#41803=ORIENTED_EDGE ( 'NONE', *, *, #4725, .F. ) ;
#41804=ORIENTED_EDGE ( 'NONE', *, *, #38929, .F. ) ;
#41805=CARTESIAN_POINT ( 'NONE',  ( -160.7804753152582293, -175.3837268820161057, -52.57768177182448710 ) ) ;
#41807=CARTESIAN_POINT ( 'NONE',  ( -151.1459075827612537, -193.5000000000000000, 69.53890913632950799 ) ) ;
#41809=CARTESIAN_POINT ( 'NONE',  ( 76.43863189440992301, -189.7472609257535510, -4.533605064403317009 ) ) ;
#41811=CARTESIAN_POINT ( 'NONE',  ( -171.7300019102062549, -193.5000000000000000, -20.83798868929510562 ) ) ;
#41812=FACE_OUTER_BOUND ( 'NONE', #45286, .T. ) ;
#41814=VECTOR ( 'NONE', #6435, 1000.000000000000000 ) ;
#41815=DIRECTION ( 'NONE',  ( -0.9982437317643222396, 0.000000000000000000, 0.05924062789370006937 ) ) ;
#41817=DIRECTION ( 'NONE',  ( -0.000000000000000000, 1.000000000000000000, -0.000000000000000000 ) ) ;
#41818=LINE ( 'NONE', #17656, #42395 ) ;
#41819=PLANE ( 'NONE',  #19573 ) ;
#41822=LINE ( 'NONE', #44996, #50820 ) ;
#41823=CARTESIAN_POINT ( 'NONE',  ( -144.8751831225492026, -193.5000000000000000, 77.99872144864772849 ) ) ;
#41824=EDGE_CURVE ( 'NONE', #32234, #2175, #6463, .T. ) ;
#41825=DIRECTION ( 'NONE',  ( -0.000000000000000000, 1.000000000000000000, -0.000000000000000000 ) ) ;
#41829=CIRCLE ( 'NONE', #28378, 125.0000000000000000 ) ;
#41830=DIRECTION ( 'NONE',  ( 0.000000000000000000, -1.000000000000000000, 0.000000000000000000 ) ) ;
#41832=DIRECTION ( 'NONE',  ( 0.6965510290630033685, 0.000000000000000000, -0.7175072570443249420 ) ) ;
#41833=VERTEX_POINT ( 'NONE', #13549 ) ;
#41836=CARTESIAN_POINT ( 'NONE',  ( -47.49008656418669005, -189.7472609257535510, 0.1476465640024920423 ) ) ;
#41840=VECTOR ( 'NONE', #20330, 1000.000000000000000 ) ;
#41841=ORIENTED_EDGE ( 'NONE', *, *, #33724, .T. ) ;
#41842=VECTOR ( 'NONE', #14703, 1000.000000000000114 ) ;
#41844=DIRECTION ( 'NONE',  ( 0.000000000000000000, 0.000000000000000000, -1.000000000000000000 ) ) ;
#41846=DIRECTION ( 'NONE',  ( -0.000000000000000000, 1.000000000000000000, -0.000000000000000000 ) ) ;
#41847=DIRECTION ( 'NONE',  ( 0.000000000000000000, -1.000000000000000000, 0.000000000000000000 ) ) ;
#41848=VERTEX_POINT ( 'NONE', #51380 ) ;
#41850=AXIS2_PLACEMENT_3D ( 'NONE', #13589, #30141, #49604 ) ;
#41852=ORIENTED_EDGE ( 'NONE', *, *, #7959, .T. ) ;
#41853=CARTESIAN_POINT ( 'NONE',  ( -114.4014177456970600, -177.1207230881787780, 105.0256126866236315 ) ) ;
#41855=LINE ( 'NONE', #32913, #25523 ) ;
#41856=ORIENTED_EDGE ( 'NONE', *, *, #2309, .F. ) ;
#41857=EDGE_CURVE ( 'NONE', #9868, #27228, #30877, .T. ) ;
#41858=LINE ( 'NONE', #17168, #19907 ) ;
#41859=DIRECTION ( 'NONE',  ( 0.000000000000000000, 1.000000000000000000, 0.000000000000000000 ) ) ;
#41862=ORIENTED_EDGE ( 'NONE', *, *, #26227, .T. ) ;
#41863=EDGE_LOOP ( 'NONE', ( #47804, #15808, #35371, #17641 ) ) ;
#41864=CARTESIAN_POINT ( 'NONE',  ( 70.98542830588607444, -177.1207230881787780, -36.78613984829961936 ) ) ;
#41865=DIRECTION ( 'NONE',  ( 0.000000000000000000, -0.000000000000000000, -1.000000000000000000 ) ) ;
#41866=ORIENTED_EDGE ( 'NONE', *, *, #22474, .F. ) ;
#41867=DIRECTION ( 'NONE',  ( -0.000000000000000000, 1.000000000000000000, -0.000000000000000000 ) ) ;
#41870=LINE ( 'NONE', #33199, #9968 ) ;
#41874=ORIENTED_EDGE ( 'NONE', *, *, #21838, .F. ) ;
#41876=AXIS2_PLACEMENT_3D ( 'NONE', #13910, #29406, #2065 ) ;
#41882=CARTESIAN_POINT ( 'NONE',  ( -169.0136227435421006, -175.3837268820161057, -33.11246405730811659 ) ) ;
#41886=ORIENTED_EDGE ( 'NONE', *, *, #30437, .T. ) ;
#41888=EDGE_LOOP ( 'NONE', ( #30941, #50040, #48299, #42977 ) ) ;
#41890=CARTESIAN_POINT ( 'NONE',  ( 64.72501964220592185, -193.5000000000000000, 53.00774697410174952 ) ) ;
#41891=CYLINDRICAL_SURFACE ( 'NONE', #14449, 125.0000000000000000 ) ;
#41892=ORIENTED_EDGE ( 'NONE', *, *, #15954, .T. ) ;
#41897=CARTESIAN_POINT ( 'NONE',  ( -48.47912675150885065, -189.7472609257535510, 6.938893903907228378E-15 ) ) ;
#41898=ORIENTED_EDGE ( 'NONE', *, *, #49004, .T. ) ;
#41899=CARTESIAN_POINT ( 'NONE',  ( -48.47912675150885065, -177.1207230881787780, 6.938893903907228378E-15 ) ) ;
#41902=LINE ( 'NONE', #9589, #36990 ) ;
#41905=ORIENTED_EDGE ( 'NONE', *, *, #14612, .F. ) ;
#41906=VERTEX_POINT ( 'NONE', #39769 ) ;
#41907=EDGE_CURVE ( 'NONE', #9601, #21200, #35076, .T. ) ;
#41908=LINE ( 'NONE', #49290, #1410 ) ;
#41909=CARTESIAN_POINT ( 'NONE',  ( 15.80042947435468470, -193.5000000000000000, 107.2060569716377927 ) ) ;
#41910=CIRCLE ( 'NONE', #52020, 125.0000000000000000 ) ;
#41911=CARTESIAN_POINT ( 'NONE',  ( -152.8713435144644848, -183.6283474603465606, -68.75510947788595217 ) ) ;
#41914=CIRCLE ( 'NONE', #16730, 125.0000000000000000 ) ;
#41916=EDGE_CURVE ( 'NONE', #20898, #38913, #11921, .T. ) ;
#41918=DIRECTION ( 'NONE',  ( 0.000000000000000000, -1.000000000000000000, -0.000000000000000000 ) ) ;
#41920=ORIENTED_EDGE ( 'NONE', *, *, #29877, .F. ) ;
#41921=ADVANCED_FACE ( 'NONE', ( #27955 ), #7221, .F. ) ;
#41922=PLANE ( 'NONE',  #49353 ) ;
#41926=VERTEX_POINT ( 'NONE', #22732 ) ;
#41928=VERTEX_POINT ( 'NONE', #3528 ) ;
#41929=VECTOR ( 'NONE', #24911, 1000.000000000000000 ) ;
#41930=ORIENTED_EDGE ( 'NONE', *, *, #10895, .T. ) ;
#41931=DIRECTION ( 'NONE',  ( 0.000000000000000000, 1.000000000000000000, 0.000000000000000000 ) ) ;
#41933=EDGE_CURVE ( 'NONE', #47240, #48128, #38742, .T. ) ;
#41935=LINE ( 'NONE', #21452, #50005 ) ;
#41936=PLANE ( 'NONE',  #10405 ) ;
#41937=PLANE ( 'NONE',  #29594 ) ;
#41938=DIRECTION ( 'NONE',  ( -0.000000000000000000, 1.000000000000000000, -0.000000000000000000 ) ) ;
#41939=LINE ( 'NONE', #50361, #122 ) ;
#41941=ORIENTED_EDGE ( 'NONE', *, *, #10714, .T. ) ;
#41942=AXIS2_PLACEMENT_3D ( 'NONE', #48362, #40205, #13138 ) ;
#41943=CYLINDRICAL_SURFACE ( 'NONE', #27278, 125.0000000000000000 ) ;
#41944=EDGE_LOOP ( 'NONE', ( #12052, #35488, #41760, #43038 ) ) ;
#41946=LINE ( 'NONE', #49849, #16219 ) ;
#41947=ORIENTED_EDGE ( 'NONE', *, *, #40559, .F. ) ;
#41950=DIRECTION ( 'NONE',  ( -0.9473263538541923934, 0.000000000000000000, 0.3202698538628350744 ) ) ;
#41951=LINE ( 'NONE', #41699, #36335 ) ;
#41953=ADVANCED_FACE ( 'NONE', ( #39000 ), #42952, .T. ) ;
#41955=DIRECTION ( 'NONE',  ( -0.000000000000000000, 1.000000000000000000, -0.000000000000000000 ) ) ;
#41956=CARTESIAN_POINT ( 'NONE',  ( 57.31108707223382481, -175.3837268820161057, -66.58401203837755133 ) ) ;
#41957=EDGE_LOOP ( 'NONE', ( #16721, #38543, #11896, #47769 ) ) ;
#41958=ORIENTED_EDGE ( 'NONE', *, *, #15998, .F. ) ;
#41959=AXIS2_PLACEMENT_3D ( 'NONE', #29816, #19034, #42691 ) ;
#41961=FACE_OUTER_BOUND ( 'NONE', #10685, .T. ) ;
#41962=CARTESIAN_POINT ( 'NONE',  ( -96.65280530915693191, -193.5000000000000000, -115.3442529744087466 ) ) ;
#41966=VERTEX_POINT ( 'NONE', #27443 ) ;
#41967=EDGE_CURVE ( 'NONE', #17878, #12249, #27699, .T. ) ;
#41969=LINE ( 'NONE', #2024, #39979 ) ;
#41970=ORIENTED_EDGE ( 'NONE', *, *, #26559, .T. ) ;
#41971=DIRECTION ( 'NONE',  ( 0.000000000000000000, 0.000000000000000000, 1.000000000000000000 ) ) ;
#41975=CIRCLE ( 'NONE', #23526, 125.0000000000000000 ) ;
#41977=CARTESIAN_POINT ( 'NONE',  ( -173.2419626162308646, -193.5000000000000000, 7.696413904698416353 ) ) ;
#41978=CARTESIAN_POINT ( 'NONE',  ( 74.80070215680143519, -193.5000000000000000, 13.35228579481200306 ) ) ;
#41982=DIRECTION ( 'NONE',  ( 0.000000000000000000, 0.000000000000000000, -1.000000000000000000 ) ) ;
#41983=ORIENTED_EDGE ( 'NONE', *, *, #41368, .F. ) ;
#41984=PLANE ( 'NONE',  #12411 ) ;
#41985=EDGE_LOOP ( 'NONE', ( #22645, #25802, #45859, #29429 ) ) ;
#41986=ORIENTED_EDGE ( 'NONE', *, *, #38466, .T. ) ;
#41987=CARTESIAN_POINT ( 'NONE',  ( 68.24201764719070695, -177.1207230881787780, -44.73448837594909833 ) ) ;
#41988=CARTESIAN_POINT ( 'NONE',  ( 67.04262753014327814, -193.5000000000000000, -47.74645837849745078 ) ) ;
#41990=DIRECTION ( 'NONE',  ( -0.9929810960135169173, 0.000000000000000000, -0.1182731709213660498 ) ) ;
#41991=VERTEX_POINT ( 'NONE', #24799 ) ;
#41992=CARTESIAN_POINT ( 'NONE',  ( 22.73247662810270597, -193.5000000000000000, -101.5140743725395254 ) ) ;
#41993=DIRECTION ( 'NONE',  ( 0.9027978299657416494, 0.000000000000000000, 0.4300652022765245608 ) ) ;
#41997=DIRECTION ( 'NONE',  ( -0.000000000000000000, 1.000000000000000000, 0.000000000000000000 ) ) ;
#41999=AXIS2_PLACEMENT_3D ( 'NONE', #3971, #19992, #15812 ) ;
#42000=AXIS2_PLACEMENT_3D ( 'NONE', #19271, #27904, #47375 ) ;
#42002=EDGE_LOOP ( 'NONE', ( #51569, #29489, #48492, #8599 ) ) ;
#42003=ORIENTED_EDGE ( 'NONE', *, *, #40655, .F. ) ;
#42004=CARTESIAN_POINT ( 'NONE',  ( -48.47912675150885065, -189.7472609257535510, 6.938893903907228378E-15 ) ) ;
#42006=CARTESIAN_POINT ( 'NONE',  ( 75.43907105790114542, -189.7472609257535510, -4.503971736580769658 ) ) ;
#42008=DIRECTION ( 'NONE',  ( 0.000000000000000000, 1.000000000000000000, -0.000000000000000000 ) ) ;
#42009=ORIENTED_EDGE ( 'NONE', *, *, #29211, .F. ) ;
#42010=ADVANCED_FACE ( 'NONE', ( #28212 ), #36893, .T. ) ;
#42012=VECTOR ( 'NONE', #6999, 1000.000000000000000 ) ;
#42014=LINE ( 'NONE', #6028, #34647 ) ;
#42015=EDGE_CURVE ( 'NONE', #30281, #7649, #8499, .T. ) ;
#42017=ADVANCED_FACE ( 'NONE', ( #40288 ), #48203, .T. ) ;
#42019=EDGE_CURVE ( 'NONE', #49683, #39625, #16403, .T. ) ;
#42020=DIRECTION ( 'NONE',  ( 0.8757349421956310831, 0.000000000000000000, 0.4827922027307550712 ) ) ;
#42021=ORIENTED_EDGE ( 'NONE', *, *, #41916, .T. ) ;
#42022=EDGE_CURVE ( 'NONE', #45184, #9630, #4842, .T. ) ;
#42023=FACE_OUTER_BOUND ( 'NONE', #13083, .T. ) ;
#42024=ORIENTED_EDGE ( 'NONE', *, *, #22980, .F. ) ;
#42026=ORIENTED_EDGE ( 'NONE', *, *, #23151, .T. ) ;
#42028=DIRECTION ( 'NONE',  ( 0.000000000000000000, 0.000000000000000000, 1.000000000000000000 ) ) ;
#42030=EDGE_CURVE ( 'NONE', #6199, #44148, #8248, .T. ) ;
#42031=EDGE_CURVE ( 'NONE', #30689, #24824, #5267, .T. ) ;
#42032=CIRCLE ( 'NONE', #23581, 125.0000000000000000 ) ;
#42033=DIRECTION ( 'NONE',  ( 0.000000000000000000, -0.000000000000000000, -1.000000000000000000 ) ) ;
#42038=ORIENTED_EDGE ( 'NONE', *, *, #28113, .T. ) ;
#42039=EDGE_CURVE ( 'NONE', #33788, #10029, #16920, .T. ) ;
#42040=DIRECTION ( 'NONE',  ( 0.000000000000000000, -1.000000000000000000, 0.000000000000000000 ) ) ;
#42041=VERTEX_POINT ( 'NONE', #45049 ) ;
#42043=ORIENTED_EDGE ( 'NONE', *, *, #19191, .F. ) ;
#42044=ADVANCED_FACE ( 'NONE', ( #32419 ), #48722, .F. ) ;
#42045=CARTESIAN_POINT ( 'NONE',  ( -48.07600332222087758, -177.1207230881787780, -0.9151456172430111335 ) ) ;
#42047=DIRECTION ( 'NONE',  ( 0.000000000000000000, 0.000000000000000000, 1.000000000000000000 ) ) ;
#42048=EDGE_LOOP ( 'NONE', ( #28392, #13605, #30927, #50830 ) ) ;
#42050=EDGE_CURVE ( 'NONE', #27166, #32896, #45553, .T. ) ;
#42051=FACE_OUTER_BOUND ( 'NONE', #747, .T. ) ;
#42052=ORIENTED_EDGE ( 'NONE', *, *, #49706, .F. ) ;
#42053=DIRECTION ( 'NONE',  ( 0.000000000000000000, 1.000000000000000000, -0.000000000000000000 ) ) ;
#42056=ORIENTED_EDGE ( 'NONE', *, *, #11312, .T. ) ;
#42057=FACE_OUTER_BOUND ( 'NONE', #11590, .T. ) ;
#42063=FACE_OUTER_BOUND ( 'NONE', #49785, .T. ) ;
#42064=EDGE_CURVE ( 'NONE', #35839, #44743, #17179, .T. ) ;
#42065=LINE ( 'NONE', #38635, #34882 ) ;
#42066=ADVANCED_FACE ( 'NONE', ( #36361 ), #13240, .T. ) ;
#42067=DIRECTION ( 'NONE',  ( 0.000000000000000000, 0.000000000000000000, 1.000000000000000000 ) ) ;
#42068=ORIENTED_EDGE ( 'NONE', *, *, #11521, .T. ) ;
#42069=CARTESIAN_POINT ( 'NONE',  ( -172.1767935149754294, -183.6283474603465606, 8.665274887906315726 ) ) ;
#42070=DIRECTION ( 'NONE',  ( -0.000000000000000000, 1.000000000000000000, -0.000000000000000000 ) ) ;
#42071=AXIS2_PLACEMENT_3D ( 'NONE', #36121, #15912, #15137 ) ;
#42072=CARTESIAN_POINT ( 'NONE',  ( -48.47912675150885065, -189.7472609257535510, 6.938893903907228378E-15 ) ) ;
#42074=VECTOR ( 'NONE', #43169, 1000.000000000000000 ) ;
#42075=CARTESIAN_POINT ( 'NONE',  ( 53.62339707355158680, -177.1207230881787780, -70.36529243996334060 ) ) ;
#42076=CARTESIAN_POINT ( 'NONE',  ( -171.2727421180348415, -183.6283474603465606, 23.38221600314377113 ) ) ;
#42077=FACE_OUTER_BOUND ( 'NONE', #35610, .T. ) ;
#42078=CARTESIAN_POINT ( 'NONE',  ( 66.36634345758743336, -193.5000000000000000, 46.76022031560705017 ) ) ;
#42080=ADVANCED_FACE ( 'NONE', ( #7987 ), #16145, .T. ) ;
#42081=EDGE_CURVE ( 'NONE', #19338, #32588, #50227, .T. ) ;
#42082=CARTESIAN_POINT ( 'NONE',  ( 68.24201764719070695, -183.6283474603465606, -44.73448837594909833 ) ) ;
#42083=CIRCLE ( 'NONE', #3478, 125.0000000000000000 ) ;
#42084=ADVANCED_FACE ( 'NONE', ( #14219 ), #46528, .T. ) ;
#42086=DIRECTION ( 'NONE',  ( 0.000000000000000000, 0.000000000000000000, -1.000000000000000000 ) ) ;
#42094=CARTESIAN_POINT ( 'NONE',  ( 74.49773146996547268, -177.1207230881787780, -22.39848972532282190 ) ) ;
#42097=DIRECTION ( 'NONE',  ( -0.5085311186492094127, 0.000000000000000000, -0.8610436117673619938 ) ) ;
#42099=EDGE_LOOP ( 'NONE', ( #21844, #23042, #20025, #40057 ) ) ;
#42100=DIRECTION ( 'NONE',  ( 0.000000000000000000, 0.000000000000000000, 1.000000000000000000 ) ) ;
#42101=EDGE_LOOP ( 'NONE', ( #36220, #25472, #28320, #17201 ) ) ;
#42102=DIRECTION ( 'NONE',  ( -0.000000000000000000, 1.000000000000000000, -0.000000000000000000 ) ) ;
#42103=AXIS2_PLACEMENT_3D ( 'NONE', #16607, #28136, #11853 ) ;
#42105=CARTESIAN_POINT ( 'NONE',  ( 6.443011874827240248, -183.6283474603465606, 112.2878385610370771 ) ) ;
#42106=LINE ( 'NONE', #26338, #31345 ) ;
#42107=VECTOR ( 'NONE', #35857, 1000.000000000000114 ) ;
#42109=EDGE_CURVE ( 'NONE', #48626, #10132, #26800, .T. ) ;
#42110=VECTOR ( 'NONE', #13708, 1000.000000000000000 ) ;
#42112=CARTESIAN_POINT ( 'NONE',  ( -172.6359455740846442, -177.1207230881787780, -14.49428645563791562 ) ) ;
#42113=CARTESIAN_POINT ( 'NONE',  ( 26.70958190211001337, -189.7472609257535510, -99.85818990449013199 ) ) ;
#42118=CIRCLE ( 'NONE', #47166, 125.0000000000000000 ) ;
#42121=DIRECTION ( 'NONE',  ( 0.7575112421616145841, 0.000000000000000000, 0.6528221181905280446 ) ) ;
#42123=VECTOR ( 'NONE', #46308, 1000.000000000000114 ) ;
#42125=CARTESIAN_POINT ( 'NONE',  ( -43.48323084606168720, -183.6283474603465606, 123.9001241957026167 ) ) ;
#42126=CARTESIAN_POINT ( 'NONE',  ( -118.9967449635792462, -175.3837268820161057, -103.2098131075562009 ) ) ;
#42128=CARTESIAN_POINT ( 'NONE',  ( -169.9131040279660567, -177.1207230881787780, 29.64437826672837417 ) ) ;
#42129=DIRECTION ( 'NONE',  ( -0.9890401873221644768, 0.000000000000000000, 0.1476465640024779702 ) ) ;
#42130=DIRECTION ( 'NONE',  ( -0.000000000000000000, 1.000000000000000000, -0.000000000000000000 ) ) ;
#42133=ORIENTED_EDGE ( 'NONE', *, *, #33005, .T. ) ;
#42136=CARTESIAN_POINT ( 'NONE',  ( 76.01188277843579044, -193.5000000000000000, 11.26891947860284482 ) ) ;
#42137=ORIENTED_EDGE ( 'NONE', *, *, #44486, .F. ) ;
#42138=AXIS2_PLACEMENT_3D ( 'NONE', #12714, #4584, #29001 ) ;
#42139=VERTEX_POINT ( 'NONE', #15242 ) ;
#42141=DIRECTION ( 'NONE',  ( -0.000000000000000000, 1.000000000000000000, -0.000000000000000000 ) ) ;
#42142=AXIS2_PLACEMENT_3D ( 'NONE', #41491, #44421, #24968 ) ;
#42143=DIRECTION ( 'NONE',  ( -0.000000000000000000, 1.000000000000000000, -0.000000000000000000 ) ) ;
#42146=ORIENTED_EDGE ( 'NONE', *, *, #39104, .F. ) ;
#42149=CARTESIAN_POINT ( 'NONE',  ( 69.88207517204676833, -175.3837268820161057, 40.19484891390057868 ) ) ;
#42152=AXIS2_PLACEMENT_3D ( 'NONE', #11820, #8932, #3956 ) ;
#42155=ORIENTED_EDGE ( 'NONE', *, *, #28624, .T. ) ;
#42156=DIRECTION ( 'NONE',  ( 0.000000000000000000, 0.000000000000000000, 1.000000000000000000 ) ) ;
#42158=AXIS2_PLACEMENT_3D ( 'NONE', #31202, #31974, #11996 ) ;
#42161=PLANE ( 'NONE',  #3557 ) ;
#42162=LINE ( 'NONE', #6446, #28038 ) ;
#42163=ORIENTED_EDGE ( 'NONE', *, *, #1352, .T. ) ;
#42164=DIRECTION ( 'NONE',  ( -0.8124868780056783146, 0.000000000000000000, -0.5829794791144762289 ) ) ;
#42165=VERTEX_POINT ( 'NONE', #31004 ) ;
#42167=VERTEX_POINT ( 'NONE', #38105 ) ;
#42168=CARTESIAN_POINT ( 'NONE',  ( -121.8391548840036620, -177.1207230881787780, -99.97252634603250954 ) ) ;
#42169=CARTESIAN_POINT ( 'NONE',  ( -63.96873441216509093, -189.7472609257535510, -123.0287672223651612 ) ) ;
#42171=DIRECTION ( 'NONE',  ( 0.000000000000000000, 1.000000000000000000, 0.000000000000000000 ) ) ;
#42174=CARTESIAN_POINT ( 'NONE',  ( -98.62206515315352817, -189.7472609257535510, 113.4093733337831225 ) ) ;
#42176=ORIENTED_EDGE ( 'NONE', *, *, #42019, .F. ) ;
#42177=AXIS2_PLACEMENT_3D ( 'NONE', #6613, #42852, #42334 ) ;
#42178=ORIENTED_EDGE ( 'NONE', *, *, #37819, .F. ) ;
#42179=CARTESIAN_POINT ( 'NONE',  ( 70.68712318874649725, -183.6283474603465606, -37.74128873232327663 ) ) ;
#42181=DIRECTION ( 'NONE',  ( 0.000000000000000000, -1.000000000000000000, 0.000000000000000000 ) ) ;
#42183=CARTESIAN_POINT ( 'NONE',  ( 18.49541618049843095, -177.1207230881787780, 105.5434062319798159 ) ) ;
#42184=DIRECTION ( 'NONE',  ( -0.000000000000000000, 1.000000000000000000, -0.000000000000000000 ) ) ;
#42185=DIRECTION ( 'NONE',  ( -0.6528221181905174975, 0.000000000000000000, -0.7575112421616236880 ) ) ;
#42186=CARTESIAN_POINT ( 'NONE',  ( -127.6327502296859535, -183.6283474603465606, -95.45105364470086329 ) ) ;
#42187=CIRCLE ( 'NONE', #3592, 125.0000000000000000 ) ;
#42188=ADVANCED_FACE ( 'NONE', ( #42057 ), #43089, .T. ) ;
#42192=AXIS2_PLACEMENT_3D ( 'NONE', #30308, #1688, #30057 ) ;
#42193=FACE_OUTER_BOUND ( 'NONE', #30237, .T. ) ;
#42195=VERTEX_POINT ( 'NONE', #38885 ) ;
#42197=ADVANCED_FACE ( 'NONE', ( #50999 ), #7098, .T. ) ;
#42198=AXIS2_PLACEMENT_3D ( 'NONE', #6801, #14428, #22823 ) ;
#42199=ORIENTED_EDGE ( 'NONE', *, *, #40353, .F. ) ;
#42200=ADVANCED_FACE ( 'NONE', ( #6069 ), #2887, .T. ) ;
#42202=EDGE_CURVE ( 'NONE', #26145, #20663, #46029, .T. ) ;
#42204=DIRECTION ( 'NONE',  ( -0.7378332790417333475, 0.000000000000000000, 0.6749830015182038956 ) ) ;
#42205=ORIENTED_EDGE ( 'NONE', *, *, #31542, .F. ) ;
#42207=VECTOR ( 'NONE', #7548, 1000.000000000000000 ) ;
#42208=CARTESIAN_POINT ( 'NONE',  ( 75.52097166332622180, -183.6283474603465606, -0.3215015308240974368 ) ) ;
#42209=PLANE ( 'NONE',  #34899 ) ;
#42211=EDGE_LOOP ( 'NONE', ( #48246, #49076, #24032, #34178 ) ) ;
#42212=CIRCLE ( 'NONE', #38013, 125.0000000000000000 ) ;
#42215=DIRECTION ( 'NONE',  ( 0.000000000000000000, 0.000000000000000000, -1.000000000000000000 ) ) ;
#42216=EDGE_CURVE ( 'NONE', #26081, #12481, #26279, .T. ) ;
#42218=CARTESIAN_POINT ( 'NONE',  ( 41.00573479224730988, -183.6283474603465606, -87.27805883780176543 ) ) ;
#42220=ORIENTED_EDGE ( 'NONE', *, *, #7324, .T. ) ;
#42221=AXIS2_PLACEMENT_3D ( 'NONE', #44133, #8139, #20221 ) ;
#42224=ORIENTED_EDGE ( 'NONE', *, *, #10581, .F. ) ;
#42226=ORIENTED_EDGE ( 'NONE', *, *, #22093, .T. ) ;
#42227=AXIS2_PLACEMENT_3D ( 'NONE', #23714, #20031, #43944 ) ;
#42229=LINE ( 'NONE', #8691, #27462 ) ;
#42230=EDGE_LOOP ( 'NONE', ( #21246, #2465, #50926, #34225 ) ) ;
#42231=CARTESIAN_POINT ( 'NONE',  ( -81.14588623932564815, -183.6283474603465606, 120.6560517527617833 ) ) ;
#42234=VECTOR ( 'NONE', #18043, 1000.000000000000114 ) ;
#42236=CARTESIAN_POINT ( 'NONE',  ( -18.31235070009513421, -193.5000000000000000, 121.3052580173829966 ) ) ;
#42238=ORIENTED_EDGE ( 'NONE', *, *, #48371, .F. ) ;
#42239=CARTESIAN_POINT ( 'NONE',  ( -73.94077438226447896, -193.5000000000000000, 122.3793467049372481 ) ) ;
#42241=CARTESIAN_POINT ( 'NONE',  ( -130.2106798473772642, -193.5000000000000000, 94.57776286494217288 ) ) ;
#42242=DIRECTION ( 'NONE',  ( 0.000000000000000000, 1.000000000000000000, 0.000000000000000000 ) ) ;
#42243=VERTEX_POINT ( 'NONE', #50732 ) ;
#42244=FACE_OUTER_BOUND ( 'NONE', #48672, .T. ) ;
#42245=VECTOR ( 'NONE', #11411, 1000.000000000000000 ) ;
#42246=DIRECTION ( 'NONE',  ( -0.5085311186492273983, 0.000000000000000000, 0.8610436117673514467 ) ) ;
#42247=EDGE_CURVE ( 'NONE', #19688, #39351, #6323, .T. ) ;
#42248=EDGE_CURVE ( 'NONE', #8523, #22453, #23128, .T. ) ;
#42250=CARTESIAN_POINT ( 'NONE',  ( 14.43219681437621205, -193.5000000000000000, 106.8558168688117860 ) ) ;
#42251=LINE ( 'NONE', #18361, #2734 ) ;
#42253=FACE_OUTER_BOUND ( 'NONE', #29781, .T. ) ;
#42254=FACE_OUTER_BOUND ( 'NONE', #46976, .T. ) ;
#42255=CIRCLE ( 'NONE', #24623, 125.0000000000000000 ) ;
#42257=ORIENTED_EDGE ( 'NONE', *, *, #7568, .F. ) ;
#42258=DIRECTION ( 'NONE',  ( -0.000000000000000000, 1.000000000000000000, -0.000000000000000000 ) ) ;
#42260=VERTEX_POINT ( 'NONE', #22347 ) ;
#42261=DIRECTION ( 'NONE',  ( 0.000000000000000000, 0.000000000000000000, -1.000000000000000000 ) ) ;
#42262=EDGE_CURVE ( 'NONE', #21231, #17420, #32283, .T. ) ;
#42263=VECTOR ( 'NONE', #10833, 1000.000000000000227 ) ;
#42264=ORIENTED_EDGE ( 'NONE', *, *, #16533, .F. ) ;
#42267=VECTOR ( 'NONE', #10960, 1000.000000000000000 ) ;
#42268=EDGE_CURVE ( 'NONE', #15701, #875, #48335, .T. ) ;
#42269=FACE_OUTER_BOUND ( 'NONE', #37447, .T. ) ;
#42271=EDGE_CURVE ( 'NONE', #29853, #3, #47825, .T. ) ;
#42272=DIRECTION ( 'NONE',  ( -0.000000000000000000, 1.000000000000000000, -0.000000000000000000 ) ) ;
#42276=ORIENTED_EDGE ( 'NONE', *, *, #14402, .F. ) ;
#42277=DIRECTION ( 'NONE',  ( 0.9960498426152165630, 0.000000000000000000, 0.08879589532293852283 ) ) ;
#42279=CARTESIAN_POINT ( 'NONE',  ( 12.99855592850622443, -193.5000000000000000, 108.8370090194294875 ) ) ;
#42280=VECTOR ( 'NONE', #50943, 1000.000000000000114 ) ;
#42281=AXIS2_PLACEMENT_3D ( 'NONE', #33278, #20942, #33009 ) ;
#42282=CARTESIAN_POINT ( 'NONE',  ( -49.44376233341720450, -189.7472609257535510, -0.2635871660690713436 ) ) ;
#42283=CARTESIAN_POINT ( 'NONE',  ( -48.47912675150885065, -175.3837268820161057, 6.938893903907228378E-15 ) ) ;
#42284=VERTEX_POINT ( 'NONE', #7366 ) ;
#42285=PLANE ( 'NONE',  #16630 ) ;
#42286=DIRECTION ( 'NONE',  ( -0.000000000000000000, 1.000000000000000000, -0.000000000000000000 ) ) ;
#42287=ORIENTED_EDGE ( 'NONE', *, *, #7454, .T. ) ;
#42290=CARTESIAN_POINT ( 'NONE',  ( -48.41988612361514299, -175.3837268820161057, -0.9982437317643144681 ) ) ;
#42291=ORIENTED_EDGE ( 'NONE', *, *, #20144, .F. ) ;
#42293=DIRECTION ( 'NONE',  ( -0.000000000000000000, 1.000000000000000000, -0.000000000000000000 ) ) ;
#42294=PLANE ( 'NONE',  #43454 ) ;
#42295=EDGE_LOOP ( 'NONE', ( #31212, #22675, #32966, #36535 ) ) ;
#42297=ORIENTED_EDGE ( 'NONE', *, *, #2754, .T. ) ;
#42298=CARTESIAN_POINT ( 'NONE',  ( -48.47912675150885065, -175.3837268820161057, 6.938893903907228378E-15 ) ) ;
#42302=ORIENTED_EDGE ( 'NONE', *, *, #16231, .F. ) ;
#42304=DIRECTION ( 'NONE',  ( -0.000000000000000000, 1.000000000000000000, -0.000000000000000000 ) ) ;
#42306=DIRECTION ( 'NONE',  ( -0.000000000000000000, 1.000000000000000000, -0.000000000000000000 ) ) ;
#42307=CYLINDRICAL_SURFACE ( 'NONE', #21754, 125.0000000000000000 ) ;
#42308=FACE_OUTER_BOUND ( 'NONE', #42486, .T. ) ;
#42309=EDGE_CURVE ( 'NONE', #16252, #30647, #3658, .T. ) ;
#42310=EDGE_CURVE ( 'NONE', #10147, #14417, #1169, .T. ) ;
#42311=ORIENTED_EDGE ( 'NONE', *, *, #2511, .T. ) ;
#42312=EDGE_CURVE ( 'NONE', #18236, #27224, #44400, .T. ) ;
#42314=CARTESIAN_POINT ( 'NONE',  ( -114.1105527140175155, -183.6283474603465606, 106.3838142112217611 ) ) ;
#42315=LINE ( 'NONE', #23138, #28120 ) ;
#42316=EDGE_CURVE ( 'NONE', #21288, #18537, #5397, .T. ) ;
#42319=DIRECTION ( 'NONE',  ( -0.000000000000000000, 1.000000000000000000, -0.000000000000000000 ) ) ;
#42321=DIRECTION ( 'NONE',  ( 0.8858462335218260097, 0.000000000000000000, -0.4639789333096864810 ) ) ;
#42322=EDGE_CURVE ( 'NONE', #25437, #47778, #35450, .T. ) ;
#42323=AXIS2_PLACEMENT_3D ( 'NONE', #29064, #40623, #17263 ) ;
#42324=VECTOR ( 'NONE', #38306, 1000.000000000000000 ) ;
#42325=DIRECTION ( 'NONE',  ( -0.000000000000000000, 1.000000000000000000, 0.000000000000000000 ) ) ;
#42327=VERTEX_POINT ( 'NONE', #51768 ) ;
#42328=ADVANCED_FACE ( 'NONE', ( #27821 ), #23886, .F. ) ;
#42329=AXIS2_PLACEMENT_3D ( 'NONE', #51391, #39532, #43497 ) ;
#42334=DIRECTION ( 'NONE',  ( 0.000000000000000000, -0.000000000000000000, -1.000000000000000000 ) ) ;
#42336=ADVANCED_FACE ( 'NONE', ( #227 ), #16270, .T. ) ;
#42339=CARTESIAN_POINT ( 'NONE',  ( -163.4524646452520926, -175.3837268820161057, 46.44493303993096589 ) ) ;
#42340=EDGE_CURVE ( 'NONE', #39776, #32877, #43973, .T. ) ;
#42341=CARTESIAN_POINT ( 'NONE',  ( -48.47912675150885065, -183.6283474603465606, 6.938893903907228378E-15 ) ) ;
#42342=DIRECTION ( 'NONE',  ( -6.978251959525016136E-17, 0.000000000000000000, 1.000000000000000000 ) ) ;
#42343=ORIENTED_EDGE ( 'NONE', *, *, #44786, .F. ) ;
#42344=VERTEX_POINT ( 'NONE', #20463 ) ;
#42345=ORIENTED_EDGE ( 'NONE', *, *, #21600, .T. ) ;
#42347=DIRECTION ( 'NONE',  ( -0.000000000000000000, 1.000000000000000000, -0.000000000000000000 ) ) ;
#42348=CARTESIAN_POINT ( 'NONE',  ( -55.05561436132770581, -175.3837268820161057, 124.8268793598474105 ) ) ;
#42351=DIRECTION ( 'NONE',  ( 0.000000000000000000, -1.000000000000000000, -0.000000000000000000 ) ) ;
#42352=CARTESIAN_POINT ( 'NONE',  ( 70.02079272397770637, -177.1207230881787780, -36.52255268223056106 ) ) ;
#42353=CARTESIAN_POINT ( 'NONE',  ( -47.92047998570519951, -189.7472609257535510, -0.8294056854501942189 ) ) ;
#42355=VERTEX_POINT ( 'NONE', #33073 ) ;
#42357=VECTOR ( 'NONE', #14980, 1000.000000000000114 ) ;
#42360=ORIENTED_EDGE ( 'NONE', *, *, #48777, .T. ) ;
#42361=AXIS2_PLACEMENT_3D ( 'NONE', #24672, #17589, #17070 ) ;
#42362=DIRECTION ( 'NONE',  ( 0.9027978299657416494, 0.000000000000000000, 0.4300652022765245608 ) ) ;
#42363=DIRECTION ( 'NONE',  ( 0.000000000000000000, 0.000000000000000000, 1.000000000000000000 ) ) ;
#42364=CARTESIAN_POINT ( 'NONE',  ( -48.30223647638628393, -175.3837268820161057, 0.9842305779476049343 ) ) ;
#42365=AXIS2_PLACEMENT_3D ( 'NONE', #3611, #51459, #6796 ) ;
#42368=DIRECTION ( 'NONE',  ( -0.000000000000000000, 1.000000000000000000, -0.000000000000000000 ) ) ;
#42369=LINE ( 'NONE', #6389, #30059 ) ;
#42370=ORIENTED_EDGE ( 'NONE', *, *, #39759, .F. ) ;
#42371=AXIS2_PLACEMENT_3D ( 'NONE', #28840, #465, #209 ) ;
#42374=CARTESIAN_POINT ( 'NONE',  ( -25.55153130240594450, -189.7472609257535510, 122.8793122007210599 ) ) ;
#42376=EDGE_CURVE ( 'NONE', #33013, #46176, #5763, .T. ) ;
#42380=AXIS2_PLACEMENT_3D ( 'NONE', #21357, #36874, #1386 ) ;
#42382=EDGE_CURVE ( 'NONE', #1918, #38465, #1013, .T. ) ;
#42383=ORIENTED_EDGE ( 'NONE', *, *, #6154, .T. ) ;
#42386=CARTESIAN_POINT ( 'NONE',  ( -140.5933766095837427, -189.7472609257535510, -84.49831343337066869 ) ) ;
#42387=CARTESIAN_POINT ( 'NONE',  ( -121.0298553105864130, -183.6283474603465606, -100.5610240384919223 ) ) ;
#42388=EDGE_LOOP ( 'NONE', ( #16968, #49919, #1783, #23502 ) ) ;
#42389=DIRECTION ( 'NONE',  ( -0.000000000000000000, -1.000000000000000000, 0.000000000000000000 ) ) ;
#42390=DIRECTION ( 'NONE',  ( -0.000000000000000000, -1.000000000000000000, 0.000000000000000000 ) ) ;
#42391=DIRECTION ( 'NONE',  ( -0.000000000000000000, 1.000000000000000000, -0.000000000000000000 ) ) ;
#42395=VECTOR ( 'NONE', #8977, 1000.000000000000000 ) ;
#42396=ADVANCED_FACE ( 'NONE', ( #40680 ), #40956, .T. ) ;
#42397=LINE ( 'NONE', #15084, #18559 ) ;
#42399=CARTESIAN_POINT ( 'NONE',  ( -87.28630321566649286, -177.1207230881787780, 118.8234112238818341 ) ) ;
#42401=VECTOR ( 'NONE', #2871, 1000.000000000000114 ) ;
#42402=VECTOR ( 'NONE', #50029, 1000.000000000000000 ) ;
#42404=ORIENTED_EDGE ( 'NONE', *, *, #4867, .T. ) ;
#42405=CARTESIAN_POINT ( 'NONE',  ( -164.6073096293132494, -183.6283474603465606, 43.47841891815207305 ) ) ;
#42406=CIRCLE ( 'NONE', #48300, 125.0000000000000000 ) ;
#42407=EDGE_CURVE ( 'NONE', #44579, #47358, #2857, .T. ) ;
#42409=EDGE_LOOP ( 'NONE', ( #50132, #29618, #10811, #5924 ) ) ;
#42413=DIRECTION ( 'NONE',  ( -0.000000000000000000, 1.000000000000000000, -0.000000000000000000 ) ) ;
#42416=LINE ( 'NONE', #35300, #7650 ) ;
#42417=VECTOR ( 'NONE', #43842, 1000.000000000000000 ) ;
#42419=ORIENTED_EDGE ( 'NONE', *, *, #38587, .F. ) ;
#42420=EDGE_LOOP ( 'NONE', ( #3681, #14039, #1889, #22992 ) ) ;
#42421=ORIENTED_EDGE ( 'NONE', *, *, #42268, .T. ) ;
#42422=CIRCLE ( 'NONE', #49152, 125.0000000000000000 ) ;
#42424=CARTESIAN_POINT ( 'NONE',  ( -48.47912675150885065, -193.5000000000000000, 6.938893903907228378E-15 ) ) ;
#42425=CARTESIAN_POINT ( 'NONE',  ( 62.86098202833237281, -193.5000000000000000, 56.81883646197908178 ) ) ;
#42426=CARTESIAN_POINT ( 'NONE',  ( -48.47912675150885065, -175.3837268820161057, 6.938893903907228378E-15 ) ) ;
#42427=ORIENTED_EDGE ( 'NONE', *, *, #472, .F. ) ;
#42428=CYLINDRICAL_SURFACE ( 'NONE', #25689, 125.0000000000000000 ) ;
#42430=ORIENTED_EDGE ( 'NONE', *, *, #24709, .F. ) ;
#42431=AXIS2_PLACEMENT_3D ( 'NONE', #51262, #15249, #50235 ) ;
#42432=DIRECTION ( 'NONE',  ( -0.000000000000000000, 1.000000000000000000, -0.000000000000000000 ) ) ;
#42433=CARTESIAN_POINT ( 'NONE',  ( -48.47912675150885065, -183.6283474603465606, 6.938893903907228378E-15 ) ) ;
#42434=VECTOR ( 'NONE', #24013, 1000.000000000000227 ) ;
#42435=AXIS2_PLACEMENT_3D ( 'NONE', #26811, #42842, #46540 ) ;
#42436=CARTESIAN_POINT ( 'NONE',  ( 75.46126020185812422, -189.7472609257535510, 3.844569333773204534 ) ) ;
#42437=EDGE_CURVE ( 'NONE', #51204, #18822, #9587, .T. ) ;
#42440=ORIENTED_EDGE ( 'NONE', *, *, #6428, .T. ) ;
#42441=DIRECTION ( 'NONE',  ( 0.000000000000000000, 0.000000000000000000, 1.000000000000000000 ) ) ;
#42443=DIRECTION ( 'NONE',  ( -0.05924062789370748011, 0.000000000000000000, -0.9982437317643217956 ) ) ;
#42445=CARTESIAN_POINT ( 'NONE',  ( -48.30901192927175458, -175.3837268820161057, -124.9998842437354227 ) ) ;
#42446=EDGE_LOOP ( 'NONE', ( #47004, #40923, #23818, #17756 ) ) ;
#42447=VECTOR ( 'NONE', #10746, 1000.000000000000000 ) ;
#42448=DIRECTION ( 'NONE',  ( 0.000000000000000000, 0.000000000000000000, 1.000000000000000000 ) ) ;
#42449=CARTESIAN_POINT ( 'NONE',  ( -8.169009709621407822, -193.5000000000000000, 118.3219948448695504 ) ) ;
#42451=AXIS2_PLACEMENT_3D ( 'NONE', #51556, #3217, #31573 ) ;
#42453=CARTESIAN_POINT ( 'NONE',  ( -47.78257572244586271, -193.5000000000000000, 0.7175072570443418174 ) ) ;
#42457=DIRECTION ( 'NONE',  ( 0.000000000000000000, 0.000000000000000000, 1.000000000000000000 ) ) ;
#42458=ORIENTED_EDGE ( 'NONE', *, *, #27566, .F. ) ;
#42459=VERTEX_POINT ( 'NONE', #9429 ) ;
#42462=EDGE_CURVE ( 'NONE', #14296, #26111, #23012, .T. ) ;
#42464=VECTOR ( 'NONE', #16816, 1000.000000000000000 ) ;
#42465=VECTOR ( 'NONE', #7297, 1000.000000000000000 ) ;
#42466=ORIENTED_EDGE ( 'NONE', *, *, #2798, .F. ) ;
#42467=DIRECTION ( 'NONE',  ( -0.000000000000000000, -1.000000000000000000, 0.000000000000000000 ) ) ;
#42470=DIRECTION ( 'NONE',  ( 0.000000000000000000, -1.000000000000000000, 0.000000000000000000 ) ) ;
#42472=CIRCLE ( 'NONE', #27349, 125.0000000000000000 ) ;
#42473=PLANE ( 'NONE',  #1731 ) ;
#42475=EDGE_LOOP ( 'NONE', ( #26769, #36065, #9845, #24497 ) ) ;
#42479=LINE ( 'NONE', #14636, #31037 ) ;
#42485=FACE_OUTER_BOUND ( 'NONE', #36211, .T. ) ;
#42486=EDGE_LOOP ( 'NONE', ( #16538, #11571, #47274, #13676 ) ) ;
#42488=EDGE_CURVE ( 'NONE', #21174, #41262, #32559, .T. ) ;
#42489=AXIS2_PLACEMENT_3D ( 'NONE', #8180, #20790, #283 ) ;
#42490=DIRECTION ( 'NONE',  ( -0.1182731709213730997, 0.000000000000000000, 0.9929810960135161402 ) ) ;
#42492=FACE_OUTER_BOUND ( 'NONE', #21963, .T. ) ;
#42495=PLANE ( 'NONE',  #36699 ) ;
#42496=VERTEX_POINT ( 'NONE', #28602 ) ;
#42497=FACE_OUTER_BOUND ( 'NONE', #8194, .T. ) ;
#42498=DIRECTION ( 'NONE',  ( 0.000000000000000000, -1.000000000000000000, 0.000000000000000000 ) ) ;
#42499=ADVANCED_FACE ( 'NONE', ( #32815 ), #37544, .T. ) ;
#42500=DIRECTION ( 'NONE',  ( 0.4566292373937077542, 0.000000000000000000, 0.8896570909947499883 ) ) ;
#42501=VERTEX_POINT ( 'NONE', #48865 ) ;
#42502=CARTESIAN_POINT ( 'NONE',  ( -48.47912675150885065, -175.3837268820161057, 6.938893903907228378E-15 ) ) ;
#42503=EDGE_LOOP ( 'NONE', ( #46951, #38796, #44216, #37006 ) ) ;
#42504=ORIENTED_EDGE ( 'NONE', *, *, #26685, .T. ) ;
#42507=VECTOR ( 'NONE', #23838, 1000.000000000000000 ) ;
#42508=CARTESIAN_POINT ( 'NONE',  ( -172.4422607493951318, -177.1207230881787780, 16.06677968424543579 ) ) ;
#42510=CARTESIAN_POINT ( 'NONE',  ( -49.46816693883101834, -183.6283474603465606, 0.1476465640024780257 ) ) ;
#42511=ORIENTED_EDGE ( 'NONE', *, *, #17747, .F. ) ;
#42512=CARTESIAN_POINT ( 'NONE',  ( -168.8371699641976420, -175.3837268820161057, 33.74820638215509661 ) ) ;
#42513=CARTESIAN_POINT ( 'NONE',  ( -100.6109117578262868, -193.5000000000000000, 112.5098962032393644 ) ) ;
#42515=CARTESIAN_POINT ( 'NONE',  ( -48.47912675150885065, -183.6283474603465606, 6.938893903907228378E-15 ) ) ;
#42518=CARTESIAN_POINT ( 'NONE',  ( -166.1003692892502102, -183.6283474603465606, -42.31126686685032467 ) ) ;
#42522=VECTOR ( 'NONE', #10843, 1000.000000000000114 ) ;
#42524=ADVANCED_FACE ( 'NONE', ( #14660 ), #38044, .T. ) ;
#42525=AXIS2_PLACEMENT_3D ( 'NONE', #10980, #14671, #50945 ) ;
#42527=CARTESIAN_POINT ( 'NONE',  ( -169.1033029113419559, -175.3837268820161057, 32.78426643622745473 ) ) ;
#42528=ORIENTED_EDGE ( 'NONE', *, *, #14105, .T. ) ;
#42529=CARTESIAN_POINT ( 'NONE',  ( 68.93474881819258826, -175.3837268820161057, 39.87457906003773900 ) ) ;
#42533=DIRECTION ( 'NONE',  ( -0.8757349421956379665, 0.000000000000000000, 0.4827922027307427477 ) ) ;
#42535=DIRECTION ( 'NONE',  ( -0.000000000000000000, 1.000000000000000000, -0.000000000000000000 ) ) ;
#42537=FACE_OUTER_BOUND ( 'NONE', #13202, .T. ) ;
#42540=ORIENTED_EDGE ( 'NONE', *, *, #21802, .F. ) ;
#42541=CARTESIAN_POINT ( 'NONE',  ( -168.4003408533108086, -177.1207230881787780, -35.26900067126609173 ) ) ;
#42542=AXIS2_PLACEMENT_3D ( 'NONE', #12973, #21126, #21389 ) ;
#42543=AXIS2_PLACEMENT_3D ( 'NONE', #10531, #46547, #15256 ) ;
#42544=ORIENTED_EDGE ( 'NONE', *, *, #43744, .F. ) ;
#42545=DIRECTION ( 'NONE',  ( -0.000000000000000000, 1.000000000000000000, -0.000000000000000000 ) ) ;
#42546=AXIS2_PLACEMENT_3D ( 'NONE', #47388, #4270, #20292 ) ;
#42547=EDGE_CURVE ( 'NONE', #38590, #5830, #6248, .T. ) ;
#42548=EDGE_CURVE ( 'NONE', #3342, #17596, #29906, .T. ) ;
#42549=DIRECTION ( 'NONE',  ( 0.000000000000000000, 1.000000000000000000, 0.000000000000000000 ) ) ;
#42550=LINE ( 'NONE', #50205, #18083 ) ;
#42551=EDGE_LOOP ( 'NONE', ( #43013, #48120, #40909, #47519 ) ) ;
#42553=DIRECTION ( 'NONE',  ( 0.000000000000000000, 0.000000000000000000, 1.000000000000000000 ) ) ;
#42554=ORIENTED_EDGE ( 'NONE', *, *, #26880, .T. ) ;
#42555=AXIS2_PLACEMENT_3D ( 'NONE', #14625, #34336, #30133 ) ;
#42556=CIRCLE ( 'NONE', #47643, 125.0000000000000000 ) ;
#42557=AXIS2_PLACEMENT_3D ( 'NONE', #13740, #17446, #1660 ) ;
#42558=CARTESIAN_POINT ( 'NONE',  ( -67.10529315269985773, -177.1207230881787780, -122.5936119678274423 ) ) ;
#42559=EDGE_LOOP ( 'NONE', ( #12412, #13555, #36538, #25135 ) ) ;
#42560=CARTESIAN_POINT ( 'NONE',  ( 55.10060313344061456, -183.6283474603465606, 68.17212999877223467 ) ) ;
#42561=ORIENTED_EDGE ( 'NONE', *, *, #17473, .T. ) ;
#42562=EDGE_CURVE ( 'NONE', #21060, #35361, #14935, .T. ) ;
#42565=CARTESIAN_POINT ( 'NONE',  ( -161.6832731452239784, -193.5000000000000000, -53.00774697410100345 ) ) ;
#42566=DIRECTION ( 'NONE',  ( -0.1768902751225592818, 0.000000000000000000, -0.9842305779475992722 ) ) ;
#42567=ORIENTED_EDGE ( 'NONE', *, *, #23560, .F. ) ;
#42569=EDGE_CURVE ( 'NONE', #11314, #28854, #7035, .T. ) ;
#42571=AXIS2_PLACEMENT_3D ( 'NONE', #51494, #43851, #15493 ) ;
#42572=LINE ( 'NONE', #10014, #36597 ) ;
#42575=EDGE_CURVE ( 'NONE', #45145, #29008, #34373, .T. ) ;
#42578=DIRECTION ( 'NONE',  ( -0.000000000000000000, 1.000000000000000000, -0.000000000000000000 ) ) ;
#42580=LINE ( 'NONE', #2889, #40823 ) ;
#42581=FACE_OUTER_BOUND ( 'NONE', #21242, .T. ) ;
#42582=LINE ( 'NONE', #26804, #50937 ) ;
#42583=VERTEX_POINT ( 'NONE', #25969 ) ;
#42589=VECTOR ( 'NONE', #47236, 1000.000000000000000 ) ;
#42593=CIRCLE ( 'NONE', #14924, 125.0000000000000000 ) ;
#42594=CARTESIAN_POINT ( 'NONE',  ( -48.47912675150885065, -177.1207230881787780, 6.938893903907228378E-15 ) ) ;
#42595=DIRECTION ( 'NONE',  ( 0.9646355819083576311, 0.000000000000000000, 0.2635871660690715101 ) ) ;
#42597=AXIS2_PLACEMENT_3D ( 'NONE', #22456, #30321, #14057 ) ;
#42598=CIRCLE ( 'NONE', #22472, 125.0000000000000000 ) ;
#42599=CARTESIAN_POINT ( 'NONE',  ( -40.90423906728906900, -189.7472609257535510, -124.7702732086912505 ) ) ;
#42600=CARTESIAN_POINT ( 'NONE',  ( -131.1972941934623975, -177.1207230881787780, 92.37913469314123915 ) ) ;
#42603=VERTEX_POINT ( 'NONE', #6000 ) ;
#42605=CARTESIAN_POINT ( 'NONE',  ( -47.97059563285962724, -193.5000000000000000, -0.8610436117673480050 ) ) ;
#42606=VECTOR ( 'NONE', #38144, 1000.000000000000114 ) ;
#42607=DIRECTION ( 'NONE',  ( 0.000000000000000000, 1.000000000000000000, -0.000000000000000000 ) ) ;
#42608=ORIENTED_EDGE ( 'NONE', *, *, #8415, .F. ) ;
#42609=VERTEX_POINT ( 'NONE', #30175 ) ;
#42612=EDGE_CURVE ( 'NONE', #12830, #5877, #14408, .T. ) ;
#42613=ADVANCED_FACE ( 'NONE', ( #51977 ), #15963, .T. ) ;
#42614=EDGE_CURVE ( 'NONE', #31046, #6126, #3599, .T. ) ;
#42615=DIRECTION ( 'NONE',  ( 0.5085311186492216251, 0.000000000000000000, -0.8610436117673548884 ) ) ;
#42616=DIRECTION ( 'NONE',  ( -0.000000000000000000, 1.000000000000000000, -0.000000000000000000 ) ) ;
#42617=ORIENTED_EDGE ( 'NONE', *, *, #46613, .F. ) ;
#42618=CARTESIAN_POINT ( 'NONE',  ( -160.3527926973206661, -175.3837268820161057, -53.48161459190840361 ) ) ;
#42620=VECTOR ( 'NONE', #23759, 1000.000000000000000 ) ;
#42621=CARTESIAN_POINT ( 'NONE',  ( -48.47912675150885065, -189.7472609257535510, 6.938893903907228378E-15 ) ) ;
#42622=FACE_OUTER_BOUND ( 'NONE', #43372, .T. ) ;
#42623=ORIENTED_EDGE ( 'NONE', *, *, #33303, .T. ) ;
#42626=PLANE ( 'NONE',  #27255 ) ;
#42628=CYLINDRICAL_SURFACE ( 'NONE', #38148, 125.0000000000000000 ) ;
#42629=AXIS2_PLACEMENT_3D ( 'NONE', #44746, #31876, #3495 ) ;
#42630=VERTEX_POINT ( 'NONE', #15708 ) ;
#42631=CARTESIAN_POINT ( 'NONE',  ( -133.0671220150036049, -183.6283474603465606, -92.03190238880749519 ) ) ;
#42633=CARTESIAN_POINT ( 'NONE',  ( -47.49008656418669005, -193.5000000000000000, -0.1476465640024710591 ) ) ;
#42634=CARTESIAN_POINT ( 'NONE',  ( -49.38192458147459263, -189.7472609257535510, -0.4300652022765235616 ) ) ;
#42635=EDGE_CURVE ( 'NONE', #47506, #48534, #16213, .T. ) ;
#42636=AXIS2_PLACEMENT_3D ( 'NONE', #23600, #15473, #38854 ) ;
#42637=ORIENTED_EDGE ( 'NONE', *, *, #45255, .F. ) ;
#42638=CARTESIAN_POINT ( 'NONE',  ( 4.109287492203097081, -183.6283474603465606, -113.3995532942337121 ) ) ;
#42639=ADVANCED_FACE ( 'NONE', ( #23829 ), #15184, .T. ) ;
#42640=LINE ( 'NONE', #22926, #5727 ) ;
#42641=ORIENTED_EDGE ( 'NONE', *, *, #20939, .T. ) ;
#42642=CARTESIAN_POINT ( 'NONE',  ( 69.14211578623219623, -193.5000000000000000, 42.31126686685117733 ) ) ;
#42644=EDGE_CURVE ( 'NONE', #6231, #22760, #31724, .T. ) ;
#42645=VERTEX_POINT ( 'NONE', #11992 ) ;
#42649=VERTEX_POINT ( 'NONE', #28020 ) ;
#42650=CARTESIAN_POINT ( 'NONE',  ( -162.9896759831413249, -193.5000000000000000, -50.12318939043961308 ) ) ;
#42651=EDGE_LOOP ( 'NONE', ( #35542, #37519, #32910, #18789 ) ) ;
#42652=CARTESIAN_POINT ( 'NONE',  ( -65.65563056894595206, -177.1207230881787780, 123.8142468240612857 ) ) ;
#42655=LINE ( 'NONE', #45829, #50046 ) ;
#42656=FACE_OUTER_BOUND ( 'NONE', #27145, .T. ) ;
#42657=DIRECTION ( 'NONE',  ( -0.9890401873221623674, 0.000000000000000000, -0.1476465640024917925 ) ) ;
#42658=ADVANCED_FACE ( 'NONE', ( #44061 ), #8065, .T. ) ;
#42660=CARTESIAN_POINT ( 'NONE',  ( 75.12566530717464275, -193.5000000000000000, 18.62405380494841367 ) ) ;
#42662=CIRCLE ( 'NONE', #1555, 124.9999999999999858 ) ;
#42664=CARTESIAN_POINT ( 'NONE',  ( 14.37129481273059106, -193.5000000000000000, -108.0501018472328241 ) ) ;
#42665=LINE ( 'NONE', #34762, #12590 ) ;
#42670=LINE ( 'NONE', #30843, #47596 ) ;
#42673=CIRCLE ( 'NONE', #48579, 125.0000000000000000 ) ;
#42675=CARTESIAN_POINT ( 'NONE',  ( 68.72094416275764672, -175.3837268820161057, -40.49875167738976955 ) ) ;
#42676=ORIENTED_EDGE ( 'NONE', *, *, #51003, .F. ) ;
#42679=EDGE_CURVE ( 'NONE', #27297, #39129, #51353, .T. ) ;
#42680=ADVANCED_FACE ( 'NONE', ( #45637 ), #8831, .T. ) ;
#42681=EDGE_CURVE ( 'NONE', #28401, #18318, #125, .T. ) ;
#42684=FACE_OUTER_BOUND ( 'NONE', #11804, .T. ) ;
#42685=VERTEX_POINT ( 'NONE', #13559 ) ;
#42686=ORIENTED_EDGE ( 'NONE', *, *, #32659, .T. ) ;
#42687=EDGE_CURVE ( 'NONE', #25337, #21157, #21188, .T. ) ;
#42689=CIRCLE ( 'NONE', #30905, 125.0000000000000000 ) ;
#42690=CARTESIAN_POINT ( 'NONE',  ( -9.671950287350391307, -183.6283474603465606, -118.8234112238815499 ) ) ;
#42691=DIRECTION ( 'NONE',  ( 0.000000000000000000, 0.000000000000000000, 1.000000000000000000 ) ) ;
#42693=LINE ( 'NONE', #39506, #41292 ) ;
#42695=VERTEX_POINT ( 'NONE', #40615 ) ;
#42698=DIRECTION ( 'NONE',  ( 0.000000000000000000, 0.000000000000000000, 1.000000000000000000 ) ) ;
#42699=CARTESIAN_POINT ( 'NONE',  ( 76.31829002442924548, -183.6283474603465606, 7.113702696402428138 ) ) ;
#42702=ORIENTED_EDGE ( 'NONE', *, *, #47796, .F. ) ;
#42703=PLANE ( 'NONE',  #5430 ) ;
#42704=CIRCLE ( 'NONE', #26754, 125.0000000000000000 ) ;
#42706=ADVANCED_FACE ( 'NONE', ( #1200 ), #28794, .T. ) ;
#42707=FACE_OUTER_BOUND ( 'NONE', #348, .T. ) ;
#42709=DIRECTION ( 'NONE',  ( 0.000000000000000000, 1.000000000000000000, 0.000000000000000000 ) ) ;
#42711=EDGE_CURVE ( 'NONE', #30763, #43156, #36701, .T. ) ;
#42716=EDGE_CURVE ( 'NONE', #6875, #29368, #33275, .T. ) ;
#42719=AXIS2_PLACEMENT_3D ( 'NONE', #2533, #46425, #9910 ) ;
#42720=DIRECTION ( 'NONE',  ( -0.6965510290629882695, 0.000000000000000000, -0.7175072570443395970 ) ) ;
#42721=VERTEX_POINT ( 'NONE', #16750 ) ;
#42722=PLANE ( 'NONE',  #3021 ) ;
#42724=DIRECTION ( 'NONE',  ( 0.9982437317643217956, 0.000000000000000000, -0.05924062789370748011 ) ) ;
#42726=EDGE_CURVE ( 'NONE', #33386, #18911, #13307, .T. ) ;
#42727=CIRCLE ( 'NONE', #9152, 125.0000000000000000 ) ;
#42730=ORIENTED_EDGE ( 'NONE', *, *, #5199, .F. ) ;
#42732=ORIENTED_EDGE ( 'NONE', *, *, #2741, .T. ) ;
#42733=ORIENTED_EDGE ( 'NONE', *, *, #38484, .T. ) ;
#42734=CARTESIAN_POINT ( 'NONE',  ( -26.53529504715431031, -189.7472609257535510, 123.0587999703026725 ) ) ;
#42737=ORIENTED_EDGE ( 'NONE', *, *, #42437, .T. ) ;
#42738=AXIS2_PLACEMENT_3D ( 'NONE', #24894, #12274, #40639 ) ;
#42739=LINE ( 'NONE', #27728, #45767 ) ;
#42740=DIRECTION ( 'NONE',  ( 0.000000000000000000, 1.000000000000000000, 0.000000000000000000 ) ) ;
#42741=ORIENTED_EDGE ( 'NONE', *, *, #33425, .T. ) ;
#42742=FACE_OUTER_BOUND ( 'NONE', #41316, .T. ) ;
#42743=VECTOR ( 'NONE', #4109, 1000.000000000000000 ) ;
#42744=EDGE_CURVE ( 'NONE', #39966, #44982, #29582, .T. ) ;
#42746=DIRECTION ( 'NONE',  ( -0.000000000000000000, 1.000000000000000000, -0.000000000000000000 ) ) ;
#42747=FACE_OUTER_BOUND ( 'NONE', #42934, .T. ) ;
#42748=VERTEX_POINT ( 'NONE', #37474 ) ;
#42749=EDGE_LOOP ( 'NONE', ( #3851, #23187, #37809, #41075 ) ) ;
#42750=ORIENTED_EDGE ( 'NONE', *, *, #1824, .T. ) ;
#42753=LINE ( 'NONE', #6756, #30199 ) ;
#42756=LINE ( 'NONE', #2551, #27210 ) ;
#42757=ORIENTED_EDGE ( 'NONE', *, *, #14238, .T. ) ;
#42758=VECTOR ( 'NONE', #22619, 1000.000000000000000 ) ;
#42759=DIRECTION ( 'NONE',  ( 0.000000000000000000, 0.000000000000000000, 1.000000000000000000 ) ) ;
#42760=ORIENTED_EDGE ( 'NONE', *, *, #27428, .F. ) ;
#42761=DIRECTION ( 'NONE',  ( 0.000000000000000000, 0.000000000000000000, -1.000000000000000000 ) ) ;
#42762=EDGE_LOOP ( 'NONE', ( #22706, #6631, #39734, #27105 ) ) ;
#42763=VERTEX_POINT ( 'NONE', #26150 ) ;
#42764=DIRECTION ( 'NONE',  ( -0.9960498426152165630, 0.000000000000000000, -0.08879589532293852283 ) ) ;
#42765=ADVANCED_FACE ( 'NONE', ( #13824 ), #10135, .T. ) ;
#42766=LINE ( 'NONE', #41977, #16583 ) ;
#42768=DIRECTION ( 'NONE',  ( 0.6068001458185890984, 0.000000000000000000, 0.7948544414133565938 ) ) ;
#42769=ORIENTED_EDGE ( 'NONE', *, *, #40345, .T. ) ;
#42772=ADVANCED_FACE ( 'NONE', ( #14091 ), #1733, .T. ) ;
#42774=DIRECTION ( 'NONE',  ( -0.000000000000000000, 1.000000000000000000, -0.000000000000000000 ) ) ;
#42775=DIRECTION ( 'NONE',  ( -0.000000000000000000, 1.000000000000000000, -0.000000000000000000 ) ) ;
#42776=CIRCLE ( 'NONE', #27653, 125.0000000000000000 ) ;
#42778=EDGE_LOOP ( 'NONE', ( #26460, #18324, #47816, #24231 ) ) ;
#42780=CARTESIAN_POINT ( 'NONE',  ( 57.12946453413545100, -175.3837268820161057, 66.87170886602000053 ) ) ;
#42784=DIRECTION ( 'NONE',  ( -0.9027978299657446470, 0.000000000000000000, 0.4300652022765183435 ) ) ;
#42787=EDGE_LOOP ( 'NONE', ( #20883, #15101, #44750, #18668 ) ) ;
#42788=DIRECTION ( 'NONE',  ( -0.5338233779648003940, 0.000000000000000000, 0.8455960035018199594 ) ) ;
#42789=ORIENTED_EDGE ( 'NONE', *, *, #32885, .T. ) ;
#42790=DIRECTION ( 'NONE',  ( -0.6749830015182196608, 0.000000000000000000, 0.7378332790417189146 ) ) ;
#42792=AXIS2_PLACEMENT_3D ( 'NONE', #40594, #13004, #17227 ) ;
#42794=DIRECTION ( 'NONE',  ( 0.000000000000000000, 0.000000000000000000, 1.000000000000000000 ) ) ;
#42795=DIRECTION ( 'NONE',  ( 0.3482016354343866471, 0.000000000000000000, 0.9374196611341253371 ) ) ;
#42797=DIRECTION ( 'NONE',  ( -0.8455960035018199594, 0.000000000000000000, -0.5338233779648003940 ) ) ;
#42798=EDGE_CURVE ( 'NONE', #22690, #41798, #10655, .T. ) ;
#42799=FACE_OUTER_BOUND ( 'NONE', #2780, .T. ) ;
#42800=ORIENTED_EDGE ( 'NONE', *, *, #20231, .F. ) ;
#42801=PLANE ( 'NONE',  #18114 ) ;
#42802=ORIENTED_EDGE ( 'NONE', *, *, #41373, .T. ) ;
#42803=DIRECTION ( 'NONE',  ( 0.000000000000000000, 0.000000000000000000, -1.000000000000000000 ) ) ;
#42804=CIRCLE ( 'NONE', #11739, 125.0000000000000000 ) ;
#42806=PLANE ( 'NONE',  #26757 ) ;
#42807=LINE ( 'NONE', #30460, #41842 ) ;
#42808=PLANE ( 'NONE',  #48399 ) ;
#42809=ORIENTED_EDGE ( 'NONE', *, *, #9534, .T. ) ;
#42810=LINE ( 'NONE', #10758, #48521 ) ;
#42811=DIRECTION ( 'NONE',  ( -0.000000000000000000, 1.000000000000000000, 0.000000000000000000 ) ) ;
#42812=ORIENTED_EDGE ( 'NONE', *, *, #34256, .F. ) ;
#42814=DIRECTION ( 'NONE',  ( -0.000000000000000000, 1.000000000000000000, -0.000000000000000000 ) ) ;
#42816=DIRECTION ( 'NONE',  ( -0.000000000000000000, 1.000000000000000000, -0.000000000000000000 ) ) ;
#42820=DIRECTION ( 'NONE',  ( -0.9266896074318370369, 0.000000000000000000, 0.3758275821142292306 ) ) ;
#42821=PLANE ( 'NONE',  #6517 ) ;
#42822=ORIENTED_EDGE ( 'NONE', *, *, #5737, .T. ) ;
#42823=ORIENTED_EDGE ( 'NONE', *, *, #12521, .T. ) ;
#42825=CARTESIAN_POINT ( 'NONE',  ( -173.4460699164830260, -193.5000000000000000, -2.874563619423202265 ) ) ;
#42826=EDGE_LOOP ( 'NONE', ( #49047, #42458, #45473, #12940 ) ) ;
#42828=CARTESIAN_POINT ( 'NONE',  ( -158.3442440847887269, -189.7472609257535510, -59.62093586438114556 ) ) ;
#42829=EDGE_LOOP ( 'NONE', ( #8404, #25757, #40418, #15496 ) ) ;
#42832=CARTESIAN_POINT ( 'NONE',  ( -9.070200226166599933, -193.5000000000000000, -117.5715283571804122 ) ) ;
#42834=DIRECTION ( 'NONE',  ( 0.000000000000000000, 1.000000000000000000, -0.000000000000000000 ) ) ;
#42837=DIRECTION ( 'NONE',  ( 0.000000000000000000, 0.000000000000000000, 1.000000000000000000 ) ) ;
#42839=DIRECTION ( 'NONE',  ( 0.000000000000000000, 1.000000000000000000, 0.000000000000000000 ) ) ;
#42840=ORIENTED_EDGE ( 'NONE', *, *, #13185, .T. ) ;
#42841=AXIS2_PLACEMENT_3D ( 'NONE', #50693, #43577, #27275 ) ;
#42842=DIRECTION ( 'NONE',  ( 0.7575112421616145841, 0.000000000000000000, 0.6528221181905280446 ) ) ;
#42843=CARTESIAN_POINT ( 'NONE',  ( -170.7635349987907318, -175.3837268820161057, -25.91377046305876775 ) ) ;
#42847=ORIENTED_EDGE ( 'NONE', *, *, #41210, .F. ) ;
#42848=EDGE_CURVE ( 'NONE', #28285, #43244, #37042, .T. ) ;
#42849=PLANE ( 'NONE',  #212 ) ;
#42852=DIRECTION ( 'NONE',  ( 0.000000000000000000, -1.000000000000000000, 0.000000000000000000 ) ) ;
#42853=PLANE ( 'NONE',  #34612 ) ;
#42854=VECTOR ( 'NONE', #108, 1000.000000000000227 ) ;
#42855=ORIENTED_EDGE ( 'NONE', *, *, #33659, .F. ) ;
#42856=EDGE_CURVE ( 'NONE', #14293, #150, #33787, .T. ) ;
#42857=LINE ( 'NONE', #34972, #10923 ) ;
#42858=EDGE_CURVE ( 'NONE', #6302, #265, #1818, .T. ) ;
#42859=VECTOR ( 'NONE', #26586, 1000.000000000000000 ) ;
#42860=VECTOR ( 'NONE', #44926, 1000.000000000000000 ) ;
#42861=DIRECTION ( 'NONE',  ( 0.000000000000000000, 1.000000000000000000, 0.000000000000000000 ) ) ;
#42862=ORIENTED_EDGE ( 'NONE', *, *, #14687, .F. ) ;
#42864=EDGE_CURVE ( 'NONE', #20728, #29853, #9374, .T. ) ;
#42867=CARTESIAN_POINT ( 'NONE',  ( -48.36085358058748795, -193.5000000000000000, 0.9929810960135245779 ) ) ;
#42869=ORIENTED_EDGE ( 'NONE', *, *, #15375, .F. ) ;
#42871=CARTESIAN_POINT ( 'NONE',  ( -84.82349129030161805, -189.7472609257535510, -119.5996955107802080 ) ) ;
#42872=DIRECTION ( 'NONE',  ( 0.000000000000000000, 1.000000000000000000, 0.000000000000000000 ) ) ;
#42874=ORIENTED_EDGE ( 'NONE', *, *, #43007, .T. ) ;
#42877=CARTESIAN_POINT ( 'NONE',  ( 69.66827051661184100, -193.5000000000000000, -40.81902153125260213 ) ) ;
#42879=DIRECTION ( 'NONE',  ( 0.000000000000000000, -1.000000000000000000, 0.000000000000000000 ) ) ;
#42884=ORIENTED_EDGE ( 'NONE', *, *, #14535, .T. ) ;
#42886=FACE_OUTER_BOUND ( 'NONE', #25095, .T. ) ;
#42888=ORIENTED_EDGE ( 'NONE', *, *, #44811, .T. ) ;
#42889=CARTESIAN_POINT ( 'NONE',  ( 54.18765407974404269, -193.5000000000000000, -69.53890913632879744 ) ) ;
#42890=AXIS2_PLACEMENT_3D ( 'NONE', #33146, #49196, #1869 ) ;
#42891=LINE ( 'NONE', #42374, #51720 ) ;
#42892=ORIENTED_EDGE ( 'NONE', *, *, #48821, .F. ) ;
#42894=DIRECTION ( 'NONE',  ( -0.000000000000000000, 1.000000000000000000, -0.000000000000000000 ) ) ;
#42895=CIRCLE ( 'NONE', #13534, 125.0000000000000000 ) ;
#42896=ORIENTED_EDGE ( 'NONE', *, *, #4076, .T. ) ;
#42897=DIRECTION ( 'NONE',  ( -0.000000000000000000, 1.000000000000000000, -0.000000000000000000 ) ) ;
#42899=DIRECTION ( 'NONE',  ( -0.9960498426152165630, 0.000000000000000000, -0.08879589532293852283 ) ) ;
#42900=CARTESIAN_POINT ( 'NONE',  ( -80.17897391495031911, -177.1207230881787780, 120.9136869416132498 ) ) ;
#42904=DIRECTION ( 'NONE',  ( 0.000000000000000000, 0.000000000000000000, -1.000000000000000000 ) ) ;
#42906=EDGE_CURVE ( 'NONE', #39429, #48052, #22218, .T. ) ;
#42908=CARTESIAN_POINT ( 'NONE',  ( 46.01898237923986557, -177.1207230881787780, -81.82363577055902226 ) ) ;
#42909=AXIS2_PLACEMENT_3D ( 'NONE', #35551, #30326, #47147 ) ;
#42910=DIRECTION ( 'NONE',  ( 0.000000000000000000, -0.000000000000000000, 1.000000000000000000 ) ) ;
#42912=CARTESIAN_POINT ( 'NONE',  ( 1.352451982137505171, -193.5000000000000000, 113.5465278748097120 ) ) ;
#42914=ORIENTED_EDGE ( 'NONE', *, *, #45786, .T. ) ;
#42917=EDGE_CURVE ( 'NONE', #45145, #12900, #34051, .T. ) ;
#42918=CARTESIAN_POINT ( 'NONE',  ( 75.67769207106684348, -193.5000000000000000, 14.49428645563876650 ) ) ;
#42919=ORIENTED_EDGE ( 'NONE', *, *, #44644, .T. ) ;
#42920=ORIENTED_EDGE ( 'NONE', *, *, #2955, .T. ) ;
#42922=DIRECTION ( 'NONE',  ( -0.000000000000000000, 1.000000000000000000, -0.000000000000000000 ) ) ;
#42923=ORIENTED_EDGE ( 'NONE', *, *, #51913, .F. ) ;
#42924=DIRECTION ( 'NONE',  ( 0.7378332790417333475, 0.000000000000000000, -0.6749830015182038956 ) ) ;
#42925=DIRECTION ( 'NONE',  ( 0.000000000000000000, 0.000000000000000000, 1.000000000000000000 ) ) ;
#42926=CIRCLE ( 'NONE', #17772, 125.0000000000000000 ) ;
#42927=EDGE_CURVE ( 'NONE', #40613, #10130, #37911, .T. ) ;
#42928=DIRECTION ( 'NONE',  ( -0.7765238627180349740, 0.000000000000000000, -0.6300878435817203194 ) ) ;
#42930=AXIS2_PLACEMENT_3D ( 'NONE', #24108, #36960, #949 ) ;
#42932=ORIENTED_EDGE ( 'NONE', *, *, #17286, .T. ) ;
#42933=CIRCLE ( 'NONE', #48840, 125.0000000000000000 ) ;
#42934=EDGE_LOOP ( 'NONE', ( #40471, #16893, #360, #1922 ) ) ;
#42935=DIRECTION ( 'NONE',  ( 0.000000000000000000, -0.000000000000000000, 1.000000000000000000 ) ) ;
#42937=DIRECTION ( 'NONE',  ( 0.6528221181905227155, 0.000000000000000000, -0.7575112421616191360 ) ) ;
#42938=CARTESIAN_POINT ( 'NONE',  ( -48.47912675150885065, -177.1207230881787780, 6.938893903907228378E-15 ) ) ;
#42945=ORIENTED_EDGE ( 'NONE', *, *, #37824, .T. ) ;
#42946=EDGE_LOOP ( 'NONE', ( #20935, #4231, #33999, #2463 ) ) ;
#42947=CARTESIAN_POINT ( 'NONE',  ( 17.15229921100054611, -177.1207230881787780, -106.3838142112212921 ) ) ;
#42948=VECTOR ( 'NONE', #2924, 1000.000000000000114 ) ;
#42950=DIRECTION ( 'NONE',  ( 0.000000000000000000, 0.000000000000000000, 1.000000000000000000 ) ) ;
#42951=DIRECTION ( 'NONE',  ( 0.000000000000000000, 0.000000000000000000, -1.000000000000000000 ) ) ;
#42952=PLANE ( 'NONE',  #37960 ) ;
#42953=DIRECTION ( 'NONE',  ( -0.000000000000000000, -1.000000000000000000, 0.000000000000000000 ) ) ;
#42954=ORIENTED_EDGE ( 'NONE', *, *, #11344, .T. ) ;
#42956=ADVANCED_FACE ( 'NONE', ( #23270 ), #3019, .T. ) ;
#42958=CARTESIAN_POINT ( 'NONE',  ( -149.9407190013152160, -175.3837268820161057, -73.01058346660458653 ) ) ;
#42959=CARTESIAN_POINT ( 'NONE',  ( -48.47912675150885065, -175.3837268820161057, 6.938893903907228378E-15 ) ) ;
#42960=ORIENTED_EDGE ( 'NONE', *, *, #5432, .F. ) ;
#42962=EDGE_CURVE ( 'NONE', #2344, #47414, #29499, .T. ) ;
#42963=DIRECTION ( 'NONE',  ( 0.000000000000000000, -1.000000000000000000, 0.000000000000000000 ) ) ;
#42966=DIRECTION ( 'NONE',  ( 0.000000000000000000, 0.000000000000000000, 1.000000000000000000 ) ) ;
#42967=ADVANCED_FACE ( 'NONE', ( #40044 ), #7743, .T. ) ;
#42970=EDGE_CURVE ( 'NONE', #38087, #1712, #23772, .T. ) ;
#42971=AXIS2_PLACEMENT_3D ( 'NONE', #2596, #25739, #18629 ) ;
#42972=CARTESIAN_POINT ( 'NONE',  ( -133.1483155860611021, -183.6283474603465606, -90.59430563621275212 ) ) ;
#42973=VERTEX_POINT ( 'NONE', #26930 ) ;
#42974=EDGE_CURVE ( 'NONE', #3147, #3202, #31657, .T. ) ;
#42975=DIRECTION ( 'NONE',  ( 0.000000000000000000, 0.000000000000000000, -1.000000000000000000 ) ) ;
#42977=ORIENTED_EDGE ( 'NONE', *, *, #51082, .F. ) ;
#42978=VERTEX_POINT ( 'NONE', #43219 ) ;
#42979=DIRECTION ( 'NONE',  ( 0.3758275821142292861, 0.000000000000000000, 0.9266896074318371479 ) ) ;
#42980=EDGE_CURVE ( 'NONE', #2935, #28959, #3499, .T. ) ;
#42982=AXIS2_PLACEMENT_3D ( 'NONE', #46303, #25280, #45521 ) ;
#42983=EDGE_CURVE ( 'NONE', #28863, #44261, #11414, .T. ) ;
#42984=DIRECTION ( 'NONE',  ( 0.9027978299657416494, 0.000000000000000000, 0.4300652022765245608 ) ) ;
#42985=AXIS2_PLACEMENT_3D ( 'NONE', #32564, #5504, #24949 ) ;
#42989=DIRECTION ( 'NONE',  ( -0.4031234292879792847, 0.000000000000000000, 0.9151456172430153524 ) ) ;
#42993=EDGE_CURVE ( 'NONE', #41579, #42167, #11683, .T. ) ;
#42994=LINE ( 'NONE', #39554, #42012 ) ;
#42995=PLANE ( 'NONE',  #3025 ) ;
#42996=EDGE_LOOP ( 'NONE', ( #40315, #30430, #45670, #45287 ) ) ;
#42997=EDGE_LOOP ( 'NONE', ( #26810, #31956, #39040, #18524 ) ) ;
#42998=EDGE_CURVE ( 'NONE', #10986, #48832, #47186, .T. ) ;
#43000=LINE ( 'NONE', #30639, #21715 ) ;
#43001=FACE_OUTER_BOUND ( 'NONE', #26713, .T. ) ;
#43002=FACE_OUTER_BOUND ( 'NONE', #25520, .T. ) ;
#43004=CARTESIAN_POINT ( 'NONE',  ( -48.59739992243020623, -193.5000000000000000, -0.9929810960135115883 ) ) ;
#43005=VECTOR ( 'NONE', #46721, 1000.000000000000114 ) ;
#43006=VERTEX_POINT ( 'NONE', #46934 ) ;
#43007=EDGE_CURVE ( 'NONE', #37393, #24991, #47430, .T. ) ;
#43010=VERTEX_POINT ( 'NONE', #7495 ) ;
#43011=DIRECTION ( 'NONE',  ( 0.000000000000000000, -1.000000000000000000, 0.000000000000000000 ) ) ;
#43012=ORIENTED_EDGE ( 'NONE', *, *, #28548, .T. ) ;
#43013=ORIENTED_EDGE ( 'NONE', *, *, #30832, .F. ) ;
#43015=DIRECTION ( 'NONE',  ( -0.000000000000000000, 0.000000000000000000, -1.000000000000000000 ) ) ;
#43016=CARTESIAN_POINT ( 'NONE',  ( 23.33927677392131628, -177.1207230881787780, -102.3089288139528747 ) ) ;
#43017=LINE ( 'NONE', #7026, #26770 ) ;
#43018=EDGE_LOOP ( 'NONE', ( #31681, #11381, #17274, #16232 ) ) ;
#43019=DIRECTION ( 'NONE',  ( 0.000000000000000000, -1.000000000000000000, 0.000000000000000000 ) ) ;
#43021=CIRCLE ( 'NONE', #43058, 125.0000000000000000 ) ;
#43023=EDGE_LOOP ( 'NONE', ( #44296, #24270, #24685, #10057 ) ) ;
#43024=CARTESIAN_POINT ( 'NONE',  ( 65.79610465833508215, -183.6283474603465606, -50.65739320401927870 ) ) ;
#43025=CIRCLE ( 'NONE', #20360, 125.0000000000000000 ) ;
#43026=DIRECTION ( 'NONE',  ( -0.4566292373937200777, 0.000000000000000000, 0.8896570909947436601 ) ) ;
#43029=CARTESIAN_POINT ( 'NONE',  ( -128.7986236165182277, -193.5000000000000000, 94.47107458416954273 ) ) ;
#43031=CARTESIAN_POINT ( 'NONE',  ( 43.86477233319988756, -175.3837268820161057, -84.24728067915975771 ) ) ;
#43032=FACE_OUTER_BOUND ( 'NONE', #8251, .T. ) ;
#43033=EDGE_CURVE ( 'NONE', #13545, #47870, #15903, .T. ) ;
#43034=ADVANCED_FACE ( 'NONE', ( #23516 ), #39529, .F. ) ;
#43035=DIRECTION ( 'NONE',  ( 0.000000000000000000, 0.000000000000000000, 1.000000000000000000 ) ) ;
#43036=CARTESIAN_POINT ( 'NONE',  ( -0.3054481938615516423, -177.1207230881787780, 115.3442529744090450 ) ) ;
#43038=ORIENTED_EDGE ( 'NONE', *, *, #27828, .T. ) ;
#43039=DIRECTION ( 'NONE',  ( 0.000000000000000000, -1.000000000000000000, 0.000000000000000000 ) ) ;
#43041=EDGE_CURVE ( 'NONE', #30065, #40321, #35585, .T. ) ;
#43042=EDGE_CURVE ( 'NONE', #21936, #44616, #2679, .T. ) ;
#43043=DIRECTION ( 'NONE',  ( 0.2920567706369628924, 0.000000000000000000, 0.9564009842765264224 ) ) ;
#43045=DIRECTION ( 'NONE',  ( -0.000000000000000000, 1.000000000000000000, -0.000000000000000000 ) ) ;
#43046=VECTOR ( 'NONE', #24350, 1000.000000000000000 ) ;
#43047=PLANE ( 'NONE',  #44592 ) ;
#43049=CARTESIAN_POINT ( 'NONE',  ( 76.43863189440992301, -193.5000000000000000, -4.533605064403313456 ) ) ;
#43050=EDGE_LOOP ( 'NONE', ( #15327, #34291, #13681, #2738 ) ) ;
#43051=AXIS2_PLACEMENT_3D ( 'NONE', #25867, #5388, #21404 ) ;
#43053=EDGE_CURVE ( 'NONE', #19112, #12481, #10913, .T. ) ;
#43054=FACE_BOUND ( 'NONE', #16535, .T. ) ;
#43055=DIRECTION ( 'NONE',  ( 0.000000000000000000, -0.000000000000000000, 1.000000000000000000 ) ) ;
#43056=CARTESIAN_POINT ( 'NONE',  ( -108.6269575285487434, -177.1207230881787780, -108.4360005853207269 ) ) ;
#43057=VECTOR ( 'NONE', #7375, 1000.000000000000000 ) ;
#43058=AXIS2_PLACEMENT_3D ( 'NONE', #13132, #29671, #21280 ) ;
#43059=VERTEX_POINT ( 'NONE', #4317 ) ;
#43060=EDGE_CURVE ( 'NONE', #21927, #21227, #37408, .T. ) ;
#43061=ORIENTED_EDGE ( 'NONE', *, *, #19778, .F. ) ;
#43062=CARTESIAN_POINT ( 'NONE',  ( -170.0502155641509034, -183.6283474603465606, -29.07697310430886262 ) ) ;
#43064=EDGE_LOOP ( 'NONE', ( #4520, #43710, #2687, #20590 ) ) ;
#43068=CARTESIAN_POINT ( 'NONE',  ( -142.9772358822569913, -177.1207230881787780, 81.82363577055970438 ) ) ;
#43070=DIRECTION ( 'NONE',  ( 0.7765238627180437447, 0.000000000000000000, -0.6300878435817094392 ) ) ;
#43072=ORIENTED_EDGE ( 'NONE', *, *, #50844, .F. ) ;
#43073=DIRECTION ( 'NONE',  ( 0.000000000000000000, -1.000000000000000000, 0.000000000000000000 ) ) ;
#43074=ORIENTED_EDGE ( 'NONE', *, *, #45099, .F. ) ;
#43075=CARTESIAN_POINT ( 'NONE',  ( -48.47912675150885065, -189.7472609257535510, 6.938893903907228378E-15 ) ) ;
#43077=ORIENTED_EDGE ( 'NONE', *, *, #2955, .F. ) ;
#43080=PLANE ( 'NONE',  #6503 ) ;
#43081=CARTESIAN_POINT ( 'NONE',  ( -116.2964108826154330, -193.5000000000000000, -105.0038855142073260 ) ) ;
#43082=VERTEX_POINT ( 'NONE', #28222 ) ;
#43084=DIRECTION ( 'NONE',  ( -0.2920567706369833760, 0.000000000000000000, 0.9564009842765202052 ) ) ;
#43085=EDGE_LOOP ( 'NONE', ( #21399, #17881, #38188, #33218 ) ) ;
#43088=VERTEX_POINT ( 'NONE', #8769 ) ;
#43089=PLANE ( 'NONE',  #23833 ) ;
#43093=ORIENTED_EDGE ( 'NONE', *, *, #10421, .F. ) ;
#43098=PLANE ( 'NONE',  #7996 ) ;
#43099=CARTESIAN_POINT ( 'NONE',  ( 75.10200014432449223, -189.7472609257535510, 10.18383939837613639 ) ) ;
#43100=ORIENTED_EDGE ( 'NONE', *, *, #51103, .F. ) ;
#43102=DIRECTION ( 'NONE',  ( -0.9785564922995017012, 0.000000000000000000, -0.2059786187411094538 ) ) ;
#43103=DIRECTION ( 'NONE',  ( 0.000000000000000000, 0.000000000000000000, 1.000000000000000000 ) ) ;
#43104=LINE ( 'NONE', #1684, #15706 ) ;
#43106=DIRECTION ( 'NONE',  ( 0.000000000000000000, 0.000000000000000000, -1.000000000000000000 ) ) ;
#43107=ORIENTED_EDGE ( 'NONE', *, *, #13446, .F. ) ;
#43108=FACE_OUTER_BOUND ( 'NONE', #31832, .T. ) ;
#43109=DIRECTION ( 'NONE',  ( 0.000000000000000000, -1.000000000000000000, 0.000000000000000000 ) ) ;
#43110=FACE_OUTER_BOUND ( 'NONE', #28474, .T. ) ;
#43111=EDGE_CURVE ( 'NONE', #13947, #42649, #33632, .T. ) ;
#43113=PLANE ( 'NONE',  #37126 ) ;
#43114=VECTOR ( 'NONE', #24360, 1000.000000000000000 ) ;
#43116=DIRECTION ( 'NONE',  ( 0.000000000000000000, -0.000000000000000000, 1.000000000000000000 ) ) ;
#43118=ADVANCED_FACE ( 'NONE', ( #21121 ), #24808, .F. ) ;
#43119=EDGE_LOOP ( 'NONE', ( #48055, #20312, #17765, #16622 ) ) ;
#43121=ORIENTED_EDGE ( 'NONE', *, *, #36139, .F. ) ;
#43122=LINE ( 'NONE', #34715, #16644 ) ;
#43123=EDGE_CURVE ( 'NONE', #18433, #43853, #44550, .T. ) ;
#43124=DIRECTION ( 'NONE',  ( -0.000000000000000000, 1.000000000000000000, -0.000000000000000000 ) ) ;
#43125=CIRCLE ( 'NONE', #23847, 125.0000000000000000 ) ;
#43129=LINE ( 'NONE', #15039, #17425 ) ;
#43130=CARTESIAN_POINT ( 'NONE',  ( 75.60865171534658202, -193.5000000000000000, -15.07392567185468124 ) ) ;
#43131=ORIENTED_EDGE ( 'NONE', *, *, #323, .F. ) ;
#43132=FACE_OUTER_BOUND ( 'NONE', #7432, .T. ) ;
#43133=ORIENTED_EDGE ( 'NONE', *, *, #21503, .F. ) ;
#43138=DIRECTION ( 'NONE',  ( 0.000000000000000000, 0.000000000000000000, 1.000000000000000000 ) ) ;
#43139=PLANE ( 'NONE',  #39915 ) ;
#43141=ADVANCED_FACE ( 'NONE', ( #40558 ), #5366, .T. ) ;
#43142=CYLINDRICAL_SURFACE ( 'NONE', #11379, 124.9999999999999858 ) ;
#43143=ORIENTED_EDGE ( 'NONE', *, *, #43212, .T. ) ;
#43145=FACE_OUTER_BOUND ( 'NONE', #11989, .T. ) ;
#43146=VERTEX_POINT ( 'NONE', #48215 ) ;
#43149=DIRECTION ( 'NONE',  ( -0.000000000000000000, 1.000000000000000000, -0.000000000000000000 ) ) ;
#43150=AXIS2_PLACEMENT_3D ( 'NONE', #25455, #45189, #21776 ) ;
#43151=ORIENTED_EDGE ( 'NONE', *, *, #4059, .F. ) ;
#43152=ADVANCED_FACE ( 'NONE', ( #642 ), #887, .T. ) ;
#43154=CARTESIAN_POINT ( 'NONE',  ( 74.48795740376235130, -183.6283474603465606, -15.97798378892165871 ) ) ;
#43156=VERTEX_POINT ( 'NONE', #8259 ) ;
#43159=EDGE_CURVE ( 'NONE', #16186, #42609, #5111, .T. ) ;
#43160=LINE ( 'NONE', #3231, #30687 ) ;
#43163=DIRECTION ( 'NONE',  ( -0.2059786187411094538, 0.000000000000000000, 0.9785564922995017012 ) ) ;
#43164=LINE ( 'NONE', #31861, #44056 ) ;
#43165=CARTESIAN_POINT ( 'NONE',  ( -28.74596282265200387, -183.6283474603465606, 123.4325817657431372 ) ) ;
#43167=CARTESIAN_POINT ( 'NONE',  ( -116.2964108826154188, -177.1207230881787780, -105.0038855142073402 ) ) ;
#43169=DIRECTION ( 'NONE',  ( -0.000000000000000000, 1.000000000000000000, -0.000000000000000000 ) ) ;
#43170=EDGE_CURVE ( 'NONE', #4741, #41311, #33206, .T. ) ;
#43172=CARTESIAN_POINT ( 'NONE',  ( 41.40822382563629134, -183.6283474603465606, 85.41934182508082074 ) ) ;
#43173=ORIENTED_EDGE ( 'NONE', *, *, #32401, .T. ) ;
#43174=ORIENTED_EDGE ( 'NONE', *, *, #49685, .F. ) ;
#43175=LINE ( 'NONE', #26375, #23247 ) ;
#43176=DIRECTION ( 'NONE',  ( 0.000000000000000000, 0.000000000000000000, 1.000000000000000000 ) ) ;
#43177=EDGE_LOOP ( 'NONE', ( #37072, #5262, #4363, #18401 ) ) ;
#43178=ORIENTED_EDGE ( 'NONE', *, *, #51375, .T. ) ;
#43179=CARTESIAN_POINT ( 'NONE',  ( 75.60865171534658202, -177.1207230881787780, -15.07392567185468124 ) ) ;
#43180=ORIENTED_EDGE ( 'NONE', *, *, #17373, .F. ) ;
#43181=CARTESIAN_POINT ( 'NONE',  ( -105.2524431885210845, -175.3837268820161057, 110.2396968984195382 ) ) ;
#43183=AXIS2_PLACEMENT_3D ( 'NONE', #5025, #25245, #32856 ) ;
#43184=AXIS2_PLACEMENT_3D ( 'NONE', #21260, #49387, #4983 ) ;
#43185=DIRECTION ( 'NONE',  ( 0.9027978299657387629, 0.000000000000000000, 0.4300652022765304450 ) ) ;
#43187=ORIENTED_EDGE ( 'NONE', *, *, #30137, .T. ) ;
#43188=VERTEX_POINT ( 'NONE', #45060 ) ;
#43189=AXIS2_PLACEMENT_3D ( 'NONE', #45577, #9314, #40829 ) ;
#43190=ORIENTED_EDGE ( 'NONE', *, *, #50449, .F. ) ;
#43191=CARTESIAN_POINT ( 'NONE',  ( -48.47912675150885065, -175.3837268820161057, 6.938893903907228378E-15 ) ) ;
#43192=DIRECTION ( 'NONE',  ( 0.5586467658036476935, 0.000000000000000000, 0.8294056854502049880 ) ) ;
#43194=AXIS2_PLACEMENT_3D ( 'NONE', #10759, #42811, #10490 ) ;
#43195=DIRECTION ( 'NONE',  ( -0.000000000000000000, 1.000000000000000000, -0.000000000000000000 ) ) ;
#43197=VERTEX_POINT ( 'NONE', #9050 ) ;
#43200=DIRECTION ( 'NONE',  ( 0.000000000000000000, 0.000000000000000000, 1.000000000000000000 ) ) ;
#43201=CARTESIAN_POINT ( 'NONE',  ( -4.176930889631405464, -189.7472609257535510, 116.8859077982279615 ) ) ;
#43202=ORIENTED_EDGE ( 'NONE', *, *, #30844, .F. ) ;
#43203=VERTEX_POINT ( 'NONE', #41096 ) ;
#43207=EDGE_LOOP ( 'NONE', ( #39660, #40805, #24654, #22727 ) ) ;
#43208=LINE ( 'NONE', #23761, #8086 ) ;
#43210=CARTESIAN_POINT ( 'NONE',  ( -48.41988612361514299, -177.1207230881787780, -0.9982437317643144681 ) ) ;
#43211=ORIENTED_EDGE ( 'NONE', *, *, #7616, .F. ) ;
#43212=EDGE_CURVE ( 'NONE', #47366, #8754, #37145, .T. ) ;
#43215=ORIENTED_EDGE ( 'NONE', *, *, #5529, .F. ) ;
#43216=DIRECTION ( 'NONE',  ( 0.000000000000000000, 1.000000000000000000, -0.000000000000000000 ) ) ;
#43217=EDGE_CURVE ( 'NONE', #650, #50927, #44670, .T. ) ;
#43219=CARTESIAN_POINT ( 'NONE',  ( 45.36094686508022988, -177.1207230881787780, -82.57748230379236531 ) ) ;
#43220=ORIENTED_EDGE ( 'NONE', *, *, #12168, .T. ) ;
#43221=CIRCLE ( 'NONE', #23086, 124.9999999999999858 ) ;
#43223=DIRECTION ( 'NONE',  ( 0.000000000000000000, 0.000000000000000000, 1.000000000000000000 ) ) ;
#43224=CARTESIAN_POINT ( 'NONE',  ( -48.47912675150885065, -175.3837268820161057, 6.938893903907228378E-15 ) ) ;
#43225=CARTESIAN_POINT ( 'NONE',  ( 64.29733702426837283, -175.3837268820161057, 53.91167979418564471 ) ) ;
#43226=DIRECTION ( 'NONE',  ( -0.000000000000000000, 1.000000000000000000, -0.000000000000000000 ) ) ;
#43228=PLANE ( 'NONE',  #42071 ) ;
#43229=ORIENTED_EDGE ( 'NONE', *, *, #23287, .T. ) ;
#43233=ORIENTED_EDGE ( 'NONE', *, *, #26186, .F. ) ;
#43234=AXIS2_PLACEMENT_3D ( 'NONE', #31612, #47665, #7459 ) ;
#43237=VECTOR ( 'NONE', #27, 1000.000000000000000 ) ;
#43241=ORIENTED_EDGE ( 'NONE', *, *, #2546, .T. ) ;
#43242=LINE ( 'NONE', #19850, #51143 ) ;
#43243=CARTESIAN_POINT ( 'NONE',  ( -142.2007120195389405, -177.1207230881787780, 81.19354792697799894 ) ) ;
#43244=VERTEX_POINT ( 'NONE', #40301 ) ;
#43246=CARTESIAN_POINT ( 'NONE',  ( -59.28786813212838069, -193.5000000000000000, 124.5318076226587323 ) ) ;
#43247=DIRECTION ( 'NONE',  ( 0.000000000000000000, -0.000000000000000000, 1.000000000000000000 ) ) ;
#43249=VERTEX_POINT ( 'NONE', #6406 ) ;
#43256=CARTESIAN_POINT ( 'NONE',  ( -48.77118352214583297, -177.1207230881787780, 0.9564009842765270886 ) ) ;
#43262=EDGE_CURVE ( 'NONE', #40095, #23489, #49590, .T. ) ;
#43263=LINE ( 'NONE', #23554, #17368 ) ;
#43265=CARTESIAN_POINT ( 'NONE',  ( -105.7090724259148118, -175.3837268820161057, 111.1293539894142839 ) ) ;
#43266=EDGE_LOOP ( 'NONE', ( #48641, #50064, #36850, #17991 ) ) ;
#43268=EDGE_CURVE ( 'NONE', #42496, #36635, #30049, .T. ) ;
#43269=LINE ( 'NONE', #39059, #13217 ) ;
#43270=AXIS2_PLACEMENT_3D ( 'NONE', #38287, #6513, #7279 ) ;
#43273=VECTOR ( 'NONE', #5433, 1000.000000000000000 ) ;
#43275=DIRECTION ( 'NONE',  ( -0.7765238627180393038, 0.000000000000000000, -0.6300878435817147682 ) ) ;
#43276=ORIENTED_EDGE ( 'NONE', *, *, #31324, .F. ) ;
#43277=EDGE_CURVE ( 'NONE', #7756, #51755, #17709, .T. ) ;
#43279=AXIS2_PLACEMENT_3D ( 'NONE', #9160, #36751, #40408 ) ;
#43280=ORIENTED_EDGE ( 'NONE', *, *, #12505, .F. ) ;
#43282=AXIS2_PLACEMENT_3D ( 'NONE', #29623, #45672, #9662 ) ;
#43283=EDGE_CURVE ( 'NONE', #32626, #30858, #6664, .T. ) ;
#43287=EDGE_CURVE ( 'NONE', #29932, #13886, #24399, .T. ) ;
#43290=LINE ( 'NONE', #44064, #2936 ) ;
#43291=ADVANCED_FACE ( 'NONE', ( #33983 ), #10081, .F. ) ;
#43292=FACE_OUTER_BOUND ( 'NONE', #39802, .T. ) ;
#43293=DIRECTION ( 'NONE',  ( -0.000000000000000000, 1.000000000000000000, -0.000000000000000000 ) ) ;
#43294=ORIENTED_EDGE ( 'NONE', *, *, #24366, .T. ) ;
#43295=DIRECTION ( 'NONE',  ( -0.000000000000000000, 1.000000000000000000, -0.000000000000000000 ) ) ;
#43296=CARTESIAN_POINT ( 'NONE',  ( -109.9568094315246185, -183.6283474603465606, -108.8370090194290754 ) ) ;
#43297=FACE_BOUND ( 'NONE', #46020, .T. ) ;
#43298=ORIENTED_EDGE ( 'NONE', *, *, #23854, .T. ) ;
#43302=CIRCLE ( 'NONE', #1364, 125.0000000000000000 ) ;
#43303=LINE ( 'NONE', #22821, #48808 ) ;
#43304=ORIENTED_EDGE ( 'NONE', *, *, #6311, .T. ) ;
#43306=ORIENTED_EDGE ( 'NONE', *, *, #11834, .F. ) ;
#43309=FACE_BOUND ( 'NONE', #44554, .T. ) ;
#43312=VERTEX_POINT ( 'NONE', #26097 ) ;
#43314=AXIS2_PLACEMENT_3D ( 'NONE', #42825, #49948, #33651 ) ;
#43317=ORIENTED_EDGE ( 'NONE', *, *, #6639, .F. ) ;
#43318=AXIS2_PLACEMENT_3D ( 'NONE', #10117, #26134, #42164 ) ;
#43319=EDGE_CURVE ( 'NONE', #25483, #23608, #14028, .T. ) ;
#43321=VERTEX_POINT ( 'NONE', #42387 ) ;
#43322=DIRECTION ( 'NONE',  ( 0.3202698538628416247, 0.000000000000000000, -0.9473263538541900619 ) ) ;
#43325=EDGE_CURVE ( 'NONE', #46128, #2222, #30301, .T. ) ;
#43326=ADVANCED_FACE ( 'NONE', ( #33732 ), #9822, .T. ) ;
#43327=ADVANCED_FACE ( 'NONE', ( #51571 ), #10854, .F. ) ;
#43332=CARTESIAN_POINT ( 'NONE',  ( -48.47912675150885065, -175.3837268820161057, 6.938893903907228378E-15 ) ) ;
#43334=AXIS2_PLACEMENT_3D ( 'NONE', #51712, #44070, #39081 ) ;
#43337=EDGE_CURVE ( 'NONE', #31562, #22071, #29539, .T. ) ;
#43338=CARTESIAN_POINT ( 'NONE',  ( -77.67449977936063021, -193.5000000000000000, -121.5427093402339267 ) ) ;
#43340=FACE_OUTER_BOUND ( 'NONE', #23491, .T. ) ;
#43341=ORIENTED_EDGE ( 'NONE', *, *, #51415, .T. ) ;
#43342=AXIS2_PLACEMENT_3D ( 'NONE', #36833, #29450, #10023 ) ;
#43343=CARTESIAN_POINT ( 'NONE',  ( 76.37123734610607073, -193.5000000000000000, 6.114457023561876703 ) ) ;
#43344=ORIENTED_EDGE ( 'NONE', *, *, #15048, .T. ) ;
#43345=EDGE_CURVE ( 'NONE', #34863, #12900, #36249, .T. ) ;
#43346=DIRECTION ( 'NONE',  ( -0.000000000000000000, 1.000000000000000000, -0.000000000000000000 ) ) ;
#43347=LINE ( 'NONE', #39636, #30847 ) ;
#43349=ADVANCED_FACE ( 'NONE', ( #39471 ), #47894, .T. ) ;
#43350=CARTESIAN_POINT ( 'NONE',  ( -49.47517659412407198, -177.1207230881787780, 0.08879589532293177823 ) ) ;
#43351=ORIENTED_EDGE ( 'NONE', *, *, #32478, .F. ) ;
#43353=VECTOR ( 'NONE', #50536, 1000.000000000000000 ) ;
#43356=VERTEX_POINT ( 'NONE', #42900 ) ;
#43357=AXIS2_PLACEMENT_3D ( 'NONE', #21318, #37857, #29198 ) ;
#43360=PLANE ( 'NONE',  #29957 ) ;
#43362=CARTESIAN_POINT ( 'NONE',  ( 76.37123734610607073, -177.1207230881787780, 6.114457023561876703 ) ) ;
#43364=VERTEX_POINT ( 'NONE', #11098 ) ;
#43367=PLANE ( 'NONE',  #24618 ) ;
#43369=EDGE_CURVE ( 'NONE', #40095, #37488, #26867, .T. ) ;
#43370=CIRCLE ( 'NONE', #22393, 125.0000000000000000 ) ;
#43371=DIRECTION ( 'NONE',  ( 0.000000000000000000, -1.000000000000000000, -0.000000000000000000 ) ) ;
#43372=EDGE_LOOP ( 'NONE', ( #29657, #28646, #10268, #12816 ) ) ;
#43373=CARTESIAN_POINT ( 'NONE',  ( -98.71382891444399377, -175.3837268820161057, -114.4616734920523555 ) ) ;
#43376=CYLINDRICAL_SURFACE ( 'NONE', #11515, 124.9999999999999858 ) ;
#43379=ORIENTED_EDGE ( 'NONE', *, *, #25165, .F. ) ;
#43380=EDGE_CURVE ( 'NONE', #37325, #27840, #17806, .T. ) ;
#43381=AXIS2_PLACEMENT_3D ( 'NONE', #49531, #45579, #9564 ) ;
#43382=CARTESIAN_POINT ( 'NONE',  ( -63.31390705753092618, -175.3837268820161057, 123.1094209424469312 ) ) ;
#43383=CIRCLE ( 'NONE', #6444, 125.0000000000000000 ) ;
#43386=VECTOR ( 'NONE', #39567, 1000.000000000000114 ) ;
#43389=ORIENTED_EDGE ( 'NONE', *, *, #39058, .T. ) ;
#43390=AXIS2_PLACEMENT_3D ( 'NONE', #16188, #28261, #4104 ) ;
#43391=EDGE_LOOP ( 'NONE', ( #7385, #18079, #13344, #10015 ) ) ;
#43392=AXIS2_PLACEMENT_3D ( 'NONE', #44124, #24417, #11797 ) ;
#43393=ORIENTED_EDGE ( 'NONE', *, *, #34387, .F. ) ;
#43394=CARTESIAN_POINT ( 'NONE',  ( -151.4272465800706016, -177.1207230881787780, 70.89911581792887318 ) ) ;
#43396=VECTOR ( 'NONE', #40498, 1000.000000000000227 ) ;
#43397=ADVANCED_FACE ( 'NONE', ( #3473 ), #22941, .T. ) ;
#43403=LINE ( 'NONE', #6367, #45311 ) ;
#43405=CARTESIAN_POINT ( 'NONE',  ( -147.2362428880188077, -177.1207230881787780, -74.98773087994455011 ) ) ;
#43407=ORIENTED_EDGE ( 'NONE', *, *, #10125, .F. ) ;
#43408=DIRECTION ( 'NONE',  ( -0.000000000000000000, 1.000000000000000000, 0.000000000000000000 ) ) ;
#43409=ORIENTED_EDGE ( 'NONE', *, *, #39488, .F. ) ;
#43410=CYLINDRICAL_SURFACE ( 'NONE', #2901, 125.0000000000000000 ) ;
#43411=ORIENTED_EDGE ( 'NONE', *, *, #24243, .T. ) ;
#43412=DIRECTION ( 'NONE',  ( 0.000000000000000000, -1.000000000000000000, 0.000000000000000000 ) ) ;
#43413=PLANE ( 'NONE',  #16241 ) ;
#43414=FACE_OUTER_BOUND ( 'NONE', #43064, .T. ) ;
#43416=ORIENTED_EDGE ( 'NONE', *, *, #33444, .T. ) ;
#43420=LINE ( 'NONE', #18726, #2973 ) ;
#43421=AXIS2_PLACEMENT_3D ( 'NONE', #5575, #14234, #30253 ) ;
#43422=ORIENTED_EDGE ( 'NONE', *, *, #45609, .T. ) ;
#43423=EDGE_CURVE ( 'NONE', #4180, #2804, #35790, .T. ) ;
#43424=CARTESIAN_POINT ( 'NONE',  ( -50.89116676070551648, -183.6283474603465606, 124.9767260852757147 ) ) ;
#43426=DIRECTION ( 'NONE',  ( -0.000000000000000000, 1.000000000000000000, -0.000000000000000000 ) ) ;
#43427=ORIENTED_EDGE ( 'NONE', *, *, #42998, .T. ) ;
#43428=CARTESIAN_POINT ( 'NONE',  ( -170.9948556092908234, -193.5000000000000000, 19.12855698118475090 ) ) ;
#43430=EDGE_CURVE ( 'NONE', #18675, #32483, #36173, .T. ) ;
#43433=ORIENTED_EDGE ( 'NONE', *, *, #41059, .F. ) ;
#43434=VECTOR ( 'NONE', #19534, 1000.000000000000227 ) ;
#43435=CARTESIAN_POINT ( 'NONE',  ( -88.78924379339709105, -183.6283474603465606, -118.3219948448692662 ) ) ;
#43436=AXIS2_PLACEMENT_3D ( 'NONE', #50001, #30275, #2153 ) ;
#43440=DIRECTION ( 'NONE',  ( -0.000000000000000000, 1.000000000000000000, -0.000000000000000000 ) ) ;
#43441=DIRECTION ( 'NONE',  ( -0.000000000000000000, 1.000000000000000000, -0.000000000000000000 ) ) ;
#43445=PLANE ( 'NONE',  #18636 ) ;
#43447=CARTESIAN_POINT ( 'NONE',  ( -136.5246168469702468, -193.5000000000000000, 87.31661597576146505 ) ) ;
#43450=CARTESIAN_POINT ( 'NONE',  ( 67.87295084395105960, -193.5000000000000000, 42.87565520599286373 ) ) ;
#43451=DIRECTION ( 'NONE',  ( 0.000000000000000000, -0.000000000000000000, 1.000000000000000000 ) ) ;
#43452=EDGE_LOOP ( 'NONE', ( #10994, #31908, #32012, #44265 ) ) ;
#43453=CIRCLE ( 'NONE', #24139, 9.999999999999994671 ) ;
#43454=AXIS2_PLACEMENT_3D ( 'NONE', #6314, #18407, #14465 ) ;
#43456=DIRECTION ( 'NONE',  ( -0.3202698538628350744, 0.000000000000000000, -0.9473263538541923934 ) ) ;
#43457=VERTEX_POINT ( 'NONE', #47644 ) ;
#43458=CARTESIAN_POINT ( 'NONE',  ( -166.2107720749848738, -193.5000000000000000, -38.92640747825594616 ) ) ;
#43459=CARTESIAN_POINT ( 'NONE',  ( -71.22983192549011733, -189.7472609257535510, -121.8950816227732759 ) ) ;
#43461=EDGE_CURVE ( 'NONE', #17455, #17248, #23962, .T. ) ;
#43462=CARTESIAN_POINT ( 'NONE',  ( -49.13194886969936448, -193.5000000000000000, -0.7575112421616214675 ) ) ;
#43465=VERTEX_POINT ( 'NONE', #11628 ) ;
#43467=DIRECTION ( 'NONE',  ( 0.000000000000000000, 0.000000000000000000, 1.000000000000000000 ) ) ;
#43469=AXIS2_PLACEMENT_3D ( 'NONE', #32967, #49015, #24569 ) ;
#43470=DIRECTION ( 'NONE',  ( -0.000000000000000000, 1.000000000000000000, -0.000000000000000000 ) ) ;
#43472=DIRECTION ( 'NONE',  ( 0.9785564922995046988, 0.000000000000000000, -0.2059786187410953262 ) ) ;
#43473=ORIENTED_EDGE ( 'NONE', *, *, #30054, .F. ) ;
#43476=AXIS2_PLACEMENT_3D ( 'NONE', #49446, #20789, #8432 ) ;
#43477=ORIENTED_EDGE ( 'NONE', *, *, #641, .F. ) ;
#43478=VERTEX_POINT ( 'NONE', #23207 ) ;
#43480=DIRECTION ( 'NONE',  ( -0.000000000000000000, 1.000000000000000000, -0.000000000000000000 ) ) ;
#43486=CARTESIAN_POINT ( 'NONE',  ( -70.75782287548091176, -175.3837268820161057, 122.9986166548864759 ) ) ;
#43487=ORIENTED_EDGE ( 'NONE', *, *, #2896, .F. ) ;
#43488=DIRECTION ( 'NONE',  ( 0.9960498426152177842, 0.000000000000000000, -0.08879589532292482545 ) ) ;
#43489=ORIENTED_EDGE ( 'NONE', *, *, #1518, .T. ) ;
#43490=DIRECTION ( 'NONE',  ( 0.000000000000000000, 0.000000000000000000, 1.000000000000000000 ) ) ;
#43491=CIRCLE ( 'NONE', #19993, 125.0000000000000000 ) ;
#43493=DIRECTION ( 'NONE',  ( -0.000000000000000000, 1.000000000000000000, -0.000000000000000000 ) ) ;
#43494=EDGE_LOOP ( 'NONE', ( #23510, #13977, #39753, #35102 ) ) ;
#43496=DIRECTION ( 'NONE',  ( 0.000000000000000000, 0.000000000000000000, 1.000000000000000000 ) ) ;
#43497=DIRECTION ( 'NONE',  ( 0.000000000000000000, 0.000000000000000000, 1.000000000000000000 ) ) ;
#43498=LINE ( 'NONE', #19572, #8927 ) ;
#43499=DIRECTION ( 'NONE',  ( 0.8294056854502049880, 0.000000000000000000, -0.5586467658036476935 ) ) ;
#43502=VERTEX_POINT ( 'NONE', #4006 ) ;
#43503=AXIS2_PLACEMENT_3D ( 'NONE', #13404, #2076, #1309 ) ;
#43505=PLANE ( 'NONE',  #14529 ) ;
#43506=VERTEX_POINT ( 'NONE', #4522 ) ;
#43507=EDGE_CURVE ( 'NONE', #210, #38978, #12123, .T. ) ;
#43509=FACE_OUTER_BOUND ( 'NONE', #37980, .T. ) ;
#43511=ADVANCED_FACE ( 'NONE', ( #9252 ), #8202, .T. ) ;
#43513=ORIENTED_EDGE ( 'NONE', *, *, #21819, .T. ) ;
#43514=DIRECTION ( 'NONE',  ( -0.000000000000000000, 1.000000000000000000, -0.000000000000000000 ) ) ;
#43515=FACE_OUTER_BOUND ( 'NONE', #49328, .T. ) ;
#43518=ADVANCED_FACE ( 'NONE', ( #16095 ), #13190, .T. ) ;
#43519=DIRECTION ( 'NONE',  ( -0.000000000000000000, 1.000000000000000000, -0.000000000000000000 ) ) ;
#43520=DIRECTION ( 'NONE',  ( -0.000000000000000000, 1.000000000000000000, -0.000000000000000000 ) ) ;
#43522=EDGE_LOOP ( 'NONE', ( #44196, #48916, #22032, #24137 ) ) ;
#43523=EDGE_CURVE ( 'NONE', #42284, #19235, #44997, .T. ) ;
#43524=ORIENTED_EDGE ( 'NONE', *, *, #4766, .F. ) ;
#43525=PLANE ( 'NONE',  #49252 ) ;
#43528=ADVANCED_FACE ( 'NONE', ( #28155 ), #25023, .T. ) ;
#43529=AXIS2_PLACEMENT_3D ( 'NONE', #26778, #26009, #42033 ) ;
#43530=CARTESIAN_POINT ( 'NONE',  ( 34.93559171950835918, -183.6283474603465606, -93.09664195018496002 ) ) ;
#43531=DIRECTION ( 'NONE',  ( 0.000000000000000000, 0.000000000000000000, 1.000000000000000000 ) ) ;
#43532=PLANE ( 'NONE',  #49068 ) ;
#43533=ORIENTED_EDGE ( 'NONE', *, *, #18247, .T. ) ;
#43534=CARTESIAN_POINT ( 'NONE',  ( -9.671950287350391307, -177.1207230881787780, -118.8234112238815499 ) ) ;
#43535=ORIENTED_EDGE ( 'NONE', *, *, #47796, .T. ) ;
#43536=DIRECTION ( 'NONE',  ( -0.000000000000000000, 1.000000000000000000, -0.000000000000000000 ) ) ;
#43537=VERTEX_POINT ( 'NONE', #20537 ) ;
#43538=VECTOR ( 'NONE', #3627, 1000.000000000000000 ) ;
#43539=ORIENTED_EDGE ( 'NONE', *, *, #15773, .T. ) ;
#43541=ADVANCED_FACE ( 'NONE', ( #16874 ), #4257, .T. ) ;
#43543=LINE ( 'NONE', #7023, #31350 ) ;
#43545=EDGE_LOOP ( 'NONE', ( #20937, #41109, #16162, #48166 ) ) ;
#43546=CARTESIAN_POINT ( 'NONE',  ( -101.9736325116273576, -177.1207230881787780, 112.9749434763330811 ) ) ;
#43549=ORIENTED_EDGE ( 'NONE', *, *, #26926, .F. ) ;
#43550=LINE ( 'NONE', #40355, #17880 ) ;
#43551=DIRECTION ( 'NONE',  ( -0.6068001458186002006, 0.000000000000000000, 0.7948544414133481562 ) ) ;
#43552=DIRECTION ( 'NONE',  ( -0.9266896074318370369, 0.000000000000000000, 0.3758275821142292306 ) ) ;
#43554=DIRECTION ( 'NONE',  ( -1.000000000000000000, 0.000000000000000000, -4.884776371667510679E-16 ) ) ;
#43555=DIRECTION ( 'NONE',  ( 0.4031234292879600778, 0.000000000000000000, 0.9151456172430237901 ) ) ;
#43556=DIRECTION ( 'NONE',  ( -0.000000000000000000, 1.000000000000000000, 0.000000000000000000 ) ) ;
#43557=ORIENTED_EDGE ( 'NONE', *, *, #36202, .F. ) ;
#43558=CARTESIAN_POINT ( 'NONE',  ( -131.8938452225253855, -183.6283474603465606, 93.09664195018558530 ) ) ;
#43560=FACE_BOUND ( 'NONE', #19789, .T. ) ;
#43561=ORIENTED_EDGE ( 'NONE', *, *, #12788, .T. ) ;
#43562=AXIS2_PLACEMENT_3D ( 'NONE', #37034, #13129, #29150 ) ;
#43565=CARTESIAN_POINT ( 'NONE',  ( -48.65601702663141737, -183.6283474603465606, -0.9842305779475923888 ) ) ;
#43566=EDGE_CURVE ( 'NONE', #10561, #4246, #12648, .T. ) ;
#43567=VERTEX_POINT ( 'NONE', #45267 ) ;
#43569=CARTESIAN_POINT ( 'NONE',  ( -30.31202594373734627, -193.5000000000000000, -123.6727797384705809 ) ) ;
#43570=ORIENTED_EDGE ( 'NONE', *, *, #2036, .T. ) ;
#43571=VECTOR ( 'NONE', #14116, 1000.000000000000000 ) ;
#43573=FACE_BOUND ( 'NONE', #46657, .T. ) ;
#43575=EDGE_LOOP ( 'NONE', ( #2919, #40811, #10760, #43304 ) ) ;
#43576=EDGE_CURVE ( 'NONE', #24186, #6302, #8452, .T. ) ;
#43577=DIRECTION ( 'NONE',  ( -0.000000000000000000, -1.000000000000000000, 0.000000000000000000 ) ) ;
#43579=ADVANCED_FACE ( 'NONE', ( #16348 ), #12393, .T. ) ;
#43580=AXIS2_PLACEMENT_3D ( 'NONE', #35849, #17126, #45253 ) ;
#43584=ORIENTED_EDGE ( 'NONE', *, *, #14684, .T. ) ;
#43585=PLANE ( 'NONE',  #48611 ) ;
#43586=EDGE_CURVE ( 'NONE', #993, #20913, #37086, .T. ) ;
#43588=DIRECTION ( 'NONE',  ( 0.000000000000000000, 0.000000000000000000, 1.000000000000000000 ) ) ;
#43592=ORIENTED_EDGE ( 'NONE', *, *, #43111, .F. ) ;
#43594=CARTESIAN_POINT ( 'NONE',  ( -78.00521078983979351, -193.5000000000000000, 121.4627941443857111 ) ) ;
#43595=EDGE_LOOP ( 'NONE', ( #10750, #17627, #9215, #45574 ) ) ;
#43596=DIRECTION ( 'NONE',  ( 0.000000000000000000, 1.000000000000000000, 0.000000000000000000 ) ) ;
#43597=CIRCLE ( 'NONE', #27535, 125.0000000000000000 ) ;
#43599=PLANE ( 'NONE',  #35962 ) ;
#43602=DIRECTION ( 'NONE',  ( 0.000000000000000000, 1.000000000000000000, 0.000000000000000000 ) ) ;
#43604=CARTESIAN_POINT ( 'NONE',  ( 72.71365293123227502, -183.6283474603465606, -30.61552143554913030 ) ) ;
#43606=PLANE ( 'NONE',  #3537 ) ;
#43607=PLANE ( 'NONE',  #26522 ) ;
#43610=FACE_OUTER_BOUND ( 'NONE', #16413, .T. ) ;
#43612=ORIENTED_EDGE ( 'NONE', *, *, #3577, .T. ) ;
#43616=CIRCLE ( 'NONE', #15944, 125.0000000000000000 ) ;
#43617=ADVANCED_FACE ( 'NONE', ( #44725 ), #24749, .T. ) ;
#43618=DIRECTION ( 'NONE',  ( -0.000000000000000000, 1.000000000000000000, -0.000000000000000000 ) ) ;
#43622=ADVANCED_FACE ( 'NONE', ( #21065 ), #17135, .T. ) ;
#43623=CARTESIAN_POINT ( 'NONE',  ( -169.1033029113419559, -189.7472609257535510, 32.78426643622744052 ) ) ;
#43624=DIRECTION ( 'NONE',  ( 0.000000000000000000, 1.000000000000000000, -0.000000000000000000 ) ) ;
#43628=ORIENTED_EDGE ( 'NONE', *, *, #4271, .T. ) ;
#43629=ORIENTED_EDGE ( 'NONE', *, *, #26294, .F. ) ;
#43630=ADVANCED_FACE ( 'NONE', ( #17912 ), #29460, .F. ) ;
#43633=CARTESIAN_POINT ( 'NONE',  ( -48.47912675150885065, -177.1207230881787780, 6.938893903907228378E-15 ) ) ;
#43637=ADVANCED_FACE ( 'NONE', ( #13703 ), #45512, .T. ) ;
#43639=EDGE_CURVE ( 'NONE', #49683, #40790, #1777, .T. ) ;
#43642=EDGE_CURVE ( 'NONE', #21275, #31707, #38118, .T. ) ;
#43643=VERTEX_POINT ( 'NONE', #46295 ) ;
#43644=LINE ( 'NONE', #36268, #12457 ) ;
#43646=CARTESIAN_POINT ( 'NONE',  ( -49.38192458147459973, -177.1207230881787780, 0.4300652022765185656 ) ) ;
#43649=AXIS2_PLACEMENT_3D ( 'NONE', #26129, #46131, #10112 ) ;
#43651=DIRECTION ( 'NONE',  ( 0.000000000000000000, 1.000000000000000000, 0.000000000000000000 ) ) ;
#43653=DIRECTION ( 'NONE',  ( 0.8757349421956310831, 0.000000000000000000, 0.4827922027307550712 ) ) ;
#43654=CARTESIAN_POINT ( 'NONE',  ( -15.48416040178639008, -183.6283474603465606, 119.5301634136914970 ) ) ;
#43655=EDGE_LOOP ( 'NONE', ( #4274, #22120, #17056, #14021 ) ) ;
#43656=DIRECTION ( 'NONE',  ( -0.9646355819083576311, 0.000000000000000000, -0.2635871660690715101 ) ) ;
#43659=ORIENTED_EDGE ( 'NONE', *, *, #41486, .F. ) ;
#43661=DIRECTION ( 'NONE',  ( 0.000000000000000000, 1.000000000000000000, -0.000000000000000000 ) ) ;
#43662=DIRECTION ( 'NONE',  ( 0.000000000000000000, -1.000000000000000000, -0.000000000000000000 ) ) ;
#43663=CARTESIAN_POINT ( 'NONE',  ( 19.33815737959698566, -193.5000000000000000, 105.0038855142078233 ) ) ;
#43667=PLANE ( 'NONE',  #14434 ) ;
#43668=PLANE ( 'NONE',  #29228 ) ;
#43669=AXIS2_PLACEMENT_3D ( 'NONE', #45660, #38268, #9645 ) ;
#43670=ORIENTED_EDGE ( 'NONE', *, *, #7511, .T. ) ;
#43672=PLANE ( 'NONE',  #8913 ) ;
#43673=CARTESIAN_POINT ( 'NONE',  ( -146.0653709326077490, -189.7472609257535510, -78.11481899503411341 ) ) ;
#43674=ORIENTED_EDGE ( 'NONE', *, *, #14930, .T. ) ;
#43676=FACE_OUTER_BOUND ( 'NONE', #25100, .T. ) ;
#43678=VERTEX_POINT ( 'NONE', #14489 ) ;
#43679=LINE ( 'NONE', #22937, #45103 ) ;
#43680=ORIENTED_EDGE ( 'NONE', *, *, #4927, .F. ) ;
#43681=LINE ( 'NONE', #31072, #23133 ) ;
#43683=ADVANCED_FACE ( 'NONE', ( #25272 ), #45766, .T. ) ;
#43684=PLANE ( 'NONE',  #38622 ) ;
#43685=DIRECTION ( 'NONE',  ( 0.000000000000000000, 0.000000000000000000, 1.000000000000000000 ) ) ;
#43686=DIRECTION ( 'NONE',  ( -0.000000000000000000, 1.000000000000000000, -0.000000000000000000 ) ) ;
#43687=ADVANCED_FACE ( 'NONE', ( #41286 ), #5573, .T. ) ;
#43690=AXIS2_PLACEMENT_3D ( 'NONE', #6912, #22944, #35027 ) ;
#43691=DIRECTION ( 'NONE',  ( -0.000000000000000000, 1.000000000000000000, -0.000000000000000000 ) ) ;
#43693=DIRECTION ( 'NONE',  ( 0.7378332790417189146, 0.000000000000000000, 0.6749830015182196608 ) ) ;
#43694=CARTESIAN_POINT ( 'NONE',  ( -146.0653709326077490, -175.3837268820161057, -78.11481899503409920 ) ) ;
#43695=CARTESIAN_POINT ( 'NONE',  ( -123.4791267515088435, -173.5000000000000284, 80.00000000000000000 ) ) ;
#43697=ORIENTED_EDGE ( 'NONE', *, *, #33741, .T. ) ;
#43699=CARTESIAN_POINT ( 'NONE',  ( -48.47912675150885065, -183.6283474603465606, 6.938893903907228378E-15 ) ) ;
#43700=VERTEX_POINT ( 'NONE', #17410 ) ;
#43702=AXIS2_PLACEMENT_3D ( 'NONE', #9851, #2220, #50323 ) ;
#43703=LINE ( 'NONE', #7703, #44987 ) ;
#43704=EDGE_CURVE ( 'NONE', #14725, #18880, #25791, .T. ) ;
#43706=CARTESIAN_POINT ( 'NONE',  ( 10.22625775207004928, -193.5000000000000000, -109.2239789693433352 ) ) ;
#43708=FACE_OUTER_BOUND ( 'NONE', #31208, .T. ) ;
#43709=DIRECTION ( 'NONE',  ( -0.000000000000000000, 1.000000000000000000, -0.000000000000000000 ) ) ;
#43710=ORIENTED_EDGE ( 'NONE', *, *, #36002, .T. ) ;
#43712=EDGE_CURVE ( 'NONE', #43188, #40339, #32506, .T. ) ;
#43713=ORIENTED_EDGE ( 'NONE', *, *, #40235, .F. ) ;
#43714=CARTESIAN_POINT ( 'NONE',  ( 44.30815888362531041, -175.3837268820161057, 83.75869879877568280 ) ) ;
#43715=DIRECTION ( 'NONE',  ( -0.9646355819083614058, 0.000000000000000000, 0.2635871660690581320 ) ) ;
#43717=FACE_OUTER_BOUND ( 'NONE', #45431, .T. ) ;
#43718=FACE_OUTER_BOUND ( 'NONE', #50893, .T. ) ;
#43719=ORIENTED_EDGE ( 'NONE', *, *, #10125, .T. ) ;
#43720=DIRECTION ( 'NONE',  ( 0.000000000000000000, 0.000000000000000000, 1.000000000000000000 ) ) ;
#43721=AXIS2_PLACEMENT_3D ( 'NONE', #30758, #27325, #43103 ) ;
#43722=CARTESIAN_POINT ( 'NONE',  ( -90.87721961371603641, -175.3837268820161057, 116.5264228893328777 ) ) ;
#43723=LINE ( 'NONE', #29250, #18197 ) ;
#43724=VECTOR ( 'NONE', #33672, 1000.000000000000114 ) ;
#43726=ORIENTED_EDGE ( 'NONE', *, *, #51006, .F. ) ;
#43727=ORIENTED_EDGE ( 'NONE', *, *, #25687, .F. ) ;
#43728=DIRECTION ( 'NONE',  ( 0.000000000000000000, 1.000000000000000000, -0.000000000000000000 ) ) ;
#43730=ORIENTED_EDGE ( 'NONE', *, *, #19617, .F. ) ;
#43735=CARTESIAN_POINT ( 'NONE',  ( -74.51199343215203896, -193.5000000000000000, -122.2591094863194598 ) ) ;
#43736=VERTEX_POINT ( 'NONE', #18934 ) ;
#43738=FACE_BOUND ( 'NONE', #36911, .T. ) ;
#43739=CARTESIAN_POINT ( 'NONE',  ( -109.9568094315246327, -193.5000000000000000, -108.8370090194290611 ) ) ;
#43740=ORIENTED_EDGE ( 'NONE', *, *, #3694, .T. ) ;
#43741=CARTESIAN_POINT ( 'NONE',  ( -48.53836737940257251, -193.5000000000000000, 0.9982437317643279018 ) ) ;
#43742=CARTESIAN_POINT ( 'NONE',  ( -162.9896759831413249, -193.5000000000000000, -50.12318939043961308 ) ) ;
#43743=CARTESIAN_POINT ( 'NONE',  ( 60.58466639580034041, -193.5000000000000000, -61.07445476073405644 ) ) ;
#43744=EDGE_CURVE ( 'NONE', #19552, #10747, #26942, .T. ) ;
#43746=VERTEX_POINT ( 'NONE', #15513 ) ;
#43747=DIRECTION ( 'NONE',  ( 0.000000000000000000, 0.000000000000000000, -1.000000000000000000 ) ) ;
#43749=ORIENTED_EDGE ( 'NONE', *, *, #22922, .F. ) ;
#43750=CARTESIAN_POINT ( 'NONE',  ( -56.05401443572774411, -193.5000000000000000, 124.7702732086912931 ) ) ;
#43751=CARTESIAN_POINT ( 'NONE',  ( -49.30901192927175458, -193.5000000000000000, -124.9972451320097093 ) ) ;
#43752=ORIENTED_EDGE ( 'NONE', *, *, #50761, .T. ) ;
#43754=VERTEX_POINT ( 'NONE', #20411 ) ;
#43761=DIRECTION ( 'NONE',  ( 0.000000000000000000, -1.000000000000000000, 0.000000000000000000 ) ) ;
#43762=EDGE_CURVE ( 'NONE', #15743, #7849, #27593, .T. ) ;
#43764=CARTESIAN_POINT ( 'NONE',  ( 69.72248760683812918, -177.1207230881787780, -37.47770156625421833 ) ) ;
#43765=LINE ( 'NONE', #12219, #38390 ) ;
#43766=DIRECTION ( 'NONE',  ( 0.000000000000000000, -0.000000000000000000, 1.000000000000000000 ) ) ;
#43767=DIRECTION ( 'NONE',  ( 0.000000000000000000, 0.000000000000000000, 1.000000000000000000 ) ) ;
#43768=ORIENTED_EDGE ( 'NONE', *, *, #2080, .F. ) ;
#43770=ORIENTED_EDGE ( 'NONE', *, *, #13771, .T. ) ;
#43772=DIRECTION ( 'NONE',  ( 0.9646355819083576311, 0.000000000000000000, 0.2635871660690715101 ) ) ;
#43773=DIRECTION ( 'NONE',  ( 0.000000000000000000, 0.000000000000000000, 1.000000000000000000 ) ) ;
#43774=CIRCLE ( 'NONE', #51373, 125.0000000000000000 ) ;
#43776=FACE_OUTER_BOUND ( 'NONE', #31918, .T. ) ;
#43781=ORIENTED_EDGE ( 'NONE', *, *, #33535, .T. ) ;
#43782=CARTESIAN_POINT ( 'NONE',  ( -127.6327502296859535, -193.5000000000000000, -95.45105364470084908 ) ) ;
#43784=EDGE_LOOP ( 'NONE', ( #30599, #16085, #163, #50312 ) ) ;
#43788=VECTOR ( 'NONE', #12898, 1000.000000000000227 ) ;
#43789=FACE_OUTER_BOUND ( 'NONE', #9041, .T. ) ;
#43790=DIRECTION ( 'NONE',  ( 0.05924062789370006937, 0.000000000000000000, 0.9982437317643222396 ) ) ;
#43791=ORIENTED_EDGE ( 'NONE', *, *, #34198, .T. ) ;
#43792=CARTESIAN_POINT ( 'NONE',  ( -48.47912675150885065, -175.3837268820161057, 6.938893903907228378E-15 ) ) ;
#43793=AXIS2_PLACEMENT_3D ( 'NONE', #49775, #46351, #26358 ) ;
#43794=ORIENTED_EDGE ( 'NONE', *, *, #25634, .T. ) ;
#43795=VECTOR ( 'NONE', #46049, 1000.000000000000114 ) ;
#43796=EDGE_CURVE ( 'NONE', #2344, #14293, #35215, .T. ) ;
#43797=EDGE_LOOP ( 'NONE', ( #9471, #43276, #24391, #10108 ) ) ;
#43800=PLANE ( 'NONE',  #40695 ) ;
#43801=DIRECTION ( 'NONE',  ( 0.000000000000000000, 0.000000000000000000, -1.000000000000000000 ) ) ;
#43802=LINE ( 'NONE', #38825, #13658 ) ;
#43803=EDGE_CURVE ( 'NONE', #17270, #50197, #14355, .T. ) ;
#43806=CARTESIAN_POINT ( 'NONE',  ( 75.04604393171729271, -189.7472609257535510, -10.84123789944573168 ) ) ;
#43807=VECTOR ( 'NONE', #48685, 1000.000000000000000 ) ;
#43808=FACE_BOUND ( 'NONE', #32200, .T. ) ;
#43809=ORIENTED_EDGE ( 'NONE', *, *, #42798, .T. ) ;
#43811=ADVANCED_FACE ( 'NONE', ( #16484 ), #51267, .T. ) ;
#43813=DIRECTION ( 'NONE',  ( -0.000000000000000000, 1.000000000000000000, 0.000000000000000000 ) ) ;
#43814=CARTESIAN_POINT ( 'NONE',  ( 75.02564229359539638, -189.7472609257535510, -19.27620354518635182 ) ) ;
#43815=EDGE_LOOP ( 'NONE', ( #37633, #10615, #5332, #11374, #31003, #44721, #3002, #26180, #44154, #11785, #1838, #39300, #1700, #48317, #28572, #47235, #40542, #19909 ) ) ;
#43816=DIRECTION ( 'NONE',  ( 0.8757349421956412971, 0.000000000000000000, -0.4827922027307366970 ) ) ;
#43817=ORIENTED_EDGE ( 'NONE', *, *, #43642, .F. ) ;
#43818=CARTESIAN_POINT ( 'NONE',  ( -134.9506378406916554, -189.7472609257535510, 90.26448786734091811 ) ) ;
#43819=FACE_BOUND ( 'NONE', #45333, .T. ) ;
#43820=DIRECTION ( 'NONE',  ( -0.8455960035018234011, 0.000000000000000000, -0.5338233779647948429 ) ) ;
#43823=VECTOR ( 'NONE', #10192, 1000.000000000000000 ) ;
#43825=EDGE_LOOP ( 'NONE', ( #16122, #6911, #17320, #50159 ) ) ;
#43828=ORIENTED_EDGE ( 'NONE', *, *, #40112, .T. ) ;
#43829=DIRECTION ( 'NONE',  ( 0.000000000000000000, -1.000000000000000000, -0.000000000000000000 ) ) ;
#43830=CARTESIAN_POINT ( 'NONE',  ( -48.02249751411514467, -193.5000000000000000, 0.8896570909947569827 ) ) ;
#43831=CIRCLE ( 'NONE', #19495, 125.0000000000000000 ) ;
#43832=VECTOR ( 'NONE', #21112, 1000.000000000000000 ) ;
#43834=CARTESIAN_POINT ( 'NONE',  ( -157.8637630444124795, -175.3837268820161057, -60.49794494914009135 ) ) ;
#43837=CARTESIAN_POINT ( 'NONE',  ( -106.4764934152196645, -213.5000000000000000, 110.7307791902283043 ) ) ;
#43839=CIRCLE ( 'NONE', #51408, 124.9999999999999858 ) ;
#43842=DIRECTION ( 'NONE',  ( -0.9785564922995017012, 0.000000000000000000, -0.2059786187411094538 ) ) ;
#43847=EDGE_CURVE ( 'NONE', #24293, #21281, #41199, .T. ) ;
#43850=VERTEX_POINT ( 'NONE', #10526 ) ;
#43851=DIRECTION ( 'NONE',  ( -0.000000000000000000, 1.000000000000000000, -0.000000000000000000 ) ) ;
#43852=DIRECTION ( 'NONE',  ( -0.5085311186492154079, 0.000000000000000000, -0.8610436117673585521 ) ) ;
#43853=VERTEX_POINT ( 'NONE', #42843 ) ;
#43854=CARTESIAN_POINT ( 'NONE',  ( -121.8391548840036620, -183.6283474603465606, -99.97252634603250954 ) ) ;
#43855=ORIENTED_EDGE ( 'NONE', *, *, #32956, .F. ) ;
#43856=FACE_OUTER_BOUND ( 'NONE', #3583, .T. ) ;
#43857=DIRECTION ( 'NONE',  ( -0.000000000000000000, 1.000000000000000000, 0.000000000000000000 ) ) ;
#43858=DIRECTION ( 'NONE',  ( -0.000000000000000000, 1.000000000000000000, -0.000000000000000000 ) ) ;
#43860=PLANE ( 'NONE',  #20733 ) ;
#43862=DIRECTION ( 'NONE',  ( 0.000000000000000000, 0.000000000000000000, -1.000000000000000000 ) ) ;
#43863=VERTEX_POINT ( 'NONE', #6849 ) ;
#43865=ADVANCED_FACE ( 'NONE', ( #34950 ), #47583, .T. ) ;
#43866=CARTESIAN_POINT ( 'NONE',  ( 43.63512310656542326, -193.5000000000000000, 84.49831343337136502 ) ) ;
#43867=CARTESIAN_POINT ( 'NONE',  ( 18.00181100848376303, -193.5000000000000000, -105.8550183720733742 ) ) ;
#43871=ORIENTED_EDGE ( 'NONE', *, *, #23986, .T. ) ;
#43872=EDGE_CURVE ( 'NONE', #21582, #38978, #2607, .T. ) ;
#43878=ORIENTED_EDGE ( 'NONE', *, *, #23126, .T. ) ;
#43879=AXIS2_PLACEMENT_3D ( 'NONE', #35211, #27322, #3160 ) ;
#43880=EDGE_LOOP ( 'NONE', ( #591, #16990, #10191, #45778 ) ) ;
#43881=VECTOR ( 'NONE', #51998, 1000.000000000000000 ) ;
#43882=VECTOR ( 'NONE', #1288, 1000.000000000000000 ) ;
#43883=CARTESIAN_POINT ( 'NONE',  ( -148.6149069237406195, -177.1207230881787780, -74.81861753132353954 ) ) ;
#43885=DIRECTION ( 'NONE',  ( 0.5085311186492154079, 0.000000000000000000, 0.8610436117673585521 ) ) ;
#43887=CARTESIAN_POINT ( 'NONE',  ( -161.2555905272864436, -175.3837268820161057, -53.91167979418489864 ) ) ;
#43888=ORIENTED_EDGE ( 'NONE', *, *, #19626, .F. ) ;
#43889=AXIS2_PLACEMENT_3D ( 'NONE', #36385, #27469, #12475 ) ;
#43891=ORIENTED_EDGE ( 'NONE', *, *, #8331, .F. ) ;
#43892=ORIENTED_EDGE ( 'NONE', *, *, #31110, .F. ) ;
#43893=ORIENTED_EDGE ( 'NONE', *, *, #12827, .T. ) ;
#43894=DIRECTION ( 'NONE',  ( -0.000000000000000000, 1.000000000000000000, -0.000000000000000000 ) ) ;
#43895=VECTOR ( 'NONE', #23515, 1000.000000000000000 ) ;
#43896=ORIENTED_EDGE ( 'NONE', *, *, #29045, .F. ) ;
#43897=AXIS2_PLACEMENT_3D ( 'NONE', #8466, #32648, #28687 ) ;
#43898=LINE ( 'NONE', #23925, #23463 ) ;
#43900=CARTESIAN_POINT ( 'NONE',  ( -89.73513343757494454, -193.5000000000000000, -117.9955164924467397 ) ) ;
#43902=ORIENTED_EDGE ( 'NONE', *, *, #16338, .T. ) ;
#43904=ORIENTED_EDGE ( 'NONE', *, *, #4162, .F. ) ;
#43907=EDGE_CURVE ( 'NONE', #18747, #43197, #714, .T. ) ;
#43908=EDGE_CURVE ( 'NONE', #16384, #38633, #4648, .T. ) ;
#43910=CARTESIAN_POINT ( 'NONE',  ( 32.34187644556187280, -175.3837268820161057, 94.04236105995857997 ) ) ;
#43912=CARTESIAN_POINT ( 'NONE',  ( -50.89116676070551648, -193.5000000000000000, 124.9767260852757147 ) ) ;
#43913=CARTESIAN_POINT ( 'NONE',  ( -77.77032474405881146, -193.5000000000000000, 120.4907712303052989 ) ) ;
#43916=EDGE_CURVE ( 'NONE', #34663, #28107, #37907, .T. ) ;
#43917=LINE ( 'NONE', #7427, #19786 ) ;
#43918=AXIS2_PLACEMENT_3D ( 'NONE', #22013, #42498, #6521 ) ;
#43919=PLANE ( 'NONE',  #36244 ) ;
#43920=ORIENTED_EDGE ( 'NONE', *, *, #31193, .T. ) ;
#43921=ADVANCED_FACE ( 'NONE', ( #21723 ), #20675, .T. ) ;
#43923=DIRECTION ( 'NONE',  ( -0.000000000000000000, 1.000000000000000000, -0.000000000000000000 ) ) ;
#43924=EDGE_CURVE ( 'NONE', #12141, #36143, #48809, .T. ) ;
#43925=FACE_OUTER_BOUND ( 'NONE', #5299, .T. ) ;
#43927=DIRECTION ( 'NONE',  ( 0.000000000000000000, -1.000000000000000000, -0.000000000000000000 ) ) ;
#43928=VECTOR ( 'NONE', #37749, 1000.000000000000114 ) ;
#43929=EDGE_CURVE ( 'NONE', #41184, #23109, #40392, .T. ) ;
#43930=FACE_OUTER_BOUND ( 'NONE', #12148, .T. ) ;
#43932=ORIENTED_EDGE ( 'NONE', *, *, #35692, .T. ) ;
#43933=LINE ( 'NONE', #11093, #3100 ) ;
#43935=EDGE_CURVE ( 'NONE', #43203, #9007, #36967, .T. ) ;
#43936=CARTESIAN_POINT ( 'NONE',  ( -136.1415351158078693, -189.7472609257535510, -89.10837311819173578 ) ) ;
#43937=CARTESIAN_POINT ( 'NONE',  ( -59.28786813212838069, -177.1207230881787780, 124.5318076226587323 ) ) ;
#43941=LINE ( 'NONE', #20282, #39016 ) ;
#43944=DIRECTION ( 'NONE',  ( -0.05924062789371441901, 0.000000000000000000, 0.9982437317643214625 ) ) ;
#43947=PLANE ( 'NONE',  #8539 ) ;
#43949=ORIENTED_EDGE ( 'NONE', *, *, #14775, .T. ) ;
#43953=DIRECTION ( 'NONE',  ( 0.000000000000000000, 0.000000000000000000, 1.000000000000000000 ) ) ;
#43954=ORIENTED_EDGE ( 'NONE', *, *, #48812, .T. ) ;
#43956=ORIENTED_EDGE ( 'NONE', *, *, #23303, .F. ) ;
#43958=PLANE ( 'NONE',  #51872 ) ;
#43960=LINE ( 'NONE', #27413, #13206 ) ;
#43961=VERTEX_POINT ( 'NONE', #40899 ) ;
#43962=ORIENTED_EDGE ( 'NONE', *, *, #15882, .F. ) ;
#43964=EDGE_CURVE ( 'NONE', #775, #26963, #10182, .T. ) ;
#43968=DIRECTION ( 'NONE',  ( -0.000000000000000000, 1.000000000000000000, -0.000000000000000000 ) ) ;
#43970=AXIS2_PLACEMENT_3D ( 'NONE', #12260, #28546, #7807 ) ;
#43971=EDGE_LOOP ( 'NONE', ( #25270, #22094, #17153, #25986 ) ) ;
#43972=FACE_OUTER_BOUND ( 'NONE', #21127, .T. ) ;
#43973=CIRCLE ( 'NONE', #41459, 125.0000000000000000 ) ;
#43975=EDGE_CURVE ( 'NONE', #9933, #17165, #41163, .T. ) ;
#43977=LINE ( 'NONE', #16391, #3934 ) ;
#43978=CARTESIAN_POINT ( 'NONE',  ( 23.54917025746143011, -183.6283474603465606, -100.9358816284410665 ) ) ;
#43980=AXIS2_PLACEMENT_3D ( 'NONE', #49581, #41157, #17260 ) ;
#43982=ORIENTED_EDGE ( 'NONE', *, *, #17309, .F. ) ;
#43983=VERTEX_POINT ( 'NONE', #25651 ) ;
#43984=VERTEX_POINT ( 'NONE', #1486 ) ;
#43986=CARTESIAN_POINT ( 'NONE',  ( -170.9669310976187830, -193.5000000000000000, -24.93467037017130394 ) ) ;
#43987=ORIENTED_EDGE ( 'NONE', *, *, #30844, .T. ) ;
#43991=ORIENTED_EDGE ( 'NONE', *, *, #13010, .T. ) ;
#43993=AXIS2_PLACEMENT_3D ( 'NONE', #30084, #6702, #1969 ) ;
#43995=CARTESIAN_POINT ( 'NONE',  ( -48.13092511607445800, -177.1207230881787780, 0.9374196611341301111 ) ) ;
#43998=EDGE_CURVE ( 'NONE', #12404, #46929, #29591, .T. ) ;
#43999=DIRECTION ( 'NONE',  ( -0.000000000000000000, 1.000000000000000000, -0.000000000000000000 ) ) ;
#44000=ORIENTED_EDGE ( 'NONE', *, *, #46933, .T. ) ;
#44002=CARTESIAN_POINT ( 'NONE',  ( -8.461066480258370603, -193.5000000000000000, 117.3655938605930231 ) ) ;
#44003=CARTESIAN_POINT ( 'NONE',  ( -41.90263914168912152, -189.7472609257535510, -124.8268793598473536 ) ) ;
#44005=CARTESIAN_POINT ( 'NONE',  ( -47.70260288879080690, -193.5000000000000000, -0.6300878435817026668 ) ) ;
#44007=EDGE_LOOP ( 'NONE', ( #36100, #42427, #36383, #22540 ) ) ;
#44009=ORIENTED_EDGE ( 'NONE', *, *, #12355, .T. ) ;
#44012=DIRECTION ( 'NONE',  ( 0.000000000000000000, 1.000000000000000000, 0.000000000000000000 ) ) ;
#44014=VECTOR ( 'NONE', #26017, 1000.000000000000114 ) ;
#44019=ADVANCED_FACE ( 'NONE', ( #1994 ), #26694, .T. ) ;
#44024=VERTEX_POINT ( 'NONE', #34060 ) ;
#44028=AXIS2_PLACEMENT_3D ( 'NONE', #46840, #50006, #14261 ) ;
#44029=PLANE ( 'NONE',  #14871 ) ;
#44030=ORIENTED_EDGE ( 'NONE', *, *, #13019, .T. ) ;
#44033=PLANE ( 'NONE',  #43390 ) ;
#44034=LINE ( 'NONE', #11717, #48662 ) ;
#44035=CARTESIAN_POINT ( 'NONE',  ( 22.03849146056077757, -193.5000000000000000, 103.2098131075567409 ) ) ;
#44038=ORIENTED_EDGE ( 'NONE', *, *, #32339, .T. ) ;
#44040=EDGE_CURVE ( 'NONE', #27293, #2653, #34814, .T. ) ;
#44041=CARTESIAN_POINT ( 'NONE',  ( 68.93474881819258826, -193.5000000000000000, 39.87457906003773900 ) ) ;
#44043=DIRECTION ( 'NONE',  ( -0.000000000000000000, 1.000000000000000000, -0.000000000000000000 ) ) ;
#44044=ORIENTED_EDGE ( 'NONE', *, *, #20547, .T. ) ;
#44045=ORIENTED_EDGE ( 'NONE', *, *, #20646, .F. ) ;
#44046=CIRCLE ( 'NONE', #50776, 125.0000000000000000 ) ;
#44047=CARTESIAN_POINT ( 'NONE',  ( -165.7578939544008847, -183.6283474603465606, -43.25148278810625868 ) ) ;
#44048=CARTESIAN_POINT ( 'NONE',  ( 68.21542617880035664, -183.6283474603465606, 41.93543928473692262 ) ) ;
#44049=VECTOR ( 'NONE', #27950, 1000.000000000000000 ) ;
#44054=CARTESIAN_POINT ( 'NONE',  ( -49.35486169370448550, -183.6283474603465606, -0.4827922027307481878 ) ) ;
#44056=VECTOR ( 'NONE', #19506, 1000.000000000000000 ) ;
#44057=ORIENTED_EDGE ( 'NONE', *, *, #17952, .T. ) ;
#44059=VECTOR ( 'NONE', #29690, 1000.000000000000000 ) ;
#44061=FACE_OUTER_BOUND ( 'NONE', #9847, .T. ) ;
#44062=PLANE ( 'NONE',  #18997 ) ;
#44063=AXIS2_PLACEMENT_3D ( 'NONE', #665, #31932, #4599 ) ;
#44064=CARTESIAN_POINT ( 'NONE',  ( -123.6678354051270077, -175.3837268820161057, 99.85818990449067201 ) ) ;
#44065=CYLINDRICAL_SURFACE ( 'NONE', #19639, 125.0000000000000000 ) ;
#44066=CARTESIAN_POINT ( 'NONE',  ( -40.24578378811990831, -193.5000000000000000, 124.7285535218268251 ) ) ;
#44067=VERTEX_POINT ( 'NONE', #2267 ) ;
#44068=AXIS2_PLACEMENT_3D ( 'NONE', #22141, #46074, #17695 ) ;
#44069=FACE_OUTER_BOUND ( 'NONE', #16921, .T. ) ;
#44070=DIRECTION ( 'NONE',  ( 0.000000000000000000, -1.000000000000000000, -0.000000000000000000 ) ) ;
#44072=AXIS2_PLACEMENT_3D ( 'NONE', #12026, #462, #28056 ) ;
#44073=FACE_BOUND ( 'NONE', #27138, .T. ) ;
#44074=VERTEX_POINT ( 'NONE', #42972 ) ;
#44076=DIRECTION ( 'NONE',  ( 0.000000000000000000, 0.000000000000000000, 1.000000000000000000 ) ) ;
#44077=ORIENTED_EDGE ( 'NONE', *, *, #47159, .F. ) ;
#44078=CARTESIAN_POINT ( 'NONE',  ( 75.46126020185813843, -175.3837268820161057, 3.844569333773209419 ) ) ;
#44080=DIRECTION ( 'NONE',  ( 0.000000000000000000, 1.000000000000000000, 0.000000000000000000 ) ) ;
#44081=VECTOR ( 'NONE', #2895, 1000.000000000000000 ) ;
#44082=FACE_BOUND ( 'NONE', #35483, .T. ) ;
#44083=DIRECTION ( 'NONE',  ( 0.5338233779647948429, 0.000000000000000000, -0.8455960035018234011 ) ) ;
#44084=CIRCLE ( 'NONE', #39046, 125.0000000000000000 ) ;
#44086=DIRECTION ( 'NONE',  ( -0.7765238627180349740, 0.000000000000000000, -0.6300878435817203194 ) ) ;
#44087=ORIENTED_EDGE ( 'NONE', *, *, #22939, .T. ) ;
#44089=EDGE_CURVE ( 'NONE', #29776, #21157, #41939, .T. ) ;
#44092=ORIENTED_EDGE ( 'NONE', *, *, #19549, .T. ) ;
#44094=DIRECTION ( 'NONE',  ( 0.000000000000000000, -1.000000000000000000, 0.000000000000000000 ) ) ;
#44095=VECTOR ( 'NONE', #23229, 1000.000000000000227 ) ;
#44097=EDGE_CURVE ( 'NONE', #38627, #22578, #31186, .T. ) ;
#44098=VECTOR ( 'NONE', #19670, 1000.000000000000000 ) ;
#44101=CARTESIAN_POINT ( 'NONE',  ( -49.42645310536304493, -175.3837268820161057, 0.3202698538628349079 ) ) ;
#44104=FACE_OUTER_BOUND ( 'NONE', #6377, .T. ) ;
#44106=EDGE_CURVE ( 'NONE', #39370, #46453, #14102, .T. ) ;
#44107=VERTEX_POINT ( 'NONE', #30119 ) ;
#44108=DIRECTION ( 'NONE',  ( 0.000000000000000000, 0.000000000000000000, 1.000000000000000000 ) ) ;
#44109=VERTEX_POINT ( 'NONE', #6728 ) ;
#44110=DIRECTION ( 'NONE',  ( 0.6068001458185834363, 0.000000000000000000, 0.7948544414133608127 ) ) ;
#44111=EDGE_LOOP ( 'NONE', ( #451, #15023, #40604, #29451 ) ) ;
#44112=CARTESIAN_POINT ( 'NONE',  ( 21.21056010634071853, -175.3837268820161057, 103.7706487676302061 ) ) ;
#44113=ORIENTED_EDGE ( 'NONE', *, *, #49783, .T. ) ;
#44116=ORIENTED_EDGE ( 'NONE', *, *, #30459, .T. ) ;
#44117=EDGE_LOOP ( 'NONE', ( #4220, #2540, #39274, #20041 ) ) ;
#44118=DIRECTION ( 'NONE',  ( 0.8124868780056863082, 0.000000000000000000, -0.5829794791144649047 ) ) ;
#44120=CARTESIAN_POINT ( 'NONE',  ( -58.29063029684667185, -193.5000000000000000, 124.6143426664034877 ) ) ;
#44121=ADVANCED_FACE ( 'NONE', ( #46163 ), #14882, .T. ) ;
#44123=DIRECTION ( 'NONE',  ( 0.000000000000000000, 0.000000000000000000, -1.000000000000000000 ) ) ;
#44124=CARTESIAN_POINT ( 'NONE',  ( -48.47912675150885065, -177.1207230881787780, 6.938893903907228378E-15 ) ) ;
#44125=CIRCLE ( 'NONE', #10550, 125.0000000000000000 ) ;
#44126=DIRECTION ( 'NONE',  ( 0.000000000000000000, 1.000000000000000000, 0.000000000000000000 ) ) ;
#44132=DIRECTION ( 'NONE',  ( 0.000000000000000000, 0.000000000000000000, 1.000000000000000000 ) ) ;
#44133=CARTESIAN_POINT ( 'NONE',  ( 49.10711742958949344, -193.5000000000000000, 78.11481899503480975 ) ) ;
#44135=DIRECTION ( 'NONE',  ( 0.000000000000000000, -1.000000000000000000, 0.000000000000000000 ) ) ;
#44136=AXIS2_PLACEMENT_3D ( 'NONE', #49448, #45490, #18144 ) ;
#44140=ORIENTED_EDGE ( 'NONE', *, *, #37813, .F. ) ;
#44141=VERTEX_POINT ( 'NONE', #14351 ) ;
#44142=AXIS2_PLACEMENT_3D ( 'NONE', #4507, #13427, #37331 ) ;
#44144=AXIS2_PLACEMENT_3D ( 'NONE', #7747, #42724, #23777 ) ;
#44145=FACE_OUTER_BOUND ( 'NONE', #31074, .T. ) ;
#44147=DIRECTION ( 'NONE',  ( 0.000000000000000000, -1.000000000000000000, 0.000000000000000000 ) ) ;
#44148=VERTEX_POINT ( 'NONE', #10142 ) ;
#44149=EDGE_CURVE ( 'NONE', #24862, #19780, #14607, .T. ) ;
#44152=EDGE_CURVE ( 'NONE', #14246, #10133, #36204, .T. ) ;
#44153=ORIENTED_EDGE ( 'NONE', *, *, #24481, .T. ) ;
#44154=ORIENTED_EDGE ( 'NONE', *, *, #31335, .T. ) ;
#44156=AXIS2_PLACEMENT_3D ( 'NONE', #19213, #18943, #11298 ) ;
#44158=CARTESIAN_POINT ( 'NONE',  ( 63.10841233855954613, -189.7472609257535510, -54.07611884703302962 ) ) ;
#44159=CIRCLE ( 'NONE', #1363, 125.0000000000000000 ) ;
#44161=ADVANCED_FACE ( 'NONE', ( #38251 ), #18301, .T. ) ;
#44164=EDGE_CURVE ( 'NONE', #4631, #43537, #22792, .T. ) ;
#44165=CARTESIAN_POINT ( 'NONE',  ( 70.19984492582109681, -193.5000000000000000, 39.24667733211968823 ) ) ;
#44167=DIRECTION ( 'NONE',  ( 0.000000000000000000, 0.000000000000000000, 1.000000000000000000 ) ) ;
#44169=EDGE_LOOP ( 'NONE', ( #25772, #15116, #12491, #43670 ) ) ;
#44170=AXIS2_PLACEMENT_3D ( 'NONE', #37974, #10378, #50595 ) ;
#44173=VECTOR ( 'NONE', #49130, 1000.000000000000000 ) ;
#44176=ORIENTED_EDGE ( 'NONE', *, *, #42993, .F. ) ;
#44178=ORIENTED_EDGE ( 'NONE', *, *, #13204, .F. ) ;
#44179=DIRECTION ( 'NONE',  ( -0.000000000000000000, 1.000000000000000000, 0.000000000000000000 ) ) ;
#44183=CYLINDRICAL_SURFACE ( 'NONE', #29878, 125.0000000000000000 ) ;
#44185=AXIS2_PLACEMENT_3D ( 'NONE', #22918, #27101, #43138 ) ;
#44186=CARTESIAN_POINT ( 'NONE',  ( -172.3334410065085933, -183.6283474603465606, -6.025661128238047226 ) ) ;
#44187=CARTESIAN_POINT ( 'NONE',  ( 5.015379008610418410, -193.5000000000000000, -112.9749434763326690 ) ) ;
#44190=LINE ( 'NONE', #24468, #24950 ) ;
#44191=DIRECTION ( 'NONE',  ( 0.000000000000000000, 0.000000000000000000, 1.000000000000000000 ) ) ;
#44192=DIRECTION ( 'NONE',  ( 0.000000000000000000, 1.000000000000000000, 0.000000000000000000 ) ) ;
#44193=VERTEX_POINT ( 'NONE', #47958 ) ;
#44194=DIRECTION ( 'NONE',  ( 0.9151456172430210145, 0.000000000000000000, -0.4031234292879665171 ) ) ;
#44196=ORIENTED_EDGE ( 'NONE', *, *, #6562, .T. ) ;
#44198=EDGE_LOOP ( 'NONE', ( #652, #45061, #26555, #50839 ) ) ;
#44199=VECTOR ( 'NONE', #36119, 1000.000000000000000 ) ;
#44200=VECTOR ( 'NONE', #36312, 1000.000000000000000 ) ;
#44202=CARTESIAN_POINT ( 'NONE',  ( 69.88207517204678254, -193.5000000000000000, 40.19484891390058579 ) ) ;
#44203=AXIS2_PLACEMENT_3D ( 'NONE', #32871, #28926, #9495 ) ;
#44205=FACE_OUTER_BOUND ( 'NONE', #22495, .T. ) ;
#44209=VECTOR ( 'NONE', #23390, 1000.000000000000000 ) ;
#44210=PLANE ( 'NONE',  #8528 ) ;
#44213=ORIENTED_EDGE ( 'NONE', *, *, #3170, .T. ) ;
#44214=CIRCLE ( 'NONE', #34982, 125.0000000000000000 ) ;
#44215=AXIS2_PLACEMENT_3D ( 'NONE', #6905, #19499, #38947 ) ;
#44216=ORIENTED_EDGE ( 'NONE', *, *, #38802, .F. ) ;
#44217=EDGE_CURVE ( 'NONE', #23438, #18322, #8271, .T. ) ;
#44222=DIRECTION ( 'NONE',  ( -0.000000000000000000, 1.000000000000000000, -0.000000000000000000 ) ) ;
#44224=ORIENTED_EDGE ( 'NONE', *, *, #26037, .F. ) ;
#44225=EDGE_LOOP ( 'NONE', ( #24832, #11535, #4608, #15191 ) ) ;
#44227=EDGE_CURVE ( 'NONE', #47448, #10566, #11167, .T. ) ;
#44228=EDGE_CURVE ( 'NONE', #40758, #38078, #3298, .T. ) ;
#44229=CARTESIAN_POINT ( 'NONE',  ( 42.45000882818163035, -175.3837268820161057, -84.30834960112932208 ) ) ;
#44230=DIRECTION ( 'NONE',  ( 0.000000000000000000, -1.000000000000000000, -0.000000000000000000 ) ) ;
#44232=VERTEX_POINT ( 'NONE', #15650 ) ;
#44235=DIRECTION ( 'NONE',  ( 0.6965510290629982615, 0.000000000000000000, -0.7175072570443298270 ) ) ;
#44236=CARTESIAN_POINT ( 'NONE',  ( -96.30460367372252506, -183.6283474603465606, -114.4068333132746176 ) ) ;
#44237=VECTOR ( 'NONE', #2560, 1000.000000000000000 ) ;
#44238=CARTESIAN_POINT ( 'NONE',  ( 38.46761263173351608, -175.3837268820161057, 89.80681772907068705 ) ) ;
#44239=CIRCLE ( 'NONE', #43421, 125.0000000000000000 ) ;
#44240=ADVANCED_FACE ( 'NONE', ( #35343 ), #43228, .T. ) ;
#44242=LINE ( 'NONE', #35562, #33975 ) ;
#44243=ORIENTED_EDGE ( 'NONE', *, *, #32952, .T. ) ;
#44244=CARTESIAN_POINT ( 'NONE',  ( 33.25242634436024503, -175.3837268820161057, -94.57776286494160445 ) ) ;
#44245=CIRCLE ( 'NONE', #21601, 125.0000000000000000 ) ;
#44246=EDGE_CURVE ( 'NONE', #49764, #33603, #42926, .T. ) ;
#44249=DIRECTION ( 'NONE',  ( -0.8455960035018272869, 0.000000000000000000, 0.5338233779647886257 ) ) ;
#44250=VERTEX_POINT ( 'NONE', #116 ) ;
#44251=ORIENTED_EDGE ( 'NONE', *, *, #32344, .F. ) ;
#44253=ORIENTED_EDGE ( 'NONE', *, *, #8160, .F. ) ;
#44254=CARTESIAN_POINT ( 'NONE',  ( -27.36201831380532923, -189.7472609257535510, -122.1886788576022411 ) ) ;
#44257=ORIENTED_EDGE ( 'NONE', *, *, #11832, .T. ) ;
#44260=CARTESIAN_POINT ( 'NONE',  ( 76.21810084846656252, -183.6283474603465606, -8.694908215727984668 ) ) ;
#44261=VERTEX_POINT ( 'NONE', #51397 ) ;
#44263=CIRCLE ( 'NONE', #26630, 125.0000000000000000 ) ;
#44264=AXIS2_PLACEMENT_3D ( 'NONE', #42353, #30274, #46574 ) ;
#44265=ORIENTED_EDGE ( 'NONE', *, *, #8027, .T. ) ;
#44266=DIRECTION ( 'NONE',  ( -0.7765238627180349740, 0.000000000000000000, -0.6300878435817203194 ) ) ;
#44267=ORIENTED_EDGE ( 'NONE', *, *, #51887, .T. ) ;
#44268=DIRECTION ( 'NONE',  ( 0.2635871660690715101, 0.000000000000000000, -0.9646355819083576311 ) ) ;
#44269=FACE_BOUND ( 'NONE', #4945, .T. ) ;
#44270=DIRECTION ( 'NONE',  ( -0.9785564922995032555, 0.000000000000000000, -0.2059786187411021818 ) ) ;
#44273=CARTESIAN_POINT ( 'NONE',  ( -115.4536696835168357, -183.6283474603465606, -105.5434062319793611 ) ) ;
#44274=DIRECTION ( 'NONE',  ( 0.000000000000000000, -1.000000000000000000, 0.000000000000000000 ) ) ;
#44275=FACE_OUTER_BOUND ( 'NONE', #7701, .T. ) ;
#44277=DIRECTION ( 'NONE',  ( 0.000000000000000000, 1.000000000000000000, 0.000000000000000000 ) ) ;
#44278=EDGE_LOOP ( 'NONE', ( #28948, #2272, #5477, #23825 ) ) ;
#44280=ORIENTED_EDGE ( 'NONE', *, *, #39759, .T. ) ;
#44281=AXIS2_PLACEMENT_3D ( 'NONE', #25129, #41400, #41143 ) ;
#44282=AXIS2_PLACEMENT_3D ( 'NONE', #22016, #1263, #25961 ) ;
#44283=CARTESIAN_POINT ( 'NONE',  ( 141.7825277784304205, -193.5000000000000000, 10.00000000000000178 ) ) ;
#44284=FACE_OUTER_BOUND ( 'NONE', #47337, .T. ) ;
#44285=ORIENTED_EDGE ( 'NONE', *, *, #17612, .F. ) ;
#44287=EDGE_CURVE ( 'NONE', #7639, #12625, #31919, .T. ) ;
#44289=EDGE_LOOP ( 'NONE', ( #4575, #8014, #31303, #36502 ) ) ;
#44291=CARTESIAN_POINT ( 'NONE',  ( -47.49008656418669005, -183.6283474603465606, 0.1476465640024920423 ) ) ;
#44293=EDGE_CURVE ( 'NONE', #29270, #27177, #16941, .T. ) ;
#44294=DIRECTION ( 'NONE',  ( 0.000000000000000000, 1.000000000000000000, 0.000000000000000000 ) ) ;
#44296=ORIENTED_EDGE ( 'NONE', *, *, #42312, .T. ) ;
#44298=EDGE_CURVE ( 'NONE', #40001, #24499, #29530, .T. ) ;
#44299=CARTESIAN_POINT ( 'NONE',  ( -48.71401279728982558, -189.7472609257535510, -0.9720229140804069745 ) ) ;
#44300=ORIENTED_EDGE ( 'NONE', *, *, #22816, .T. ) ;
#44302=FACE_OUTER_BOUND ( 'NONE', #21146, .T. ) ;
#44303=CIRCLE ( 'NONE', #12394, 125.0000000000000000 ) ;
#44304=ADVANCED_FACE ( 'NONE', ( #24552 ), #1424, .T. ) ;
#44306=DIRECTION ( 'NONE',  ( 0.9929810960135178055, 0.000000000000000000, -0.1182731709213592358 ) ) ;
#44307=ORIENTED_EDGE ( 'NONE', *, *, #243, .F. ) ;
#44308=ORIENTED_EDGE ( 'NONE', *, *, #12778, .T. ) ;
#44309=ADVANCED_FACE ( 'NONE', ( #5377 ), #32949, .T. ) ;
#44310=EDGE_LOOP ( 'NONE', ( #31320, #30989, #29324, #2441 ) ) ;
#44311=CIRCLE ( 'NONE', #20821, 125.0000000000000000 ) ;
#44312=CARTESIAN_POINT ( 'NONE',  ( -48.47912675150885065, -177.1207230881787780, 6.938893903907228378E-15 ) ) ;
#44315=CARTESIAN_POINT ( 'NONE',  ( -111.8989814360438686, -189.7472609257535510, -107.7168604805787169 ) ) ;
#44318=ORIENTED_EDGE ( 'NONE', *, *, #27781, .T. ) ;
#44319=EDGE_CURVE ( 'NONE', #12735, #4174, #32443, .T. ) ;
#44321=ORIENTED_EDGE ( 'NONE', *, *, #17300, .T. ) ;
#44325=VECTOR ( 'NONE', #50282, 1000.000000000000114 ) ;
#44327=CIRCLE ( 'NONE', #15816, 125.0000000000000000 ) ;
#44328=LINE ( 'NONE', #8316, #41722 ) ;
#44329=CARTESIAN_POINT ( 'NONE',  ( -47.48307690889363641, -189.7472609257535510, -0.08879589532292464504 ) ) ;
#44330=VECTOR ( 'NONE', #32900, 1000.000000000000000 ) ;
#44332=DIRECTION ( 'NONE',  ( -0.1182731709213730997, 0.000000000000000000, 0.9929810960135161402 ) ) ;
#44333=ORIENTED_EDGE ( 'NONE', *, *, #4867, .F. ) ;
#44335=VERTEX_POINT ( 'NONE', #21392 ) ;
#44336=EDGE_CURVE ( 'NONE', #32514, #47785, #33494, .T. ) ;
#44337=EDGE_CURVE ( 'NONE', #12908, #49461, #22001, .T. ) ;
#44339=DIRECTION ( 'NONE',  ( -0.000000000000000000, 1.000000000000000000, -0.000000000000000000 ) ) ;
#44340=AXIS2_PLACEMENT_3D ( 'NONE', #19292, #4030, #20048 ) ;
#44341=CARTESIAN_POINT ( 'NONE',  ( -50.89116676070555911, -183.6283474603465606, 124.9767260852757147 ) ) ;
#44342=DIRECTION ( 'NONE',  ( 0.000000000000000000, -0.000000000000000000, 1.000000000000000000 ) ) ;
#44343=CARTESIAN_POINT ( 'NONE',  ( 68.79964045138289919, -193.5000000000000000, 43.25148278810711133 ) ) ;
#44344=CARTESIAN_POINT ( 'NONE',  ( -0.3054481938615516423, -183.6283474603465606, 115.3442529744090450 ) ) ;
#44345=VERTEX_POINT ( 'NONE', #894 ) ;
#44346=DIRECTION ( 'NONE',  ( 0.7765238627180393038, 0.000000000000000000, 0.6300878435817147682 ) ) ;
#44348=AXIS2_PLACEMENT_3D ( 'NONE', #14463, #10496, #26529 ) ;
#44349=FACE_BOUND ( 'NONE', #39799, .T. ) ;
#44350=ORIENTED_EDGE ( 'NONE', *, *, #140, .T. ) ;
#44353=EDGE_CURVE ( 'NONE', #47028, #17270, #44531, .T. ) ;
#44355=EDGE_CURVE ( 'NONE', #33506, #34708, #8517, .T. ) ;
#44356=DIRECTION ( 'NONE',  ( 0.9473263538541946138, 0.000000000000000000, -0.3202698538628279690 ) ) ;
#44358=EDGE_CURVE ( 'NONE', #42260, #18995, #29536, .T. ) ;
#44361=DIRECTION ( 'NONE',  ( -0.000000000000000000, 1.000000000000000000, -0.000000000000000000 ) ) ;
#44362=CIRCLE ( 'NONE', #21702, 125.0000000000000000 ) ;
#44365=DIRECTION ( 'NONE',  ( -0.000000000000000000, 1.000000000000000000, -0.000000000000000000 ) ) ;
#44367=CARTESIAN_POINT ( 'NONE',  ( -60.80616967713025645, -177.1207230881787780, -123.3865623328508150 ) ) ;
#44369=ORIENTED_EDGE ( 'NONE', *, *, #19463, .T. ) ;
#44370=LINE ( 'NONE', #28048, #36825 ) ;
#44372=ORIENTED_EDGE ( 'NONE', *, *, #51887, .F. ) ;
#44374=DIRECTION ( 'NONE',  ( -0.6300878435817203194, 0.000000000000000000, 0.7765238627180349740 ) ) ;
#44376=ADVANCED_FACE ( 'NONE', ( #16697 ), #12975, .T. ) ;
#44377=VECTOR ( 'NONE', #47490, 1000.000000000000114 ) ;
#44379=DIRECTION ( 'NONE',  ( 0.000000000000000000, 0.000000000000000000, 1.000000000000000000 ) ) ;
#44383=ORIENTED_EDGE ( 'NONE', *, *, #5411, .T. ) ;
#44384=ORIENTED_EDGE ( 'NONE', *, *, #36288, .T. ) ;
#44385=DIRECTION ( 'NONE',  ( 0.9842305779475954974, 0.000000000000000000, 0.1768902751225803205 ) ) ;
#44387=CARTESIAN_POINT ( 'NONE',  ( -49.45768324380835423, -177.1207230881787780, 0.2059786187410958813 ) ) ;
#44389=FACE_OUTER_BOUND ( 'NONE', #7225, .T. ) ;
#44390=DIRECTION ( 'NONE',  ( -0.2920567706369833760, 0.000000000000000000, 0.9564009842765202052 ) ) ;
#44393=DIRECTION ( 'NONE',  ( 0.000000000000000000, -1.000000000000000000, 0.000000000000000000 ) ) ;
#44394=ORIENTED_EDGE ( 'NONE', *, *, #50415, .T. ) ;
#44396=DIRECTION ( 'NONE',  ( 0.000000000000000000, 1.000000000000000000, 0.000000000000000000 ) ) ;
#44397=VECTOR ( 'NONE', #16618, 999.9999999999998863 ) ;
#44399=AXIS2_PLACEMENT_3D ( 'NONE', #40982, #44674, #16292 ) ;
#44400=LINE ( 'NONE', #51502, #12943 ) ;
#44402=CARTESIAN_POINT ( 'NONE',  ( -48.47912675150885065, -183.6283474603465606, 6.938893903907228378E-15 ) ) ;
#44403=AXIS2_PLACEMENT_3D ( 'NONE', #28321, #44374, #16514 ) ;
#44404=DIRECTION ( 'NONE',  ( 0.000000000000000000, 1.000000000000000000, 0.000000000000000000 ) ) ;
#44405=EDGE_LOOP ( 'NONE', ( #23870, #30299, #2293, #29601 ) ) ;
#44407=CARTESIAN_POINT ( 'NONE',  ( -88.49718702276014426, -177.1207230881787780, -117.3655938605927531 ) ) ;
#44409=LINE ( 'NONE', #39912, #47276 ) ;
#44410=VERTEX_POINT ( 'NONE', #32699 ) ;
#44411=VECTOR ( 'NONE', #42989, 1000.000000000000114 ) ;
#44412=LINE ( 'NONE', #31804, #47516 ) ;
#44415=EDGE_LOOP ( 'NONE', ( #45177, #24185, #36649, #15365 ) ) ;
#44416=EDGE_CURVE ( 'NONE', #39427, #9601, #5211, .T. ) ;
#44419=CIRCLE ( 'NONE', #14228, 125.0000000000000000 ) ;
#44420=DIRECTION ( 'NONE',  ( 0.9960498426152158968, 0.000000000000000000, 0.08879589532294571153 ) ) ;
#44421=DIRECTION ( 'NONE',  ( 0.000000000000000000, -1.000000000000000000, 0.000000000000000000 ) ) ;
#44424=VERTEX_POINT ( 'NONE', #49265 ) ;
#44425=CARTESIAN_POINT ( 'NONE',  ( -173.4787860028527007, -177.1207230881787780, 0.2918682030023981300 ) ) ;
#44427=ORIENTED_EDGE ( 'NONE', *, *, #30225, .F. ) ;
#44428=ORIENTED_EDGE ( 'NONE', *, *, #15418, .T. ) ;
#44429=AXIS2_PLACEMENT_3D ( 'NONE', #8530, #11950, #16708 ) ;
#44431=EDGE_CURVE ( 'NONE', #37437, #16495, #49699, .T. ) ;
#44432=PLANE ( 'NONE',  #45205 ) ;
#44433=VECTOR ( 'NONE', #27218, 1000.000000000000000 ) ;
#44434=DIRECTION ( 'NONE',  ( -0.000000000000000000, 1.000000000000000000, -0.000000000000000000 ) ) ;
#44435=DIRECTION ( 'NONE',  ( 0.000000000000000000, 1.000000000000000000, -0.000000000000000000 ) ) ;
#44436=LINE ( 'NONE', #20250, #19099 ) ;
#44437=CARTESIAN_POINT ( 'NONE',  ( -48.30901192927175458, -193.5000000000000000, -124.9998842437354227 ) ) ;
#44440=LINE ( 'NONE', #8426, #50835 ) ;
#44442=DIRECTION ( 'NONE',  ( -0.000000000000000000, 1.000000000000000000, 0.000000000000000000 ) ) ;
#44443=LINE ( 'NONE', #4497, #35005 ) ;
#44444=EDGE_LOOP ( 'NONE', ( #50900, #44989, #10803, #51868 ) ) ;
#44445=CARTESIAN_POINT ( 'NONE',  ( 68.59638248015004081, -177.1207230881787780, -43.79868877201405297 ) ) ;
#44446=ADVANCED_FACE ( 'NONE', ( #39700 ), #35773, .T. ) ;
#44447=PLANE ( 'NONE',  #43476 ) ;
#44448=DIRECTION ( 'NONE',  ( 0.000000000000000000, -0.000000000000000000, 1.000000000000000000 ) ) ;
#44452=CARTESIAN_POINT ( 'NONE',  ( -81.14588623932559130, -177.1207230881787780, 120.6560517527617975 ) ) ;
#44453=CARTESIAN_POINT ( 'NONE',  ( 73.79319191488886531, -183.6283474603465606, 20.63201007055493008 ) ) ;
#44454=ADVANCED_FACE ( 'NONE', ( #37 ), #43919, .F. ) ;
#44456=DIRECTION ( 'NONE',  ( 0.000000000000000000, 0.000000000000000000, 1.000000000000000000 ) ) ;
#44459=DIRECTION ( 'NONE',  ( -1.000000000000000000, 0.000000000000000000, -4.884776371667511665E-16 ) ) ;
#44461=ADVANCED_FACE ( 'NONE', ( #32619 ), #39964, .T. ) ;
#44462=VERTEX_POINT ( 'NONE', #36040 ) ;
#44463=DIRECTION ( 'NONE',  ( 0.000000000000000000, 0.000000000000000000, 1.000000000000000000 ) ) ;
#44464=ORIENTED_EDGE ( 'NONE', *, *, #45256, .F. ) ;
#44466=CARTESIAN_POINT ( 'NONE',  ( -48.93575598890255662, -183.6283474603465606, -0.8896570909947461026 ) ) ;
#44468=FACE_OUTER_BOUND ( 'NONE', #17375, .T. ) ;
#44472=ADVANCED_FACE ( 'NONE', ( #35511 ), #43667, .T. ) ;
#44475=DIRECTION ( 'NONE',  ( -0.4566292373937018145, 0.000000000000000000, -0.8896570909947529859 ) ) ;
#44477=VERTEX_POINT ( 'NONE', #36547 ) ;
#44479=FACE_OUTER_BOUND ( 'NONE', #22997, .T. ) ;
#44484=VERTEX_POINT ( 'NONE', #23686 ) ;
#44486=EDGE_CURVE ( 'NONE', #31562, #3689, #27881, .T. ) ;
#44487=DIRECTION ( 'NONE',  ( -0.1476465640024918202, 0.000000000000000000, 0.9890401873221624784 ) ) ;
#44489=FACE_OUTER_BOUND ( 'NONE', #32855, .T. ) ;
#44490=EDGE_LOOP ( 'NONE', ( #26999, #38359, #10163, #38559 ) ) ;
#44491=ORIENTED_EDGE ( 'NONE', *, *, #5168, .F. ) ;
#44494=DIRECTION ( 'NONE',  ( 0.9960498426152158968, 0.000000000000000000, 0.08879589532294571153 ) ) ;
#44496=ORIENTED_EDGE ( 'NONE', *, *, #6016, .F. ) ;
#44497=AXIS2_PLACEMENT_3D ( 'NONE', #10223, #45996, #26505 ) ;
#44498=LINE ( 'NONE', #28702, #16140 ) ;
#44500=ORIENTED_EDGE ( 'NONE', *, *, #17883, .F. ) ;
#44501=LINE ( 'NONE', #8484, #18804 ) ;
#44503=PLANE ( 'NONE',  #28973 ) ;
#44506=VERTEX_POINT ( 'NONE', #47881 ) ;
#44507=DIRECTION ( 'NONE',  ( 0.000000000000000000, 0.000000000000000000, 1.000000000000000000 ) ) ;
#44508=DIRECTION ( 'NONE',  ( -0.000000000000000000, -1.000000000000000000, 0.000000000000000000 ) ) ;
#44509=ORIENTED_EDGE ( 'NONE', *, *, #5067, .T. ) ;
#44510=PLANE ( 'NONE',  #36636 ) ;
#44511=DIRECTION ( 'NONE',  ( 0.000000000000000000, -0.000000000000000000, -1.000000000000000000 ) ) ;
#44512=EDGE_CURVE ( 'NONE', #2310, #47870, #34555, .T. ) ;
#44513=EDGE_CURVE ( 'NONE', #38668, #10865, #20264, .T. ) ;
#44514=ORIENTED_EDGE ( 'NONE', *, *, #15202, .F. ) ;
#44516=CARTESIAN_POINT ( 'NONE',  ( -48.59739992243020623, -175.3837268820161057, -0.9929810960135115883 ) ) ;
#44517=AXIS2_PLACEMENT_3D ( 'NONE', #22973, #6442, #30082 ) ;
#44520=DIRECTION ( 'NONE',  ( 0.4566292373937200777, 0.000000000000000000, -0.8896570909947436601 ) ) ;
#44521=ORIENTED_EDGE ( 'NONE', *, *, #42030, .T. ) ;
#44523=VERTEX_POINT ( 'NONE', #44453 ) ;
#44524=LINE ( 'NONE', #32693, #1341 ) ;
#44525=PLANE ( 'NONE',  #16341 ) ;
#44529=EDGE_CURVE ( 'NONE', #5680, #33758, #32091, .T. ) ;
#44531=LINE ( 'NONE', #651, #24501 ) ;
#44532=VERTEX_POINT ( 'NONE', #44710 ) ;
#44533=VERTEX_POINT ( 'NONE', #12103 ) ;
#44534=EDGE_CURVE ( 'NONE', #22690, #23646, #41276, .T. ) ;
#44535=AXIS2_PLACEMENT_3D ( 'NONE', #1757, #45928, #33305 ) ;
#44536=LINE ( 'NONE', #8521, #21840 ) ;
#44537=CARTESIAN_POINT ( 'NONE',  ( -146.8460685364478309, -193.5000000000000000, 75.49882471933938177 ) ) ;
#44539=EDGE_CURVE ( 'NONE', #38792, #1503, #51557, .T. ) ;
#44540=ORIENTED_EDGE ( 'NONE', *, *, #25364, .T. ) ;
#44541=DIRECTION ( 'NONE',  ( -0.000000000000000000, 1.000000000000000000, -0.000000000000000000 ) ) ;
#44542=LINE ( 'NONE', #8529, #27089 ) ;
#44544=LINE ( 'NONE', #51662, #12535 ) ;
#44545=EDGE_LOOP ( 'NONE', ( #8099, #33884, #41420, #14361 ) ) ;
#44547=EDGE_LOOP ( 'NONE', ( #22133, #3674, #40461, #29492 ) ) ;
#44548=FACE_OUTER_BOUND ( 'NONE', #20349, .T. ) ;
#44550=CIRCLE ( 'NONE', #32047, 125.0000000000000000 ) ;
#44553=ORIENTED_EDGE ( 'NONE', *, *, #18740, .T. ) ;
#44554=EDGE_LOOP ( 'NONE', ( #8480, #43487, #25081, #11217 ) ) ;
#44557=LINE ( 'NONE', #27488, #21567 ) ;
#44558=LINE ( 'NONE', #5148, #8358 ) ;
#44561=CARTESIAN_POINT ( 'NONE',  ( 43.63512310656542326, -175.3837268820161057, 84.49831343337136502 ) ) ;
#44566=EDGE_LOOP ( 'NONE', ( #40638, #40409, #2557, #16179 ) ) ;
#44568=CARTESIAN_POINT ( 'NONE',  ( 38.71172987070728055, -193.5000000000000000, -89.56983042009262874 ) ) ;
#44569=CARTESIAN_POINT ( 'NONE',  ( -92.16375985330358844, -189.7472609257535510, 117.1181148702521710 ) ) ;
#44571=LINE ( 'NONE', #12514, #38895 ) ;
#44573=EDGE_CURVE ( 'NONE', #15652, #40282, #26028, .T. ) ;
#44575=EDGE_LOOP ( 'NONE', ( #10073, #16208, #25699, #5518 ) ) ;
#44576=DIRECTION ( 'NONE',  ( -0.5586467658036594619, 0.000000000000000000, 0.8294056854501971054 ) ) ;
#44579=VERTEX_POINT ( 'NONE', #10016 ) ;
#44580=DIRECTION ( 'NONE',  ( -0.9151456172430237901, 0.000000000000000000, 0.4031234292879600778 ) ) ;
#44582=CARTESIAN_POINT ( 'NONE',  ( -48.93575598890255662, -175.3837268820161057, -0.8896570909947461026 ) ) ;
#44583=DIRECTION ( 'NONE',  ( 0.000000000000000000, 0.000000000000000000, 1.000000000000000000 ) ) ;
#44584=DIRECTION ( 'NONE',  ( 0.000000000000000000, 0.000000000000000000, 1.000000000000000000 ) ) ;
#44585=CARTESIAN_POINT ( 'NONE',  ( -156.7610986364826999, -183.6283474603465606, -62.45009659481510766 ) ) ;
#44586=DIRECTION ( 'NONE',  ( -0.000000000000000000, 1.000000000000000000, -0.000000000000000000 ) ) ;
#44588=ORIENTED_EDGE ( 'NONE', *, *, #40693, .T. ) ;
#44589=CARTESIAN_POINT ( 'NONE',  ( -48.47912675150885065, -189.7472609257535510, 6.938893903907228378E-15 ) ) ;
#44590=CARTESIAN_POINT ( 'NONE',  ( -40.90423906728906900, -189.7472609257535510, -124.7702732086912505 ) ) ;
#44591=EDGE_CURVE ( 'NONE', #37488, #34495, #33414, .T. ) ;
#44592=AXIS2_PLACEMENT_3D ( 'NONE', #23586, #39088, #39600 ) ;
#44594=FACE_BOUND ( 'NONE', #49082, .T. ) ;
#44595=EDGE_LOOP ( 'NONE', ( #5621, #22712, #7984, #24505 ) ) ;
#44596=ADVANCED_FACE ( 'NONE', ( #29704 ), #9744, .T. ) ;
#44598=FACE_OUTER_BOUND ( 'NONE', #31618, .T. ) ;
#44599=EDGE_LOOP ( 'NONE', ( #19859, #50881, #9318, #14354 ) ) ;
#44601=EDGE_CURVE ( 'NONE', #4155, #16698, #12753, .T. ) ;
#44603=LINE ( 'NONE', #23846, #38035 ) ;
#44604=ORIENTED_EDGE ( 'NONE', *, *, #33529, .F. ) ;
#44606=CARTESIAN_POINT ( 'NONE',  ( -48.47912675150885065, -189.7472609257535510, 6.938893903907228378E-15 ) ) ;
#44608=FACE_BOUND ( 'NONE', #26881, .T. ) ;
#44609=DIRECTION ( 'NONE',  ( 0.000000000000000000, 0.000000000000000000, -1.000000000000000000 ) ) ;
#44611=CARTESIAN_POINT ( 'NONE',  ( -213.8817838414232426, -213.5000000000000000, 10.00000000000002842 ) ) ;
#44612=EDGE_CURVE ( 'NONE', #39243, #26852, #9234, .T. ) ;
#44615=DIRECTION ( 'NONE',  ( 0.000000000000000000, -0.000000000000000000, 1.000000000000000000 ) ) ;
#44616=VERTEX_POINT ( 'NONE', #33129 ) ;
#44617=LINE ( 'NONE', #49608, #25928 ) ;
#44619=DIRECTION ( 'NONE',  ( 0.000000000000000000, -1.000000000000000000, 0.000000000000000000 ) ) ;
#44620=VECTOR ( 'NONE', #4325, 1000.000000000000000 ) ;
#44621=AXIS2_PLACEMENT_3D ( 'NONE', #43739, #19064, #31136 ) ;
#44623=LINE ( 'NONE', #28836, #29268 ) ;
#44624=EDGE_CURVE ( 'NONE', #16474, #31485, #5555, .T. ) ;
#44626=ORIENTED_EDGE ( 'NONE', *, *, #24697, .T. ) ;
#44627=DIRECTION ( 'NONE',  ( -0.7378332790417285736, 0.000000000000000000, 0.6749830015182091136 ) ) ;
#44628=CARTESIAN_POINT ( 'NONE',  ( -172.7479958471414250, -177.1207230881787780, -13.49993235881364129 ) ) ;
#44629=ORIENTED_EDGE ( 'NONE', *, *, #6815, .T. ) ;
#44630=ORIENTED_EDGE ( 'NONE', *, *, #39358, .T. ) ;
#44631=DIRECTION ( 'NONE',  ( 0.000000000000000000, 0.000000000000000000, 1.000000000000000000 ) ) ;
#44632=ORIENTED_EDGE ( 'NONE', *, *, #31630, .F. ) ;
#44636=DIRECTION ( 'NONE',  ( -0.2348860457809842095, 0.000000000000000000, 0.9720229140804107493 ) ) ;
#44637=ADVANCED_FACE ( 'NONE', ( #1610, #13175, #25256, #48919 ), #17892, .F. ) ;
#44638=DIRECTION ( 'NONE',  ( 0.000000000000000000, 0.000000000000000000, 1.000000000000000000 ) ) ;
#44639=ORIENTED_EDGE ( 'NONE', *, *, #11473, .T. ) ;
#44641=DIRECTION ( 'NONE',  ( 0.000000000000000000, 0.000000000000000000, -1.000000000000000000 ) ) ;
#44644=EDGE_CURVE ( 'NONE', #10381, #9360, #33906, .T. ) ;
#44647=CARTESIAN_POINT ( 'NONE',  ( -171.6469053867624837, -177.1207230881787780, -14.34663989163545850 ) ) ;
#44648=AXIS2_PLACEMENT_3D ( 'NONE', #51412, #31415, #5855 ) ;
#44651=DIRECTION ( 'NONE',  ( 0.000000000000000000, -1.000000000000000000, 0.000000000000000000 ) ) ;
#44656=DIRECTION ( 'NONE',  ( 0.7378332790417285736, 0.000000000000000000, -0.6749830015182091136 ) ) ;
#44657=LINE ( 'NONE', #47831, #19632 ) ;
#44658=PLANE ( 'NONE',  #9730 ) ;
#44659=CARTESIAN_POINT ( 'NONE',  ( 45.24245851652181472, -193.5000000000000000, -81.19354792697731682 ) ) ;
#44660=EDGE_LOOP ( 'NONE', ( #39255, #7903, #38041, #51124 ) ) ;
#44661=VERTEX_POINT ( 'NONE', #2102 ) ;
#44663=EDGE_CURVE ( 'NONE', #33019, #33038, #20298, .T. ) ;
#44665=DIRECTION ( 'NONE',  ( 0.000000000000000000, 0.000000000000000000, -1.000000000000000000 ) ) ;
#44666=EDGE_CURVE ( 'NONE', #21902, #47743, #47045, .T. ) ;
#44667=PLANE ( 'NONE',  #39664 ) ;
#44670=CIRCLE ( 'NONE', #18633, 125.0000000000000000 ) ;
#44671=ORIENTED_EDGE ( 'NONE', *, *, #24050, .F. ) ;
#44673=VECTOR ( 'NONE', #22049, 1000.000000000000227 ) ;
#44674=DIRECTION ( 'NONE',  ( 0.000000000000000000, 1.000000000000000000, 0.000000000000000000 ) ) ;
#44675=CARTESIAN_POINT ( 'NONE',  ( -71.40672220061269115, -193.5000000000000000, -122.8793122007208751 ) ) ;
#44676=DIRECTION ( 'NONE',  ( 0.000000000000000000, -1.000000000000000000, 0.000000000000000000 ) ) ;
#44677=DIRECTION ( 'NONE',  ( 0.000000000000000000, -1.000000000000000000, 0.000000000000000000 ) ) ;
#44678=ORIENTED_EDGE ( 'NONE', *, *, #1245, .T. ) ;
#44679=DIRECTION ( 'NONE',  ( -0.6528221181905280446, 0.000000000000000000, 0.7575112421616145841 ) ) ;
#44680=LINE ( 'NONE', #4478, #50364 ) ;
#44681=VECTOR ( 'NONE', #21339, 1000.000000000000000 ) ;
#44683=CIRCLE ( 'NONE', #19497, 125.0000000000000000 ) ;
#44688=ORIENTED_EDGE ( 'NONE', *, *, #3174, .T. ) ;
#44689=DIRECTION ( 'NONE',  ( 0.000000000000000000, 0.000000000000000000, 1.000000000000000000 ) ) ;
#44693=CARTESIAN_POINT ( 'NONE',  ( -48.47912675150885065, -177.1207230881787780, 6.938893903907228378E-15 ) ) ;
#44694=ORIENTED_EDGE ( 'NONE', *, *, #18794, .T. ) ;
#44697=LINE ( 'NONE', #16854, #3753 ) ;
#44698=VECTOR ( 'NONE', #13887, 1000.000000000000000 ) ;
#44704=DIRECTION ( 'NONE',  ( 0.000000000000000000, -0.000000000000000000, -1.000000000000000000 ) ) ;
#44706=CARTESIAN_POINT ( 'NONE',  ( 61.69163308845453031, -177.1207230881787780, -56.90809649257491287 ) ) ;
#44707=EDGE_LOOP ( 'NONE', ( #11109, #40735, #16508, #36466 ) ) ;
#44709=FACE_OUTER_BOUND ( 'NONE', #48207, .T. ) ;
#44710=CARTESIAN_POINT ( 'NONE',  ( -109.0835867659424565, -177.1207230881787780, -109.3256576763154726 ) ) ;
#44711=CARTESIAN_POINT ( 'NONE',  ( 46.40005841627162653, -177.1207230881787780, 81.38144888055276738 ) ) ;
#44712=ORIENTED_EDGE ( 'NONE', *, *, #46373, .F. ) ;
#44715=DIRECTION ( 'NONE',  ( 0.9027978299657416494, 0.000000000000000000, 0.4300652022765245608 ) ) ;
#44717=AXIS2_PLACEMENT_3D ( 'NONE', #5455, #21473, #37495 ) ;
#44718=PLANE ( 'NONE',  #48292 ) ;
#44719=ORIENTED_EDGE ( 'NONE', *, *, #7346, .T. ) ;
#44720=DIRECTION ( 'NONE',  ( 0.000000000000000000, -1.000000000000000000, -0.000000000000000000 ) ) ;
#44721=ORIENTED_EDGE ( 'NONE', *, *, #45900, .T. ) ;
#44722=AXIS2_PLACEMENT_3D ( 'NONE', #17001, #48277, #24875 ) ;
#44724=CARTESIAN_POINT ( 'NONE',  ( 32.59960422616972409, -189.7472609257535510, -93.82025162277999186 ) ) ;
#44725=FACE_OUTER_BOUND ( 'NONE', #867, .T. ) ;
#44726=ADVANCED_FACE ( 'NONE', ( #10775 ), #18413, .T. ) ;
#44727=FACE_OUTER_BOUND ( 'NONE', #49033, .T. ) ;
#44730=VECTOR ( 'NONE', #41767, 1000.000000000000000 ) ;
#44732=DIRECTION ( 'NONE',  ( -0.3482016354343995812, 0.000000000000000000, 0.9374196611341205632 ) ) ;
#44733=CARTESIAN_POINT ( 'NONE',  ( -49.38192458147459973, -193.5000000000000000, 0.4300652022765185656 ) ) ;
#44735=LINE ( 'NONE', #17144, #21981 ) ;
#44736=VERTEX_POINT ( 'NONE', #6319 ) ;
#44738=ORIENTED_EDGE ( 'NONE', *, *, #27572, .T. ) ;
#44739=PLANE ( 'NONE',  #39213 ) ;
#44740=ADVANCED_FACE ( 'NONE', ( #14470 ), #22083, .T. ) ;
#44741=VECTOR ( 'NONE', #34767, 1000.000000000000114 ) ;
#44743=VERTEX_POINT ( 'NONE', #22613 ) ;
#44744=ORIENTED_EDGE ( 'NONE', *, *, #19532, .F. ) ;
#44746=CARTESIAN_POINT ( 'NONE',  ( -48.47912675150885065, -175.3837268820161057, 6.938893903907228378E-15 ) ) ;
#44747=DIRECTION ( 'NONE',  ( 0.000000000000000000, 0.000000000000000000, 1.000000000000000000 ) ) ;
#44749=VECTOR ( 'NONE', #494, 1000.000000000000000 ) ;
#44750=ORIENTED_EDGE ( 'NONE', *, *, #34059, .F. ) ;
#44754=CARTESIAN_POINT ( 'NONE',  ( -131.8938452225253855, -177.1207230881787780, 93.09664195018558530 ) ) ;
#44755=PLANE ( 'NONE',  #50383 ) ;
#44756=PLANE ( 'NONE',  #7347 ) ;
#44759=DIRECTION ( 'NONE',  ( 0.000000000000000000, -1.000000000000000000, 0.000000000000000000 ) ) ;
#44760=CYLINDRICAL_SURFACE ( 'NONE', #23913, 125.0000000000000000 ) ;
#44763=EDGE_LOOP ( 'NONE', ( #14890, #49445, #31483, #23238 ) ) ;
#44765=AXIS2_PLACEMENT_3D ( 'NONE', #4656, #16230, #19910 ) ;
#44767=EDGE_CURVE ( 'NONE', #49365, #7639, #38882, .T. ) ;
#44768=CARTESIAN_POINT ( 'NONE',  ( -161.4019114581581391, -189.7472609257535510, 53.60452120946272458 ) ) ;
#44769=LINE ( 'NONE', #32674, #8968 ) ;
#44771=ADVANCED_FACE ( 'NONE', ( #10503 ), #2626, .T. ) ;
#44772=ORIENTED_EDGE ( 'NONE', *, *, #7927, .F. ) ;
#44773=DIRECTION ( 'NONE',  ( 0.000000000000000000, -1.000000000000000000, 0.000000000000000000 ) ) ;
#44774=DIRECTION ( 'NONE',  ( 0.000000000000000000, 1.000000000000000000, 0.000000000000000000 ) ) ;
#44775=EDGE_LOOP ( 'NONE', ( #35698, #9416, #43306, #22012 ) ) ;
#44776=CARTESIAN_POINT ( 'NONE',  ( -52.47502265695602119, -177.1207230881787780, -124.9361149384469485 ) ) ;
#44778=DIRECTION ( 'NONE',  ( -0.000000000000000000, 1.000000000000000000, -0.000000000000000000 ) ) ;
#44780=CARTESIAN_POINT ( 'NONE',  ( -105.2524431885210703, -189.7472609257535510, 110.2396968984195382 ) ) ;
#44783=DIRECTION ( 'NONE',  ( -0.000000000000000000, 1.000000000000000000, -0.000000000000000000 ) ) ;
#44785=CARTESIAN_POINT ( 'NONE',  ( -170.7635349987907603, -193.5000000000000000, -25.91377046305877130 ) ) ;
#44786=EDGE_CURVE ( 'NONE', #28153, #34735, #51251, .T. ) ;
#44788=EDGE_CURVE ( 'NONE', #22822, #13519, #46363, .T. ) ;
#44789=DIRECTION ( 'NONE',  ( 0.8757349421956310831, 0.000000000000000000, 0.4827922027307550712 ) ) ;
#44791=DIRECTION ( 'NONE',  ( -0.000000000000000000, 1.000000000000000000, -0.000000000000000000 ) ) ;
#44792=PLANE ( 'NONE',  #29942 ) ;
#44794=CARTESIAN_POINT ( 'NONE',  ( -38.66762320617017679, -183.6283474603465606, -124.6143426664033740 ) ) ;
#44795=EDGE_LOOP ( 'NONE', ( #1132, #25107, #5983, #51295 ) ) ;
#44800=CARTESIAN_POINT ( 'NONE',  ( -47.92047998570520662, -177.1207230881787780, 0.8294056854502119824 ) ) ;
#44801=VERTEX_POINT ( 'NONE', #23624 ) ;
#44803=CARTESIAN_POINT ( 'NONE',  ( -48.77118352214583297, -183.6283474603465606, 0.9564009842765270886 ) ) ;
#44805=ORIENTED_EDGE ( 'NONE', *, *, #11561, .F. ) ;
#44806=DIRECTION ( 'NONE',  ( -0.000000000000000000, 1.000000000000000000, -0.000000000000000000 ) ) ;
#44809=DIRECTION ( 'NONE',  ( 0.000000000000000000, -1.000000000000000000, -0.000000000000000000 ) ) ;
#44811=EDGE_CURVE ( 'NONE', #20535, #9367, #21177, .T. ) ;
#44812=LINE ( 'NONE', #20369, #12666 ) ;
#44816=AXIS2_PLACEMENT_3D ( 'NONE', #44343, #8068, #48276 ) ;
#44817=ORIENTED_EDGE ( 'NONE', *, *, #30459, .F. ) ;
#44818=LINE ( 'NONE', #9856, #23253 ) ;
#44819=DIRECTION ( 'NONE',  ( -0.000000000000000000, 1.000000000000000000, -0.000000000000000000 ) ) ;
#44823=ORIENTED_EDGE ( 'NONE', *, *, #41272, .F. ) ;
#44824=ADVANCED_FACE ( 'NONE', ( #4190 ), #11549, .T. ) ;
#44825=AXIS2_PLACEMENT_3D ( 'NONE', #19929, #44619, #35961 ) ;
#44826=ADVANCED_FACE ( 'NONE', ( #47564 ), #43606, .F. ) ;
#44831=EDGE_CURVE ( 'NONE', #12470, #19399, #16541, .T. ) ;
#44832=CARTESIAN_POINT ( 'NONE',  ( -154.6193097927903182, -175.3837268820161057, -66.02470404298124151 ) ) ;
#44837=EDGE_LOOP ( 'NONE', ( #31557, #25633, #30297, #35142 ) ) ;
#44838=CARTESIAN_POINT ( 'NONE',  ( -154.2693405752510500, -189.7472609257535510, 66.58401203837827609 ) ) ;
#44840=ORIENTED_EDGE ( 'NONE', *, *, #38428, .T. ) ;
#44841=DIRECTION ( 'NONE',  ( 0.000000000000000000, 0.000000000000000000, -1.000000000000000000 ) ) ;
#44843=DIRECTION ( 'NONE',  ( 0.000000000000000000, 0.000000000000000000, 1.000000000000000000 ) ) ;
#44844=AXIS2_PLACEMENT_3D ( 'NONE', #26335, #46325, #22143 ) ;
#44845=LINE ( 'NONE', #32757, #7142 ) ;
#44846=VECTOR ( 'NONE', #50932, 1000.000000000000000 ) ;
#44849=CARTESIAN_POINT ( 'NONE',  ( -124.4642912599203726, -175.3837268820161057, 99.25348746834863789 ) ) ;
#44850=VERTEX_POINT ( 'NONE', #32025 ) ;
#44852=CARTESIAN_POINT ( 'NONE',  ( -169.6464974000608379, -193.5000000000000000, 26.35287080855540154 ) ) ;
#44855=FACE_BOUND ( 'NONE', #2410, .T. ) ;
#44856=ORIENTED_EDGE ( 'NONE', *, *, #12695, .T. ) ;
#44858=ORIENTED_EDGE ( 'NONE', *, *, #45601, .T. ) ;
#44862=VECTOR ( 'NONE', #10891, 1000.000000000000227 ) ;
#44863=ORIENTED_EDGE ( 'NONE', *, *, #20547, .F. ) ;
#44865=PLANE ( 'NONE',  #42738 ) ;
#44868=VERTEX_POINT ( 'NONE', #28075 ) ;
#44870=ADVANCED_FACE ( 'NONE', ( #20461 ), #31508, .F. ) ;
#44871=EDGE_CURVE ( 'NONE', #34929, #20197, #1893, .T. ) ;
#44873=EDGE_LOOP ( 'NONE', ( #41886, #5382, #27244, #36697 ) ) ;
#44874=ADVANCED_FACE ( 'NONE', ( #40174 ), #11793, .T. ) ;
#44876=DIRECTION ( 'NONE',  ( 0.5586467658036476935, 0.000000000000000000, 0.8294056854502049880 ) ) ;
#44877=CARTESIAN_POINT ( 'NONE',  ( -134.9506378406916554, -193.5000000000000000, 90.26448786734091811 ) ) ;
#44878=EDGE_LOOP ( 'NONE', ( #41524, #48367, #29522, #28339 ) ) ;
#44880=ADVANCED_FACE ( 'NONE', ( #43856 ), #7856, .T. ) ;
#44881=VECTOR ( 'NONE', #9221, 1000.000000000000000 ) ;
#44882=CARTESIAN_POINT ( 'NONE',  ( 73.32083127613157103, -193.5000000000000000, 28.10285082451656535 ) ) ;
#44886=AXIS2_PLACEMENT_3D ( 'NONE', #51326, #16097, #32109 ) ;
#44888=CARTESIAN_POINT ( 'NONE',  ( -48.18706998087187543, -175.3837268820161057, -0.9564009842765152092 ) ) ;
#44889=CARTESIAN_POINT ( 'NONE',  ( -44.48323084606168720, -193.5000000000000000, 123.9361149384469769 ) ) ;
#44891=FACE_OUTER_BOUND ( 'NONE', #20950, .T. ) ;
#44892=DIRECTION ( 'NONE',  ( 0.000000000000000000, -1.000000000000000000, 0.000000000000000000 ) ) ;
#44893=ORIENTED_EDGE ( 'NONE', *, *, #35916, .T. ) ;
#44894=ORIENTED_EDGE ( 'NONE', *, *, #20427, .F. ) ;
#44897=LINE ( 'NONE', #32014, #34865 ) ;
#44899=CARTESIAN_POINT ( 'NONE',  ( -137.6740394605055826, -193.5000000000000000, -86.14171647324862136 ) ) ;
#44900=VERTEX_POINT ( 'NONE', #48067 ) ;
#44903=DIRECTION ( 'NONE',  ( 0.000000000000000000, -1.000000000000000000, 0.000000000000000000 ) ) ;
#44906=VECTOR ( 'NONE', #19796, 999.9999999999998863 ) ;
#44908=ORIENTED_EDGE ( 'NONE', *, *, #14112, .F. ) ;
#44909=FACE_OUTER_BOUND ( 'NONE', #40169, .T. ) ;
#44910=FACE_OUTER_BOUND ( 'NONE', #9267, .T. ) ;
#44912=CARTESIAN_POINT ( 'NONE',  ( -48.47912675150885065, -175.3837268820161057, 6.938893903907228378E-15 ) ) ;
#44913=ORIENTED_EDGE ( 'NONE', *, *, #12934, .T. ) ;
#44914=LINE ( 'NONE', #32818, #31441 ) ;
#44916=DIRECTION ( 'NONE',  ( -0.9473263538541899509, 0.000000000000000000, -0.3202698538628415692 ) ) ;
#44918=ADVANCED_FACE ( 'NONE', ( #225 ), #48331, .T. ) ;
#44919=DIRECTION ( 'NONE',  ( 0.05924062789370748011, 0.000000000000000000, 0.9982437317643217956 ) ) ;
#44922=VECTOR ( 'NONE', #1787, 1000.000000000000000 ) ;
#44925=CIRCLE ( 'NONE', #10513, 125.0000000000000000 ) ;
#44926=DIRECTION ( 'NONE',  ( 0.7378332790417285736, 0.000000000000000000, -0.6749830015182091136 ) ) ;
#44927=CARTESIAN_POINT ( 'NONE',  ( 33.25242634436024503, -193.5000000000000000, -94.57776286494160445 ) ) ;
#44929=ORIENTED_EDGE ( 'NONE', *, *, #34011, .F. ) ;
#44932=ADVANCED_FACE ( 'NONE', ( #4975 ), #17581, .T. ) ;
#44934=DIRECTION ( 'NONE',  ( 0.000000000000000000, 0.000000000000000000, 1.000000000000000000 ) ) ;
#44937=LINE ( 'NONE', #8411, #1873 ) ;
#44938=VECTOR ( 'NONE', #42922, 1000.000000000000000 ) ;
#44939=VERTEX_POINT ( 'NONE', #760 ) ;
#44940=EDGE_CURVE ( 'NONE', #39601, #21117, #29572, .T. ) ;
#44943=FACE_OUTER_BOUND ( 'NONE', #11840, .T. ) ;
#44944=ADVANCED_FACE ( 'NONE', ( #41740 ), #45434, .T. ) ;
#44945=AXIS2_PLACEMENT_3D ( 'NONE', #7590, #43073, #51752 ) ;
#44946=DIRECTION ( 'NONE',  ( -0.000000000000000000, 1.000000000000000000, -0.000000000000000000 ) ) ;
#44947=EDGE_LOOP ( 'NONE', ( #15419, #41866, #7106, #9905 ) ) ;
#44950=ORIENTED_EDGE ( 'NONE', *, *, #2650, .T. ) ;
#44951=VECTOR ( 'NONE', #45228, 1000.000000000000114 ) ;
#44954=ADVANCED_FACE ( 'NONE', ( #48861 ), #12836, .T. ) ;
#44955=ADVANCED_FACE ( 'NONE', ( #49381 ), #40678, .F. ) ;
#44956=CARTESIAN_POINT ( 'NONE',  ( -48.47912675150885065, -175.3837268820161057, 6.938893903907228378E-15 ) ) ;
#44957=ADVANCED_FACE ( 'NONE', ( #44909 ), #45692, .T. ) ;
#44958=EDGE_CURVE ( 'NONE', #30858, #28774, #1269, .T. ) ;
#44959=CARTESIAN_POINT ( 'NONE',  ( -47.78257572244586271, -177.1207230881787780, 0.7175072570443418174 ) ) ;
#44964=AXIS2_PLACEMENT_3D ( 'NONE', #4516, #560, #40494 ) ;
#44966=DIRECTION ( 'NONE',  ( -0.000000000000000000, 1.000000000000000000, -0.000000000000000000 ) ) ;
#44968=ORIENTED_EDGE ( 'NONE', *, *, #46430, .F. ) ;
#44969=CARTESIAN_POINT ( 'NONE',  ( 41.41233698655026529, -193.5000000000000000, 86.85922373029363541 ) ) ;
#44970=LINE ( 'NONE', #5288, #28287 ) ;
#44972=VECTOR ( 'NONE', #24234, 1000.000000000000000 ) ;
#44974=LINE ( 'NONE', #24727, #22515 ) ;
#44976=LINE ( 'NONE', #16602, #34050 ) ;
#44979=DIRECTION ( 'NONE',  ( -0.000000000000000000, 1.000000000000000000, -0.000000000000000000 ) ) ;
#44981=CARTESIAN_POINT ( 'NONE',  ( -11.17913199888832843, -175.3837268820161057, 119.3051146910914326 ) ) ;
#44982=VERTEX_POINT ( 'NONE', #44647 ) ;
#44984=FACE_OUTER_BOUND ( 'NONE', #40058, .T. ) ;
#44987=VECTOR ( 'NONE', #34517, 1000.000000000000000 ) ;
#44988=DIRECTION ( 'NONE',  ( -0.000000000000000000, 1.000000000000000000, -0.000000000000000000 ) ) ;
#44989=ORIENTED_EDGE ( 'NONE', *, *, #44353, .F. ) ;
#44990=AXIS2_PLACEMENT_3D ( 'NONE', #49103, #44385, #28062 ) ;
#44991=LINE ( 'NONE', #1862, #13017 ) ;
#44994=LINE ( 'NONE', #41283, #26285 ) ;
#44996=CARTESIAN_POINT ( 'NONE',  ( 66.03142248012326831, -183.6283474603465606, 50.12318939044041599 ) ) ;
#44997=LINE ( 'NONE', #832, #34488 ) ;
#44998=LINE ( 'NONE', #28418, #12615 ) ;
#45000=DIRECTION ( 'NONE',  ( -0.2635871660690648488, 0.000000000000000000, -0.9646355819083595184 ) ) ;
#45004=PLANE ( 'NONE',  #13567 ) ;
#45005=CYLINDRICAL_SURFACE ( 'NONE', #14485, 125.0000000000000000 ) ;
#45008=AXIS2_PLACEMENT_3D ( 'NONE', #24734, #1069, #28919 ) ;
#45011=EDGE_CURVE ( 'NONE', #25286, #42685, #15325, .T. ) ;
#45013=CARTESIAN_POINT ( 'NONE',  ( 73.62243227112291777, -193.5000000000000000, 21.61797988633237821 ) ) ;
#45016=ORIENTED_EDGE ( 'NONE', *, *, #51709, .F. ) ;
#45017=VECTOR ( 'NONE', #20621, 999.9999999999998863 ) ;
#45018=VERTEX_POINT ( 'NONE', #25198 ) ;
#45019=DIRECTION ( 'NONE',  ( 0.08879589532293853671, 0.000000000000000000, -0.9960498426152166740 ) ) ;
#45020=CIRCLE ( 'NONE', #24858, 125.0000000000000000 ) ;
#45021=VECTOR ( 'NONE', #50480, 1000.000000000000000 ) ;
#45023=AXIS2_PLACEMENT_3D ( 'NONE', #25255, #20794, #49453 ) ;
#45024=DIRECTION ( 'NONE',  ( -0.000000000000000000, 1.000000000000000000, -0.000000000000000000 ) ) ;
#45026=VERTEX_POINT ( 'NONE', #2821 ) ;
#45027=AXIS2_PLACEMENT_3D ( 'NONE', #29846, #21967, #46409 ) ;
#45028=PLANE ( 'NONE',  #45359 ) ;
#45029=DIRECTION ( 'NONE',  ( 0.000000000000000000, 0.000000000000000000, 1.000000000000000000 ) ) ;
#45031=EDGE_CURVE ( 'NONE', #33001, #37750, #46463, .T. ) ;
#45032=CYLINDRICAL_SURFACE ( 'NONE', #10485, 10.00000000000000178 ) ;
#45034=LINE ( 'NONE', #9025, #27196 ) ;
#45035=ORIENTED_EDGE ( 'NONE', *, *, #15735, .T. ) ;
#45036=CARTESIAN_POINT ( 'NONE',  ( -166.1003692892502102, -177.1207230881787780, -42.31126686685032467 ) ) ;
#45037=CARTESIAN_POINT ( 'NONE',  ( -74.51199343215203896, -177.1207230881787780, -122.2591094863194598 ) ) ;
#45038=LINE ( 'NONE', #41325, #28234 ) ;
#45039=EDGE_CURVE ( 'NONE', #3419, #30279, #34370, .T. ) ;
#45041=VECTOR ( 'NONE', #16758, 1000.000000000000000 ) ;
#45042=ORIENTED_EDGE ( 'NONE', *, *, #50955, .T. ) ;
#45044=VECTOR ( 'NONE', #46609, 1000.000000000000000 ) ;
#45046=ORIENTED_EDGE ( 'NONE', *, *, #47196, .T. ) ;
#45047=DIRECTION ( 'NONE',  ( 0.000000000000000000, 0.000000000000000000, 1.000000000000000000 ) ) ;
#45048=VECTOR ( 'NONE', #13955, 999.9999999999998863 ) ;
#45049=CARTESIAN_POINT ( 'NONE',  ( -12.76653800058363863, -189.7472609257535510, -119.7898618611245070 ) ) ;
#45050=ORIENTED_EDGE ( 'NONE', *, *, #48097, .T. ) ;
#45051=DIRECTION ( 'NONE',  ( 0.000000000000000000, 0.000000000000000000, 1.000000000000000000 ) ) ;
#45053=EDGE_LOOP ( 'NONE', ( #2854, #3771, #47813, #43726 ) ) ;
#45055=ORIENTED_EDGE ( 'NONE', *, *, #21838, .T. ) ;
#45056=FACE_BOUND ( 'NONE', #24323, .T. ) ;
#45057=AXIS2_PLACEMENT_3D ( 'NONE', #13003, #20914, #13536 ) ;
#45060=CARTESIAN_POINT ( 'NONE',  ( -31.30262293407084329, -183.6283474603465606, -123.8142468240611436 ) ) ;
#45061=ORIENTED_EDGE ( 'NONE', *, *, #41508, .T. ) ;
#45063=AXIS2_PLACEMENT_3D ( 'NONE', #37142, #13247, #36899 ) ;
#45066=CARTESIAN_POINT ( 'NONE',  ( 62.86098202833237281, -177.1207230881787780, 56.81883646197908178 ) ) ;
#45067=VECTOR ( 'NONE', #23300, 1000.000000000000000 ) ;
#45068=DIRECTION ( 'NONE',  ( 0.000000000000000000, 0.000000000000000000, -1.000000000000000000 ) ) ;
#45069=EDGE_LOOP ( 'NONE', ( #12508, #6322, #4235, #18054 ) ) ;
#45070=CARTESIAN_POINT ( 'NONE',  ( 62.59443091842027940, -177.1207230881787780, -57.33816169485140790 ) ) ;
#45071=CIRCLE ( 'NONE', #13127, 125.0000000000000000 ) ;
#45072=ORIENTED_EDGE ( 'NONE', *, *, #42015, .F. ) ;
#45074=LINE ( 'NONE', #23217, #8397 ) ;
#45075=CARTESIAN_POINT ( 'NONE',  ( -48.47912675150885065, -177.1207230881787780, 6.938893903907228378E-15 ) ) ;
#45076=ORIENTED_EDGE ( 'NONE', *, *, #12364, .F. ) ;
#45077=ORIENTED_EDGE ( 'NONE', *, *, #32622, .F. ) ;
#45078=CARTESIAN_POINT ( 'NONE',  ( 72.68824389704327871, -193.5000000000000000, -26.35287080855459507 ) ) ;
#45081=DIRECTION ( 'NONE',  ( -0.9785564922995060311, 0.000000000000000000, 0.2059786187410889424 ) ) ;
#45084=VERTEX_POINT ( 'NONE', #14156 ) ;
#45085=CARTESIAN_POINT ( 'NONE',  ( -48.30901192927175458, -189.7472609257535510, -124.9998842437354227 ) ) ;
#45086=ORIENTED_EDGE ( 'NONE', *, *, #14298, .F. ) ;
#45087=LINE ( 'NONE', #29803, #32541 ) ;
#45089=VECTOR ( 'NONE', #30568, 1000.000000000000000 ) ;
#45093=ORIENTED_EDGE ( 'NONE', *, *, #23689, .T. ) ;
#45094=ORIENTED_EDGE ( 'NONE', *, *, #30513, .T. ) ;
#45095=DIRECTION ( 'NONE',  ( -0.2920567706369833760, 0.000000000000000000, 0.9564009842765202052 ) ) ;
#45097=VECTOR ( 'NONE', #35060, 999.9999999999998863 ) ;
#45098=VECTOR ( 'NONE', #11839, 1000.000000000000000 ) ;
#45099=EDGE_CURVE ( 'NONE', #42685, #46449, #39072, .T. ) ;
#45101=AXIS2_PLACEMENT_3D ( 'NONE', #12626, #15824, #35765 ) ;
#45103=VECTOR ( 'NONE', #42897, 1000.000000000000000 ) ;
#45104=DIRECTION ( 'NONE',  ( 0.000000000000000000, -1.000000000000000000, 0.000000000000000000 ) ) ;
#45107=DIRECTION ( 'NONE',  ( -0.9960498426152177842, 0.000000000000000000, 0.08879589532292482545 ) ) ;
#45108=EDGE_LOOP ( 'NONE', ( #2381, #29063, #40283, #47858 ) ) ;
#45112=CARTESIAN_POINT ( 'NONE',  ( -165.2002711502080672, -183.6283474603465606, 44.73448837594998651 ) ) ;
#45114=DIRECTION ( 'NONE',  ( 0.000000000000000000, -1.000000000000000000, -0.000000000000000000 ) ) ;
#45115=VERTEX_POINT ( 'NONE', #34869 ) ;
#45116=LINE ( 'NONE', #5166, #4026 ) ;
#45117=VERTEX_POINT ( 'NONE', #22278 ) ;
#45120=AXIS2_PLACEMENT_3D ( 'NONE', #26140, #34037, #29314 ) ;
#45121=AXIS2_PLACEMENT_3D ( 'NONE', #23878, #39894, #49112 ) ;
#45124=EDGE_CURVE ( 'NONE', #1095, #19776, #25965, .T. ) ;
#45127=DIRECTION ( 'NONE',  ( -0.000000000000000000, 1.000000000000000000, -0.000000000000000000 ) ) ;
#45128=ORIENTED_EDGE ( 'NONE', *, *, #7699, .F. ) ;
#45129=PLANE ( 'NONE',  #45681 ) ;
#45133=FACE_BOUND ( 'NONE', #47401, .T. ) ;
#45135=VECTOR ( 'NONE', #39803, 1000.000000000000000 ) ;
#45140=CARTESIAN_POINT ( 'NONE',  ( -171.2727421180348415, -177.1207230881787780, 23.38221600314376047 ) ) ;
#45141=VERTEX_POINT ( 'NONE', #29902 ) ;
#45142=DIRECTION ( 'NONE',  ( 0.8858462335218260097, 0.000000000000000000, 0.4639789333096864810 ) ) ;
#45143=EDGE_CURVE ( 'NONE', #30058, #41128, #5998, .T. ) ;
#45144=AXIS2_PLACEMENT_3D ( 'NONE', #11855, #17650, #5300 ) ;
#45145=VERTEX_POINT ( 'NONE', #34616 ) ;
#45148=CARTESIAN_POINT ( 'NONE',  ( -125.5794209599708751, -183.6283474603465606, 97.11716833071891131 ) ) ;
#45149=EDGE_CURVE ( 'NONE', #43478, #40260, #10967, .T. ) ;
#45150=FACE_BOUND ( 'NONE', #30336, .T. ) ;
#45151=DIRECTION ( 'NONE',  ( 0.000000000000000000, 0.000000000000000000, -1.000000000000000000 ) ) ;
#45153=DIRECTION ( 'NONE',  ( 0.000000000000000000, 0.000000000000000000, 1.000000000000000000 ) ) ;
#45154=ORIENTED_EDGE ( 'NONE', *, *, #41769, .F. ) ;
#45156=ORIENTED_EDGE ( 'NONE', *, *, #16489, .T. ) ;
#45157=CARTESIAN_POINT ( 'NONE',  ( -105.7090724259147976, -175.3837268820161057, 111.1293539894142697 ) ) ;
#45160=AXIS2_PLACEMENT_3D ( 'NONE', #2376, #37847, #42047 ) ;
#45161=VERTEX_POINT ( 'NONE', #22801 ) ;
#45163=DIRECTION ( 'NONE',  ( 0.000000000000000000, 0.000000000000000000, 1.000000000000000000 ) ) ;
#45164=CARTESIAN_POINT ( 'NONE',  ( -135.4258661347518000, -189.7472609257535510, -89.80681772907016125 ) ) ;
#45165=LINE ( 'NONE', #45939, #2012 ) ;
#45166=ORIENTED_EDGE ( 'NONE', *, *, #37875, .F. ) ;
#45167=CIRCLE ( 'NONE', #42629, 125.0000000000000000 ) ;
#45171=CARTESIAN_POINT ( 'NONE',  ( -49.17567778057185990, -193.5000000000000000, 0.7175072570443320474 ) ) ;
#45172=FACE_OUTER_BOUND ( 'NONE', #40938, .T. ) ;
#45173=ORIENTED_EDGE ( 'NONE', *, *, #41548, .F. ) ;
#45175=VERTEX_POINT ( 'NONE', #38301 ) ;
#45176=CARTESIAN_POINT ( 'NONE',  ( 57.66105628977221187, -175.3837268820161057, 66.02470404298190942 ) ) ;
#45177=ORIENTED_EDGE ( 'NONE', *, *, #37206, .F. ) ;
#45178=CARTESIAN_POINT ( 'NONE',  ( 76.31829002442924548, -177.1207230881787780, 7.113702696402420145 ) ) ;
#45179=ORIENTED_EDGE ( 'NONE', *, *, #49427, .T. ) ;
#45180=CARTESIAN_POINT ( 'NONE',  ( -36.15208382588832592, -177.1207230881787780, 123.3865623328509145 ) ) ;
#45181=CARTESIAN_POINT ( 'NONE',  ( -172.2804936848317823, -177.1207230881787780, -7.024906801078572016 ) ) ;
#45182=ORIENTED_EDGE ( 'NONE', *, *, #48140, .F. ) ;
#45183=LINE ( 'NONE', #20991, #22498 ) ;
#45184=VERTEX_POINT ( 'NONE', #18085 ) ;
#45186=VERTEX_POINT ( 'NONE', #3080 ) ;
#45188=CARTESIAN_POINT ( 'NONE',  ( -147.6585554144535593, -183.6283474603465606, 76.08180419845380982 ) ) ;
#45189=DIRECTION ( 'NONE',  ( -0.000000000000000000, 1.000000000000000000, 0.000000000000000000 ) ) ;
#45190=PLANE ( 'NONE',  #47572 ) ;
#45191=ORIENTED_EDGE ( 'NONE', *, *, #33007, .T. ) ;
#45196=DIRECTION ( 'NONE',  ( 0.000000000000000000, 0.000000000000000000, 1.000000000000000000 ) ) ;
#45197=PLANE ( 'NONE',  #50545 ) ;
#45199=DIRECTION ( 'NONE',  ( 0.000000000000000000, 0.000000000000000000, -1.000000000000000000 ) ) ;
#45200=DIRECTION ( 'NONE',  ( 0.8757349421956379665, 0.000000000000000000, -0.4827922027307427477 ) ) ;
#45201=VECTOR ( 'NONE', #14014, 1000.000000000000000 ) ;
#45202=VERTEX_POINT ( 'NONE', #2569 ) ;
#45204=VECTOR ( 'NONE', #37836, 1000.000000000000000 ) ;
#45205=AXIS2_PLACEMENT_3D ( 'NONE', #8418, #15809, #24199 ) ;
#45207=CARTESIAN_POINT ( 'NONE',  ( 66.42899531795131907, -177.1207230881787780, 49.20491319441622124 ) ) ;
#45210=EDGE_CURVE ( 'NONE', #43643, #12625, #6258, .T. ) ;
#45211=EDGE_LOOP ( 'NONE', ( #50325, #25007, #49602, #4716 ) ) ;
#45212=EDGE_CURVE ( 'NONE', #23257, #36997, #50663, .T. ) ;
#45213=FACE_OUTER_BOUND ( 'NONE', #22661, .T. ) ;
#45214=EDGE_CURVE ( 'NONE', #20956, #12246, #10712, .T. ) ;
#45215=FACE_OUTER_BOUND ( 'NONE', #35956, .T. ) ;
#45216=DIRECTION ( 'NONE',  ( 0.000000000000000000, -0.000000000000000000, -1.000000000000000000 ) ) ;
#45217=DIRECTION ( 'NONE',  ( 0.000000000000000000, 0.000000000000000000, 1.000000000000000000 ) ) ;
#45218=EDGE_CURVE ( 'NONE', #37576, #43853, #51975, .T. ) ;
#45219=ORIENTED_EDGE ( 'NONE', *, *, #14086, .T. ) ;
#45221=DIRECTION ( 'NONE',  ( 0.000000000000000000, -0.000000000000000000, 1.000000000000000000 ) ) ;
#45222=CIRCLE ( 'NONE', #22555, 125.0000000000000000 ) ;
#45223=DIRECTION ( 'NONE',  ( 0.3202698538628279690, 0.000000000000000000, 0.9473263538541946138 ) ) ;
#45224=ORIENTED_EDGE ( 'NONE', *, *, #17913, .F. ) ;
#45225=DIRECTION ( 'NONE',  ( -0.000000000000000000, -1.000000000000000000, 0.000000000000000000 ) ) ;
#45226=ORIENTED_EDGE ( 'NONE', *, *, #12811, .T. ) ;
#45227=LINE ( 'NONE', #33388, #1557 ) ;
#45228=DIRECTION ( 'NONE',  ( 0.1768902751225733261, 0.000000000000000000, -0.9842305779475966077 ) ) ;
#45234=AXIS2_PLACEMENT_3D ( 'NONE', #41189, #13081, #33046 ) ;
#45236=VERTEX_POINT ( 'NONE', #31450 ) ;
#45239=EDGE_LOOP ( 'NONE', ( #38568, #45860, #22942, #33526 ) ) ;
#45240=CARTESIAN_POINT ( 'NONE',  ( 74.03660210627325000, -189.7472609257535510, -19.12855698118388048 ) ) ;
#45243=EDGE_LOOP ( 'NONE', ( #26747, #33771, #48720, #45915 ) ) ;
#45245=EDGE_CURVE ( 'NONE', #117, #41297, #47498, .T. ) ;
#45246=CIRCLE ( 'NONE', #22579, 125.0000000000000000 ) ;
#45247=DIRECTION ( 'NONE',  ( -0.1182731709213523247, 0.000000000000000000, -0.9929810960135185827 ) ) ;
#45248=DIRECTION ( 'NONE',  ( -0.000000000000000000, 1.000000000000000000, -0.000000000000000000 ) ) ;
#45250=ORIENTED_EDGE ( 'NONE', *, *, #34843, .F. ) ;
#45251=CYLINDRICAL_SURFACE ( 'NONE', #33264, 125.0000000000000000 ) ;
#45252=CARTESIAN_POINT ( 'NONE',  ( -48.47912675150885065, -175.3837268820161057, 6.938893903907228378E-15 ) ) ;
#45253=DIRECTION ( 'NONE',  ( 0.000000000000000000, 0.000000000000000000, -1.000000000000000000 ) ) ;
#45255=EDGE_CURVE ( 'NONE', #11111, #36214, #39340, .T. ) ;
#45256=EDGE_CURVE ( 'NONE', #49289, #11294, #3868, .T. ) ;
#45257=EDGE_LOOP ( 'NONE', ( #9544, #50225, #33065, #11540 ) ) ;
#45258=ADVANCED_FACE ( 'NONE', ( #11990 ), #27514, .T. ) ;
#45262=VECTOR ( 'NONE', #12245, 1000.000000000000000 ) ;
#45263=LINE ( 'NONE', #20534, #43396 ) ;
#45264=EDGE_LOOP ( 'NONE', ( #31872, #44805, #37241, #31480 ) ) ;
#45267=CARTESIAN_POINT ( 'NONE',  ( -72.72541169915515979, -177.1207230881787780, 121.6072260099955429 ) ) ;
#45269=CARTESIAN_POINT ( 'NONE',  ( -163.3872488209693756, -193.5000000000000000, -49.20491319441543254 ) ) ;
#45271=EDGE_CURVE ( 'NONE', #46508, #23360, #51460, .T. ) ;
#45275=DIRECTION ( 'NONE',  ( -0.4566292373937200777, 0.000000000000000000, 0.8896570909947436601 ) ) ;
#45277=VERTEX_POINT ( 'NONE', #7292 ) ;
#45278=EDGE_CURVE ( 'NONE', #3888, #50437, #39584, .T. ) ;
#45279=ORIENTED_EDGE ( 'NONE', *, *, #555, .F. ) ;
#45280=FACE_OUTER_BOUND ( 'NONE', #27965, .T. ) ;
#45281=EDGE_CURVE ( 'NONE', #2342, #7429, #43550, .T. ) ;
#45282=EDGE_CURVE ( 'NONE', #32802, #39370, #47764, .T. ) ;
#45283=DIRECTION ( 'NONE',  ( 0.000000000000000000, 0.000000000000000000, 1.000000000000000000 ) ) ;
#45286=EDGE_LOOP ( 'NONE', ( #27722, #9946, #16826, #11781 ) ) ;
#45287=ORIENTED_EDGE ( 'NONE', *, *, #14673, .T. ) ;
#45289=DIRECTION ( 'NONE',  ( -0.7765238627180437447, 0.000000000000000000, 0.6300878435817094392 ) ) ;
#45290=PLANE ( 'NONE',  #30831 ) ;
#45291=ORIENTED_EDGE ( 'NONE', *, *, #1601, .F. ) ;
#45293=AXIS2_PLACEMENT_3D ( 'NONE', #31129, #47696, #27176 ) ;
#45296=ORIENTED_EDGE ( 'NONE', *, *, #46878, .F. ) ;
#45297=PLANE ( 'NONE',  #42380 ) ;
#45299=PLANE ( 'NONE',  #44844 ) ;
#45302=CARTESIAN_POINT ( 'NONE',  ( -71.40672220061267694, -189.7472609257535510, -122.8793122007208751 ) ) ;
#45304=ORIENTED_EDGE ( 'NONE', *, *, #34825, .F. ) ;
#45305=ORIENTED_EDGE ( 'NONE', *, *, #42917, .T. ) ;
#45306=FACE_OUTER_BOUND ( 'NONE', #2502, .T. ) ;
#45308=VECTOR ( 'NONE', #39029, 1000.000000000000227 ) ;
#45309=ORIENTED_EDGE ( 'NONE', *, *, #35555, .T. ) ;
#45310=CARTESIAN_POINT ( 'NONE',  ( 76.47090317495664635, -175.3837268820161057, -3.534122433557446374 ) ) ;
#45311=VECTOR ( 'NONE', #7405, 1000.000000000000114 ) ;
#45312=EDGE_CURVE ( 'NONE', #22578, #34663, #15181, .T. ) ;
#45313=EDGE_CURVE ( 'NONE', #1806, #18280, #39840, .T. ) ;
#45316=CARTESIAN_POINT ( 'NONE',  ( -129.9529520667707914, -193.5000000000000000, -94.79987230211959570 ) ) ;
#45317=EDGE_CURVE ( 'NONE', #6723, #46797, #49777, .T. ) ;
#45318=ADVANCED_FACE ( 'NONE', ( #27245 ), #9110, .F. ) ;
#45319=VERTEX_POINT ( 'NONE', #36420 ) ;
#45320=PLANE ( 'NONE',  #28225 ) ;
#45323=DIRECTION ( 'NONE',  ( 0.000000000000000000, 1.000000000000000000, -0.000000000000000000 ) ) ;
#45324=ORIENTED_EDGE ( 'NONE', *, *, #47421, .F. ) ;
#45326=CARTESIAN_POINT ( 'NONE',  ( -106.4764934152196645, -213.5000000000000000, 110.7307791902283043 ) ) ;
#45327=CARTESIAN_POINT ( 'NONE',  ( -101.5170032742336446, -193.5000000000000000, 112.0852863853383354 ) ) ;
#45329=AXIS2_PLACEMENT_3D ( 'NONE', #41962, #6505, #22248 ) ;
#45330=ORIENTED_EDGE ( 'NONE', *, *, #14759, .T. ) ;
#45331=CARTESIAN_POINT ( 'NONE',  ( -99.02518858244150124, -189.7472609257535510, 114.3245189510261355 ) ) ;
#45333=EDGE_LOOP ( 'NONE', ( #8619, #33291, #46041, #32465 ) ) ;
#45334=EDGE_CURVE ( 'NONE', #10698, #51182, #29606, .T. ) ;
#45335=CARTESIAN_POINT ( 'NONE',  ( 68.59638248015004081, -177.1207230881787780, -43.79868877201405297 ) ) ;
#45336=CARTESIAN_POINT ( 'NONE',  ( -128.7986236165182561, -175.3837268820161057, 94.47107458416955694 ) ) ;
#45337=ORIENTED_EDGE ( 'NONE', *, *, #33380, .T. ) ;
#45340=ADVANCED_FACE ( 'NONE', ( #8569 ), #1198, .T. ) ;
#45342=VERTEX_POINT ( 'NONE', #420 ) ;
#45343=VECTOR ( 'NONE', #29016, 1000.000000000000000 ) ;
#45344=LINE ( 'NONE', #29545, #424 ) ;
#45345=ORIENTED_EDGE ( 'NONE', *, *, #49903, .T. ) ;
#45347=DIRECTION ( 'NONE',  ( 0.000000000000000000, -1.000000000000000000, 0.000000000000000000 ) ) ;
#45349=LINE ( 'NONE', #9080, #29931 ) ;
#45350=EDGE_LOOP ( 'NONE', ( #35010, #25511, #8096, #42884 ) ) ;
#45351=ORIENTED_EDGE ( 'NONE', *, *, #7569, .T. ) ;
#45352=VERTEX_POINT ( 'NONE', #948 ) ;
#45354=CARTESIAN_POINT ( 'NONE',  ( 71.15591247552653442, -193.5000000000000000, 36.22785377504035154 ) ) ;
#45356=CARTESIAN_POINT ( 'NONE',  ( 48.47907891923915713, -175.3837268820161057, 78.89300572996904748 ) ) ;
#45357=EDGE_LOOP ( 'NONE', ( #454, #42504 ) ) ;
#45359=AXIS2_PLACEMENT_3D ( 'NONE', #9018, #25053, #41060 ) ;
#45360=AXIS2_PLACEMENT_3D ( 'NONE', #26627, #14289, #46353 ) ;
#45364=CYLINDRICAL_SURFACE ( 'NONE', #23813, 125.0000000000000000 ) ;
#45365=ORIENTED_EDGE ( 'NONE', *, *, #18476, .F. ) ;
#45366=CARTESIAN_POINT ( 'NONE',  ( -71.40672220061269115, -189.7472609257535510, -122.8793122007208751 ) ) ;
#45367=DIRECTION ( 'NONE',  ( 0.000000000000000000, 0.000000000000000000, 1.000000000000000000 ) ) ;
#45369=CARTESIAN_POINT ( 'NONE',  ( -169.1033029113419559, -193.5000000000000000, 32.78426643622745473 ) ) ;
#45371=DIRECTION ( 'NONE',  ( -0.4827922027307427477, 0.000000000000000000, -0.8757349421956379665 ) ) ;
#45373=DIRECTION ( 'NONE',  ( -0.8858462335218260097, -0.000000000000000000, 0.4639789333096864810 ) ) ;
#45379=ORIENTED_EDGE ( 'NONE', *, *, #11188, .F. ) ;
#45381=PLANE ( 'NONE',  #12916 ) ;
#45383=DIRECTION ( 'NONE',  ( -0.9842305779475967187, 0.000000000000000000, -0.1768902751225733538 ) ) ;
#45386=CYLINDRICAL_SURFACE ( 'NONE', #9785, 125.0000000000000000 ) ;
#45387=ORIENTED_EDGE ( 'NONE', *, *, #12054, .T. ) ;
#45389=CARTESIAN_POINT ( 'NONE',  ( -106.4764934152197497, -213.5000000000000000, -110.7307791902282759 ) ) ;
#45391=PLANE ( 'NONE',  #50499 ) ;
#45392=ORIENTED_EDGE ( 'NONE', *, *, #43041, .F. ) ;
#45393=CARTESIAN_POINT ( 'NONE',  ( -11.17913199888832487, -189.7472609257535510, 119.3051146910914468 ) ) ;
#45397=VECTOR ( 'NONE', #7873, 1000.000000000000000 ) ;
#45401=ORIENTED_EDGE ( 'NONE', *, *, #36343, .T. ) ;
#45403=FACE_OUTER_BOUND ( 'NONE', #37392, .T. ) ;
#45404=ORIENTED_EDGE ( 'NONE', *, *, #36090, .T. ) ;
#45406=ORIENTED_EDGE ( 'NONE', *, *, #6311, .F. ) ;
#45407=CARTESIAN_POINT ( 'NONE',  ( -47.64924157374594671, -189.7472609257535510, 124.9972451320097377 ) ) ;
#45409=AXIS2_PLACEMENT_3D ( 'NONE', #1443, #17496, #13530 ) ;
#45410=ORIENTED_EDGE ( 'NONE', *, *, #49773, .F. ) ;
#45411=DIRECTION ( 'NONE',  ( -0.000000000000000000, 1.000000000000000000, -0.000000000000000000 ) ) ;
#45412=DIRECTION ( 'NONE',  ( 0.000000000000000000, -1.000000000000000000, 0.000000000000000000 ) ) ;
#45416=DIRECTION ( 'NONE',  ( -0.000000000000000000, 1.000000000000000000, -0.000000000000000000 ) ) ;
#45418=ORIENTED_EDGE ( 'NONE', *, *, #4777, .T. ) ;
#45419=CARTESIAN_POINT ( 'NONE',  ( -40.30502441601360886, -193.5000000000000000, 123.7303097900624920 ) ) ;
#45422=ORIENTED_EDGE ( 'NONE', *, *, #31605, .F. ) ;
#45425=EDGE_LOOP ( 'NONE', ( #18354, #9794, #25389, #45418 ) ) ;
#45426=DIRECTION ( 'NONE',  ( 0.000000000000000000, 0.000000000000000000, -1.000000000000000000 ) ) ;
#45427=ADVANCED_FACE ( 'NONE', ( #32753 ), #1476, .T. ) ;
#45428=CARTESIAN_POINT ( 'NONE',  ( 73.32083127613157103, -183.6283474603465606, 28.10285082451656535 ) ) ;
#45430=LINE ( 'NONE', #37784, #3163 ) ;
#45431=EDGE_LOOP ( 'NONE', ( #46214, #13713, #31751, #36590 ) ) ;
#45432=AXIS2_PLACEMENT_3D ( 'NONE', #27528, #10983, #27007 ) ;
#45433=EDGE_LOOP ( 'NONE', ( #43791, #11201, #2456, #30588 ) ) ;
#45434=PLANE ( 'NONE',  #35453 ) ;
#45435=EDGE_CURVE ( 'NONE', #41297, #35501, #32940, .T. ) ;
#45437=DIRECTION ( 'NONE',  ( 0.000000000000000000, 0.000000000000000000, 1.000000000000000000 ) ) ;
#45438=DIRECTION ( 'NONE',  ( 0.000000000000000000, -1.000000000000000000, 0.000000000000000000 ) ) ;
#45439=ORIENTED_EDGE ( 'NONE', *, *, #41857, .T. ) ;
#45440=PLANE ( 'NONE',  #19805 ) ;
#45441=LINE ( 'NONE', #768, #18841 ) ;
#45442=ADVANCED_FACE ( 'NONE', ( #8830 ), #41410, .T. ) ;
#45446=FACE_OUTER_BOUND ( 'NONE', #42475, .T. ) ;
#45449=ORIENTED_EDGE ( 'NONE', *, *, #10965, .T. ) ;
#45450=VECTOR ( 'NONE', #30015, 1000.000000000000227 ) ;
#45452=DIRECTION ( 'NONE',  ( 0.000000000000000000, 1.000000000000000000, -0.000000000000000000 ) ) ;
#45455=DIRECTION ( 'NONE',  ( 0.9785564922995046988, 0.000000000000000000, -0.2059786187410953262 ) ) ;
#45457=PLANE ( 'NONE',  #18399 ) ;
#45458=CARTESIAN_POINT ( 'NONE',  ( -23.99795575808071035, -193.5000000000000000, -122.5792489240757703 ) ) ;
#45459=DIRECTION ( 'NONE',  ( -0.000000000000000000, 1.000000000000000000, -0.000000000000000000 ) ) ;
#45460=DIRECTION ( 'NONE',  ( 0.9785564922995046988, 0.000000000000000000, -0.2059786187410953262 ) ) ;
#45461=AXIS2_PLACEMENT_3D ( 'NONE', #20611, #45583, #20347 ) ;
#45462=DIRECTION ( 'NONE',  ( 0.000000000000000000, -1.000000000000000000, 0.000000000000000000 ) ) ;
#45464=CARTESIAN_POINT ( 'NONE',  ( -140.0851925571752474, -189.7472609257535510, 83.57229767764225414 ) ) ;
#45465=EDGE_LOOP ( 'NONE', ( #2673, #44671, #21405, #30561 ) ) ;
#45469=CARTESIAN_POINT ( 'NONE',  ( -118.4510020108455137, -175.3837268820161057, 103.5805805771131674 ) ) ;
#45471=CARTESIAN_POINT ( 'NONE',  ( -11.80936624585915418, -193.5000000000000000, -119.5003291395395735 ) ) ;
#45473=ORIENTED_EDGE ( 'NONE', *, *, #48234, .T. ) ;
#45475=AXIS2_PLACEMENT_3D ( 'NONE', #41111, #28490, #40313 ) ;
#45477=DIRECTION ( 'NONE',  ( 0.000000000000000000, 0.000000000000000000, -1.000000000000000000 ) ) ;
#45478=VERTEX_POINT ( 'NONE', #9618 ) ;
#45479=DIRECTION ( 'NONE',  ( -0.000000000000000000, 1.000000000000000000, -0.000000000000000000 ) ) ;
#45480=LINE ( 'NONE', #37594, #24981 ) ;
#45481=ORIENTED_EDGE ( 'NONE', *, *, #8650, .F. ) ;
#45482=VECTOR ( 'NONE', #9924, 1000.000000000000000 ) ;
#45486=VERTEX_POINT ( 'NONE', #25636 ) ;
#45487=ADVANCED_FACE ( 'NONE', ( #37208 ), #5426, .T. ) ;
#45489=LINE ( 'NONE', #32861, #7317 ) ;
#45490=DIRECTION ( 'NONE',  ( -0.000000000000000000, 1.000000000000000000, -0.000000000000000000 ) ) ;
#45491=VERTEX_POINT ( 'NONE', #14600 ) ;
#45492=EDGE_LOOP ( 'NONE', ( #4963, #2558, #43187, #37616 ) ) ;
#45493=EDGE_CURVE ( 'NONE', #42501, #39634, #8644, .T. ) ;
#45495=DIRECTION ( 'NONE',  ( 0.000000000000000000, -1.000000000000000000, 0.000000000000000000 ) ) ;
#45496=EDGE_CURVE ( 'NONE', #1315, #18280, #26928, .T. ) ;
#45497=DIRECTION ( 'NONE',  ( 0.9473263538541923934, 0.000000000000000000, -0.3202698538628350744 ) ) ;
#45499=CARTESIAN_POINT ( 'NONE',  ( -172.2424017797220870, -183.6283474603465606, 7.666780576875855679 ) ) ;
#45502=AXIS2_PLACEMENT_3D ( 'NONE', #22341, #7095, #34176 ) ;
#45504=ORIENTED_EDGE ( 'NONE', *, *, #39173, .T. ) ;
#45505=VECTOR ( 'NONE', #50295, 999.9999999999998863 ) ;
#45506=DIRECTION ( 'NONE',  ( -0.9646355819083576311, 0.000000000000000000, -0.2635871660690715101 ) ) ;
#45507=FACE_OUTER_BOUND ( 'NONE', #38052, .T. ) ;
#45508=VECTOR ( 'NONE', #16884, 1000.000000000000114 ) ;
#45509=CARTESIAN_POINT ( 'NONE',  ( -29.73468717939733708, -177.1207230881787780, 123.5865930638410930 ) ) ;
#45510=ORIENTED_EDGE ( 'NONE', *, *, #11556, .F. ) ;
#45511=CARTESIAN_POINT ( 'NONE',  ( -49.38192458147459973, -189.7472609257535510, 0.4300652022765185656 ) ) ;
#45512=CYLINDRICAL_SURFACE ( 'NONE', #26087, 125.0000000000000000 ) ;
#45514=PLANE ( 'NONE',  #14052 ) ;
#45516=CARTESIAN_POINT ( 'NONE',  ( 70.98542830588607444, -177.1207230881787780, -36.78613984829961936 ) ) ;
#45518=AXIS2_PLACEMENT_3D ( 'NONE', #11135, #48708, #20059 ) ;
#45520=DIRECTION ( 'NONE',  ( -0.000000000000000000, 1.000000000000000000, -0.000000000000000000 ) ) ;
#45521=DIRECTION ( 'NONE',  ( 0.000000000000000000, -0.000000000000000000, 1.000000000000000000 ) ) ;
#45522=ORIENTED_EDGE ( 'NONE', *, *, #48210, .T. ) ;
#45524=DIRECTION ( 'NONE',  ( -0.000000000000000000, 1.000000000000000000, -0.000000000000000000 ) ) ;
#45525=DIRECTION ( 'NONE',  ( -0.6749830015182091136, 0.000000000000000000, -0.7378332790417285736 ) ) ;
#45526=CARTESIAN_POINT ( 'NONE',  ( -34.51936650669028239, -193.5000000000000000, -124.2180546213278092 ) ) ;
#45527=EDGE_LOOP ( 'NONE', ( #21367, #41516, #4071, #50998 ) ) ;
#45528=EDGE_LOOP ( 'NONE', ( #26835, #32152, #31673, #17873 ) ) ;
#45529=ORIENTED_EDGE ( 'NONE', *, *, #30401, .F. ) ;
#45530=CARTESIAN_POINT ( 'NONE',  ( -173.3294908491238004, -193.5000000000000000, -6.114457023560960991 ) ) ;
#45531=ADVANCED_FACE ( 'NONE', ( #46932 ), #25905, .T. ) ;
#45532=ADVANCED_FACE ( 'NONE', ( #46660 ), #38239, .F. ) ;
#45533=EDGE_CURVE ( 'NONE', #32182, #16051, #30884, .T. ) ;
#45534=LINE ( 'NONE', #9525, #8509 ) ;
#45537=ADVANCED_FACE ( 'NONE', ( #45890 ), #10912, .T. ) ;
#45538=CIRCLE ( 'NONE', #18707, 125.0000000000000568 ) ;
#45539=LINE ( 'NONE', #48446, #24374 ) ;
#45541=ORIENTED_EDGE ( 'NONE', *, *, #31579, .T. ) ;
#45543=ADVANCED_FACE ( 'NONE', ( #10134 ), #38511, .F. ) ;
#45544=CARTESIAN_POINT ( 'NONE',  ( -48.82732838694323618, -183.6283474603465606, -0.9374196611341184537 ) ) ;
#45548=CARTESIAN_POINT ( 'NONE',  ( 65.38692482895589819, -183.6283474603465606, -51.57055649762702387 ) ) ;
#45549=EDGE_CURVE ( 'NONE', #45874, #24651, #2508, .T. ) ;
#45550=LINE ( 'NONE', #44768, #285 ) ;
#45552=AXIS2_PLACEMENT_3D ( 'NONE', #29935, #1034, #45217 ) ;
#45553=CIRCLE ( 'NONE', #25401, 125.0000000000000000 ) ;
#45555=ORIENTED_EDGE ( 'NONE', *, *, #39764, .F. ) ;
#45556=VECTOR ( 'NONE', #11488, 1000.000000000000114 ) ;
#45557=ORIENTED_EDGE ( 'NONE', *, *, #34960, .T. ) ;
#45558=VECTOR ( 'NONE', #17717, 1000.000000000000114 ) ;
#45560=ADVANCED_FACE ( 'NONE', ( #22217 ), #37733, .T. ) ;
#45562=ORIENTED_EDGE ( 'NONE', *, *, #42983, .F. ) ;
#45563=CARTESIAN_POINT ( 'NONE',  ( -170.0502155641509319, -177.1207230881787780, -29.07697310430877735 ) ) ;
#45565=EDGE_LOOP ( 'NONE', ( #31271, #18810, #46910, #51588 ) ) ;
#45566=CARTESIAN_POINT ( 'NONE',  ( 61.06976976088562026, -193.5000000000000000, -60.19999396110170409 ) ) ;
#45567=VECTOR ( 'NONE', #23348, 1000.000000000000114 ) ;
#45569=VERTEX_POINT ( 'NONE', #34551 ) ;
#45570=CARTESIAN_POINT ( 'NONE',  ( -109.0835867659423712, -183.6283474603465606, -109.3256576763155294 ) ) ;
#45571=ORIENTED_EDGE ( 'NONE', *, *, #40051, .F. ) ;
#45572=DIRECTION ( 'NONE',  ( 0.000000000000000000, -1.000000000000000000, 0.000000000000000000 ) ) ;
#45573=CARTESIAN_POINT ( 'NONE',  ( -47.60339180931321579, -177.1207230881787780, -0.4827922027307358088 ) ) ;
#45574=ORIENTED_EDGE ( 'NONE', *, *, #31088, .T. ) ;
#45576=DIRECTION ( 'NONE',  ( 0.000000000000000000, 0.000000000000000000, 1.000000000000000000 ) ) ;
#45577=CARTESIAN_POINT ( 'NONE',  ( 76.52053249983504202, -193.5000000000000000, -0.2918682030015403162 ) ) ;
#45578=CARTESIAN_POINT ( 'NONE',  ( -147.6585554144535024, -193.5000000000000000, 76.08180419845385245 ) ) ;
#45579=DIRECTION ( 'NONE',  ( -0.000000000000000000, -1.000000000000000000, 0.000000000000000000 ) ) ;
#45580=ADVANCED_FACE ( 'NONE', ( #50603 ), #10654, .T. ) ;
#45581=AXIS2_PLACEMENT_3D ( 'NONE', #10614, #26643, #50564 ) ;
#45583=DIRECTION ( 'NONE',  ( 0.000000000000000000, -1.000000000000000000, 0.000000000000000000 ) ) ;
#45589=ORIENTED_EDGE ( 'NONE', *, *, #35540, .T. ) ;
#45590=DIRECTION ( 'NONE',  ( -0.000000000000000000, 1.000000000000000000, -0.000000000000000000 ) ) ;
#45591=AXIS2_PLACEMENT_3D ( 'NONE', #18679, #11031, #51511 ) ;
#45592=AXIS2_PLACEMENT_3D ( 'NONE', #3368, #31217, #26766 ) ;
#45594=DIRECTION ( 'NONE',  ( 0.000000000000000000, 0.000000000000000000, 1.000000000000000000 ) ) ;
#45595=AXIS2_PLACEMENT_3D ( 'NONE', #28422, #5317, #576 ) ;
#45596=ORIENTED_EDGE ( 'NONE', *, *, #49139, .T. ) ;
#45597=CARTESIAN_POINT ( 'NONE',  ( -22.44626007086656116, -177.1207230881787780, 122.2591094863196872 ) ) ;
#45598=EDGE_LOOP ( 'NONE', ( #4330, #37362, #39922, #18955 ) ) ;
#45600=CARTESIAN_POINT ( 'NONE',  ( -91.81555821786915317, -193.5000000000000000, 116.1806952091180563 ) ) ;
#45601=EDGE_CURVE ( 'NONE', #39890, #42685, #22738, .T. ) ;
#45602=EDGE_CURVE ( 'NONE', #9008, #36633, #105, .T. ) ;
#45603=EDGE_CURVE ( 'NONE', #172, #19493, #230, .T. ) ;
#45604=AXIS2_PLACEMENT_3D ( 'NONE', #967, #36974, #10670 ) ;
#45605=CARTESIAN_POINT ( 'NONE',  ( -161.2555905272864436, -175.3837268820161057, -53.91167979418489864 ) ) ;
#45606=CARTESIAN_POINT ( 'NONE',  ( 5.015379008610445943, -183.6283474603465606, -112.9749434763326690 ) ) ;
#45608=ORIENTED_EDGE ( 'NONE', *, *, #15707, .F. ) ;
#45609=EDGE_CURVE ( 'NONE', #7466, #4324, #6959, .T. ) ;
#45610=ORIENTED_EDGE ( 'NONE', *, *, #23402, .F. ) ;
#45615=VECTOR ( 'NONE', #41817, 1000.000000000000000 ) ;
#45616=ORIENTED_EDGE ( 'NONE', *, *, #17663, .T. ) ;
#45617=ADVANCED_FACE ( 'NONE', ( #51908 ), #36112, .T. ) ;
#45618=AXIS2_PLACEMENT_3D ( 'NONE', #20043, #44222, #47909 ) ;
#45620=CARTESIAN_POINT ( 'NONE',  ( -49.08592689732745384, -193.5000000000000000, 0.7948544414133550395 ) ) ;
#45621=ORIENTED_EDGE ( 'NONE', *, *, #47791, .F. ) ;
#45622=ORIENTED_EDGE ( 'NONE', *, *, #39764, .T. ) ;
#45623=ADVANCED_FACE ( 'NONE', ( #3017 ), #28219, .T. ) ;
#45626=ADVANCED_FACE ( 'NONE', ( #23269 ), #19817, .T. ) ;
#45629=EDGE_LOOP ( 'NONE', ( #27153, #39105, #46539, #9869 ) ) ;
#45630=CARTESIAN_POINT ( 'NONE',  ( -166.6807411098556031, -193.5000000000000000, 37.47770156625504967 ) ) ;
#45636=AXIS2_PLACEMENT_3D ( 'NONE', #37531, #17313, #45426 ) ;
#45637=FACE_OUTER_BOUND ( 'NONE', #4035, .T. ) ;
#45639=LINE ( 'NONE', #17773, #34860 ) ;
#45640=FACE_OUTER_BOUND ( 'NONE', #18202, .T. ) ;
#45643=EDGE_CURVE ( 'NONE', #37290, #51892, #3645, .T. ) ;
#45645=FACE_BOUND ( 'NONE', #38853, .T. ) ;
#45647=DIRECTION ( 'NONE',  ( 0.000000000000000000, 0.000000000000000000, 1.000000000000000000 ) ) ;
#45648=VERTEX_POINT ( 'NONE', #51142 ) ;
#45649=AXIS2_PLACEMENT_3D ( 'NONE', #46227, #14418, #18859 ) ;
#45651=PLANE ( 'NONE',  #14573 ) ;
#45652=VERTEX_POINT ( 'NONE', #27706 ) ;
#45653=CIRCLE ( 'NONE', #31336, 125.0000000000000000 ) ;
#45654=CARTESIAN_POINT ( 'NONE',  ( -129.5578577291868214, -175.3837268820161057, 93.82025162278054609 ) ) ;
#45655=CARTESIAN_POINT ( 'NONE',  ( -48.36085358058748795, -175.3837268820161057, 0.9929810960135245779 ) ) ;
#45656=CARTESIAN_POINT ( 'NONE',  ( -104.8182102393454045, -189.7472609257535510, 111.5836353223472770 ) ) ;
#45657=ORIENTED_EDGE ( 'NONE', *, *, #9895, .T. ) ;
#45660=CARTESIAN_POINT ( 'NONE',  ( -160.2705093830644216, -193.5000000000000000, -55.92572546981520532 ) ) ;
#45663=ORIENTED_EDGE ( 'NONE', *, *, #37824, .F. ) ;
#45664=ORIENTED_EDGE ( 'NONE', *, *, #34397, .F. ) ;
#45665=DIRECTION ( 'NONE',  ( 0.000000000000000000, -0.000000000000000000, -1.000000000000000000 ) ) ;
#45666=CARTESIAN_POINT ( 'NONE',  ( -99.02518858244150124, -189.7472609257535510, 114.3245189510261355 ) ) ;
#45667=ORIENTED_EDGE ( 'NONE', *, *, #44319, .F. ) ;
#45668=DIRECTION ( 'NONE',  ( -0.000000000000000000, 1.000000000000000000, -0.000000000000000000 ) ) ;
#45669=PLANE ( 'NONE',  #29701 ) ;
#45670=ORIENTED_EDGE ( 'NONE', *, *, #15929, .T. ) ;
#45672=DIRECTION ( 'NONE',  ( -0.000000000000000000, -1.000000000000000000, 0.000000000000000000 ) ) ;
#45673=EDGE_LOOP ( 'NONE', ( #22468, #15619, #12428, #49855 ) ) ;
#45674=CARTESIAN_POINT ( 'NONE',  ( -75.48985759771373694, -183.6283474603465606, -122.0467960216648606 ) ) ;
#45675=ORIENTED_EDGE ( 'NONE', *, *, #41136, .T. ) ;
#45676=ORIENTED_EDGE ( 'NONE', *, *, #13790, .F. ) ;
#45678=ORIENTED_EDGE ( 'NONE', *, *, #35291, .F. ) ;
#45681=AXIS2_PLACEMENT_3D ( 'NONE', #21194, #45383, #49324 ) ;
#45683=AXIS2_PLACEMENT_3D ( 'NONE', #36482, #48069, #482 ) ;
#45684=DIRECTION ( 'NONE',  ( -0.000000000000000000, 1.000000000000000000, -0.000000000000000000 ) ) ;
#45686=ORIENTED_EDGE ( 'NONE', *, *, #20192, .F. ) ;
#45688=ORIENTED_EDGE ( 'NONE', *, *, #21600, .F. ) ;
#45691=ORIENTED_EDGE ( 'NONE', *, *, #18248, .T. ) ;
#45692=CYLINDRICAL_SURFACE ( 'NONE', #26190, 125.0000000000000000 ) ;
#45693=CARTESIAN_POINT ( 'NONE',  ( 74.48795740376235130, -177.1207230881787780, -15.97798378892165871 ) ) ;
#45697=LINE ( 'NONE', #41992, #35746 ) ;
#45698=CARTESIAN_POINT ( 'NONE',  ( 41.00573479224730988, -183.6283474603465606, -87.27805883780176543 ) ) ;
#45701=DIRECTION ( 'NONE',  ( -0.9473263538541946138, 0.000000000000000000, 0.3202698538628279690 ) ) ;
#45707=EDGE_LOOP ( 'NONE', ( #34615, #37418, #26938, #14195 ) ) ;
#45709=DIRECTION ( 'NONE',  ( 0.000000000000000000, 0.000000000000000000, 1.000000000000000000 ) ) ;
#45710=CARTESIAN_POINT ( 'NONE',  ( 75.27070168362158142, -193.5000000000000000, 17.63462396184792524 ) ) ;
#45711=ORIENTED_EDGE ( 'NONE', *, *, #10772, .T. ) ;
#45712=CARTESIAN_POINT ( 'NONE',  ( -170.6250538923603131, -175.3837268820161057, 26.55884942729649723 ) ) ;
#45716=CARTESIAN_POINT ( 'NONE',  ( -107.6930423737362190, -183.6283474603465606, 110.0850225811110761 ) ) ;
#45717=CIRCLE ( 'NONE', #51595, 125.0000000000000000 ) ;
#45718=AXIS2_PLACEMENT_3D ( 'NONE', #8903, #5242, #41473 ) ;
#45720=EDGE_CURVE ( 'NONE', #29784, #18925, #7494, .T. ) ;
#45721=CARTESIAN_POINT ( 'NONE',  ( 57.12946453413545100, -189.7472609257535510, 66.87170886601998632 ) ) ;
#45724=DIRECTION ( 'NONE',  ( -0.7948544414133523750, 0.000000000000000000, -0.6068001458185945385 ) ) ;
#45725=ORIENTED_EDGE ( 'NONE', *, *, #14675, .T. ) ;
#45726=LINE ( 'NONE', #9718, #35923 ) ;
#45727=ORIENTED_EDGE ( 'NONE', *, *, #44152, .T. ) ;
#45729=ORIENTED_EDGE ( 'NONE', *, *, #42614, .F. ) ;
#45730=CIRCLE ( 'NONE', #390, 125.0000000000000000 ) ;
#45734=PLANE ( 'NONE',  #19951 ) ;
#45736=EDGE_LOOP ( 'NONE', ( #6832, #1389, #43107, #10922 ) ) ;
#45737=EDGE_CURVE ( 'NONE', #33164, #45018, #3792, .T. ) ;
#45738=FACE_OUTER_BOUND ( 'NONE', #4102, .T. ) ;
#45739=VERTEX_POINT ( 'NONE', #32168 ) ;
#45741=EDGE_LOOP ( 'NONE', ( #46982, #19297, #22144, #9675 ) ) ;
#45742=DIRECTION ( 'NONE',  ( -0.000000000000000000, 1.000000000000000000, -0.000000000000000000 ) ) ;
#45746=EDGE_LOOP ( 'NONE', ( #30127, #50395, #299, #38012 ) ) ;
#45747=PLANE ( 'NONE',  #40788 ) ;
#45754=DIRECTION ( 'NONE',  ( 0.000000000000000000, -0.000000000000000000, -1.000000000000000000 ) ) ;
#45755=AXIS2_PLACEMENT_3D ( 'NONE', #13359, #751, #25443 ) ;
#45756=PLANE ( 'NONE',  #30772 ) ;
#45761=LINE ( 'NONE', #20808, #30641 ) ;
#45762=VECTOR ( 'NONE', #33864, 1000.000000000000000 ) ;
#45763=LINE ( 'NONE', #46040, #1077 ) ;
#45766=PLANE ( 'NONE',  #51277 ) ;
#45767=VECTOR ( 'NONE', #6743, 1000.000000000000114 ) ;
#45768=CARTESIAN_POINT ( 'NONE',  ( -49.40581635894069024, -193.5000000000000000, 0.3758275821142362250 ) ) ;
#45773=VECTOR ( 'NONE', #20709, 999.9999999999998863 ) ;
#45774=CARTESIAN_POINT ( 'NONE',  ( -48.47912675150885065, -193.5000000000000000, 1.000000000000006883 ) ) ;
#45775=FACE_OUTER_BOUND ( 'NONE', #41384, .T. ) ;
#45776=CARTESIAN_POINT ( 'NONE',  ( 37.99238433767461487, -193.5000000000000000, -90.26448786734027863 ) ) ;
#45777=EDGE_LOOP ( 'NONE', ( #37321, #28057, #47332, #6239 ) ) ;
#45778=ORIENTED_EDGE ( 'NONE', *, *, #12756, .T. ) ;
#45779=DIRECTION ( 'NONE',  ( -0.4031234292879792847, 0.000000000000000000, 0.9151456172430153524 ) ) ;
#45780=EDGE_CURVE ( 'NONE', #8838, #29027, #37080, .T. ) ;
#45784=ORIENTED_EDGE ( 'NONE', *, *, #2103, .F. ) ;
#45786=EDGE_CURVE ( 'NONE', #27512, #26450, #13439, .T. ) ;
#45790=AXIS2_PLACEMENT_3D ( 'NONE', #32154, #28718, #40808 ) ;
#45793=DIRECTION ( 'NONE',  ( -0.000000000000000000, 1.000000000000000000, 0.000000000000000000 ) ) ;
#45794=VERTEX_POINT ( 'NONE', #4314 ) ;
#45796=CARTESIAN_POINT ( 'NONE',  ( -48.47912675150885065, -175.3837268820161057, 6.938893903907228378E-15 ) ) ;
#45798=AXIS2_PLACEMENT_3D ( 'NONE', #24092, #40099, #404 ) ;
#45799=ADVANCED_FACE ( 'NONE', ( #24291 ), #22098, .T. ) ;
#45800=AXIS2_PLACEMENT_3D ( 'NONE', #25643, #29844, #25911 ) ;
#45801=LINE ( 'NONE', #26073, #38170 ) ;
#45803=DIRECTION ( 'NONE',  ( 0.6749830015182142207, 0.000000000000000000, -0.7378332790417239107 ) ) ;
#45804=ORIENTED_EDGE ( 'NONE', *, *, #21503, .T. ) ;
#45805=CARTESIAN_POINT ( 'NONE',  ( -98.10897907742936752, -189.7472609257535510, 114.7252272087849292 ) ) ;
#45806=AXIS2_PLACEMENT_3D ( 'NONE', #16861, #33412, #33128 ) ;
#45808=DIRECTION ( 'NONE',  ( 0.000000000000000000, -1.000000000000000000, -0.000000000000000000 ) ) ;
#45809=VECTOR ( 'NONE', #15883, 1000.000000000000000 ) ;
#45811=ORIENTED_EDGE ( 'NONE', *, *, #22709, .F. ) ;
#45814=ORIENTED_EDGE ( 'NONE', *, *, #2816, .T. ) ;
#45822=AXIS2_PLACEMENT_3D ( 'NONE', #49392, #41480, #26222 ) ;
#45823=CARTESIAN_POINT ( 'NONE',  ( -47.49008656418669005, -175.3837268820161057, -0.1476465640024710591 ) ) ;
#45825=DIRECTION ( 'NONE',  ( -0.000000000000000000, 1.000000000000000000, -0.000000000000000000 ) ) ;
#45827=VECTOR ( 'NONE', #22614, 1000.000000000000000 ) ;
#45828=AXIS2_PLACEMENT_3D ( 'NONE', #47320, #22876, #38896 ) ;
#45829=CARTESIAN_POINT ( 'NONE',  ( 42.45000882818163035, -193.5000000000000000, -84.30834960112932208 ) ) ;
#45832=LINE ( 'NONE', #22169, #45907 ) ;
#45834=CARTESIAN_POINT ( 'NONE',  ( -144.0067397530739584, -177.1207230881787780, -80.61932246194587037 ) ) ;
#45835=ORIENTED_EDGE ( 'NONE', *, *, #46315, .T. ) ;
#45836=DIRECTION ( 'NONE',  ( -0.7175072570443395970, 0.000000000000000000, 0.6965510290629882695 ) ) ;
#45843=AXIS2_PLACEMENT_3D ( 'NONE', #12707, #36903, #25577 ) ;
#45844=VERTEX_POINT ( 'NONE', #29203 ) ;
#45846=VECTOR ( 'NONE', #38269, 1000.000000000000114 ) ;
#45847=EDGE_CURVE ( 'NONE', #29842, #4246, #26039, .T. ) ;
#45848=AXIS2_PLACEMENT_3D ( 'NONE', #6451, #6952, #47685 ) ;
#45850=ORIENTED_EDGE ( 'NONE', *, *, #22494, .F. ) ;
#45854=PLANE ( 'NONE',  #9900 ) ;
#45857=CARTESIAN_POINT ( 'NONE',  ( -213.8817838414232426, -213.5000000000000000, 10.00000000000002842 ) ) ;
#45858=DIRECTION ( 'NONE',  ( -0.7575112421616191360, 0.000000000000000000, -0.6528221181905227155 ) ) ;
#45859=ORIENTED_EDGE ( 'NONE', *, *, #16517, .T. ) ;
#45860=ORIENTED_EDGE ( 'NONE', *, *, #44097, .F. ) ;
#45866=DIRECTION ( 'NONE',  ( 0.000000000000000000, 0.000000000000000000, -1.000000000000000000 ) ) ;
#45867=LINE ( 'NONE', #25883, #23071 ) ;
#45868=ORIENTED_EDGE ( 'NONE', *, *, #6632, .T. ) ;
#45869=AXIS2_PLACEMENT_3D ( 'NONE', #14139, #26974, #2554 ) ;
#45871=DIRECTION ( 'NONE',  ( -0.000000000000000000, -1.000000000000000000, 0.000000000000000000 ) ) ;
#45873=ADVANCED_FACE ( 'NONE', ( #49462 ), #25267, .T. ) ;
#45874=VERTEX_POINT ( 'NONE', #5305 ) ;
#45876=CARTESIAN_POINT ( 'NONE',  ( -48.07600332222087758, -193.5000000000000000, -0.9151456172430111335 ) ) ;
#45879=AXIS2_PLACEMENT_3D ( 'NONE', #9694, #50177, #34388 ) ;
#45883=VERTEX_POINT ( 'NONE', #1618 ) ;
#45884=CARTESIAN_POINT ( 'NONE',  ( -47.57632892154311577, -177.1207230881787780, 0.4300652022765314997 ) ) ;
#45885=VECTOR ( 'NONE', #36930, 999.9999999999998863 ) ;
#45888=EDGE_CURVE ( 'NONE', #28628, #50885, #21322, .T. ) ;
#45890=FACE_OUTER_BOUND ( 'NONE', #36185, .T. ) ;
#45892=DIRECTION ( 'NONE',  ( 0.9473263538541946138, 0.000000000000000000, -0.3202698538628279690 ) ) ;
#45894=EDGE_CURVE ( 'NONE', #840, #3228, #1078, .T. ) ;
#45895=EDGE_CURVE ( 'NONE', #15769, #40690, #25784, .T. ) ;
#45896=CARTESIAN_POINT ( 'NONE',  ( -111.3295483157475445, -193.5000000000000000, 108.0501018472332504 ) ) ;
#45898=FACE_OUTER_BOUND ( 'NONE', #11944, .T. ) ;
#45899=CARTESIAN_POINT ( 'NONE',  ( -56.71246971489870958, -189.7472609257535510, -124.7285535218267540 ) ) ;
#45900=EDGE_CURVE ( 'NONE', #38948, #42748, #33854, .T. ) ;
#45901=CARTESIAN_POINT ( 'NONE',  ( 76.46082103836693022, -193.5000000000000000, 3.874202661595785191 ) ) ;
#45902=ADVANCED_FACE ( 'NONE', ( #42063 ), #38111, .F. ) ;
#45904=FACE_BOUND ( 'NONE', #8249, .T. ) ;
#45906=CIRCLE ( 'NONE', #49277, 125.0000000000000000 ) ;
#45907=VECTOR ( 'NONE', #42130, 1000.000000000000000 ) ;
#45908=EDGE_CURVE ( 'NONE', #39220, #43850, #40549, .T. ) ;
#45912=EDGE_LOOP ( 'NONE', ( #26325, #15784, #30572, #50791 ) ) ;
#45914=EDGE_CURVE ( 'NONE', #40260, #41906, #50486, .T. ) ;
#45915=ORIENTED_EDGE ( 'NONE', *, *, #18769, .F. ) ;
#45916=EDGE_CURVE ( 'NONE', #43457, #25456, #2894, .T. ) ;
#45917=DIRECTION ( 'NONE',  ( -0.7378332790417239107, 0.000000000000000000, -0.6749830015182142207 ) ) ;
#45918=VECTOR ( 'NONE', #45095, 1000.000000000000114 ) ;
#45921=VECTOR ( 'NONE', #43470, 1000.000000000000000 ) ;
#45922=CARTESIAN_POINT ( 'NONE',  ( -173.4460699164830260, -175.3837268820161057, -2.874563619423225802 ) ) ;
#45923=ORIENTED_EDGE ( 'NONE', *, *, #26613, .F. ) ;
#45928=DIRECTION ( 'NONE',  ( 0.000000000000000000, 1.000000000000000000, 0.000000000000000000 ) ) ;
#45929=LINE ( 'NONE', #9914, #45846 ) ;
#45930=ORIENTED_EDGE ( 'NONE', *, *, #3807, .F. ) ;
#45931=EDGE_LOOP ( 'NONE', ( #36655, #46640, #5658, #14888 ) ) ;
#45932=ADVANCED_FACE ( 'NONE', ( #23137 ), #50739, .T. ) ;
#45934=CIRCLE ( 'NONE', #11505, 125.0000000000000000 ) ;
#45935=DIRECTION ( 'NONE',  ( 0.000000000000000000, 0.000000000000000000, -1.000000000000000000 ) ) ;
#45938=DIRECTION ( 'NONE',  ( -0.3482016354344059095, 0.000000000000000000, 0.9374196611341183427 ) ) ;
#45939=CARTESIAN_POINT ( 'NONE',  ( -130.2106798473772642, -189.7472609257535510, 94.57776286494221551 ) ) ;
#45940=ORIENTED_EDGE ( 'NONE', *, *, #40463, .F. ) ;
#45941=EDGE_CURVE ( 'NONE', #14246, #33159, #35207, .T. ) ;
#45943=PLANE ( 'NONE',  #31590 ) ;
#45945=LINE ( 'NONE', #29367, #19743 ) ;
#45947=AXIS2_PLACEMENT_3D ( 'NONE', #36816, #1059, #40737 ) ;
#45951=CARTESIAN_POINT ( 'NONE',  ( -48.36085358058748795, -189.7472609257535510, 0.9929810960135245779 ) ) ;
#45952=CARTESIAN_POINT ( 'NONE',  ( -4.176930889631405464, -193.5000000000000000, 116.8859077982279615 ) ) ;
#45953=ORIENTED_EDGE ( 'NONE', *, *, #25607, .T. ) ;
#45954=AXIS2_PLACEMENT_3D ( 'NONE', #50193, #30203, #33874 ) ;
#45958=CARTESIAN_POINT ( 'NONE',  ( -126.3604277550461319, -183.6283474603465606, 96.49160960477098570 ) ) ;
#45960=ORIENTED_EDGE ( 'NONE', *, *, #14480, .F. ) ;
#45962=AXIS2_PLACEMENT_3D ( 'NONE', #38983, #10111, #39257 ) ;
#45963=CARTESIAN_POINT ( 'NONE',  ( -18.95304271317702671, -175.3837268820161057, -121.4627941443854979 ) ) ;
#45966=DIRECTION ( 'NONE',  ( 0.9646355819083556327, 0.000000000000000000, 0.2635871660690782825 ) ) ;
#45969=DIRECTION ( 'NONE',  ( 0.000000000000000000, -1.000000000000000000, 0.000000000000000000 ) ) ;
#45970=DIRECTION ( 'NONE',  ( -0.000000000000000000, 1.000000000000000000, -0.000000000000000000 ) ) ;
#45972=EDGE_CURVE ( 'NONE', #50885, #18264, #39150, .T. ) ;
#45978=DIRECTION ( 'NONE',  ( 0.000000000000000000, 1.000000000000000000, 0.000000000000000000 ) ) ;
#45979=EDGE_CURVE ( 'NONE', #14211, #20982, #3407, .T. ) ;
#45981=ADVANCED_FACE ( 'NONE', ( #38891 ), #18927, .T. ) ;
#45983=ORIENTED_EDGE ( 'NONE', *, *, #35606, .T. ) ;
#45986=DIRECTION ( 'NONE',  ( -0.000000000000000000, 1.000000000000000000, -0.000000000000000000 ) ) ;
#45987=VERTEX_POINT ( 'NONE', #15248 ) ;
#45990=CARTESIAN_POINT ( 'NONE',  ( -173.4724443937511751, -183.6283474603465606, 1.292495564989516454 ) ) ;
#45993=DIRECTION ( 'NONE',  ( 0.000000000000000000, 0.000000000000000000, 1.000000000000000000 ) ) ;
#45994=VECTOR ( 'NONE', #17218, 1000.000000000000114 ) ;
#45996=DIRECTION ( 'NONE',  ( -1.000000000000000000, 0.000000000000000000, -0.000000000000000000 ) ) ;
#45997=EDGE_LOOP ( 'NONE', ( #22609, #37652, #12786, #17696 ) ) ;
#45999=DIRECTION ( 'NONE',  ( 0.000000000000000000, 0.000000000000000000, 1.000000000000000000 ) ) ;
#46004=FACE_OUTER_BOUND ( 'NONE', #15897, .T. ) ;
#46005=ORIENTED_EDGE ( 'NONE', *, *, #2217, .F. ) ;
#46006=VECTOR ( 'NONE', #47543, 1000.000000000000000 ) ;
#46011=DIRECTION ( 'NONE',  ( 0.000000000000000000, -1.000000000000000000, 0.000000000000000000 ) ) ;
#46012=VERTEX_POINT ( 'NONE', #3157 ) ;
#46015=PLANE ( 'NONE',  #46620 ) ;
#46017=DIRECTION ( 'NONE',  ( 0.000000000000000000, 0.000000000000000000, -1.000000000000000000 ) ) ;
#46020=EDGE_LOOP ( 'NONE', ( #27811, #30867, #7979, #22128 ) ) ;
#46022=DIRECTION ( 'NONE',  ( -0.8757349421956379665, 0.000000000000000000, 0.4827922027307427477 ) ) ;
#46023=( GEOMETRIC_REPRESENTATION_CONTEXT ( 3 ) GLOBAL_UNCERTAINTY_ASSIGNED_CONTEXT ( ( #1713 ) ) GLOBAL_UNIT_ASSIGNED_CONTEXT ( ( #20522, #39453, #291 ) ) REPRESENTATION_CONTEXT ( 'NONE', 'WORKASPACE' ) );
#46024=ORIENTED_EDGE ( 'NONE', *, *, #28541, .F. ) ;
#46029=LINE ( 'NONE', #34179, #50703 ) ;
#46032=PLANE ( 'NONE',  #13392 ) ;
#46033=VECTOR ( 'NONE', #43894, 1000.000000000000000 ) ;
#46035=EDGE_LOOP ( 'NONE', ( #8857, #47191, #10396, #39570 ) ) ;
#46036=EDGE_CURVE ( 'NONE', #47996, #51413, #22357, .T. ) ;
#46038=DIRECTION ( 'NONE',  ( 0.000000000000000000, 0.000000000000000000, 1.000000000000000000 ) ) ;
#46039=CARTESIAN_POINT ( 'NONE',  ( -48.47912675150885065, -175.3837268820161057, 6.938893903907228378E-15 ) ) ;
#46040=CARTESIAN_POINT ( 'NONE',  ( -170.2790847791494855, -183.6283474603465606, -28.10285082451569494 ) ) ;
#46041=ORIENTED_EDGE ( 'NONE', *, *, #22642, .T. ) ;
#46043=CARTESIAN_POINT ( 'NONE',  ( -105.8382074681673117, -193.5000000000000000, -109.9360785596604586 ) ) ;
#46045=CARTESIAN_POINT ( 'NONE',  ( -7.515176836080578404, -193.5000000000000000, 117.0391155081705250 ) ) ;
#46046=CARTESIAN_POINT ( 'NONE',  ( -48.47912675150885065, -183.6283474603465606, 6.938893903907228378E-15 ) ) ;
#46048=AXIS2_PLACEMENT_3D ( 'NONE', #18658, #27039, #30991 ) ;
#46049=DIRECTION ( 'NONE',  ( 0.9995608365087944591, 0.000000000000000000, -0.02963332782255633305 ) ) ;
#46050=ADVANCED_FACE ( 'NONE', ( #2637 ), #38382, .T. ) ;
#46051=DIRECTION ( 'NONE',  ( 0.000000000000000000, -1.000000000000000000, 0.000000000000000000 ) ) ;
#46055=CARTESIAN_POINT ( 'NONE',  ( -59.28786813212836648, -183.6283474603465606, 124.5318076226587465 ) ) ;
#46057=ORIENTED_EDGE ( 'NONE', *, *, #5091, .F. ) ;
#46059=ORIENTED_EDGE ( 'NONE', *, *, #45916, .T. ) ;
#46061=ORIENTED_EDGE ( 'NONE', *, *, #5327, .F. ) ;
#46064=ADVANCED_FACE ( 'NONE', ( #27320 ), #43367, .T. ) ;
#46065=CARTESIAN_POINT ( 'NONE',  ( -145.0195698084541505, -193.5000000000000000, 79.40367028273128369 ) ) ;
#46066=CARTESIAN_POINT ( 'NONE',  ( -47.63353074800703268, -175.3837268820161057, 0.5338233779648018373 ) ) ;
#46070=VECTOR ( 'NONE', #6232, 1000.000000000000114 ) ;
#46073=EDGE_CURVE ( 'NONE', #6422, #47448, #3666, .T. ) ;
#46074=DIRECTION ( 'NONE',  ( -0.9564009842765223146, 0.000000000000000000, -0.2920567706369764371 ) ) ;
#46078=CARTESIAN_POINT ( 'NONE',  ( -48.47912675150885065, -175.3837268820161057, 6.938893903907228378E-15 ) ) ;
#46080=LINE ( 'NONE', #37125, #24042 ) ;
#46081=VECTOR ( 'NONE', #44332, 1000.000000000000000 ) ;
#46082=EDGE_CURVE ( 'NONE', #21402, #22201, #28084, .T. ) ;
#46083=ORIENTED_EDGE ( 'NONE', *, *, #8802, .F. ) ;
#46085=PLANE ( 'NONE',  #13057 ) ;
#46086=CARTESIAN_POINT ( 'NONE',  ( 72.95485052494851175, -193.5000000000000000, -29.64437826672757481 ) ) ;
#46087=ORIENTED_EDGE ( 'NONE', *, *, #45218, .T. ) ;
#46089=ORIENTED_EDGE ( 'NONE', *, *, #9347, .F. ) ;
#46091=DIRECTION ( 'NONE',  ( -0.000000000000000000, 1.000000000000000000, -0.000000000000000000 ) ) ;
#46093=FACE_OUTER_BOUND ( 'NONE', #50258, .T. ) ;
#46096=ORIENTED_EDGE ( 'NONE', *, *, #13331, .T. ) ;
#46098=LINE ( 'NONE', #49253, #4427 ) ;
#46099=AXIS2_PLACEMENT_3D ( 'NONE', #16829, #32833, #48885 ) ;
#46100=CARTESIAN_POINT ( 'NONE',  ( -48.65601702663141737, -177.1207230881787780, -0.9842305779475923888 ) ) ;
#46101=DIRECTION ( 'NONE',  ( -0.000000000000000000, 1.000000000000000000, -0.000000000000000000 ) ) ;
#46104=DIRECTION ( 'NONE',  ( 0.000000000000000000, 0.000000000000000000, -1.000000000000000000 ) ) ;
#46107=ORIENTED_EDGE ( 'NONE', *, *, #39706, .T. ) ;
#46110=AXIS2_PLACEMENT_3D ( 'NONE', #33296, #25162, #12547 ) ;
#46111=EDGE_CURVE ( 'NONE', #11646, #30315, #15508, .T. ) ;
#46112=CARTESIAN_POINT ( 'NONE',  ( -121.1142239062970418, -177.1207230881787780, 101.7307360698549132 ) ) ;
#46116=CYLINDRICAL_SURFACE ( 'NONE', #571, 125.0000000000000000 ) ;
#46117=EDGE_CURVE ( 'NONE', #38778, #32529, #40584, .T. ) ;
#46118=VECTOR ( 'NONE', #33657, 1000.000000000000000 ) ;
#46120=EDGE_LOOP ( 'NONE', ( #11072, #1262, #14065, #35918 ) ) ;
#46121=CARTESIAN_POINT ( 'NONE',  ( -149.1282321233095161, -175.3837268820161057, -72.42760398749013007 ) ) ;
#46122=ORIENTED_EDGE ( 'NONE', *, *, #2575, .F. ) ;
#46123=DIRECTION ( 'NONE',  ( -0.000000000000000000, 1.000000000000000000, -0.000000000000000000 ) ) ;
#46124=CARTESIAN_POINT ( 'NONE',  ( 2.669657140899367676, -175.3837268820161057, 114.0561348912355726 ) ) ;
#46125=DIRECTION ( 'NONE',  ( 0.000000000000000000, -0.000000000000000000, 1.000000000000000000 ) ) ;
#46126=CARTESIAN_POINT ( 'NONE',  ( -48.07600332222087758, -183.6283474603465606, -0.9151456172430111335 ) ) ;
#46127=VERTEX_POINT ( 'NONE', #32033 ) ;
#46128=VERTEX_POINT ( 'NONE', #28610 ) ;
#46129=VERTEX_POINT ( 'NONE', #44407 ) ;
#46130=CARTESIAN_POINT ( 'NONE',  ( -166.9492939735806090, -193.5000000000000000, 39.87254040532603483 ) ) ;
#46131=DIRECTION ( 'NONE',  ( 0.000000000000000000, 1.000000000000000000, -0.000000000000000000 ) ) ;
#46133=DIRECTION ( 'NONE',  ( -0.9785564922995032555, 0.000000000000000000, -0.2059786187411021818 ) ) ;
#46138=EDGE_CURVE ( 'NONE', #29888, #48694, #44657, .T. ) ;
#46139=PLANE ( 'NONE',  #43318 ) ;
#46141=CARTESIAN_POINT ( 'NONE',  ( -122.3978016498073345, -183.6283474603465606, -100.8019320314827070 ) ) ;
#46145=DIRECTION ( 'NONE',  ( -0.000000000000000000, 1.000000000000000000, -0.000000000000000000 ) ) ;
#46148=EDGE_CURVE ( 'NONE', #31562, #13288, #47576, .T. ) ;
#46149=CARTESIAN_POINT ( 'NONE',  ( -104.8182102393454045, -193.5000000000000000, 111.5836353223472912 ) ) ;
#46150=ORIENTED_EDGE ( 'NONE', *, *, #22460, .T. ) ;
#46152=VECTOR ( 'NONE', #1177, 1000.000000000000114 ) ;
#46153=ORIENTED_EDGE ( 'NONE', *, *, #22996, .T. ) ;
#46159=CARTESIAN_POINT ( 'NONE',  ( -78.64590280292340196, -189.7472609257535510, -121.3052580173827266 ) ) ;
#46160=LINE ( 'NONE', #46408, #29723 ) ;
#46161=CARTESIAN_POINT ( 'NONE',  ( 75.28414827670442833, -177.1207230881787780, -7.666780576874956843 ) ) ;
#46162=DIRECTION ( 'NONE',  ( -0.000000000000000000, 1.000000000000000000, -0.000000000000000000 ) ) ;
#46163=FACE_OUTER_BOUND ( 'NONE', #44795, .T. ) ;
#46164=ADVANCED_FACE ( 'NONE', ( #35722 ), #39910, .F. ) ;
#46165=ORIENTED_EDGE ( 'NONE', *, *, #45214, .F. ) ;
#46167=CYLINDRICAL_SURFACE ( 'NONE', #10400, 125.0000000000000000 ) ;
#46169=VERTEX_POINT ( 'NONE', #16279 ) ;
#46171=EDGE_LOOP ( 'NONE', ( #8735, #30915, #2666, #9130 ) ) ;
#46173=DIRECTION ( 'NONE',  ( 0.000000000000000000, 0.000000000000000000, 1.000000000000000000 ) ) ;
#46174=DIRECTION ( 'NONE',  ( -0.8757349421956412971, 0.000000000000000000, 0.4827922027307366970 ) ) ;
#46175=CARTESIAN_POINT ( 'NONE',  ( -173.4787860028527007, -177.1207230881787780, 0.2918682030023981300 ) ) ;
#46176=VERTEX_POINT ( 'NONE', #35996 ) ;
#46179=DIRECTION ( 'NONE',  ( 0.8896570909947436601, 0.000000000000000000, 0.4566292373937200777 ) ) ;
#46180=DIRECTION ( 'NONE',  ( 0.000000000000000000, -0.000000000000000000, -1.000000000000000000 ) ) ;
#46183=VECTOR ( 'NONE', #47717, 1000.000000000000000 ) ;
#46184=VERTEX_POINT ( 'NONE', #48079 ) ;
#46186=PLANE ( 'NONE',  #45329 ) ;
#46188=CARTESIAN_POINT ( 'NONE',  ( -18.95304271317703382, -189.7472609257535510, -121.4627941443854837 ) ) ;
#46190=DIRECTION ( 'NONE',  ( 0.000000000000000000, -1.000000000000000000, 0.000000000000000000 ) ) ;
#46191=ORIENTED_EDGE ( 'NONE', *, *, #22112, .F. ) ;
#46193=EDGE_CURVE ( 'NONE', #14965, #49533, #4987, .T. ) ;
#46197=VERTEX_POINT ( 'NONE', #21526 ) ;
#46198=CARTESIAN_POINT ( 'NONE',  ( -144.2430459457361280, -175.3837268820161057, 78.77358243914956404 ) ) ;
#46199=EDGE_LOOP ( 'NONE', ( #13030, #11701, #11887, #18290 ) ) ;
#46200=ORIENTED_EDGE ( 'NONE', *, *, #38757, .T. ) ;
#46203=DIRECTION ( 'NONE',  ( 0.000000000000000000, 0.000000000000000000, -1.000000000000000000 ) ) ;
#46204=ORIENTED_EDGE ( 'NONE', *, *, #11587, .T. ) ;
#46206=VERTEX_POINT ( 'NONE', #25462 ) ;
#46208=DIRECTION ( 'NONE',  ( 0.7378332790417285736, 0.000000000000000000, -0.6749830015182091136 ) ) ;
#46209=VERTEX_POINT ( 'NONE', #37555 ) ;
#46210=EDGE_CURVE ( 'NONE', #6055, #2868, #47331, .T. ) ;
#46212=VERTEX_POINT ( 'NONE', #1798 ) ;
#46213=ADVANCED_FACE ( 'NONE', ( #45446 ), #9962, .T. ) ;
#46214=ORIENTED_EDGE ( 'NONE', *, *, #35540, .F. ) ;
#46216=LINE ( 'NONE', #2822, #13858 ) ;
#46218=CARTESIAN_POINT ( 'NONE',  ( -23.01747912075234836, -177.1207230881787780, -122.3793467049370634 ) ) ;
#46221=CARTESIAN_POINT ( 'NONE',  ( -133.8011377042516301, -183.6283474603465606, -91.35181687837437892 ) ) ;
#46222=LINE ( 'NONE', #26217, #31477 ) ;
#46224=CARTESIAN_POINT ( 'NONE',  ( -55.05561436132772002, -175.3837268820161057, 124.8268793598474105 ) ) ;
#46225=DIRECTION ( 'NONE',  ( -0.9890401873221623674, 0.000000000000000000, -0.1476465640024917925 ) ) ;
#46227=CARTESIAN_POINT ( 'NONE',  ( 19.33815737959698566, -183.6283474603465606, 105.0038855142078233 ) ) ;
#46228=CARTESIAN_POINT ( 'NONE',  ( -49.45768324380835423, -193.5000000000000000, -0.2059786187411025149 ) ) ;
#46234=DIRECTION ( 'NONE',  ( -0.000000000000000000, 1.000000000000000000, -0.000000000000000000 ) ) ;
#46235=LINE ( 'NONE', #18372, #26092 ) ;
#46237=CARTESIAN_POINT ( 'NONE',  ( -161.2555905272864436, -175.3837268820161057, -53.91167979418489864 ) ) ;
#46239=EDGE_CURVE ( 'NONE', #35941, #45486, #13380, .T. ) ;
#46241=VECTOR ( 'NONE', #24572, 1000.000000000000227 ) ;
#46243=LINE ( 'NONE', #14186, #13617 ) ;
#46244=CARTESIAN_POINT ( 'NONE',  ( 57.66105628977221897, -175.3837268820161057, 66.02470404298190942 ) ) ;
#46245=CARTESIAN_POINT ( 'NONE',  ( -19.28375372365792728, -175.3837268820161057, 121.5427093402341256 ) ) ;
#46247=LINE ( 'NONE', #38338, #457 ) ;
#46248=VERTEX_POINT ( 'NONE', #17593 ) ;
#46250=CARTESIAN_POINT ( 'NONE',  ( -151.4272465800706300, -183.6283474603465606, 70.89911581792885897 ) ) ;
#46251=VERTEX_POINT ( 'NONE', #29392 ) ;
#46252=LINE ( 'NONE', #26253, #15032 ) ;
#46253=VECTOR ( 'NONE', #28672, 1000.000000000000114 ) ;
#46254=ADVANCED_FACE ( 'NONE', ( #33081 ), #13897, .T. ) ;
#46259=CARTESIAN_POINT ( 'NONE',  ( -48.47912675150885065, -183.6283474603465606, 6.938893903907228378E-15 ) ) ;
#46261=ORIENTED_EDGE ( 'NONE', *, *, #34404, .F. ) ;
#46263=CARTESIAN_POINT ( 'NONE',  ( -49.17567778057184569, -175.3837268820161057, -0.7175072570443327136 ) ) ;
#46266=ORIENTED_EDGE ( 'NONE', *, *, #25312, .T. ) ;
#46271=CARTESIAN_POINT ( 'NONE',  ( -166.9492939735806090, -189.7472609257535510, 39.87254040532606325 ) ) ;
#46272=VERTEX_POINT ( 'NONE', #32820 ) ;
#46273=EDGE_LOOP ( 'NONE', ( #17624, #19988, #10617, #19476 ) ) ;
#46274=CARTESIAN_POINT ( 'NONE',  ( -153.4237445717492392, -193.5000000000000000, 66.05018866041351089 ) ) ;
#46275=ORIENTED_EDGE ( 'NONE', *, *, #964, .T. ) ;
#46277=DIRECTION ( 'NONE',  ( 0.000000000000000000, -1.000000000000000000, 0.000000000000000000 ) ) ;
#46278=CIRCLE ( 'NONE', #28644, 124.9999999999999858 ) ;
#46279=EDGE_CURVE ( 'NONE', #51589, #44868, #2580, .T. ) ;
#46281=DIRECTION ( 'NONE',  ( 0.9995608365087946812, 0.000000000000000000, -0.02963332782254913048 ) ) ;
#46284=CARTESIAN_POINT ( 'NONE',  ( 36.19006208304271865, -193.5000000000000000, 90.59430563621340582 ) ) ;
#46286=ADVANCED_FACE ( 'NONE', ( #42253 ), #22288, .T. ) ;
#46287=VERTEX_POINT ( 'NONE', #27256 ) ;
#46289=CARTESIAN_POINT ( 'NONE',  ( -73.94077438226447896, -177.1207230881787780, 122.3793467049372481 ) ) ;
#46290=FACE_OUTER_BOUND ( 'NONE', #29253, .T. ) ;
#46291=ADVANCED_FACE ( 'NONE', ( #50426 ), #15192, .T. ) ;
#46292=FACE_OUTER_BOUND ( 'NONE', #2030, .T. ) ;
#46293=VERTEX_POINT ( 'NONE', #47258 ) ;
#46294=CARTESIAN_POINT ( 'NONE',  ( -37.78865854180984485, -177.1207230881787780, -123.5388265266451242 ) ) ;
#46295=CARTESIAN_POINT ( 'NONE',  ( -159.0901268547125653, -177.1207230881787780, 58.22548115875958530 ) ) ;
#46297=PLANE ( 'NONE',  #5932 ) ;
#46298=CARTESIAN_POINT ( 'NONE',  ( -84.85683048652070681, -193.5000000000000000, 118.5439281552633304 ) ) ;
#46303=CARTESIAN_POINT ( 'NONE',  ( -166.6265240196292439, -189.7472609257535510, 40.81902153125349741 ) ) ;
#46304=EDGE_LOOP ( 'NONE', ( #23857, #13591, #22492, #6929 ) ) ;
#46306=VECTOR ( 'NONE', #29143, 1000.000000000000114 ) ;
#46308=DIRECTION ( 'NONE',  ( -0.2920567706369833760, 0.000000000000000000, 0.9564009842765202052 ) ) ;
#46310=ORIENTED_EDGE ( 'NONE', *, *, #38706, .F. ) ;
#46311=VECTOR ( 'NONE', #36740, 1000.000000000000000 ) ;
#46315=EDGE_CURVE ( 'NONE', #39193, #26105, #14168, .T. ) ;
#46316=DIRECTION ( 'NONE',  ( 0.02963332782256331357, 0.000000000000000000, -0.9995608365087942371 ) ) ;
#46317=DIRECTION ( 'NONE',  ( 0.9720229140804089729, 0.000000000000000000, 0.2348860457809911206 ) ) ;
#46320=DIRECTION ( 'NONE',  ( 0.000000000000000000, 1.000000000000000000, 0.000000000000000000 ) ) ;
#46322=EDGE_LOOP ( 'NONE', ( #48827, #23424, #39622, #23937 ) ) ;
#46323=DIRECTION ( 'NONE',  ( -0.000000000000000000, 1.000000000000000000, -0.000000000000000000 ) ) ;
#46325=DIRECTION ( 'NONE',  ( 0.000000000000000000, 1.000000000000000000, -0.000000000000000000 ) ) ;
#46326=AXIS2_PLACEMENT_3D ( 'NONE', #24733, #32341, #40746 ) ;
#46327=ORIENTED_EDGE ( 'NONE', *, *, #48982, .T. ) ;
#46330=AXIS2_PLACEMENT_3D ( 'NONE', #12766, #40889, #17255 ) ;
#46331=CARTESIAN_POINT ( 'NONE',  ( -49.03777351731250889, -177.1207230881787780, 0.8294056854502042109 ) ) ;
#46334=CARTESIAN_POINT ( 'NONE',  ( -132.6364218684650211, -193.5000000000000000, 92.42591454022807795 ) ) ;
#46335=FACE_OUTER_BOUND ( 'NONE', #37202, .T. ) ;
#46336=ORIENTED_EDGE ( 'NONE', *, *, #27541, .T. ) ;
#46339=CARTESIAN_POINT ( 'NONE',  ( 34.93559171950835918, -193.5000000000000000, -93.09664195018497423 ) ) ;
#46340=VERTEX_POINT ( 'NONE', #7303 ) ;
#46342=VECTOR ( 'NONE', #16104, 1000.000000000000114 ) ;
#46344=EDGE_CURVE ( 'NONE', #31839, #47039, #26483, .T. ) ;
#46345=ORIENTED_EDGE ( 'NONE', *, *, #41761, .T. ) ;
#46346=CARTESIAN_POINT ( 'NONE',  ( -47.47956591500005885, -175.3837268820161057, 0.02963332782257025594 ) ) ;
#46347=ORIENTED_EDGE ( 'NONE', *, *, #15071, .F. ) ;
#46349=VECTOR ( 'NONE', #37715, 1000.000000000000000 ) ;
#46350=DIRECTION ( 'NONE',  ( 0.9982437317643210184, 0.000000000000000000, 0.05924062789372143423 ) ) ;
#46351=DIRECTION ( 'NONE',  ( 0.000000000000000000, 1.000000000000000000, 0.000000000000000000 ) ) ;
#46352=EDGE_LOOP ( 'NONE', ( #16525, #466, #13840, #51983 ) ) ;
#46353=DIRECTION ( 'NONE',  ( 0.000000000000000000, 0.000000000000000000, -1.000000000000000000 ) ) ;
#46356=ORIENTED_EDGE ( 'NONE', *, *, #7872, .T. ) ;
#46359=CARTESIAN_POINT ( 'NONE',  ( -123.6678354051270077, -193.5000000000000000, 99.85818990449067201 ) ) ;
#46360=CARTESIAN_POINT ( 'NONE',  ( 40.71578595748727736, -193.5000000000000000, 86.14171647324928927 ) ) ;
#46362=ORIENTED_EDGE ( 'NONE', *, *, #15331, .F. ) ;
#46363=CIRCLE ( 'NONE', #39608, 125.0000000000000000 ) ;
#46364=ORIENTED_EDGE ( 'NONE', *, *, #11119, .F. ) ;
#46365=LINE ( 'NONE', #19017, #18219 ) ;
#46366=AXIS2_PLACEMENT_3D ( 'NONE', #49721, #838, #49203 ) ;
#46367=ADVANCED_FACE ( 'NONE', ( #31204 ), #18612, .T. ) ;
#46368=LINE ( 'NONE', #10352, #44741 ) ;
#46369=EDGE_LOOP ( 'NONE', ( #39359, #45086, #31957, #21759 ) ) ;
#46370=FACE_OUTER_BOUND ( 'NONE', #32287, .T. ) ;
#46373=EDGE_CURVE ( 'NONE', #3759, #37475, #17104, .T. ) ;
#46374=LINE ( 'NONE', #39497, #49651 ) ;
#46376=ORIENTED_EDGE ( 'NONE', *, *, #23677, .T. ) ;
#46378=ORIENTED_EDGE ( 'NONE', *, *, #42340, .F. ) ;
#46381=CARTESIAN_POINT ( 'NONE',  ( 73.09196206113300320, -177.1207230881787780, 29.07697310430963356 ) ) ;
#46382=DIRECTION ( 'NONE',  ( 0.000000000000000000, -1.000000000000000000, 0.000000000000000000 ) ) ;
#46383=AXIS2_PLACEMENT_3D ( 'NONE', #51203, #19635, #15451 ) ;
#46384=EDGE_CURVE ( 'NONE', #24976, #39182, #23072, .T. ) ;
#46385=VECTOR ( 'NONE', #21666, 1000.000000000000000 ) ;
#46386=DIRECTION ( 'NONE',  ( 0.8757349421956310831, 0.000000000000000000, 0.4827922027307550712 ) ) ;
#46388=EDGE_LOOP ( 'NONE', ( #23454, #9833, #12120, #4461 ) ) ;
#46389=EDGE_CURVE ( 'NONE', #40815, #20971, #6541, .T. ) ;
#46392=EDGE_LOOP ( 'NONE', ( #46500, #25115, #30537, #41778 ) ) ;
#46395=CARTESIAN_POINT ( 'NONE',  ( -36.09284319799462537, -177.1207230881787780, 124.3848060646152618 ) ) ;
#46396=AXIS2_PLACEMENT_3D ( 'NONE', #29057, #48547, #12764 ) ;
#46397=EDGE_CURVE ( 'NONE', #13886, #32088, #10726, .T. ) ;
#46399=DIRECTION ( 'NONE',  ( 0.6528221181905174975, 0.000000000000000000, 0.7575112421616236880 ) ) ;
#46400=ORIENTED_EDGE ( 'NONE', *, *, #34591, .F. ) ;
#46401=DIRECTION ( 'NONE',  ( -0.8124868780056825335, 0.000000000000000000, 0.5829794791144703447 ) ) ;
#46403=ORIENTED_EDGE ( 'NONE', *, *, #51396, .T. ) ;
#46404=DIRECTION ( 'NONE',  ( 0.000000000000000000, 0.000000000000000000, 1.000000000000000000 ) ) ;
#46406=ORIENTED_EDGE ( 'NONE', *, *, #48032, .T. ) ;
#46407=CARTESIAN_POINT ( 'NONE',  ( -94.25732089370191602, -183.6283474603465606, 116.3157639405754935 ) ) ;
#46408=CARTESIAN_POINT ( 'NONE',  ( -66.64622755927952369, -183.6283474603465606, 123.6727797384707372 ) ) ;
#46409=DIRECTION ( 'NONE',  ( 0.000000000000000000, 0.000000000000000000, 1.000000000000000000 ) ) ;
#46410=VECTOR ( 'NONE', #34187, 1000.000000000000227 ) ;
#46414=ORIENTED_EDGE ( 'NONE', *, *, #11935, .T. ) ;
#46415=VECTOR ( 'NONE', #23528, 1000.000000000000114 ) ;
#46418=EDGE_CURVE ( 'NONE', #28684, #51929, #14945, .T. ) ;
#46422=EDGE_CURVE ( 'NONE', #19489, #6776, #32197, .T. ) ;
#46423=PLANE ( 'NONE',  #31856 ) ;
#46425=DIRECTION ( 'NONE',  ( -0.000000000000000000, 1.000000000000000000, -0.000000000000000000 ) ) ;
#46426=PLANE ( 'NONE',  #47277 ) ;
#46429=VECTOR ( 'NONE', #34185, 1000.000000000000000 ) ;
#46430=EDGE_CURVE ( 'NONE', #24824, #13353, #39080, .T. ) ;
#46431=CARTESIAN_POINT ( 'NONE',  ( -48.47912675150885065, -177.1207230881787780, 6.938893903907228378E-15 ) ) ;
#46432=DIRECTION ( 'NONE',  ( 0.000000000000000000, 1.000000000000000000, 0.000000000000000000 ) ) ;
#46433=ORIENTED_EDGE ( 'NONE', *, *, #27148, .F. ) ;
#46435=EDGE_CURVE ( 'NONE', #2077, #51235, #35149, .T. ) ;
#46436=ADVANCED_FACE ( 'NONE', ( #44069 ), #36177, .F. ) ;
#46441=EDGE_CURVE ( 'NONE', #10769, #8260, #15716, .T. ) ;
#46444=ORIENTED_EDGE ( 'NONE', *, *, #7143, .F. ) ;
#46446=CARTESIAN_POINT ( 'NONE',  ( 72.14504940832446778, -193.5000000000000000, -32.78426643622660208 ) ) ;
#46448=FACE_OUTER_BOUND ( 'NONE', #20190, .T. ) ;
#46449=VERTEX_POINT ( 'NONE', #11745 ) ;
#46450=VECTOR ( 'NONE', #312, 1000.000000000000000 ) ;
#46451=ORIENTED_EDGE ( 'NONE', *, *, #6154, .F. ) ;
#46453=VERTEX_POINT ( 'NONE', #4383 ) ;
#46457=AXIS2_PLACEMENT_3D ( 'NONE', #30902, #14357, #14891 ) ;
#46460=CARTESIAN_POINT ( 'NONE',  ( -128.2395503755045638, -183.6283474603465606, -96.24590808611421267 ) ) ;
#46462=EDGE_LOOP ( 'NONE', ( #26031, #23094, #20682, #51535 ) ) ;
#46463=LINE ( 'NONE', #41987, #44698 ) ;
#46464=CARTESIAN_POINT ( 'NONE',  ( -19.18792875895802652, -193.5000000000000000, -120.4907712303050715 ) ) ;
#46466=ORIENTED_EDGE ( 'NONE', *, *, #51362, .T. ) ;
#46467=LINE ( 'NONE', #49386, #24843 ) ;
#46468=AXIS2_PLACEMENT_3D ( 'NONE', #10977, #43039, #7045 ) ;
#46470=DIRECTION ( 'NONE',  ( -0.000000000000000000, 1.000000000000000000, -0.000000000000000000 ) ) ;
#46471=CARTESIAN_POINT ( 'NONE',  ( 0.7476021451244393434, -193.5000000000000000, -113.8100815915415751 ) ) ;
#46472=ORIENTED_EDGE ( 'NONE', *, *, #12784, .T. ) ;
#46473=CARTESIAN_POINT ( 'NONE',  ( -47.82630463331832971, -183.6283474603465606, -0.7575112421616121416 ) ) ;
#46475=AXIS2_PLACEMENT_3D ( 'NONE', #38824, #19380, #39345 ) ;
#46477=ORIENTED_EDGE ( 'NONE', *, *, #39433, .T. ) ;
#46479=EDGE_CURVE ( 'NONE', #35187, #25387, #28295, .T. ) ;
#46483=EDGE_CURVE ( 'NONE', #42583, #10747, #35399, .T. ) ;
#46484=FACE_OUTER_BOUND ( 'NONE', #23533, .T. ) ;
#46485=VERTEX_POINT ( 'NONE', #39850 ) ;
#46487=CARTESIAN_POINT ( 'NONE',  ( -48.59739992243020623, -193.5000000000000000, -0.9929810960135115883 ) ) ;
#46489=LINE ( 'NONE', #34895, #1909 ) ;
#46491=LINE ( 'NONE', #46244, #11518 ) ;
#46492=EDGE_CURVE ( 'NONE', #13810, #18089, #15453, .T. ) ;
#46493=CARTESIAN_POINT ( 'NONE',  ( -19.28375372365792728, -193.5000000000000000, 121.5427093402341541 ) ) ;
#46494=ORIENTED_EDGE ( 'NONE', *, *, #22051, .F. ) ;
#46495=EDGE_CURVE ( 'NONE', #45117, #33386, #23339, .T. ) ;
#46500=ORIENTED_EDGE ( 'NONE', *, *, #43380, .F. ) ;
#46501=CARTESIAN_POINT ( 'NONE',  ( 12.54192669111252378, -193.5000000000000000, 107.9473519284347276 ) ) ;
#46504=VECTOR ( 'NONE', #39644, 1000.000000000000000 ) ;
#46505=AXIS2_PLACEMENT_3D ( 'NONE', #23834, #47767, #23574 ) ;
#46507=CARTESIAN_POINT ( 'NONE',  ( 76.52053249983504202, -193.5000000000000000, -0.2918682030015403162 ) ) ;
#46508=VERTEX_POINT ( 'NONE', #47507 ) ;
#46512=FACE_OUTER_BOUND ( 'NONE', #1985, .T. ) ;
#46513=ORIENTED_EDGE ( 'NONE', *, *, #40353, .T. ) ;
#46514=DIRECTION ( 'NONE',  ( 0.000000000000000000, 1.000000000000000000, 0.000000000000000000 ) ) ;
#46516=LINE ( 'NONE', #50468, #3227 ) ;
#46517=DIRECTION ( 'NONE',  ( 0.000000000000000000, 0.000000000000000000, 1.000000000000000000 ) ) ;
#46518=CARTESIAN_POINT ( 'NONE',  ( -158.9435005891548087, -177.1207230881787780, -56.33604425924758630 ) ) ;
#46522=VERTEX_POINT ( 'NONE', #20155 ) ;
#46525=DIRECTION ( 'NONE',  ( 0.9027978299657446470, 0.000000000000000000, -0.4300652022765183435 ) ) ;
#46526=LINE ( 'NONE', #38626, #9732 ) ;
#46528=PLANE ( 'NONE',  #28024 ) ;
#46529=CARTESIAN_POINT ( 'NONE',  ( -124.9871112439422092, -189.7472609257535510, -98.85104101073277150 ) ) ;
#46533=ORIENTED_EDGE ( 'NONE', *, *, #45124, .T. ) ;
#46537=EDGE_CURVE ( 'NONE', #3688, #13519, #39591, .T. ) ;
#46539=ORIENTED_EDGE ( 'NONE', *, *, #29149, .T. ) ;
#46540=DIRECTION ( 'NONE',  ( 0.6528221181905280446, 0.000000000000000000, -0.7575112421616145841 ) ) ;
#46543=VECTOR ( 'NONE', #43858, 1000.000000000000000 ) ;
#46545=PLANE ( 'NONE',  #2544 ) ;
#46547=DIRECTION ( 'NONE',  ( 0.8896570909947499883, 0.000000000000000000, -0.4566292373937077542 ) ) ;
#46548=EDGE_CURVE ( 'NONE', #36281, #29476, #50702, .T. ) ;
#46549=EDGE_CURVE ( 'NONE', #4051, #1404, #16297, .T. ) ;
#46550=VECTOR ( 'NONE', #111, 1000.000000000000000 ) ;
#46552=ADVANCED_FACE ( 'NONE', ( #25146 ), #45129, .T. ) ;
#46553=DIRECTION ( 'NONE',  ( -0.9890401873221623674, 0.000000000000000000, -0.1476465640024917925 ) ) ;
#46555=DIRECTION ( 'NONE',  ( 0.000000000000000000, 1.000000000000000000, 0.000000000000000000 ) ) ;
#46556=VERTEX_POINT ( 'NONE', #36965 ) ;
#46557=ADVANCED_FACE ( 'NONE', ( #955 ), #33014, .T. ) ;
#46560=EDGE_CURVE ( 'NONE', #15815, #30216, #20945, .T. ) ;
#46561=FACE_OUTER_BOUND ( 'NONE', #26027, .T. ) ;
#46562=EDGE_LOOP ( 'NONE', ( #13873, #52031, #25544, #37830 ) ) ;
#46563=ORIENTED_EDGE ( 'NONE', *, *, #8285, .F. ) ;
#46564=EDGE_CURVE ( 'NONE', #44736, #35501, #710, .T. ) ;
#46565=ORIENTED_EDGE ( 'NONE', *, *, #11504, .F. ) ;
#46569=LINE ( 'NONE', #10553, #2843 ) ;
#46570=ORIENTED_EDGE ( 'NONE', *, *, #47198, .F. ) ;
#46572=PLANE ( 'NONE',  #4901 ) ;
#46573=CARTESIAN_POINT ( 'NONE',  ( -56.05401443572774411, -175.3837268820161057, 124.7702732086913073 ) ) ;
#46574=DIRECTION ( 'NONE',  ( 0.000000000000000000, 0.000000000000000000, 1.000000000000000000 ) ) ;
#46576=ORIENTED_EDGE ( 'NONE', *, *, #2036, .F. ) ;
#46577=VECTOR ( 'NONE', #29383, 999.9999999999998863 ) ;
#46582=ORIENTED_EDGE ( 'NONE', *, *, #17856, .F. ) ;
#46584=CARTESIAN_POINT ( 'NONE',  ( -48.47912675150885065, -177.1207230881787780, 6.938893903907228378E-15 ) ) ;
#46586=DIRECTION ( 'NONE',  ( 0.000000000000000000, 0.000000000000000000, -1.000000000000000000 ) ) ;
#46587=EDGE_CURVE ( 'NONE', #2175, #11425, #36423, .T. ) ;
#46588=EDGE_LOOP ( 'NONE', ( #3191, #50788, #31634, #16906 ) ) ;
#46589=LINE ( 'NONE', #46334, #25627 ) ;
#46590=FACE_OUTER_BOUND ( 'NONE', #8468, .T. ) ;
#46592=VECTOR ( 'NONE', #24393, 1000.000000000000000 ) ;
#46596=VERTEX_POINT ( 'NONE', #33280 ) ;
#46597=CARTESIAN_POINT ( 'NONE',  ( -114.9600645115007040, -177.1207230881787780, 105.8550183720738573 ) ) ;
#46600=ORIENTED_EDGE ( 'NONE', *, *, #5117, .F. ) ;
#46601=DIRECTION ( 'NONE',  ( -0.9266896074318291543, 0.000000000000000000, -0.3758275821142488260 ) ) ;
#46602=EDGE_LOOP ( 'NONE', ( #25086, #20864, #8448, #50079 ) ) ;
#46603=LINE ( 'NONE', #39222, #17241 ) ;
#46604=DIRECTION ( 'NONE',  ( 0.9890401873221654760, 0.000000000000000000, -0.1476465640024710868 ) ) ;
#46605=ORIENTED_EDGE ( 'NONE', *, *, #23689, .F. ) ;
#46606=EDGE_CURVE ( 'NONE', #25483, #13304, #39793, .T. ) ;
#46609=DIRECTION ( 'NONE',  ( -0.000000000000000000, 1.000000000000000000, -0.000000000000000000 ) ) ;
#46611=ORIENTED_EDGE ( 'NONE', *, *, #23924, .F. ) ;
#46613=EDGE_CURVE ( 'NONE', #24955, #17439, #41457, .T. ) ;
#46614=EDGE_LOOP ( 'NONE', ( #36016, #34903, #15171, #8371 ) ) ;
#46615=VECTOR ( 'NONE', #5307, 1000.000000000000000 ) ;
#46617=LINE ( 'NONE', #26371, #36069 ) ;
#46618=CARTESIAN_POINT ( 'NONE',  ( -63.09433862318517328, -175.3837268820161057, -124.1426420773539405 ) ) ;
#46620=AXIS2_PLACEMENT_3D ( 'NONE', #7592, #36219, #28064 ) ;
#46621=VECTOR ( 'NONE', #30552, 1000.000000000000000 ) ;
#46622=ORIENTED_EDGE ( 'NONE', *, *, #6736, .F. ) ;
#46625=LINE ( 'NONE', #30317, #38878 ) ;
#46628=VECTOR ( 'NONE', #10953, 1000.000000000000000 ) ;
#46631=CARTESIAN_POINT ( 'NONE',  ( -40.90423906728908321, -175.3837268820161057, -124.7702732086912363 ) ) ;
#46632=CARTESIAN_POINT ( 'NONE',  ( -101.0675409952199999, -193.5000000000000000, 113.3995532942341100 ) ) ;
#46634=DIRECTION ( 'NONE',  ( 0.2920567706369694982, 0.000000000000000000, 0.9564009842765243130 ) ) ;
#46636=CARTESIAN_POINT ( 'NONE',  ( -99.62791064391784346, -189.7472609257535510, -114.0561348912352173 ) ) ;
#46639=ADVANCED_FACE ( 'NONE', ( #3772 ), #12682, .T. ) ;
#46640=ORIENTED_EDGE ( 'NONE', *, *, #29236, .F. ) ;
#46641=CIRCLE ( 'NONE', #14752, 124.9999999999999858 ) ;
#46642=DIRECTION ( 'NONE',  ( 0.000000000000000000, 0.000000000000000000, -1.000000000000000000 ) ) ;
#46645=CARTESIAN_POINT ( 'NONE',  ( -136.1415351158078693, -193.5000000000000000, -89.10837311819173578 ) ) ;
#46652=CARTESIAN_POINT ( 'NONE',  ( 72.31641062551800303, -189.7472609257535510, 32.14713283941990341 ) ) ;
#46653=VECTOR ( 'NONE', #23191, 1000.000000000000000 ) ;
#46654=CIRCLE ( 'NONE', #36539, 125.0000000000000000 ) ;
#46655=DIRECTION ( 'NONE',  ( 0.9473263538541899509, 0.000000000000000000, 0.3202698538628415692 ) ) ;
#46656=DIRECTION ( 'NONE',  ( 0.000000000000000000, -0.000000000000000000, 1.000000000000000000 ) ) ;
#46657=EDGE_LOOP ( 'NONE', ( #22898, #41003, #20966, #50560 ) ) ;
#46658=CARTESIAN_POINT ( 'NONE',  ( -47.97059563285962724, -177.1207230881787780, -0.8610436117673480050 ) ) ;
#46660=FACE_OUTER_BOUND ( 'NONE', #28484, .T. ) ;
#46661=VECTOR ( 'NONE', #48915, 1000.000000000000000 ) ;
#46663=ORIENTED_EDGE ( 'NONE', *, *, #18815, .F. ) ;
#46664=FACE_OUTER_BOUND ( 'NONE', #2292, .T. ) ;
#46665=LINE ( 'NONE', #42449, #345 ) ;
#46666=DIRECTION ( 'NONE',  ( -0.000000000000000000, 1.000000000000000000, -0.000000000000000000 ) ) ;
#46667=ADVANCED_FACE ( 'NONE', ( #48455 ), #3511, .F. ) ;
#46668=CIRCLE ( 'NONE', #45806, 125.0000000000000000 ) ;
#46669=CARTESIAN_POINT ( 'NONE',  ( -238.7407812814481076, -213.5000000000000000, -9.999999999999987566 ) ) ;
#46672=ORIENTED_EDGE ( 'NONE', *, *, #19191, .T. ) ;
#46673=DIRECTION ( 'NONE',  ( -0.000000000000000000, 1.000000000000000000, -0.000000000000000000 ) ) ;
#46674=ORIENTED_EDGE ( 'NONE', *, *, #2583, .T. ) ;
#46675=VERTEX_POINT ( 'NONE', #12160 ) ;
#46676=DIRECTION ( 'NONE',  ( -0.4566292373937200777, 0.000000000000000000, 0.8896570909947436601 ) ) ;
#46677=ORIENTED_EDGE ( 'NONE', *, *, #12317, .T. ) ;
#46678=LINE ( 'NONE', #38772, #20951 ) ;
#46679=VECTOR ( 'NONE', #3354, 1000.000000000000000 ) ;
#46680=VECTOR ( 'NONE', #36171, 1000.000000000000000 ) ;
#46684=ADVANCED_FACE ( 'NONE', ( #43972 ), #23747, .T. ) ;
#46685=ORIENTED_EDGE ( 'NONE', *, *, #23100, .F. ) ;
#46686=DIRECTION ( 'NONE',  ( 0.000000000000000000, -0.000000000000000000, 1.000000000000000000 ) ) ;
#46687=AXIS2_PLACEMENT_3D ( 'NONE', #50997, #30482, #14994 ) ;
#46688=AXIS2_PLACEMENT_3D ( 'NONE', #32350, #11858, #7917 ) ;
#46695=CARTESIAN_POINT ( 'NONE',  ( -171.4559849729830603, -193.5000000000000000, 22.39848972532369942 ) ) ;
#46696=VECTOR ( 'NONE', #24798, 1000.000000000000000 ) ;
#46697=AXIS2_PLACEMENT_3D ( 'NONE', #1339, #25779, #33911 ) ;
#46698=CARTESIAN_POINT ( 'NONE',  ( -103.4012653778457462, -193.5000000000000000, -112.2878385610366649 ) ) ;
#46699=VECTOR ( 'NONE', #8909, 1000.000000000000000 ) ;
#46701=VECTOR ( 'NONE', #38572, 1000.000000000000000 ) ;
#46702=CARTESIAN_POINT ( 'NONE',  ( -30.31202594373734627, -177.1207230881787780, -123.6727797384705809 ) ) ;
#46705=AXIS2_PLACEMENT_3D ( 'NONE', #42298, #30479, #2100 ) ;
#46707=CARTESIAN_POINT ( 'NONE',  ( -48.47912675150885065, -189.7472609257535510, 6.938893903907228378E-15 ) ) ;
#46708=ORIENTED_EDGE ( 'NONE', *, *, #14336, .F. ) ;
#46709=CARTESIAN_POINT ( 'NONE',  ( -48.47912675150885065, -177.1207230881787780, 6.938893903907228378E-15 ) ) ;
#46711=ORIENTED_EDGE ( 'NONE', *, *, #39173, .F. ) ;
#46712=FACE_OUTER_BOUND ( 'NONE', #44873, .T. ) ;
#46713=ORIENTED_EDGE ( 'NONE', *, *, #21870, .F. ) ;
#46714=CYLINDRICAL_SURFACE ( 'NONE', #21277, 125.0000000000000000 ) ;
#46717=LINE ( 'NONE', #35135, #20832 ) ;
#46718=ORIENTED_EDGE ( 'NONE', *, *, #31716, .T. ) ;
#46721=DIRECTION ( 'NONE',  ( 0.6528221181905174975, 0.000000000000000000, 0.7575112421616236880 ) ) ;
#46722=CIRCLE ( 'NONE', #43381, 125.0000000000000000 ) ;
#46724=VECTOR ( 'NONE', #34504, 1000.000000000000000 ) ;
#46725=DIRECTION ( 'NONE',  ( 0.000000000000000000, -0.000000000000000000, -1.000000000000000000 ) ) ;
#46726=DIRECTION ( 'NONE',  ( -0.000000000000000000, 1.000000000000000000, -0.000000000000000000 ) ) ;
#46728=DIRECTION ( 'NONE',  ( -0.9995608365087940150, 0.000000000000000000, -0.02963332782257007206 ) ) ;
#46731=DIRECTION ( 'NONE',  ( 0.000000000000000000, 0.000000000000000000, 1.000000000000000000 ) ) ;
#46732=DIRECTION ( 'NONE',  ( 0.5586467658036476935, 0.000000000000000000, 0.8294056854502049880 ) ) ;
#46733=EDGE_CURVE ( 'NONE', #11828, #10147, #44501, .T. ) ;
#46736=DIRECTION ( 'NONE',  ( -0.000000000000000000, 1.000000000000000000, -0.000000000000000000 ) ) ;
#46740=CIRCLE ( 'NONE', #15678, 125.0000000000000000 ) ;
#46741=EDGE_CURVE ( 'NONE', #24085, #13319, #20579, .T. ) ;
#46742=AXIS2_PLACEMENT_3D ( 'NONE', #50229, #15244, #22349 ) ;
#46744=AXIS2_PLACEMENT_3D ( 'NONE', #29497, #1906, #29756 ) ;
#46745=VECTOR ( 'NONE', #10331, 1000.000000000000000 ) ;
#46746=DIRECTION ( 'NONE',  ( 0.8455960035018199594, 0.000000000000000000, 0.5338233779648003940 ) ) ;
#46749=AXIS2_PLACEMENT_3D ( 'NONE', #14313, #45858, #50324 ) ;
#46752=CARTESIAN_POINT ( 'NONE',  ( -26.20043062753591201, -189.7472609257535510, -122.9986166548862911 ) ) ;
#46753=PLANE ( 'NONE',  #49753 ) ;
#46754=EDGE_CURVE ( 'NONE', #50412, #19338, #32669, .T. ) ;
#46755=FACE_OUTER_BOUND ( 'NONE', #41343, .T. ) ;
#46758=PLANE ( 'NONE',  #39062 ) ;
#46759=VERTEX_POINT ( 'NONE', #27688 ) ;
#46760=CARTESIAN_POINT ( 'NONE',  ( 38.48673058372651923, -193.5000000000000000, 88.39086586114802913 ) ) ;
#46761=AXIS2_PLACEMENT_3D ( 'NONE', #20030, #40506, #12397 ) ;
#46763=CARTESIAN_POINT ( 'NONE',  ( -49.17567778057184569, -193.5000000000000000, -0.7175072570443327136 ) ) ;
#46764=CIRCLE ( 'NONE', #29947, 125.0000000000000000 ) ;
#46765=DIRECTION ( 'NONE',  ( 0.000000000000000000, 0.000000000000000000, 1.000000000000000000 ) ) ;
#46769=DIRECTION ( 'NONE',  ( -0.000000000000000000, 1.000000000000000000, -0.000000000000000000 ) ) ;
#46772=AXIS2_PLACEMENT_3D ( 'NONE', #12677, #28700, #45029 ) ;
#46774=CARTESIAN_POINT ( 'NONE',  ( -161.4184887245413904, -183.6283474603465606, 51.19472891551358629 ) ) ;
#46776=DIRECTION ( 'NONE',  ( 0.000000000000000000, 1.000000000000000000, 0.000000000000000000 ) ) ;
#46777=VERTEX_POINT ( 'NONE', #16130 ) ;
#46778=EDGE_CURVE ( 'NONE', #39629, #24186, #32146, .T. ) ;
#46779=ADVANCED_FACE ( 'NONE', ( #48190 ), #28194, .T. ) ;
#46780=AXIS2_PLACEMENT_3D ( 'NONE', #28181, #44230, #12931 ) ;
#46781=DIRECTION ( 'NONE',  ( -0.000000000000000000, -1.000000000000000000, 0.000000000000000000 ) ) ;
#46783=CARTESIAN_POINT ( 'NONE',  ( -48.47912675150885065, -183.6283474603465606, 6.938893903907228378E-15 ) ) ;
#46785=ORIENTED_EDGE ( 'NONE', *, *, #25356, .F. ) ;
#46786=CIRCLE ( 'NONE', #30007, 125.0000000000000000 ) ;
#46787=CYLINDRICAL_SURFACE ( 'NONE', #47530, 15.00000000000000000 ) ;
#46788=ORIENTED_EDGE ( 'NONE', *, *, #19086, .F. ) ;
#46790=CARTESIAN_POINT ( 'NONE',  ( -92.78132261338706144, -175.3837268820161057, -116.8859077982276631 ) ) ;
#46791=ORIENTED_EDGE ( 'NONE', *, *, #39121, .F. ) ;
#46793=CARTESIAN_POINT ( 'NONE',  ( -48.47912675150885065, -175.3837268820161057, 6.938893903907228378E-15 ) ) ;
#46794=CARTESIAN_POINT ( 'NONE',  ( 45.36094686508022988, -193.5000000000000000, -82.57748230379237953 ) ) ;
#46796=PLANE ( 'NONE',  #29911 ) ;
#46797=VERTEX_POINT ( 'NONE', #51885 ) ;
#46798=EDGE_CURVE ( 'NONE', #16397, #23451, #7722, .T. ) ;
#46800=DIRECTION ( 'NONE',  ( 0.000000000000000000, -1.000000000000000000, 0.000000000000000000 ) ) ;
#46801=ADVANCED_FACE ( 'NONE', ( #47928 ), #11907, .T. ) ;
#46802=CARTESIAN_POINT ( 'NONE',  ( 27.23560471289045992, -175.3837268820161057, 99.45993886622845537 ) ) ;
#46807=CARTESIAN_POINT ( 'NONE',  ( -172.4465090799742484, -189.7472609257535510, -2.844930291600662908 ) ) ;
#46808=DIRECTION ( 'NONE',  ( 0.000000000000000000, -1.000000000000000000, 0.000000000000000000 ) ) ;
#46810=AXIS2_PLACEMENT_3D ( 'NONE', #8535, #20367, #32196 ) ;
#46811=EDGE_CURVE ( 'NONE', #121, #40458, #41855, .T. ) ;
#46812=CARTESIAN_POINT ( 'NONE',  ( -121.5885020763900997, -193.5000000000000000, -101.3904297239420913 ) ) ;
#46815=AXIS2_PLACEMENT_3D ( 'NONE', #13527, #17217, #9077 ) ;
#46816=DIRECTION ( 'NONE',  ( -0.2635871660690783380, 0.000000000000000000, 0.9646355819083558547 ) ) ;
#46818=DIRECTION ( 'NONE',  ( -0.000000000000000000, 1.000000000000000000, -0.000000000000000000 ) ) ;
#46819=CARTESIAN_POINT ( 'NONE',  ( 74.68865188374466868, -177.1207230881787780, 14.34663989163627740 ) ) ;
#46821=ORIENTED_EDGE ( 'NONE', *, *, #1872, .T. ) ;
#46824=CARTESIAN_POINT ( 'NONE',  ( 40.71578595748725604, -183.6283474603465606, 86.14171647324928927 ) ) ;
#46827=ORIENTED_EDGE ( 'NONE', *, *, #50822, .F. ) ;
#46829=DIRECTION ( 'NONE',  ( 0.9266896074318291543, 0.000000000000000000, 0.3758275821142488260 ) ) ;
#46831=VERTEX_POINT ( 'NONE', #5871 ) ;
#46834=CARTESIAN_POINT ( 'NONE',  ( 75.78974234412359579, -183.6283474603465606, 13.49993235881449394 ) ) ;
#46835=VECTOR ( 'NONE', #3006, 1000.000000000000114 ) ;
#46837=DIRECTION ( 'NONE',  ( 0.08879589532292483933, 0.000000000000000000, 0.9960498426152178952 ) ) ;
#46838=ORIENTED_EDGE ( 'NONE', *, *, #11773, .F. ) ;
#46839=AXIS2_PLACEMENT_3D ( 'NONE', #35647, #51697, #15702 ) ;
#46840=CARTESIAN_POINT ( 'NONE',  ( 5.015379008610418410, -193.5000000000000000, -112.9749434763326690 ) ) ;
#46841=ORIENTED_EDGE ( 'NONE', *, *, #39617, .F. ) ;
#46842=CARTESIAN_POINT ( 'NONE',  ( -49.21696003055058810, -193.5000000000000000, 0.6749830015182108900 ) ) ;
#46844=ORIENTED_EDGE ( 'NONE', *, *, #42744, .F. ) ;
#46845=ADVANCED_FACE ( 'NONE', ( #37655 ), #33704, .F. ) ;
#46846=EDGE_CURVE ( 'NONE', #20850, #4823, #7071, .T. ) ;
#46847=ADVANCED_FACE ( 'NONE', ( #28968 ), #21097, .T. ) ;
#46850=FACE_OUTER_BOUND ( 'NONE', #33144, .T. ) ;
#46851=ORIENTED_EDGE ( 'NONE', *, *, #29945, .T. ) ;
#46853=VECTOR ( 'NONE', #7191, 1000.000000000000000 ) ;
#46854=EDGE_LOOP ( 'NONE', ( #21560, #10830, #26206, #405 ) ) ;
#46857=EDGE_LOOP ( 'NONE', ( #43855, #41444, #48571, #13418 ) ) ;
#46858=EDGE_CURVE ( 'NONE', #12980, #10123, #19658, .T. ) ;
#46859=CARTESIAN_POINT ( 'NONE',  ( -18.31235070009513777, -189.7472609257535510, 121.3052580173829824 ) ) ;
#46861=ORIENTED_EDGE ( 'NONE', *, *, #14759, .F. ) ;
#46863=EDGE_CURVE ( 'NONE', #4854, #11814, #45034, .T. ) ;
#46864=LINE ( 'NONE', #10848, #33165 ) ;
#46867=EDGE_LOOP ( 'NONE', ( #19599, #25899, #51478, #25343 ) ) ;
#46868=CARTESIAN_POINT ( 'NONE',  ( -147.8383830610225971, -177.1207230881787780, -74.18852968774183410 ) ) ;
#46871=CARTESIAN_POINT ( 'NONE',  ( -52.47502265695602119, -177.1207230881787780, -124.9361149384469485 ) ) ;
#46872=CARTESIAN_POINT ( 'NONE',  ( -151.9915035862630646, -183.6283474603465606, 70.07273251429430161 ) ) ;
#46875=DIRECTION ( 'NONE',  ( 0.000000000000000000, -0.000000000000000000, 1.000000000000000000 ) ) ;
#46877=LINE ( 'NONE', #27129, #45044 ) ;
#46878=EDGE_CURVE ( 'NONE', #19748, #33685, #41320, .T. ) ;
#46879=ORIENTED_EDGE ( 'NONE', *, *, #4844, .T. ) ;
#46881=AXIS2_PLACEMENT_3D ( 'NONE', #3989, #28138, #48133 ) ;
#46883=VECTOR ( 'NONE', #49673, 1000.000000000000000 ) ;
#46884=LINE ( 'NONE', #46359, #10190 ) ;
#46885=CARTESIAN_POINT ( 'NONE',  ( 36.84288420123322538, -177.1207230881787780, 91.35181687837501840 ) ) ;
#46886=CARTESIAN_POINT ( 'NONE',  ( -47.53180039765465636, -177.1207230881787780, -0.3202698538628280800 ) ) ;
#46887=EDGE_LOOP ( 'NONE', ( #20008, #29761, #43878, #44113 ) ) ;
#46888=AXIS2_PLACEMENT_3D ( 'NONE', #41246, #5535, #8946 ) ;
#46890=CARTESIAN_POINT ( 'NONE',  ( 72.71365293123227502, -177.1207230881787780, -30.61552143554913030 ) ) ;
#46892=CARTESIAN_POINT ( 'NONE',  ( 43.86477233319988756, -175.3837268820161057, -84.24728067915975771 ) ) ;
#46893=VECTOR ( 'NONE', #9919, 1000.000000000000000 ) ;
#46896=ORIENTED_EDGE ( 'NONE', *, *, #28500, .F. ) ;
#46897=PLANE ( 'NONE',  #6528 ) ;
#46898=DIRECTION ( 'NONE',  ( 0.000000000000000000, -1.000000000000000000, 0.000000000000000000 ) ) ;
#46899=CARTESIAN_POINT ( 'NONE',  ( -118.4380981977755880, -189.7472609257535510, -102.3804074221059892 ) ) ;
#46900=DIRECTION ( 'NONE',  ( 0.9982437317643210184, 0.000000000000000000, 0.05924062789372143423 ) ) ;
#46901=ORIENTED_EDGE ( 'NONE', *, *, #17028, .F. ) ;
#46902=ORIENTED_EDGE ( 'NONE', *, *, #30836, .T. ) ;
#46904=AXIS2_PLACEMENT_3D ( 'NONE', #49310, #45371, #9359 ) ;
#46907=LINE ( 'NONE', #10887, #30824 ) ;
#46909=FACE_OUTER_BOUND ( 'NONE', #35595, .T. ) ;
#46910=ORIENTED_EDGE ( 'NONE', *, *, #25745, .F. ) ;
#46911=EDGE_CURVE ( 'NONE', #4103, #18062, #8743, .T. ) ;
#46915=LINE ( 'NONE', #35069, #9759 ) ;
#46916=ADVANCED_FACE ( 'NONE', ( #29246 ), #45299, .T. ) ;
#46917=EDGE_CURVE ( 'NONE', #50927, #13015, #2934, .T. ) ;
#46918=VERTEX_POINT ( 'NONE', #34230 ) ;
#46921=CIRCLE ( 'NONE', #51129, 125.0000000000000000 ) ;
#46923=DIRECTION ( 'NONE',  ( -0.1182731709213660498, 0.000000000000000000, 0.9929810960135169173 ) ) ;
#46925=CARTESIAN_POINT ( 'NONE',  ( -139.0630283577175987, -183.6283474603465606, -86.13684908212449898 ) ) ;
#46926=AXIS2_PLACEMENT_3D ( 'NONE', #40651, #9400, #29098 ) ;
#46929=VERTEX_POINT ( 'NONE', #10829 ) ;
#46930=CARTESIAN_POINT ( 'NONE',  ( -25.55153130240594450, -189.7472609257535510, 122.8793122007210599 ) ) ;
#46932=FACE_OUTER_BOUND ( 'NONE', #6509, .T. ) ;
#46933=EDGE_CURVE ( 'NONE', #48929, #18230, #30280, .T. ) ;
#46934=CARTESIAN_POINT ( 'NONE',  ( -168.1386673294336163, -175.3837268820161057, 32.52067927015838222 ) ) ;
#46935=ORIENTED_EDGE ( 'NONE', *, *, #49093, .T. ) ;
#46936=CARTESIAN_POINT ( 'NONE',  ( -133.0671220150036334, -177.1207230881787780, -92.03190238880748097 ) ) ;
#46938=FACE_OUTER_BOUND ( 'NONE', #46854, .T. ) ;
#46939=CARTESIAN_POINT ( 'NONE',  ( -104.8182102393454045, -175.3837268820161057, 111.5836353223472912 ) ) ;
#46940=EDGE_CURVE ( 'NONE', #5804, #8278, #7140, .T. ) ;
#46942=CARTESIAN_POINT ( 'NONE',  ( -48.47912675150885065, -183.6283474603465606, 6.938893903907228378E-15 ) ) ;
#46943=ORIENTED_EDGE ( 'NONE', *, *, #22870, .T. ) ;
#46944=LINE ( 'NONE', #6732, #21441 ) ;
#46945=CARTESIAN_POINT ( 'NONE',  ( -47.78257572244585560, -193.5000000000000000, -0.7175072570443230546 ) ) ;
#46946=ORIENTED_EDGE ( 'NONE', *, *, #13677, .F. ) ;
#46947=ORIENTED_EDGE ( 'NONE', *, *, #34658, .T. ) ;
#46948=LINE ( 'NONE', #34327, #33841 ) ;
#46949=ORIENTED_EDGE ( 'NONE', *, *, #40407, .T. ) ;
#46950=DIRECTION ( 'NONE',  ( -0.000000000000000000, 1.000000000000000000, -0.000000000000000000 ) ) ;
#46951=ORIENTED_EDGE ( 'NONE', *, *, #38198, .T. ) ;
#46952=VECTOR ( 'NONE', #49141, 1000.000000000000114 ) ;
#46954=DIRECTION ( 'NONE',  ( 0.000000000000000000, 0.000000000000000000, 1.000000000000000000 ) ) ;
#46956=DIRECTION ( 'NONE',  ( 0.000000000000000000, -0.000000000000000000, -1.000000000000000000 ) ) ;
#46957=( GEOMETRIC_REPRESENTATION_CONTEXT ( 3 ) GLOBAL_UNCERTAINTY_ASSIGNED_CONTEXT ( ( #5409 ) ) GLOBAL_UNIT_ASSIGNED_CONTEXT ( ( #30388, #50908, #5730 ) ) REPRESENTATION_CONTEXT ( 'NONE', 'WORKASPACE' ) );
#46960=LINE ( 'NONE', #10683, #24038 ) ;
#46961=ORIENTED_EDGE ( 'NONE', *, *, #45210, .F. ) ;
#46962=ORIENTED_EDGE ( 'NONE', *, *, #11033, .F. ) ;
#46964=LINE ( 'NONE', #26183, #19200 ) ;
#46967=CARTESIAN_POINT ( 'NONE',  ( -75.48985759771373694, -177.1207230881787780, -122.0467960216648748 ) ) ;
#46968=FACE_OUTER_BOUND ( 'NONE', #51232, .T. ) ;
#46972=VECTOR ( 'NONE', #15122, 1000.000000000000114 ) ;
#46974=EDGE_LOOP ( 'NONE', ( #29507, #23346, #50573, #39603 ) ) ;
#46975=LINE ( 'NONE', #30928, #46628 ) ;
#46976=EDGE_LOOP ( 'NONE', ( #33325, #34567, #8853, #32015 ) ) ;
#46977=ORIENTED_EDGE ( 'NONE', *, *, #45312, .T. ) ;
#46980=LINE ( 'NONE', #11732, #33871 ) ;
#46981=FACE_OUTER_BOUND ( 'NONE', #40270, .T. ) ;
#46982=ORIENTED_EDGE ( 'NONE', *, *, #47073, .F. ) ;
#46983=CARTESIAN_POINT ( 'NONE',  ( 4.109287492203097081, -177.1207230881787780, -113.3995532942337121 ) ) ;
#46987=CARTESIAN_POINT ( 'NONE',  ( 42.10477485469927927, -177.1207230881787780, 86.13684908212515268 ) ) ;
#46988=ADVANCED_FACE ( 'NONE', ( #18715 ), #42628, .T. ) ;
#46989=CARTESIAN_POINT ( 'NONE',  ( 68.59638248015004081, -177.1207230881787780, -43.79868877201405297 ) ) ;
#46990=DIRECTION ( 'NONE',  ( 0.000000000000000000, 0.000000000000000000, 1.000000000000000000 ) ) ;
#46992=CARTESIAN_POINT ( 'NONE',  ( 76.37123734610607073, -183.6283474603465606, 6.114457023561876703 ) ) ;
#46993=LINE ( 'NONE', #22806, #37340 ) ;
#46994=LINE ( 'NONE', #42250, #5361 ) ;
#46995=FACE_OUTER_BOUND ( 'NONE', #47927, .T. ) ;
#46996=ORIENTED_EDGE ( 'NONE', *, *, #44336, .F. ) ;
#46997=DIRECTION ( 'NONE',  ( -0.000000000000000000, 1.000000000000000000, -0.000000000000000000 ) ) ;
#46998=CARTESIAN_POINT ( 'NONE',  ( -159.5526844214375615, -193.5000000000000000, 57.33816169485226055 ) ) ;
#46999=ADVANCED_FACE ( 'NONE', ( #19238 ), #34729, .T. ) ;
#47000=DIRECTION ( 'NONE',  ( -0.000000000000000000, 1.000000000000000000, -0.000000000000000000 ) ) ;
#47001=EDGE_LOOP ( 'NONE', ( #43719, #5722, #27484, #3721 ) ) ;
#47002=CARTESIAN_POINT ( 'NONE',  ( 55.91309001144629320, -183.6283474603465606, 68.75510947788671956 ) ) ;
#47003=CYLINDRICAL_SURFACE ( 'NONE', #45432, 124.9999999999999858 ) ;
#47004=ORIENTED_EDGE ( 'NONE', *, *, #28871, .F. ) ;
#47005=CYLINDRICAL_SURFACE ( 'NONE', #47256, 125.0000000000000000 ) ;
#47006=EDGE_CURVE ( 'NONE', #19975, #37889, #15044, .T. ) ;
#47008=VECTOR ( 'NONE', #2018, 1000.000000000000114 ) ;
#47009=AXIS2_PLACEMENT_3D ( 'NONE', #48748, #12718, #7506 ) ;
#47010=FACE_OUTER_BOUND ( 'NONE', #49694, .T. ) ;
#47011=FACE_BOUND ( 'NONE', #26061, .T. ) ;
#47014=VERTEX_POINT ( 'NONE', #6642 ) ;
#47015=EDGE_CURVE ( 'NONE', #39351, #8427, #17206, .T. ) ;
#47016=EDGE_LOOP ( 'NONE', ( #22180, #2268, #11304, #14567 ) ) ;
#47017=LINE ( 'NONE', #46760, #7426 ) ;
#47020=PLANE ( 'NONE',  #15857 ) ;
#47021=EDGE_CURVE ( 'NONE', #18124, #47386, #2068, .T. ) ;
#47023=CARTESIAN_POINT ( 'NONE',  ( -48.64924157374594671, -193.5000000000000000, 124.9998842437354227 ) ) ;
#47025=ORIENTED_EDGE ( 'NONE', *, *, #10528, .F. ) ;
#47027=CARTESIAN_POINT ( 'NONE',  ( -50.89116676070551648, -177.1207230881787780, 124.9767260852757147 ) ) ;
#47028=VERTEX_POINT ( 'NONE', #38150 ) ;
#47030=CARTESIAN_POINT ( 'NONE',  ( -144.6608085595393902, -193.5000000000000000, -78.26291788638665992 ) ) ;
#47036=EDGE_LOOP ( 'NONE', ( #17810, #370, #16946, #41118 ) ) ;
#47038=DIRECTION ( 'NONE',  ( -0.000000000000000000, 1.000000000000000000, -0.000000000000000000 ) ) ;
#47039=VERTEX_POINT ( 'NONE', #23180 ) ;
#47040=VERTEX_POINT ( 'NONE', #18206 ) ;
#47041=AXIS2_PLACEMENT_3D ( 'NONE', #28188, #40013, #51605 ) ;
#47042=VECTOR ( 'NONE', #18743, 1000.000000000000341 ) ;
#47043=DIRECTION ( 'NONE',  ( -0.000000000000000000, 1.000000000000000000, -0.000000000000000000 ) ) ;
#47044=VERTEX_POINT ( 'NONE', #39197 ) ;
#47045=LINE ( 'NONE', #39136, #33744 ) ;
#47046=LINE ( 'NONE', #10260, #10593 ) ;
#47047=ORIENTED_EDGE ( 'NONE', *, *, #29349, .F. ) ;
#47049=CARTESIAN_POINT ( 'NONE',  ( 28.62116745695381326, -193.5000000000000000, -97.11716833071837129 ) ) ;
#47050=CARTESIAN_POINT ( 'NONE',  ( -130.0559183202350084, -193.5000000000000000, -93.38753978496592367 ) ) ;
#47052=DIRECTION ( 'NONE',  ( 0.000000000000000000, -0.000000000000000000, 1.000000000000000000 ) ) ;
#47055=DIRECTION ( 'NONE',  ( 0.2348860457809842095, 0.000000000000000000, -0.9720229140804107493 ) ) ;
#47056=FACE_OUTER_BOUND ( 'NONE', #11572, .T. ) ;
#47057=DIRECTION ( 'NONE',  ( 0.000000000000000000, -0.000000000000000000, 1.000000000000000000 ) ) ;
#47058=VERTEX_POINT ( 'NONE', #36279 ) ;
#47060=CARTESIAN_POINT ( 'NONE',  ( 26.52087324849106054, -198.5000000000000000, -60.00000000000003553 ) ) ;
#47065=ORIENTED_EDGE ( 'NONE', *, *, #16233, .T. ) ;
#47067=FACE_OUTER_BOUND ( 'NONE', #20672, .T. ) ;
#47068=DIRECTION ( 'NONE',  ( 0.000000000000000000, 0.000000000000000000, -1.000000000000000000 ) ) ;
#47071=AXIS2_PLACEMENT_3D ( 'NONE', #45573, #17972, #26623 ) ;
#47072=ORIENTED_EDGE ( 'NONE', *, *, #49697, .T. ) ;
#47073=EDGE_CURVE ( 'NONE', #346, #10684, #47871, .T. ) ;
#47074=EDGE_CURVE ( 'NONE', #35097, #30216, #32328, .T. ) ;
#47079=VERTEX_POINT ( 'NONE', #23936 ) ;
#47081=CARTESIAN_POINT ( 'NONE',  ( -98.71382891444399377, -175.3837268820161057, -114.4616734920523555 ) ) ;
#47082=ADVANCED_FACE ( 'NONE', ( #32080 ), #7416, .T. ) ;
#47083=DIRECTION ( 'NONE',  ( -0.9995608365087942371, 0.000000000000000000, -0.02963332782256331357 ) ) ;
#47086=DIRECTION ( 'NONE',  ( 0.000000000000000000, 0.000000000000000000, -1.000000000000000000 ) ) ;
#47087=DIRECTION ( 'NONE',  ( -0.8294056854502090959, 0.000000000000000000, 0.5586467658036415873 ) ) ;
#47092=VECTOR ( 'NONE', #23799, 1000.000000000000000 ) ;
#47094=VERTEX_POINT ( 'NONE', #3977 ) ;
#47097=DIRECTION ( 'NONE',  ( -0.1182731709213523247, 0.000000000000000000, -0.9929810960135185827 ) ) ;
#47100=CARTESIAN_POINT ( 'NONE',  ( -1.230335819511596540, -177.1207230881787780, 115.7261930397108358 ) ) ;
#47103=ORIENTED_EDGE ( 'NONE', *, *, #5676, .F. ) ;
#47104=DIRECTION ( 'NONE',  ( 0.000000000000000000, 0.000000000000000000, 1.000000000000000000 ) ) ;
#47105=CARTESIAN_POINT ( 'NONE',  ( -45.06671089634843952, -193.5000000000000000, -124.9534129907280402 ) ) ;
#47106=VERTEX_POINT ( 'NONE', #20001 ) ;
#47108=AXIS2_PLACEMENT_3D ( 'NONE', #28417, #32106, #48151 ) ;
#47110=ORIENTED_EDGE ( 'NONE', *, *, #8208, .T. ) ;
#47112=CARTESIAN_POINT ( 'NONE',  ( 64.29733702426840125, -175.3837268820161057, 53.91167979418565892 ) ) ;
#47113=CIRCLE ( 'NONE', #41240, 125.0000000000000000 ) ;
#47114=VERTEX_POINT ( 'NONE', #20256 ) ;
#47116=ORIENTED_EDGE ( 'NONE', *, *, #23067, .T. ) ;
#47117=VECTOR ( 'NONE', #49005, 1000.000000000000000 ) ;
#47119=DIRECTION ( 'NONE',  ( 0.9960498426152165630, 0.000000000000000000, 0.08879589532293852283 ) ) ;
#47120=VERTEX_POINT ( 'NONE', #40474 ) ;
#47121=CARTESIAN_POINT ( 'NONE',  ( -135.4258661347518853, -175.3837268820161057, -89.80681772907007598 ) ) ;
#47123=CARTESIAN_POINT ( 'NONE',  ( -19.28375372365792728, -193.5000000000000000, 121.5427093402341541 ) ) ;
#47125=CIRCLE ( 'NONE', #21949, 125.0000000000000000 ) ;
#47126=DIRECTION ( 'NONE',  ( 0.000000000000000000, 0.000000000000000000, -1.000000000000000000 ) ) ;
#47128=DIRECTION ( 'NONE',  ( 0.000000000000000000, -1.000000000000000000, 0.000000000000000000 ) ) ;
#47129=EDGE_LOOP ( 'NONE', ( #17430, #40575, #347, #21159 ) ) ;
#47130=EDGE_CURVE ( 'NONE', #31203, #36752, #20511, .T. ) ;
#47131=ORIENTED_EDGE ( 'NONE', *, *, #4123, .T. ) ;
#47134=CARTESIAN_POINT ( 'NONE',  ( 76.31829002442924548, -177.1207230881787780, 7.113702696402420145 ) ) ;
#47135=EDGE_CURVE ( 'NONE', #14246, #44579, #11601, .T. ) ;
#47136=CARTESIAN_POINT ( 'NONE',  ( -48.47912675150885065, -183.6283474603465606, 6.938893903907228378E-15 ) ) ;
#47137=EDGE_LOOP ( 'NONE', ( #4586, #24536, #32145, #38851 ) ) ;
#47139=DIRECTION ( 'NONE',  ( 0.9995608365087946812, 0.000000000000000000, -0.02963332782254913048 ) ) ;
#47141=EDGE_LOOP ( 'NONE', ( #42291, #11477, #4112, #6526 ) ) ;
#47142=DIRECTION ( 'NONE',  ( -0.000000000000000000, 1.000000000000000000, -0.000000000000000000 ) ) ;
#47143=CARTESIAN_POINT ( 'NONE',  ( -49.13194886969938580, -177.1207230881787780, 0.7575112421616214675 ) ) ;
#47144=ADVANCED_FACE ( 'NONE', ( #3444 ), #7653, .T. ) ;
#47147=DIRECTION ( 'NONE',  ( 0.000000000000000000, 0.000000000000000000, 1.000000000000000000 ) ) ;
#47152=ADVANCED_FACE ( 'NONE', ( #23672 ), #43410, .T. ) ;
#47153=VECTOR ( 'NONE', #13972, 1000.000000000000114 ) ;
#47154=ORIENTED_EDGE ( 'NONE', *, *, #49004, .F. ) ;
#47157=LINE ( 'NONE', #51120, #18490 ) ;
#47158=FACE_OUTER_BOUND ( 'NONE', #592, .T. ) ;
#47159=EDGE_CURVE ( 'NONE', #49057, #49769, #13163, .T. ) ;
#47160=CARTESIAN_POINT ( 'NONE',  ( 23.54917025746144432, -193.5000000000000000, -100.9358816284410381 ) ) ;
#47162=EDGE_LOOP ( 'NONE', ( #2914, #36088, #24765, #20736 ) ) ;
#47163=EDGE_CURVE ( 'NONE', #16495, #16650, #9734, .T. ) ;
#47165=DIRECTION ( 'NONE',  ( -0.000000000000000000, 1.000000000000000000, -0.000000000000000000 ) ) ;
#47166=AXIS2_PLACEMENT_3D ( 'NONE', #38710, #11363, #34763 ) ;
#47168=VERTEX_POINT ( 'NONE', #5286 ) ;
#47169=AXIS2_PLACEMENT_3D ( 'NONE', #28577, #40390, #51537 ) ;
#47170=CARTESIAN_POINT ( 'NONE',  ( -168.4003408533108086, -177.1207230881787780, -35.26900067126612726 ) ) ;
#47171=CARTESIAN_POINT ( 'NONE',  ( -91.22542124915045747, -189.7472609257535510, 117.4638425504669783 ) ) ;
#47175=VERTEX_POINT ( 'NONE', #17636 ) ;
#47176=DIRECTION ( 'NONE',  ( -0.9890401873221633666, 0.000000000000000000, -0.1476465640024850756 ) ) ;
#47177=EDGE_CURVE ( 'NONE', #14469, #51370, #44697, .T. ) ;
#47178=ORIENTED_EDGE ( 'NONE', *, *, #904, .F. ) ;
#47179=CARTESIAN_POINT ( 'NONE',  ( -173.2765435274470178, -193.5000000000000000, -7.113702696401505321 ) ) ;
#47181=ORIENTED_EDGE ( 'NONE', *, *, #34784, .T. ) ;
#47183=FACE_OUTER_BOUND ( 'NONE', #25676, .T. ) ;
#47185=CARTESIAN_POINT ( 'NONE',  ( -111.3295483157475729, -189.7472609257535510, 108.0501018472332362 ) ) ;
#47186=CIRCLE ( 'NONE', #25347, 125.0000000000000000 ) ;
#47187=CARTESIAN_POINT ( 'NONE',  ( 8.750818922897911634, -175.3837268820161057, -111.1293539894138576 ) ) ;
#47188=AXIS2_PLACEMENT_3D ( 'NONE', #48631, #12603, #28623 ) ;
#47189=DIRECTION ( 'NONE',  ( -0.2348860457809911206, 0.000000000000000000, 0.9720229140804089729 ) ) ;
#47191=ORIENTED_EDGE ( 'NONE', *, *, #50706, .F. ) ;
#47193=PLANE ( 'NONE',  #6132 ) ;
#47194=ORIENTED_EDGE ( 'NONE', *, *, #1926, .T. ) ;
#47195=EDGE_CURVE ( 'NONE', #29294, #27708, #25553, .T. ) ;
#47196=EDGE_CURVE ( 'NONE', #43465, #3202, #49682, .T. ) ;
#47198=EDGE_CURVE ( 'NONE', #43364, #32964, #810, .T. ) ;
#47200=ADVANCED_FACE ( 'NONE', ( #24723 ), #29432, .T. ) ;
#47201=ORIENTED_EDGE ( 'NONE', *, *, #23417, .T. ) ;
#47204=EDGE_CURVE ( 'NONE', #49045, #14293, #377, .T. ) ;
#47206=VECTOR ( 'NONE', #25285, 1000.000000000000000 ) ;
#47207=ORIENTED_EDGE ( 'NONE', *, *, #26836, .T. ) ;
#47212=PLANE ( 'NONE',  #32509 ) ;
#47213=EDGE_CURVE ( 'NONE', #23398, #42501, #36815, .T. ) ;
#47215=FACE_OUTER_BOUND ( 'NONE', #10385, .T. ) ;
#47216=ORIENTED_EDGE ( 'NONE', *, *, #5473, .T. ) ;
#47217=ORIENTED_EDGE ( 'NONE', *, *, #15342, .T. ) ;
#47218=EDGE_CURVE ( 'NONE', #2378, #32936, #37062, .T. ) ;
#47219=VERTEX_POINT ( 'NONE', #21573 ) ;
#47221=PLANE ( 'NONE',  #27669 ) ;
#47222=ADVANCED_FACE ( 'NONE', ( #49168 ), #12623, .F. ) ;
#47224=DIRECTION ( 'NONE',  ( -0.2635871660690648488, 0.000000000000000000, -0.9646355819083595184 ) ) ;
#47227=ORIENTED_EDGE ( 'NONE', *, *, #3849, .T. ) ;
#47228=EDGE_CURVE ( 'NONE', #28733, #48345, #45717, .T. ) ;
#47229=EDGE_CURVE ( 'NONE', #41296, #37599, #8784, .T. ) ;
#47230=AXIS2_PLACEMENT_3D ( 'NONE', #6350, #26051, #2130 ) ;
#47231=DIRECTION ( 'NONE',  ( 0.000000000000000000, -0.000000000000000000, -1.000000000000000000 ) ) ;
#47233=CARTESIAN_POINT ( 'NONE',  ( 61.38599058177058510, -175.3837268820161057, 59.62093586438192716 ) ) ;
#47234=ORIENTED_EDGE ( 'NONE', *, *, #2224, .T. ) ;
#47235=ORIENTED_EDGE ( 'NONE', *, *, #18255, .T. ) ;
#47236=DIRECTION ( 'NONE',  ( -0.000000000000000000, 1.000000000000000000, -0.000000000000000000 ) ) ;
#47237=DIRECTION ( 'NONE',  ( -0.4300652022765183435, 0.000000000000000000, -0.9027978299657446470 ) ) ;
#47238=CARTESIAN_POINT ( 'NONE',  ( -1.771278280434267272, -193.5000000000000000, -115.9455772817710226 ) ) ;
#47239=CARTESIAN_POINT ( 'NONE',  ( 24.15597040328004752, -193.5000000000000000, -101.7307360698543874 ) ) ;
#47240=VERTEX_POINT ( 'NONE', #1057 ) ;
#47241=LINE ( 'NONE', #27511, #25860 ) ;
#47243=VECTOR ( 'NONE', #17025, 1000.000000000000114 ) ;
#47245=EDGE_CURVE ( 'NONE', #3854, #9931, #25500, .T. ) ;
#47246=ORIENTED_EDGE ( 'NONE', *, *, #51636, .F. ) ;
#47247=DIRECTION ( 'NONE',  ( 0.000000000000000000, -1.000000000000000000, 0.000000000000000000 ) ) ;
#47248=AXIS2_PLACEMENT_3D ( 'NONE', #25913, #34316, #25398 ) ;
#47251=VERTEX_POINT ( 'NONE', #37324 ) ;
#47252=LINE ( 'NONE', #46992, #29905 ) ;
#47253=CARTESIAN_POINT ( 'NONE',  ( -172.1767935149754294, -177.1207230881787780, 8.665274887906315726 ) ) ;
#47254=LINE ( 'NONE', #6265, #12044 ) ;
#47255=CARTESIAN_POINT ( 'NONE',  ( 55.91309001144629320, -193.5000000000000000, 68.75510947788671956 ) ) ;
#47256=AXIS2_PLACEMENT_3D ( 'NONE', #38327, #2343, #34637 ) ;
#47257=ORIENTED_EDGE ( 'NONE', *, *, #12121, .T. ) ;
#47258=CARTESIAN_POINT ( 'NONE',  ( 48.47907891923915003, -175.3837268820161057, 78.89300572996906169 ) ) ;
#47262=CARTESIAN_POINT ( 'NONE',  ( 38.46761263173350187, -189.7472609257535510, 89.80681772907071547 ) ) ;
#47264=FACE_OUTER_BOUND ( 'NONE', #24125, .T. ) ;
#47266=EDGE_LOOP ( 'NONE', ( #47720, #6904, #46663, #21424 ) ) ;
#47268=DIRECTION ( 'NONE',  ( -0.000000000000000000, 1.000000000000000000, -0.000000000000000000 ) ) ;
#47269=EDGE_LOOP ( 'NONE', ( #26975, #37341, #9691, #36334 ) ) ;
#47272=FACE_BOUND ( 'NONE', #44763, .T. ) ;
#47274=ORIENTED_EDGE ( 'NONE', *, *, #45643, .T. ) ;
#47275=LINE ( 'NONE', #23357, #49577 ) ;
#47276=VECTOR ( 'NONE', #8398, 1000.000000000000114 ) ;
#47277=AXIS2_PLACEMENT_3D ( 'NONE', #50625, #23019, #46954 ) ;
#47278=ORIENTED_EDGE ( 'NONE', *, *, #4364, .T. ) ;
#47282=ORIENTED_EDGE ( 'NONE', *, *, #30773, .F. ) ;
#47284=DIRECTION ( 'NONE',  ( 0.000000000000000000, 1.000000000000000000, -0.000000000000000000 ) ) ;
#47285=VECTOR ( 'NONE', #3305, 1000.000000000000114 ) ;
#47286=EDGE_CURVE ( 'NONE', #28978, #3704, #18029, .T. ) ;
#47288=ORIENTED_EDGE ( 'NONE', *, *, #36863, .F. ) ;
#47290=CARTESIAN_POINT ( 'NONE',  ( -49.32472275501067571, -193.5000000000000000, -0.5338233779647935107 ) ) ;
#47294=LINE ( 'NONE', #24158, #48260 ) ;
#47296=VERTEX_POINT ( 'NONE', #18139 ) ;
#47297=DIRECTION ( 'NONE',  ( -0.000000000000000000, 1.000000000000000000, -0.000000000000000000 ) ) ;
#47299=DIRECTION ( 'NONE',  ( -0.8124868780056783146, 0.000000000000000000, -0.5829794791144762289 ) ) ;
#47301=ORIENTED_EDGE ( 'NONE', *, *, #48027, .T. ) ;
#47302=VECTOR ( 'NONE', #18953, 1000.000000000000000 ) ;
#47303=LINE ( 'NONE', #47562, #41625 ) ;
#47304=VERTEX_POINT ( 'NONE', #30987 ) ;
#47306=DIRECTION ( 'NONE',  ( -0.000000000000000000, 1.000000000000000000, -0.000000000000000000 ) ) ;
#47307=EDGE_LOOP ( 'NONE', ( #51943, #36823, #27590, #47116 ) ) ;
#47310=LINE ( 'NONE', #34181, #31596 ) ;
#47312=EDGE_LOOP ( 'NONE', ( #27598, #40610, #9016, #35677 ) ) ;
#47315=DIRECTION ( 'NONE',  ( 0.000000000000000000, -1.000000000000000000, 0.000000000000000000 ) ) ;
#47316=CARTESIAN_POINT ( 'NONE',  ( -48.47912675150885065, -177.1207230881787780, 6.938893903907228378E-15 ) ) ;
#47317=LINE ( 'NONE', #3668, #2766 ) ;
#47318=ORIENTED_EDGE ( 'NONE', *, *, #27276, .F. ) ;
#47320=CARTESIAN_POINT ( 'NONE',  ( -48.47912675150885065, -175.3837268820161057, 6.938893903907228378E-15 ) ) ;
#47322=FACE_OUTER_BOUND ( 'NONE', #36122, .T. ) ;
#47324=ORIENTED_EDGE ( 'NONE', *, *, #27305, .T. ) ;
#47325=EDGE_CURVE ( 'NONE', #5817, #1492, #7081, .T. ) ;
#47327=CARTESIAN_POINT ( 'NONE',  ( -157.5429198988176438, -189.7472609257535510, 61.07445476073478829 ) ) ;
#47328=CARTESIAN_POINT ( 'NONE',  ( -48.47912675150885065, -189.7472609257535510, 125.0000000000000000 ) ) ;
#47329=DIRECTION ( 'NONE',  ( 0.000000000000000000, 0.000000000000000000, 1.000000000000000000 ) ) ;
#47330=FACE_OUTER_BOUND ( 'NONE', #32420, .T. ) ;
#47331=CIRCLE ( 'NONE', #38908, 125.0000000000000000 ) ;
#47332=ORIENTED_EDGE ( 'NONE', *, *, #35536, .F. ) ;
#47336=VERTEX_POINT ( 'NONE', #38360 ) ;
#47337=EDGE_LOOP ( 'NONE', ( #19613, #17833, #47533, #48433 ) ) ;
#47340=CARTESIAN_POINT ( 'NONE',  ( -66.46933728415694986, -183.6283474603465606, 122.6885491605231380 ) ) ;
#47341=VECTOR ( 'NONE', #48583, 1000.000000000000114 ) ;
#47342=EDGE_LOOP ( 'NONE', ( #21449, #4670, #50851, #6230 ) ) ;
#47345=DIRECTION ( 'NONE',  ( 0.000000000000000000, -1.000000000000000000, 0.000000000000000000 ) ) ;
#47346=CARTESIAN_POINT ( 'NONE',  ( -48.47912675150885065, -177.1207230881787780, 6.938893903907228378E-15 ) ) ;
#47347=ORIENTED_EDGE ( 'NONE', *, *, #5444, .F. ) ;
#47348=CARTESIAN_POINT ( 'NONE',  ( -48.47912675150885065, -189.7472609257535510, 6.938893903907228378E-15 ) ) ;
#47349=ORIENTED_EDGE ( 'NONE', *, *, #14510, .T. ) ;
#47350=CARTESIAN_POINT ( 'NONE',  ( 50.70030191143631271, -193.5000000000000000, -76.08180419845318454 ) ) ;
#47352=DIRECTION ( 'NONE',  ( 0.000000000000000000, 0.000000000000000000, -1.000000000000000000 ) ) ;
#47354=FACE_OUTER_BOUND ( 'NONE', #35638, .T. ) ;
#47355=CARTESIAN_POINT ( 'NONE',  ( 9.518239912201957864, -213.5000000000000000, -110.7307791902283043 ) ) ;
#47358=VERTEX_POINT ( 'NONE', #42560 ) ;
#47359=DIRECTION ( 'NONE',  ( -0.9564009842765264224, 0.000000000000000000, 0.2920567706369628924 ) ) ;
#47360=ORIENTED_EDGE ( 'NONE', *, *, #32929, .F. ) ;
#47361=PLANE ( 'NONE',  #19864 ) ;
#47362=AXIS2_PLACEMENT_3D ( 'NONE', #25824, #1116, #5609 ) ;
#47365=EDGE_CURVE ( 'NONE', #13363, #18053, #30469, .T. ) ;
#47366=VERTEX_POINT ( 'NONE', #14205 ) ;
#47368=FACE_OUTER_BOUND ( 'NONE', #23728, .T. ) ;
#47369=AXIS2_PLACEMENT_3D ( 'NONE', #44003, #4074, #20092 ) ;
#47370=EDGE_CURVE ( 'NONE', #8060, #4209, #34668, .T. ) ;
#47371=PLANE ( 'NONE',  #44215 ) ;
#47372=ORIENTED_EDGE ( 'NONE', *, *, #47987, .F. ) ;
#47375=DIRECTION ( 'NONE',  ( 0.000000000000000000, 0.000000000000000000, -1.000000000000000000 ) ) ;
#47376=CARTESIAN_POINT ( 'NONE',  ( -154.6193097927903182, -175.3837268820161057, -66.02470404298122730 ) ) ;
#47377=FACE_OUTER_BOUND ( 'NONE', #32707, .T. ) ;
#47378=EDGE_CURVE ( 'NONE', #13340, #48355, #4590, .T. ) ;
#47379=VECTOR ( 'NONE', #9344, 1000.000000000000000 ) ;
#47380=EDGE_CURVE ( 'NONE', #26396, #18665, #30222, .T. ) ;
#47381=DIRECTION ( 'NONE',  ( 0.000000000000000000, -1.000000000000000000, 0.000000000000000000 ) ) ;
#47383=DIRECTION ( 'NONE',  ( -0.8757349421956345248, 0.000000000000000000, -0.4827922027307490205 ) ) ;
#47385=LINE ( 'NONE', #43447, #35401 ) ;
#47386=VERTEX_POINT ( 'NONE', #22072 ) ;
#47387=EDGE_LOOP ( 'NONE', ( #41407, #28887, #9218, #29566 ) ) ;
#47388=CARTESIAN_POINT ( 'NONE',  ( -48.47912675150885065, -183.6283474603465606, 6.938893903907228378E-15 ) ) ;
#47389=CARTESIAN_POINT ( 'NONE',  ( -172.0839188101925004, -175.3837268820161057, -18.62405380494756812 ) ) ;
#47391=EDGE_LOOP ( 'NONE', ( #18412, #30996, #15274, #5517 ) ) ;
#47398=CIRCLE ( 'NONE', #2069, 125.0000000000000000 ) ;
#47399=PLANE ( 'NONE',  #33654 ) ;
#47400=CARTESIAN_POINT ( 'NONE',  ( 7.991501969728822985, -175.3837268820161057, 110.3950557015152754 ) ) ;
#47401=EDGE_LOOP ( 'NONE', ( #3361, #50535, #10404, #35071 ) ) ;
#47403=AXIS2_PLACEMENT_3D ( 'NONE', #22687, #10338, #50552 ) ;
#47405=FACE_OUTER_BOUND ( 'NONE', #21181, .T. ) ;
#47406=DIRECTION ( 'NONE',  ( 0.000000000000000000, -1.000000000000000000, 0.000000000000000000 ) ) ;
#47408=PLANE ( 'NONE',  #12997 ) ;
#47409=ORIENTED_EDGE ( 'NONE', *, *, #50203, .F. ) ;
#47413=PLANE ( 'NONE',  #34092 ) ;
#47414=VERTEX_POINT ( 'NONE', #10763 ) ;
#47415=ORIENTED_EDGE ( 'NONE', *, *, #29856, .F. ) ;
#47416=CARTESIAN_POINT ( 'NONE',  ( -62.43888699632653783, -193.5000000000000000, 124.2180546213279371 ) ) ;
#47417=LINE ( 'NONE', #38229, #30846 ) ;
#47418=ORIENTED_EDGE ( 'NONE', *, *, #20678, .F. ) ;
#47420=DIRECTION ( 'NONE',  ( 0.000000000000000000, -1.000000000000000000, 0.000000000000000000 ) ) ;
#47421=EDGE_CURVE ( 'NONE', #34513, #1466, #35642, .T. ) ;
#47422=EDGE_CURVE ( 'NONE', #50178, #43983, #37300, .T. ) ;
#47425=DIRECTION ( 'NONE',  ( -0.000000000000000000, 1.000000000000000000, -0.000000000000000000 ) ) ;
#47426=ORIENTED_EDGE ( 'NONE', *, *, #33191, .F. ) ;
#47428=FACE_BOUND ( 'NONE', #25448, .T. ) ;
#47430=LINE ( 'NONE', #31911, #13491 ) ;
#47431=ORIENTED_EDGE ( 'NONE', *, *, #17913, .T. ) ;
#47432=AXIS2_PLACEMENT_3D ( 'NONE', #45952, #35073, #31123 ) ;
#47433=AXIS2_PLACEMENT_3D ( 'NONE', #13763, #12526, #10333 ) ;
#47436=DIRECTION ( 'NONE',  ( 0.7378332790417239107, 0.000000000000000000, 0.6749830015182142207 ) ) ;
#47437=EDGE_CURVE ( 'NONE', #19237, #47120, #26524, .T. ) ;
#47438=CARTESIAN_POINT ( 'NONE',  ( 25.43954814678888710, -193.5000000000000000, 100.8019320314832754 ) ) ;
#47440=EDGE_CURVE ( 'NONE', #40906, #39314, #38867, .T. ) ;
#47444=EDGE_CURVE ( 'NONE', #18213, #36857, #7138, .T. ) ;
#47445=AXIS2_PLACEMENT_3D ( 'NONE', #2303, #43536, #30652 ) ;
#47446=LINE ( 'NONE', #50879, #28132 ) ;
#47448=VERTEX_POINT ( 'NONE', #3136 ) ;
#47451=ORIENTED_EDGE ( 'NONE', *, *, #46495, .F. ) ;
#47452=CARTESIAN_POINT ( 'NONE',  ( -52.47502265695602119, -193.5000000000000000, -124.9361149384469485 ) ) ;
#47453=AXIS2_PLACEMENT_3D ( 'NONE', #39441, #16067, #3442 ) ;
#47454=AXIS2_PLACEMENT_3D ( 'NONE', #5537, #49933, #21562 ) ;
#47455=LINE ( 'NONE', #50372, #39378 ) ;
#47456=EDGE_LOOP ( 'NONE', ( #9840, #48213, #51156, #25823 ) ) ;
#47457=DIRECTION ( 'NONE',  ( -0.000000000000000000, 1.000000000000000000, -0.000000000000000000 ) ) ;
#47458=LINE ( 'NONE', #13208, #47206 ) ;
#47459=ORIENTED_EDGE ( 'NONE', *, *, #18840, .F. ) ;
#47460=CARTESIAN_POINT ( 'NONE',  ( -47.47956591500005885, -193.5000000000000000, 0.02963332782257025594 ) ) ;
#47462=LINE ( 'NONE', #4346, #31607 ) ;
#47464=ORIENTED_EDGE ( 'NONE', *, *, #15115, .T. ) ;
#47467=CARTESIAN_POINT ( 'NONE',  ( -54.99637373343401237, -189.7472609257535510, 123.8286356280830773 ) ) ;
#47469=PLANE ( 'NONE',  #51168 ) ;
#47470=AXIS2_PLACEMENT_3D ( 'NONE', #51307, #23450, #51065 ) ;
#47471=FACE_OUTER_BOUND ( 'NONE', #44117, .T. ) ;
#47472=FACE_OUTER_BOUND ( 'NONE', #45673, .T. ) ;
#47473=VERTEX_POINT ( 'NONE', #33894 ) ;
#47474=AXIS2_PLACEMENT_3D ( 'NONE', #43373, #27061, #30497 ) ;
#47475=CARTESIAN_POINT ( 'NONE',  ( -12.42681898335384894, -193.5000000000000000, 118.6432945265039365 ) ) ;
#47476=ADVANCED_FACE ( 'NONE', ( #13938 ), #46015, .T. ) ;
#47477=VERTEX_POINT ( 'NONE', #35972 ) ;
#47479=DIRECTION ( 'NONE',  ( 0.000000000000000000, 1.000000000000000000, 0.000000000000000000 ) ) ;
#47482=LINE ( 'NONE', #50653, #10699 ) ;
#47483=VECTOR ( 'NONE', #42566, 1000.000000000000000 ) ;
#47485=VECTOR ( 'NONE', #49580, 1000.000000000000000 ) ;
#47486=ADVANCED_FACE ( 'NONE', ( #43340 ), #31774, .T. ) ;
#47489=EDGE_CURVE ( 'NONE', #9353, #23327, #1284, .T. ) ;
#47490=DIRECTION ( 'NONE',  ( 0.1768902751225733261, 0.000000000000000000, -0.9842305779475966077 ) ) ;
#47491=ORIENTED_EDGE ( 'NONE', *, *, #43319, .F. ) ;
#47492=DIRECTION ( 'NONE',  ( 0.000000000000000000, -1.000000000000000000, 0.000000000000000000 ) ) ;
#47493=AXIS2_PLACEMENT_3D ( 'NONE', #15487, #31497, #11534 ) ;
#47494=ORIENTED_EDGE ( 'NONE', *, *, #50203, .T. ) ;
#47496=CIRCLE ( 'NONE', #43282, 125.0000000000000000 ) ;
#47498=LINE ( 'NONE', #28286, #40512 ) ;
#47500=ADVANCED_FACE ( 'NONE', ( #39381 ), #23612, .T. ) ;
#47501=FACE_OUTER_BOUND ( 'NONE', #39649, .T. ) ;
#47503=LINE ( 'NONE', #22563, #14588 ) ;
#47504=LINE ( 'NONE', #26998, #45556 ) ;
#47505=EDGE_CURVE ( 'NONE', #39776, #20552, #47294, .T. ) ;
#47506=VERTEX_POINT ( 'NONE', #23375 ) ;
#47507=CARTESIAN_POINT ( 'NONE',  ( 59.29945538372742675, -183.6283474603465606, 63.31490529818493940 ) ) ;
#47509=EDGE_CURVE ( 'NONE', #36297, #47114, #19170, .T. ) ;
#47511=ORIENTED_EDGE ( 'NONE', *, *, #25402, .T. ) ;
#47512=CIRCLE ( 'NONE', #4701, 125.0000000000000000 ) ;
#47513=ADVANCED_FACE ( 'NONE', ( #19415 ), #40166, .F. ) ;
#47514=DIRECTION ( 'NONE',  ( 0.000000000000000000, 0.000000000000000000, -1.000000000000000000 ) ) ;
#47515=VECTOR ( 'NONE', #45497, 999.9999999999998863 ) ;
#47516=VECTOR ( 'NONE', #32296, 999.9999999999998863 ) ;
#47518=EDGE_CURVE ( 'NONE', #24853, #33118, #19943, .T. ) ;
#47519=ORIENTED_EDGE ( 'NONE', *, *, #127, .T. ) ;
#47520=DIRECTION ( 'NONE',  ( -0.000000000000000000, 1.000000000000000000, -0.000000000000000000 ) ) ;
#47522=EDGE_CURVE ( 'NONE', #32234, #32749, #48321, .T. ) ;
#47523=DIRECTION ( 'NONE',  ( 0.000000000000000000, 0.000000000000000000, 1.000000000000000000 ) ) ;
#47524=FACE_BOUND ( 'NONE', #35194, .T. ) ;
#47525=VECTOR ( 'NONE', #25594, 1000.000000000000000 ) ;
#47526=DIRECTION ( 'NONE',  ( -0.000000000000000000, 1.000000000000000000, -0.000000000000000000 ) ) ;
#47529=CIRCLE ( 'NONE', #31685, 125.0000000000000568 ) ;
#47530=AXIS2_PLACEMENT_3D ( 'NONE', #30233, #10773, #17646 ) ;
#47531=DIRECTION ( 'NONE',  ( -0.9982437317643214625, 0.000000000000000000, -0.05924062789371441901 ) ) ;
#47533=ORIENTED_EDGE ( 'NONE', *, *, #48210, .F. ) ;
#47534=EDGE_CURVE ( 'NONE', #10132, #32136, #13021, .T. ) ;
#47536=AXIS2_PLACEMENT_3D ( 'NONE', #870, #48715, #44249 ) ;
#47537=DIRECTION ( 'NONE',  ( 0.5085311186492094127, 0.000000000000000000, 0.8610436117673619938 ) ) ;
#47539=FACE_OUTER_BOUND ( 'NONE', #43545, .T. ) ;
#47541=DIRECTION ( 'NONE',  ( 0.8757349421956345248, 0.000000000000000000, 0.4827922027307490205 ) ) ;
#47542=ORIENTED_EDGE ( 'NONE', *, *, #51029, .T. ) ;
#47543=DIRECTION ( 'NONE',  ( -0.000000000000000000, 1.000000000000000000, -0.000000000000000000 ) ) ;
#47547=CIRCLE ( 'NONE', #28204, 125.0000000000000000 ) ;
#47548=DIRECTION ( 'NONE',  ( 0.000000000000000000, 0.000000000000000000, 1.000000000000000000 ) ) ;
#47549=ORIENTED_EDGE ( 'NONE', *, *, #861, .F. ) ;
#47550=DIRECTION ( 'NONE',  ( -0.2920567706369628924, 0.000000000000000000, -0.9564009842765264224 ) ) ;
#47553=ADVANCED_FACE ( 'NONE', ( #51238 ), #47812, .T. ) ;
#47554=EDGE_CURVE ( 'NONE', #2758, #45184, #43221, .T. ) ;
#47555=CARTESIAN_POINT ( 'NONE',  ( 42.10477485469927927, -183.6283474603465606, 86.13684908212515268 ) ) ;
#47557=DIRECTION ( 'NONE',  ( -0.000000000000000000, 1.000000000000000000, -0.000000000000000000 ) ) ;
#47562=CARTESIAN_POINT ( 'NONE',  ( -140.5933766095837427, -175.3837268820161057, -84.49831343337065448 ) ) ;
#47564=FACE_OUTER_BOUND ( 'NONE', #9480, .T. ) ;
#47565=CIRCLE ( 'NONE', #2242, 125.0000000000000000 ) ;
#47566=DIRECTION ( 'NONE',  ( 0.000000000000000000, 1.000000000000000000, 0.000000000000000000 ) ) ;
#47569=CARTESIAN_POINT ( 'NONE',  ( -47.51449116960048968, -189.7472609257535510, -0.2635871660690578544 ) ) ;
#47570=DIRECTION ( 'NONE',  ( 0.000000000000000000, 1.000000000000000000, -0.000000000000000000 ) ) ;
#47571=VECTOR ( 'NONE', #7305, 1000.000000000000000 ) ;
#47572=AXIS2_PLACEMENT_3D ( 'NONE', #34114, #41990, #17585 ) ;
#47573=CARTESIAN_POINT ( 'NONE',  ( -98.71382891444399377, -193.5000000000000000, -114.4616734920523555 ) ) ;
#47575=VECTOR ( 'NONE', #15604, 1000.000000000000000 ) ;
#47576=LINE ( 'NONE', #43866, #17136 ) ;
#47577=DIRECTION ( 'NONE',  ( -0.000000000000000000, 1.000000000000000000, -0.000000000000000000 ) ) ;
#47578=CIRCLE ( 'NONE', #32444, 125.0000000000000000 ) ;
#47580=VERTEX_POINT ( 'NONE', #1254 ) ;
#47582=ADVANCED_FACE ( 'NONE', ( #29631 ), #48595, .T. ) ;
#47583=PLANE ( 'NONE',  #18554 ) ;
#47584=LINE ( 'NONE', #3946, #9304 ) ;
#47585=CARTESIAN_POINT ( 'NONE',  ( -158.3442440847887269, -189.7472609257535510, -59.62093586438114556 ) ) ;
#47586=EDGE_LOOP ( 'NONE', ( #42954, #38196, #20785, #20933 ) ) ;
#47588=ORIENTED_EDGE ( 'NONE', *, *, #26340, .T. ) ;
#47589=ADVANCED_FACE ( 'NONE', ( #4966 ), #33331, .T. ) ;
#47590=VECTOR ( 'NONE', #15135, 1000.000000000000000 ) ;
#47591=DIRECTION ( 'NONE',  ( 0.000000000000000000, -1.000000000000000000, -0.000000000000000000 ) ) ;
#47592=VECTOR ( 'NONE', #51087, 1000.000000000000000 ) ;
#47593=LINE ( 'NONE', #32053, #40447 ) ;
#47596=VECTOR ( 'NONE', #2471, 1000.000000000000114 ) ;
#47597=ORIENTED_EDGE ( 'NONE', *, *, #8864, .T. ) ;
#47598=PLANE ( 'NONE',  #29370 ) ;
#47599=EDGE_LOOP ( 'NONE', ( #39118, #30962, #42205, #49037 ) ) ;
#47601=ORIENTED_EDGE ( 'NONE', *, *, #40903, .T. ) ;
#47603=ORIENTED_EDGE ( 'NONE', *, *, #18656, .T. ) ;
#47604=FACE_OUTER_BOUND ( 'NONE', #31137, .T. ) ;
#47605=VECTOR ( 'NONE', #48123, 1000.000000000000114 ) ;
#47606=CIRCLE ( 'NONE', #15726, 125.0000000000000000 ) ;
#47608=CIRCLE ( 'NONE', #9004, 125.0000000000000000 ) ;
#47609=ORIENTED_EDGE ( 'NONE', *, *, #35944, .T. ) ;
#47613=DIRECTION ( 'NONE',  ( -0.000000000000000000, 1.000000000000000000, 0.000000000000000000 ) ) ;
#47615=ORIENTED_EDGE ( 'NONE', *, *, #51649, .F. ) ;
#47616=LINE ( 'NONE', #12089, #18891 ) ;
#47619=ORIENTED_EDGE ( 'NONE', *, *, #51858, .T. ) ;
#47621=CARTESIAN_POINT ( 'NONE',  ( 63.31225588004632243, -183.6283474603465606, 55.92572546981597981 ) ) ;
#47626=LINE ( 'NONE', #11610, #14787 ) ;
#47629=ORIENTED_EDGE ( 'NONE', *, *, #18815, .T. ) ;
#47630=CARTESIAN_POINT ( 'NONE',  ( 18.49541618049842384, -183.6283474603465606, 105.5434062319798016 ) ) ;
#47631=VECTOR ( 'NONE', #24763, 1000.000000000000227 ) ;
#47632=DIRECTION ( 'NONE',  ( 0.000000000000000000, 0.000000000000000000, -1.000000000000000000 ) ) ;
#47634=CARTESIAN_POINT ( 'NONE',  ( -36.09284319799462537, -193.5000000000000000, 124.3848060646152618 ) ) ;
#47638=ORIENTED_EDGE ( 'NONE', *, *, #20431, .F. ) ;
#47639=LINE ( 'NONE', #20024, #9001 ) ;
#47640=VERTEX_POINT ( 'NONE', #24655 ) ;
#47641=VECTOR ( 'NONE', #48445, 1000.000000000000000 ) ;
#47642=DIRECTION ( 'NONE',  ( 0.000000000000000000, -0.000000000000000000, 1.000000000000000000 ) ) ;
#47643=AXIS2_PLACEMENT_3D ( 'NONE', #47346, #15541, #19470 ) ;
#47644=CARTESIAN_POINT ( 'NONE',  ( 51.65665342072241373, -183.6283474603465606, 74.81861753132420745 ) ) ;
#47646=AXIS2_PLACEMENT_3D ( 'NONE', #15437, #47237, #19367 ) ;
#47648=CYLINDRICAL_SURFACE ( 'NONE', #2073, 125.0000000000000000 ) ;
#47650=AXIS2_PLACEMENT_3D ( 'NONE', #47569, #31255, #34684 ) ;
#47651=DIRECTION ( 'NONE',  ( 0.000000000000000000, -1.000000000000000000, 0.000000000000000000 ) ) ;
#47656=ORIENTED_EDGE ( 'NONE', *, *, #36433, .F. ) ;
#47659=EDGE_CURVE ( 'NONE', #1035, #6177, #21245, .T. ) ;
#47660=CARTESIAN_POINT ( 'NONE',  ( 71.35177504360963496, -193.5000000000000000, 31.88354567335082734 ) ) ;
#47662=CIRCLE ( 'NONE', #49395, 124.9999999999999858 ) ;
#47663=VECTOR ( 'NONE', #47818, 1000.000000000000114 ) ;
#47665=DIRECTION ( 'NONE',  ( 0.000000000000000000, -1.000000000000000000, 0.000000000000000000 ) ) ;
#47666=ORIENTED_EDGE ( 'NONE', *, *, #9012, .T. ) ;
#47667=CARTESIAN_POINT ( 'NONE',  ( 37.77106160267051393, -189.7472609257535510, 89.08931047202638354 ) ) ;
#47669=CIRCLE ( 'NONE', #2350, 125.0000000000000000 ) ;
#47670=DIRECTION ( 'NONE',  ( 0.000000000000000000, -0.000000000000000000, -1.000000000000000000 ) ) ;
#47671=LINE ( 'NONE', #23732, #12356 ) ;
#47673=ORIENTED_EDGE ( 'NONE', *, *, #23706, .T. ) ;
#47675=EDGE_CURVE ( 'NONE', #15950, #33788, #25591, .T. ) ;
#47679=CARTESIAN_POINT ( 'NONE',  ( -140.8230258362169707, -175.3837268820161057, 84.24728067916045404 ) ) ;
#47680=DIRECTION ( 'NONE',  ( -0.000000000000000000, 1.000000000000000000, 0.000000000000000000 ) ) ;
#47682=CARTESIAN_POINT ( 'NONE',  ( -47.74129347246713451, -193.5000000000000000, 0.6749830015182212151 ) ) ;
#47684=CARTESIAN_POINT ( 'NONE',  ( -167.6453766917639427, -177.1207230881787780, 37.74128873232411507 ) ) ;
#47685=DIRECTION ( 'NONE',  ( 0.000000000000000000, 0.000000000000000000, -1.000000000000000000 ) ) ;
#47687=ORIENTED_EDGE ( 'NONE', *, *, #25960, .T. ) ;
#47688=ORIENTED_EDGE ( 'NONE', *, *, #32331, .F. ) ;
#47689=EDGE_CURVE ( 'NONE', #2646, #27986, #37264, .T. ) ;
#47690=EDGE_LOOP ( 'NONE', ( #42823, #50709, #51306, #39083 ) ) ;
#47691=LINE ( 'NONE', #50855, #410 ) ;
#47692=FACE_OUTER_BOUND ( 'NONE', #31062, .T. ) ;
#47696=DIRECTION ( 'NONE',  ( 0.02963332782256331357, 0.000000000000000000, -0.9995608365087942371 ) ) ;
#47698=LINE ( 'NONE', #32163, #19997 ) ;
#47699=EDGE_LOOP ( 'NONE', ( #11940, #18395, #27282, #46327 ) ) ;
#47701=AXIS2_PLACEMENT_3D ( 'NONE', #42236, #10188, #14399 ) ;
#47702=CIRCLE ( 'NONE', #31859, 125.0000000000000000 ) ;
#47703=DIRECTION ( 'NONE',  ( -0.000000000000000000, 1.000000000000000000, -0.000000000000000000 ) ) ;
#47705=VERTEX_POINT ( 'NONE', #21499 ) ;
#47706=AXIS2_PLACEMENT_3D ( 'NONE', #16843, #36802, #28637 ) ;
#47709=FACE_OUTER_BOUND ( 'NONE', #17146, .T. ) ;
#47710=CARTESIAN_POINT ( 'NONE',  ( -79.88691714431334390, -177.1207230881787780, 119.9572859573367367 ) ) ;
#47711=EDGE_CURVE ( 'NONE', #40896, #6302, #470, .T. ) ;
#47712=EDGE_LOOP ( 'NONE', ( #25314, #20068, #11684, #7826 ) ) ;
#47716=CIRCLE ( 'NONE', #40115, 125.0000000000000000 ) ;
#47717=DIRECTION ( 'NONE',  ( -0.000000000000000000, 1.000000000000000000, -0.000000000000000000 ) ) ;
#47718=DIRECTION ( 'NONE',  ( 0.000000000000000000, -0.000000000000000000, 1.000000000000000000 ) ) ;
#47719=ORIENTED_EDGE ( 'NONE', *, *, #33060, .F. ) ;
#47720=ORIENTED_EDGE ( 'NONE', *, *, #24744, .T. ) ;
#47722=CIRCLE ( 'NONE', #20022, 125.0000000000000000 ) ;
#47728=DIRECTION ( 'NONE',  ( 0.1768902751225666370, 0.000000000000000000, 0.9842305779475979399 ) ) ;
#47732=CARTESIAN_POINT ( 'NONE',  ( 41.00573479224733120, -193.5000000000000000, -87.27805883780175122 ) ) ;
#47733=CARTESIAN_POINT ( 'NONE',  ( 59.29945538372744096, -183.6283474603465606, 63.31490529818492519 ) ) ;
#47734=ORIENTED_EDGE ( 'NONE', *, *, #14484, .T. ) ;
#47736=VERTEX_POINT ( 'NONE', #4432 ) ;
#47737=CARTESIAN_POINT ( 'NONE',  ( 37.99238433767461487, -189.7472609257535510, -90.26448786734027863 ) ) ;
#47738=CARTESIAN_POINT ( 'NONE',  ( -47.63353074800702558, -193.5000000000000000, -0.5338233779647817423 ) ) ;
#47739=AXIS2_PLACEMENT_3D ( 'NONE', #46930, #31131, #35079 ) ;
#47742=CARTESIAN_POINT ( 'NONE',  ( -173.0003472773501585, -175.3837268820161057, 10.93003379476953363 ) ) ;
#47743=VERTEX_POINT ( 'NONE', #13091 ) ;
#47747=DIRECTION ( 'NONE',  ( -0.000000000000000000, 1.000000000000000000, -0.000000000000000000 ) ) ;
#47749=DIRECTION ( 'NONE',  ( 0.5085311186492154079, 0.000000000000000000, 0.8610436117673585521 ) ) ;
#47750=VERTEX_POINT ( 'NONE', #3005 ) ;
#47751=VECTOR ( 'NONE', #31754, 1000.000000000000000 ) ;
#47753=ADVANCED_FACE ( 'NONE', ( #29894 ), #15118, .F. ) ;
#47756=ADVANCED_FACE ( 'NONE', ( #22729 ), #19049, .T. ) ;
#47757=DIRECTION ( 'NONE',  ( -0.000000000000000000, 1.000000000000000000, -0.000000000000000000 ) ) ;
#47758=PLANE ( 'NONE',  #37660 ) ;
#47759=VERTEX_POINT ( 'NONE', #25955 ) ;
#47764=LINE ( 'NONE', #27761, #48944 ) ;
#47767=DIRECTION ( 'NONE',  ( -0.000000000000000000, 1.000000000000000000, -0.000000000000000000 ) ) ;
#47768=DIRECTION ( 'NONE',  ( 0.8124868780056783146, 0.000000000000000000, 0.5829794791144762289 ) ) ;
#47769=ORIENTED_EDGE ( 'NONE', *, *, #35151, .T. ) ;
#47771=CARTESIAN_POINT ( 'NONE',  ( -4.794493649713349015, -193.5000000000000000, -117.1181148702518726 ) ) ;
#47772=FACE_BOUND ( 'NONE', #50439, .T. ) ;
#47775=CARTESIAN_POINT ( 'NONE',  ( 67.04262753014327814, -189.7472609257535510, -47.74645837849745078 ) ) ;
#47776=CIRCLE ( 'NONE', #4069, 125.0000000000000000 ) ;
#47777=DIRECTION ( 'NONE',  ( 0.000000000000000000, 0.000000000000000000, 1.000000000000000000 ) ) ;
#47778=VERTEX_POINT ( 'NONE', #47170 ) ;
#47779=LINE ( 'NONE', #24127, #18733 ) ;
#47780=ORIENTED_EDGE ( 'NONE', *, *, #36067, .F. ) ;
#47781=CIRCLE ( 'NONE', #28436, 125.0000000000000000 ) ;
#47783=FACE_BOUND ( 'NONE', #23746, .T. ) ;
#47784=DIRECTION ( 'NONE',  ( 0.5586467658036594619, 0.000000000000000000, -0.8294056854501971054 ) ) ;
#47785=VERTEX_POINT ( 'NONE', #6956 ) ;
#47786=EDGE_CURVE ( 'NONE', #31544, #47106, #11144, .T. ) ;
#47787=EDGE_CURVE ( 'NONE', #9277, #25409, #27169, .T. ) ;
#47788=EDGE_CURVE ( 'NONE', #4302, #48486, #13875, .T. ) ;
#47791=EDGE_CURVE ( 'NONE', #37366, #37251, #15366, .T. ) ;
#47792=AXIS2_PLACEMENT_3D ( 'NONE', #25263, #11922, #20078 ) ;
#47793=ORIENTED_EDGE ( 'NONE', *, *, #51826, .F. ) ;
#47794=CARTESIAN_POINT ( 'NONE',  ( -48.47912675150885065, -177.1207230881787780, 6.938893903907228378E-15 ) ) ;
#47796=EDGE_CURVE ( 'NONE', #35424, #34486, #47691, .T. ) ;
#47797=FACE_OUTER_BOUND ( 'NONE', #40647, .T. ) ;
#47798=ADVANCED_FACE ( 'NONE', ( #23254 ), #19310, .T. ) ;
#47800=EDGE_CURVE ( 'NONE', #716, #25977, #9936, .T. ) ;
#47801=EDGE_CURVE ( 'NONE', #7649, #26442, #31375, .T. ) ;
#47803=DIRECTION ( 'NONE',  ( -0.1476465640024918202, 0.000000000000000000, 0.9890401873221624784 ) ) ;
#47804=ORIENTED_EDGE ( 'NONE', *, *, #33949, .T. ) ;
#47806=ORIENTED_EDGE ( 'NONE', *, *, #41047, .F. ) ;
#47811=ORIENTED_EDGE ( 'NONE', *, *, #29945, .F. ) ;
#47812=PLANE ( 'NONE',  #4625 ) ;
#47813=ORIENTED_EDGE ( 'NONE', *, *, #11696, .T. ) ;
#47815=CARTESIAN_POINT ( 'NONE',  ( -48.88225018079683082, -193.5000000000000000, 0.9151456172430223468 ) ) ;
#47816=ORIENTED_EDGE ( 'NONE', *, *, #10541, .T. ) ;
#47817=DIRECTION ( 'NONE',  ( 0.5085311186492216251, 0.000000000000000000, -0.8610436117673548884 ) ) ;
#47818=DIRECTION ( 'NONE',  ( -0.05924062789372142729, 0.000000000000000000, 0.9982437317643209074 ) ) ;
#47822=VERTEX_POINT ( 'NONE', #33837 ) ;
#47824=CARTESIAN_POINT ( 'NONE',  ( 71.73509643893275722, -183.6283474603465606, -30.40954281680804172 ) ) ;
#47825=LINE ( 'NONE', #32028, #46504 ) ;
#47826=FACE_OUTER_BOUND ( 'NONE', #36248, .T. ) ;
#47827=PLANE ( 'NONE',  #50121 ) ;
#47829=ORIENTED_EDGE ( 'NONE', *, *, #26595, .F. ) ;
#47831=CARTESIAN_POINT ( 'NONE',  ( -124.1938582159088327, -189.7472609257535510, -99.45993886622791536 ) ) ;
#47832=EDGE_CURVE ( 'NONE', #1331, #47304, #20561, .T. ) ;
#47833=DIRECTION ( 'NONE',  ( -0.1768902751225592818, 0.000000000000000000, -0.9842305779475992722 ) ) ;
#47835=DIRECTION ( 'NONE',  ( -0.2348860457809707758, 0.000000000000000000, -0.9720229140804138579 ) ) ;
#47836=ORIENTED_EDGE ( 'NONE', *, *, #21832, .F. ) ;
#47837=DIRECTION ( 'NONE',  ( 0.000000000000000000, 0.000000000000000000, 1.000000000000000000 ) ) ;
#47839=CARTESIAN_POINT ( 'NONE',  ( 7.403327498934737960, -189.7472609257535510, -110.6939782313521192 ) ) ;
#47840=VERTEX_POINT ( 'NONE', #34794 ) ;
#47843=ORIENTED_EDGE ( 'NONE', *, *, #8050, .F. ) ;
#47844=EDGE_CURVE ( 'NONE', #117, #44736, #6327, .T. ) ;
#47846=VECTOR ( 'NONE', #41239, 1000.000000000000000 ) ;
#47850=ORIENTED_EDGE ( 'NONE', *, *, #33572, .T. ) ;
#47852=EDGE_CURVE ( 'NONE', #26723, #16129, #24530, .T. ) ;
#47855=ADVANCED_FACE ( 'NONE', ( #51895 ), #20071, .T. ) ;
#47857=ORIENTED_EDGE ( 'NONE', *, *, #26288, .F. ) ;
#47858=ORIENTED_EDGE ( 'NONE', *, *, #37819, .T. ) ;
#47860=ORIENTED_EDGE ( 'NONE', *, *, #29861, .F. ) ;
#47861=VECTOR ( 'NONE', #43715, 999.9999999999998863 ) ;
#47862=CIRCLE ( 'NONE', #31079, 125.0000000000000000 ) ;
#47863=CARTESIAN_POINT ( 'NONE',  ( -140.5285791076019279, -175.3837268820161057, -83.08371579725672973 ) ) ;
#47864=PLANE ( 'NONE',  #28560 ) ;
#47868=EDGE_CURVE ( 'NONE', #11130, #29227, #19804, .T. ) ;
#47870=VERTEX_POINT ( 'NONE', #44254 ) ;
#47871=LINE ( 'NONE', #27870, #9621 ) ;
#47873=EDGE_CURVE ( 'NONE', #28133, #19912, #19769, .T. ) ;
#47875=CARTESIAN_POINT ( 'NONE',  ( 73.79319191488886531, -177.1207230881787780, 20.63201007055493008 ) ) ;
#47876=LINE ( 'NONE', #48125, #26553 ) ;
#47877=LINE ( 'NONE', #11849, #23176 ) ;
#47878=ORIENTED_EDGE ( 'NONE', *, *, #10403, .F. ) ;
#47881=CARTESIAN_POINT ( 'NONE',  ( -131.9398708394020332, -177.1207230881787780, 91.70840728318374602 ) ) ;
#47884=CARTESIAN_POINT ( 'NONE',  ( 76.51419089073347379, -177.1207230881787780, -1.292495564988661139 ) ) ;
#47885=CARTESIAN_POINT ( 'NONE',  ( -172.2289551866394106, -189.7472609257535510, -17.63462396184707970 ) ) ;
#47886=CARTESIAN_POINT ( 'NONE',  ( 68.24201764719070695, -177.1207230881787780, -44.73448837594910543 ) ) ;
#47887=ORIENTED_EDGE ( 'NONE', *, *, #13552, .T. ) ;
#47888=FACE_OUTER_BOUND ( 'NONE', #35344, .T. ) ;
#47892=ORIENTED_EDGE ( 'NONE', *, *, #12717, .F. ) ;
#47893=CARTESIAN_POINT ( 'NONE',  ( -48.47912675150885065, -175.3837268820161057, 6.938893903907228378E-15 ) ) ;
#47894=PLANE ( 'NONE',  #27016 ) ;
#47898=VECTOR ( 'NONE', #38143, 1000.000000000000000 ) ;
#47900=PLANE ( 'NONE',  #42227 ) ;
#47902=DIRECTION ( 'NONE',  ( 0.1182731709213660498, 0.000000000000000000, -0.9929810960135169173 ) ) ;
#47903=CARTESIAN_POINT ( 'NONE',  ( -173.4787860028527007, -183.6283474603465606, 0.2918682030023308505 ) ) ;
#47904=ORIENTED_EDGE ( 'NONE', *, *, #52009, .F. ) ;
#47905=ORIENTED_EDGE ( 'NONE', *, *, #2595, .F. ) ;
#47907=EDGE_CURVE ( 'NONE', #28151, #11654, #8858, .T. ) ;
#47908=CARTESIAN_POINT ( 'NONE',  ( -48.98765787015805984, -193.5000000000000000, -0.8610436117673551104 ) ) ;
#47909=DIRECTION ( 'NONE',  ( 0.000000000000000000, 0.000000000000000000, 1.000000000000000000 ) ) ;
#47911=EDGE_LOOP ( 'NONE', ( #8736, #35384, #11761, #19938 ) ) ;
#47913=ORIENTED_EDGE ( 'NONE', *, *, #47015, .T. ) ;
#47914=DIRECTION ( 'NONE',  ( 0.000000000000000000, 0.000000000000000000, 1.000000000000000000 ) ) ;
#47916=LINE ( 'NONE', #7954, #39528 ) ;
#47917=LINE ( 'NONE', #7196, #47575 ) ;
#47918=VERTEX_POINT ( 'NONE', #93 ) ;
#47921=CARTESIAN_POINT ( 'NONE',  ( -48.47912675150885065, -183.6283474603465606, 6.938893903907228378E-15 ) ) ;
#47922=PLANE ( 'NONE',  #28519 ) ;
#47923=LINE ( 'NONE', #23494, #45921 ) ;
#47924=ADVANCED_FACE ( 'NONE', ( #48718 ), #16399, .T. ) ;
#47926=DIRECTION ( 'NONE',  ( 0.000000000000000000, -0.000000000000000000, 1.000000000000000000 ) ) ;
#47927=EDGE_LOOP ( 'NONE', ( #31815, #26828, #22439, #3280 ) ) ;
#47928=FACE_OUTER_BOUND ( 'NONE', #38444, .T. ) ;
#47930=CARTESIAN_POINT ( 'NONE',  ( 23.33927677392130917, -183.6283474603465606, -102.3089288139528747 ) ) ;
#47933=EDGE_CURVE ( 'NONE', #47705, #7370, #28993, .T. ) ;
#47935=ORIENTED_EDGE ( 'NONE', *, *, #49755, .T. ) ;
#47938=CARTESIAN_POINT ( 'NONE',  ( -49.44376233341720450, -175.3837268820161057, -0.2635871660690713436 ) ) ;
#47939=FACE_OUTER_BOUND ( 'NONE', #8313, .T. ) ;
#47940=ORIENTED_EDGE ( 'NONE', *, *, #14835, .T. ) ;
#47944=VERTEX_POINT ( 'NONE', #24278 ) ;
#47947=CARTESIAN_POINT ( 'NONE',  ( -142.9772358822569629, -183.6283474603465606, 81.82363577055970438 ) ) ;
#47949=CIRCLE ( 'NONE', #48782, 125.0000000000000000 ) ;
#47950=CARTESIAN_POINT ( 'NONE',  ( -27.18512803868276251, -189.7472609257535510, -123.1729094355498404 ) ) ;
#47951=ORIENTED_EDGE ( 'NONE', *, *, #10937, .T. ) ;
#47953=DIRECTION ( 'NONE',  ( 0.000000000000000000, 0.000000000000000000, 1.000000000000000000 ) ) ;
#47954=DIRECTION ( 'NONE',  ( 0.000000000000000000, 0.000000000000000000, -1.000000000000000000 ) ) ;
#47955=PLANE ( 'NONE',  #19888 ) ;
#47956=ADVANCED_FACE ( 'NONE', ( #8494 ), #32924, .T. ) ;
#47958=CARTESIAN_POINT ( 'NONE',  ( -27.18512803868275540, -175.3837268820161057, -123.1729094355498262 ) ) ;
#47959=ORIENTED_EDGE ( 'NONE', *, *, #10270, .T. ) ;
#47961=DIRECTION ( 'NONE',  ( -0.6528221181905280446, 0.000000000000000000, 0.7575112421616145841 ) ) ;
#47962=DIRECTION ( 'NONE',  ( 0.000000000000000000, 1.000000000000000000, -0.000000000000000000 ) ) ;
#47964=AXIS2_PLACEMENT_3D ( 'NONE', #49060, #13317, #16759 ) ;
#47965=ORIENTED_EDGE ( 'NONE', *, *, #43123, .T. ) ;
#47966=DIRECTION ( 'NONE',  ( -0.000000000000000000, 1.000000000000000000, -0.000000000000000000 ) ) ;
#47967=EDGE_CURVE ( 'NONE', #4130, #14785, #36534, .T. ) ;
#47968=AXIS2_PLACEMENT_3D ( 'NONE', #35654, #7551, #8327 ) ;
#47969=AXIS2_PLACEMENT_3D ( 'NONE', #18497, #19009, #51095 ) ;
#47971=EDGE_CURVE ( 'NONE', #41557, #50211, #44084, .T. ) ;
#47972=ORIENTED_EDGE ( 'NONE', *, *, #15202, .T. ) ;
#47973=PLANE ( 'NONE',  #13034 ) ;
#47977=FACE_OUTER_BOUND ( 'NONE', #16685, .T. ) ;
#47978=CARTESIAN_POINT ( 'NONE',  ( 5.015379008610445943, -183.6283474603465606, -112.9749434763326690 ) ) ;
#47979=CARTESIAN_POINT ( 'NONE',  ( -137.2261550162227479, -183.6283474603465606, 86.60307583628416239 ) ) ;
#47981=VECTOR ( 'NONE', #18802, 1000.000000000000000 ) ;
#47987=EDGE_CURVE ( 'NONE', #4203, #38934, #49166, .T. ) ;
#47991=EDGE_LOOP ( 'NONE', ( #41621, #49164, #37890, #18288 ) ) ;
#47992=CARTESIAN_POINT ( 'NONE',  ( -146.8460685364478877, -183.6283474603465606, 75.49882471933933914 ) ) ;
#47993=EDGE_LOOP ( 'NONE', ( #33713, #26138 ) ) ;
#47995=VERTEX_POINT ( 'NONE', #23758 ) ;
#47996=VERTEX_POINT ( 'NONE', #39763 ) ;
#47997=CARTESIAN_POINT ( 'NONE',  ( -48.36085358058748085, -183.6283474603465606, -0.9929810960135100339 ) ) ;
#48000=CARTESIAN_POINT ( 'NONE',  ( -165.1736796818183564, -177.1207230881787780, -41.93543928473609839 ) ) ;
#48002=ORIENTED_EDGE ( 'NONE', *, *, #51229, .T. ) ;
#48003=CARTESIAN_POINT ( 'NONE',  ( -48.47912675150885065, -183.6283474603465606, 6.938893903907228378E-15 ) ) ;
#48004=VECTOR ( 'NONE', #27707, 1000.000000000000114 ) ;
#48006=VECTOR ( 'NONE', #23715, 1000.000000000000000 ) ;
#48008=DIRECTION ( 'NONE',  ( 0.5586467658036535777, 0.000000000000000000, -0.8294056854502011022 ) ) ;
#48009=CARTESIAN_POINT ( 'NONE',  ( 4.109287492203100634, -193.5000000000000000, -113.3995532942336979 ) ) ;
#48011=ADVANCED_FACE ( 'NONE', ( #22150 ), #33714, .T. ) ;
#48012=DIRECTION ( 'NONE',  ( 0.000000000000000000, 1.000000000000000000, 0.000000000000000000 ) ) ;
#48013=DIRECTION ( 'NONE',  ( -0.9027978299657387629, 0.000000000000000000, -0.4300652022765304450 ) ) ;
#48015=DIRECTION ( 'NONE',  ( -0.000000000000000000, 1.000000000000000000, -0.000000000000000000 ) ) ;
#48019=FACE_BOUND ( 'NONE', #26331, .T. ) ;
#48020=VERTEX_POINT ( 'NONE', #49759 ) ;
#48023=CARTESIAN_POINT ( 'NONE',  ( -137.2624501260119985, -183.6283474603465606, 87.99159897727967916 ) ) ;
#48024=DIRECTION ( 'NONE',  ( 0.000000000000000000, 1.000000000000000000, 0.000000000000000000 ) ) ;
#48025=ORIENTED_EDGE ( 'NONE', *, *, #47177, .T. ) ;
#48027=EDGE_CURVE ( 'NONE', #51992, #47640, #22295, .T. ) ;
#48028=ORIENTED_EDGE ( 'NONE', *, *, #38464, .T. ) ;
#48030=EDGE_CURVE ( 'NONE', #27697, #13519, #33966, .T. ) ;
#48031=DIRECTION ( 'NONE',  ( -0.000000000000000000, 1.000000000000000000, 0.000000000000000000 ) ) ;
#48032=EDGE_CURVE ( 'NONE', #51044, #11395, #41077, .T. ) ;
#48033=FACE_BOUND ( 'NONE', #28754, .T. ) ;
#48034=PLANE ( 'NONE',  #40493 ) ;
#48036=AXIS2_PLACEMENT_3D ( 'NONE', #19682, #23385, #12580 ) ;
#48037=DIRECTION ( 'NONE',  ( -0.000000000000000000, 1.000000000000000000, 0.000000000000000000 ) ) ;
#48039=AXIS2_PLACEMENT_3D ( 'NONE', #12920, #32890, #48941 ) ;
#48041=CARTESIAN_POINT ( 'NONE',  ( -163.0741914257288272, -175.3837268820161057, 47.37063079638398477 ) ) ;
#48043=DIRECTION ( 'NONE',  ( 0.000000000000000000, 0.000000000000000000, -1.000000000000000000 ) ) ;
#48046=AXIS2_PLACEMENT_3D ( 'NONE', #36102, #12445, #25071 ) ;
#48048=LINE ( 'NONE', #4683, #45773 ) ;
#48051=DIRECTION ( 'NONE',  ( -0.000000000000000000, 1.000000000000000000, 0.000000000000000000 ) ) ;
#48052=VERTEX_POINT ( 'NONE', #17452 ) ;
#48053=VECTOR ( 'NONE', #16480, 1000.000000000000000 ) ;
#48054=AXIS2_PLACEMENT_3D ( 'NONE', #9308, #45572, #25574 ) ;
#48055=ORIENTED_EDGE ( 'NONE', *, *, #33380, .F. ) ;
#48056=DIRECTION ( 'NONE',  ( 0.000000000000000000, -1.000000000000000000, -0.000000000000000000 ) ) ;
#48059=VERTEX_POINT ( 'NONE', #37132 ) ;
#48060=VECTOR ( 'NONE', #13388, 1000.000000000000000 ) ;
#48061=DIRECTION ( 'NONE',  ( 0.8455960035018272869, 0.000000000000000000, -0.5338233779647886257 ) ) ;
#48062=EDGE_LOOP ( 'NONE', ( #26148, #39524, #20874, #48426 ) ) ;
#48065=VERTEX_POINT ( 'NONE', #33473 ) ;
#48066=ORIENTED_EDGE ( 'NONE', *, *, #10840, .F. ) ;
#48067=CARTESIAN_POINT ( 'NONE',  ( -2.700932609314990351, -177.1207230881787780, -116.3157639405751667 ) ) ;
#48068=LINE ( 'NONE', #44120, #31549 ) ;
#48069=DIRECTION ( 'NONE',  ( 0.000000000000000000, 1.000000000000000000, -0.000000000000000000 ) ) ;
#48070=CARTESIAN_POINT ( 'NONE',  ( 38.46761263173350898, -189.7472609257535510, 89.80681772907070126 ) ) ;
#48071=DIRECTION ( 'NONE',  ( 0.000000000000000000, -0.000000000000000000, 1.000000000000000000 ) ) ;
#48072=VECTOR ( 'NONE', #37983, 1000.000000000000114 ) ;
#48074=EDGE_CURVE ( 'NONE', #45175, #27697, #17175, .T. ) ;
#48076=ORIENTED_EDGE ( 'NONE', *, *, #13638, .T. ) ;
#48079=CARTESIAN_POINT ( 'NONE',  ( -169.9883746053192795, -189.7472609257535510, -24.72869175143020826 ) ) ;
#48080=DIRECTION ( 'NONE',  ( 0.000000000000000000, 0.000000000000000000, -1.000000000000000000 ) ) ;
#48082=DIRECTION ( 'NONE',  ( 0.000000000000000000, 0.000000000000000000, 1.000000000000000000 ) ) ;
#48084=CARTESIAN_POINT ( 'NONE',  ( -46.06708674231130374, -183.6283474603465606, -124.9767260852756863 ) ) ;
#48085=ADVANCED_FACE ( 'NONE', ( #45306 ), #25316, .F. ) ;
#48086=DIRECTION ( 'NONE',  ( 0.9646355819083594074, 0.000000000000000000, -0.2635871660690647933 ) ) ;
#48088=ORIENTED_EDGE ( 'NONE', *, *, #12668, .T. ) ;
#48095=PLANE ( 'NONE',  #30920 ) ;
#48096=VECTOR ( 'NONE', #1356, 1000.000000000000000 ) ;
#48097=EDGE_CURVE ( 'NONE', #41262, #11883, #44125, .T. ) ;
#48098=CARTESIAN_POINT ( 'NONE',  ( -167.6453766917639427, -193.5000000000000000, 37.74128873232411507 ) ) ;
#48099=CARTESIAN_POINT ( 'NONE',  ( 73.09196206113300320, -183.6283474603465606, 29.07697310430964421 ) ) ;
#48100=PLANE ( 'NONE',  #49716 ) ;
#48101=ADVANCED_FACE ( 'NONE', ( #30035 ), #46085, .T. ) ;
#48104=DIRECTION ( 'NONE',  ( 0.000000000000000000, -1.000000000000000000, 0.000000000000000000 ) ) ;
#48105=VERTEX_POINT ( 'NONE', #1398 ) ;
#48106=VERTEX_POINT ( 'NONE', #1666 ) ;
#48107=ORIENTED_EDGE ( 'NONE', *, *, #47177, .F. ) ;
#48109=DIRECTION ( 'NONE',  ( -0.6528221181905174975, 0.000000000000000000, -0.7575112421616236880 ) ) ;
#48110=VECTOR ( 'NONE', #23394, 1000.000000000000000 ) ;
#48111=ORIENTED_EDGE ( 'NONE', *, *, #17958, .T. ) ;
#48112=EDGE_CURVE ( 'NONE', #37279, #26450, #7179, .T. ) ;
#48113=AXIS2_PLACEMENT_3D ( 'NONE', #7184, #14305, #43451 ) ;
#48116=CARTESIAN_POINT ( 'NONE',  ( -100.6109117578263152, -183.6283474603465606, 112.5098962032393359 ) ) ;
#48118=ORIENTED_EDGE ( 'NONE', *, *, #10172, .T. ) ;
#48119=CARTESIAN_POINT ( 'NONE',  ( 35.67816836544800196, -177.1207230881787780, -92.42591454022745268 ) ) ;
#48120=ORIENTED_EDGE ( 'NONE', *, *, #32392, .F. ) ;
#48121=DIRECTION ( 'NONE',  ( 0.000000000000000000, 0.000000000000000000, -1.000000000000000000 ) ) ;
#48122=ORIENTED_EDGE ( 'NONE', *, *, #5327, .T. ) ;
#48123=DIRECTION ( 'NONE',  ( -0.9995608365087940150, 0.000000000000000000, -0.02963332782257007206 ) ) ;
#48125=CARTESIAN_POINT ( 'NONE',  ( -101.9736325116273576, -177.1207230881787780, 112.9749434763330811 ) ) ;
#48126=CARTESIAN_POINT ( 'NONE',  ( 68.24201764719070695, -183.6283474603465606, -44.73448837594909833 ) ) ;
#48127=VECTOR ( 'NONE', #18450, 1000.000000000000000 ) ;
#48128=VERTEX_POINT ( 'NONE', #34238 ) ;
#48132=DIRECTION ( 'NONE',  ( -0.7765238627180482966, 0.000000000000000000, 0.6300878435817038881 ) ) ;
#48133=DIRECTION ( 'NONE',  ( 0.000000000000000000, 0.000000000000000000, -1.000000000000000000 ) ) ;
#48134=ORIENTED_EDGE ( 'NONE', *, *, #47074, .T. ) ;
#48135=CARTESIAN_POINT ( 'NONE',  ( 47.70255505652111339, -189.7472609257535510, 78.26291788638732783 ) ) ;
#48136=LINE ( 'NONE', #47885, #31558 ) ;
#48137=LINE ( 'NONE', #8193, #17331 ) ;
#48139=EDGE_CURVE ( 'NONE', #9556, #30483, #51681, .T. ) ;
#48140=EDGE_CURVE ( 'NONE', #1324, #51755, #38435, .T. ) ;
#48141=ORIENTED_EDGE ( 'NONE', *, *, #22345, .T. ) ;
#48142=EDGE_CURVE ( 'NONE', #2545, #4861, #31316, .T. ) ;
#48143=CARTESIAN_POINT ( 'NONE',  ( 23.33927677392130917, -193.5000000000000000, -102.3089288139528747 ) ) ;
#48145=EDGE_CURVE ( 'NONE', #8800, #42139, #26491, .T. ) ;
#48147=CARTESIAN_POINT ( 'NONE',  ( 70.20858612167234014, -183.6283474603465606, 35.90758392117750475 ) ) ;
#48148=EDGE_LOOP ( 'NONE', ( #23408, #19014, #35093, #12942 ) ) ;
#48149=DIRECTION ( 'NONE',  ( 0.000000000000000000, 1.000000000000000000, -0.000000000000000000 ) ) ;
#48150=ADVANCED_FACE ( 'NONE', ( #42886 ), #15300, .T. ) ;
#48151=DIRECTION ( 'NONE',  ( 0.000000000000000000, -0.000000000000000000, 1.000000000000000000 ) ) ;
#48152=VECTOR ( 'NONE', #19134, 1000.000000000000000 ) ;
#48153=PLANE ( 'NONE',  #42000 ) ;
#48155=CARTESIAN_POINT ( 'NONE',  ( -133.8011377042516301, -177.1207230881787780, -91.35181687837437892 ) ) ;
#48156=EDGE_CURVE ( 'NONE', #20663, #48860, #30686, .T. ) ;
#48157=CIRCLE ( 'NONE', #40554, 125.0000000000000000 ) ;
#48158=EDGE_CURVE ( 'NONE', #20663, #39795, #14270, .T. ) ;
#48162=DIRECTION ( 'NONE',  ( -0.000000000000000000, 1.000000000000000000, -0.000000000000000000 ) ) ;
#48163=CARTESIAN_POINT ( 'NONE',  ( -95.37971604807238180, -183.6283474603465606, -114.7887733785764226 ) ) ;
#48165=EDGE_CURVE ( 'NONE', #23027, #25456, #8040, .T. ) ;
#48166=ORIENTED_EDGE ( 'NONE', *, *, #34639, .T. ) ;
#48167=CARTESIAN_POINT ( 'NONE',  ( -78.64590280292341617, -189.7472609257535510, -121.3052580173827408 ) ) ;
#48168=VECTOR ( 'NONE', #20439, 1000.000000000000000 ) ;
#48169=EDGE_CURVE ( 'NONE', #34175, #10145, #35258, .T. ) ;
#48170=PLANE ( 'NONE',  #23767 ) ;
#48172=ORIENTED_EDGE ( 'NONE', *, *, #15400, .F. ) ;
#48173=ORIENTED_EDGE ( 'NONE', *, *, #7183, .F. ) ;
#48174=CARTESIAN_POINT ( 'NONE',  ( -49.03777351731250889, -193.5000000000000000, 0.8294056854502042109 ) ) ;
#48177=CARTESIAN_POINT ( 'NONE',  ( -88.49718702276017268, -193.5000000000000000, -117.3655938605927389 ) ) ;
#48179=ORIENTED_EDGE ( 'NONE', *, *, #7513, .F. ) ;
#48180=ADVANCED_FACE ( 'NONE', ( #34484 ), #50533, .T. ) ;
#48181=VERTEX_POINT ( 'NONE', #42638 ) ;
#48182=ADVANCED_FACE ( 'NONE', ( #14532 ), #22669, .T. ) ;
#48183=CARTESIAN_POINT ( 'NONE',  ( -5.732832253866452454, -175.3837268820161057, -117.4638425504666799 ) ) ;
#48184=PLANE ( 'NONE',  #32736 ) ;
#48187=CARTESIAN_POINT ( 'NONE',  ( -170.7514454179067513, -183.6283474603465606, -20.63201007055403480 ) ) ;
#48188=VECTOR ( 'NONE', #4555, 1000.000000000000114 ) ;
#48189=ORIENTED_EDGE ( 'NONE', *, *, #41657, .T. ) ;
#48190=FACE_OUTER_BOUND ( 'NONE', #38933, .T. ) ;
#48192=CARTESIAN_POINT ( 'NONE',  ( 11.10560377650619301, -183.6283474603465606, -108.7464374498168951 ) ) ;
#48193=CARTESIAN_POINT ( 'NONE',  ( 56.46549106873199264, -189.7472609257535510, -66.05018866041272929 ) ) ;
#48197=EDGE_LOOP ( 'NONE', ( #7994, #17459, #26888, #2966 ) ) ;
#48199=CARTESIAN_POINT ( 'NONE',  ( -133.8011377042516301, -183.6283474603465606, -91.35181687837437892 ) ) ;
#48200=CARTESIAN_POINT ( 'NONE',  ( 58.48829670243886625, -183.6283474603465606, -64.67588669375805921 ) ) ;
#48203=PLANE ( 'NONE',  #23699 ) ;
#48204=EDGE_CURVE ( 'NONE', #38453, #19435, #46589, .T. ) ;
#48205=CARTESIAN_POINT ( 'NONE',  ( -49.42645310536303782, -183.6283474603465606, -0.3202698538628417357 ) ) ;
#48207=EDGE_LOOP ( 'NONE', ( #39203, #42257, #31166, #22265 ) ) ;
#48209=AXIS2_PLACEMENT_3D ( 'NONE', #2492, #22976, #38987 ) ;
#48210=EDGE_CURVE ( 'NONE', #12390, #32491, #11336, .T. ) ;
#48211=ORIENTED_EDGE ( 'NONE', *, *, #28833, .F. ) ;
#48212=CARTESIAN_POINT ( 'NONE',  ( -123.8574911141017765, -193.5000000000000000, 98.45863302693528851 ) ) ;
#48213=ORIENTED_EDGE ( 'NONE', *, *, #14626, .F. ) ;
#48214=DIRECTION ( 'NONE',  ( -0.000000000000000000, 1.000000000000000000, -0.000000000000000000 ) ) ;
#48215=CARTESIAN_POINT ( 'NONE',  ( 56.46549106873199975, -175.3837268820161057, -66.05018866041274350 ) ) ;
#48216=ORIENTED_EDGE ( 'NONE', *, *, #34108, .F. ) ;
#48219=CARTESIAN_POINT ( 'NONE',  ( 74.61260187273138911, -177.1207230881787780, -14.98512977653175149 ) ) ;
#48224=EDGE_LOOP ( 'NONE', ( #43351, #478, #24553, #8399 ) ) ;
#48225=EDGE_CURVE ( 'NONE', #42327, #32964, #43420, .T. ) ;
#48226=CARTESIAN_POINT ( 'NONE',  ( 26.70958190211000982, -175.3837268820161057, -99.85818990449013199 ) ) ;
#48227=DIRECTION ( 'NONE',  ( 0.000000000000000000, -1.000000000000000000, 0.000000000000000000 ) ) ;
#48228=ORIENTED_EDGE ( 'NONE', *, *, #15823, .T. ) ;
#48231=ORIENTED_EDGE ( 'NONE', *, *, #31518, .T. ) ;
#48233=CIRCLE ( 'NONE', #25560, 125.0000000000000000 ) ;
#48234=EDGE_CURVE ( 'NONE', #653, #672, #19486, .T. ) ;
#48235=DIRECTION ( 'NONE',  ( -0.000000000000000000, 1.000000000000000000, -0.000000000000000000 ) ) ;
#48238=CARTESIAN_POINT ( 'NONE',  ( -47.78257572244585560, -177.1207230881787780, -0.7175072570443230546 ) ) ;
#48239=ORIENTED_EDGE ( 'NONE', *, *, #22029, .T. ) ;
#48240=PLANE ( 'NONE',  #23332 ) ;
#48241=LINE ( 'NONE', #48511, #31672 ) ;
#48242=PLANE ( 'NONE',  #7619 ) ;
#48243=CARTESIAN_POINT ( 'NONE',  ( -1.230335819511603423, -193.5000000000000000, 115.7261930397108216 ) ) ;
#48245=ORIENTED_EDGE ( 'NONE', *, *, #33844, .F. ) ;
#48246=ORIENTED_EDGE ( 'NONE', *, *, #23642, .F. ) ;
#48247=CARTESIAN_POINT ( 'NONE',  ( -135.4258661347518853, -175.3837268820161057, -89.80681772907007598 ) ) ;
#48248=FACE_OUTER_BOUND ( 'NONE', #41284, .T. ) ;
#48249=DIRECTION ( 'NONE',  ( 0.000000000000000000, 0.000000000000000000, -1.000000000000000000 ) ) ;
#48251=DIRECTION ( 'NONE',  ( 0.000000000000000000, -1.000000000000000000, -0.000000000000000000 ) ) ;
#48253=VERTEX_POINT ( 'NONE', #25510 ) ;
#48254=CARTESIAN_POINT ( 'NONE',  ( -115.4536696835168641, -177.1207230881787780, -105.5434062319793185 ) ) ;
#48257=VECTOR ( 'NONE', #43026, 1000.000000000000114 ) ;
#48258=DIRECTION ( 'NONE',  ( 0.000000000000000000, 0.000000000000000000, 1.000000000000000000 ) ) ;
#48259=LINE ( 'NONE', #49307, #27478 ) ;
#48260=VECTOR ( 'NONE', #16010, 1000.000000000000000 ) ;
#48261=VECTOR ( 'NONE', #15965, 1000.000000000000000 ) ;
#48262=DIRECTION ( 'NONE',  ( 0.000000000000000000, 1.000000000000000000, 0.000000000000000000 ) ) ;
#48263=EDGE_CURVE ( 'NONE', #26317, #51929, #33416, .T. ) ;
#48264=CARTESIAN_POINT ( 'NONE',  ( -1.578537454945990293, -193.5000000000000000, 114.7887733785766926 ) ) ;
#48265=ORIENTED_EDGE ( 'NONE', *, *, #34012, .T. ) ;
#48266=DIRECTION ( 'NONE',  ( -0.000000000000000000, 1.000000000000000000, 0.000000000000000000 ) ) ;
#48268=AXIS2_PLACEMENT_3D ( 'NONE', #11496, #22820, #2839 ) ;
#48269=ORIENTED_EDGE ( 'NONE', *, *, #30406, .T. ) ;
#48270=CARTESIAN_POINT ( 'NONE',  ( -128.2395503755045638, -183.6283474603465606, -96.24590808611419845 ) ) ;
#48271=AXIS2_PLACEMENT_3D ( 'NONE', #20445, #48051, #16522 ) ;
#48273=FACE_OUTER_BOUND ( 'NONE', #18990, .T. ) ;
#48274=AXIS2_PLACEMENT_3D ( 'NONE', #41897, #6432, #9846 ) ;
#48275=DIRECTION ( 'NONE',  ( 4.884776371667510679E-16, 0.000000000000000000, -1.000000000000000000 ) ) ;
#48276=DIRECTION ( 'NONE',  ( 0.9266896074318291543, 0.000000000000000000, 0.3758275821142488260 ) ) ;
#48277=DIRECTION ( 'NONE',  ( -0.8896570909947530970, 0.000000000000000000, 0.4566292373937018700 ) ) ;
#48278=ORIENTED_EDGE ( 'NONE', *, *, #2173, .T. ) ;
#48279=VECTOR ( 'NONE', #4232, 1000.000000000000000 ) ;
#48281=CARTESIAN_POINT ( 'NONE',  ( -168.8371699641976420, -189.7472609257535510, 33.74820638215509661 ) ) ;
#48283=FACE_BOUND ( 'NONE', #35868, .T. ) ;
#48285=EDGE_CURVE ( 'NONE', #28119, #27646, #44159, .T. ) ;
#48286=DIRECTION ( 'NONE',  ( -0.1182731709213660498, 0.000000000000000000, 0.9929810960135169173 ) ) ;
#48288=VERTEX_POINT ( 'NONE', #44711 ) ;
#48289=DIRECTION ( 'NONE',  ( 0.7765238627180393038, 0.000000000000000000, 0.6300878435817147682 ) ) ;
#48291=CARTESIAN_POINT ( 'NONE',  ( -164.6246685127424882, -189.7472609257535510, -46.20836643930983456 ) ) ;
#48292=AXIS2_PLACEMENT_3D ( 'NONE', #32355, #23698, #39464 ) ;
#48293=FACE_BOUND ( 'NONE', #3218, .T. ) ;
#48294=CARTESIAN_POINT ( 'NONE',  ( -140.5933766095837427, -175.3837268820161057, -84.49831343337065448 ) ) ;
#48295=VECTOR ( 'NONE', #42368, 1000.000000000000000 ) ;
#48296=CIRCLE ( 'NONE', #11366, 124.9999999999999858 ) ;
#48299=ORIENTED_EDGE ( 'NONE', *, *, #8348, .T. ) ;
#48300=AXIS2_PLACEMENT_3D ( 'NONE', #24367, #24121, #36437 ) ;
#48301=VERTEX_POINT ( 'NONE', #49178 ) ;
#48302=CARTESIAN_POINT ( 'NONE',  ( 56.77503207194101265, -175.3837268820161057, -67.42819922234311036 ) ) ;
#48303=EDGE_CURVE ( 'NONE', #18993, #17406, #14810, .T. ) ;
#48304=VERTEX_POINT ( 'NONE', #25006 ) ;
#48306=DIRECTION ( 'NONE',  ( 0.000000000000000000, 0.000000000000000000, -1.000000000000000000 ) ) ;
#48307=VECTOR ( 'NONE', #516, 1000.000000000000000 ) ;
#48308=DIRECTION ( 'NONE',  ( 0.9266896074318317078, 0.000000000000000000, 0.3758275821142421647 ) ) ;
#48309=AXIS2_PLACEMENT_3D ( 'NONE', #28334, #28587, #44631 ) ;
#48312=DIRECTION ( 'NONE',  ( 0.2920567706369764371, 0.000000000000000000, -0.9564009842765223146 ) ) ;
#48314=ORIENTED_EDGE ( 'NONE', *, *, #39268, .F. ) ;
#48317=ORIENTED_EDGE ( 'NONE', *, *, #40944, .T. ) ;
#48318=VERTEX_POINT ( 'NONE', #5828 ) ;
#48320=ORIENTED_EDGE ( 'NONE', *, *, #31759, .T. ) ;
#48321=LINE ( 'NONE', #35702, #3797 ) ;
#48323=EDGE_CURVE ( 'NONE', #21876, #37521, #13176, .T. ) ;
#48324=PLANE ( 'NONE',  #35100 ) ;
#48325=ORIENTED_EDGE ( 'NONE', *, *, #26501, .T. ) ;
#48326=CARTESIAN_POINT ( 'NONE',  ( -154.6193097927903182, -193.5000000000000000, -66.02470404298122730 ) ) ;
#48329=EDGE_CURVE ( 'NONE', #49227, #17596, #37608, .T. ) ;
#48330=ORIENTED_EDGE ( 'NONE', *, *, #38741, .F. ) ;
#48331=CYLINDRICAL_SURFACE ( 'NONE', #13639, 125.0000000000000000 ) ;
#48333=VECTOR ( 'NONE', #21786, 1000.000000000000000 ) ;
#48334=DIRECTION ( 'NONE',  ( 0.000000000000000000, -1.000000000000000000, 0.000000000000000000 ) ) ;
#48335=LINE ( 'NONE', #3931, #7884 ) ;
#48337=CARTESIAN_POINT ( 'NONE',  ( -146.0653709326077490, -193.5000000000000000, -78.11481899503411341 ) ) ;
#48339=FACE_OUTER_BOUND ( 'NONE', #20729, .T. ) ;
#48343=DIRECTION ( 'NONE',  ( 0.000000000000000000, 0.000000000000000000, -1.000000000000000000 ) ) ;
#48344=PLANE ( 'NONE',  #9496 ) ;
#48345=VERTEX_POINT ( 'NONE', #36829 ) ;
#48346=DIRECTION ( 'NONE',  ( 0.6965510290630033685, 0.000000000000000000, -0.7175072570443249420 ) ) ;
#48347=AXIS2_PLACEMENT_3D ( 'NONE', #19243, #39960, #31309 ) ;
#48349=AXIS2_PLACEMENT_3D ( 'NONE', #5949, #23518, #36116 ) ;
#48350=CARTESIAN_POINT ( 'NONE',  ( 48.69345348225013481, -175.3837268820161057, -78.62880929222873760 ) ) ;
#48352=ORIENTED_EDGE ( 'NONE', *, *, #18447, .F. ) ;
#48353=ORIENTED_EDGE ( 'NONE', *, *, #33375, .T. ) ;
#48355=VERTEX_POINT ( 'NONE', #41809 ) ;
#48356=AXIS2_PLACEMENT_3D ( 'NONE', #18545, #34559, #1484 ) ;
#48357=CARTESIAN_POINT ( 'NONE',  ( 76.37123734610607073, -193.5000000000000000, 6.114457023561876703 ) ) ;
#48359=DIRECTION ( 'NONE',  ( 0.8610436117673514467, 0.000000000000000000, 0.5085311186492273983 ) ) ;
#48360=PLANE ( 'NONE',  #25400 ) ;
#48361=ORIENTED_EDGE ( 'NONE', *, *, #1863, .T. ) ;
#48362=CARTESIAN_POINT ( 'NONE',  ( 32.99469856375238663, -193.5000000000000000, 94.79987230212020677 ) ) ;
#48363=ORIENTED_EDGE ( 'NONE', *, *, #51641, .T. ) ;
#48364=ORIENTED_EDGE ( 'NONE', *, *, #36239, .F. ) ;
#48366=AXIS2_PLACEMENT_3D ( 'NONE', #14411, #45969, #29646 ) ;
#48367=ORIENTED_EDGE ( 'NONE', *, *, #26037, .T. ) ;
#48368=CARTESIAN_POINT ( 'NONE',  ( -49.38192458147459973, -193.5000000000000000, 0.4300652022765185656 ) ) ;
#48369=AXIS2_PLACEMENT_3D ( 'NONE', #18923, #50232, #10267 ) ;
#48371=EDGE_CURVE ( 'NONE', #13513, #45342, #49693, .T. ) ;
#48372=CARTESIAN_POINT ( 'NONE',  ( -49.47868758801764955, -189.7472609257535510, 0.02963332782255607284 ) ) ;
#48374=PLANE ( 'NONE',  #48480 ) ;
#48375=DIRECTION ( 'NONE',  ( 0.000000000000000000, 0.000000000000000000, -1.000000000000000000 ) ) ;
#48376=VERTEX_POINT ( 'NONE', #37071 ) ;
#48380=FACE_OUTER_BOUND ( 'NONE', #16777, .T. ) ;
#48381=AXIS2_PLACEMENT_3D ( 'NONE', #33074, #30176, #45966 ) ;
#48382=ORIENTED_EDGE ( 'NONE', *, *, #29189, .T. ) ;
#48383=CARTESIAN_POINT ( 'NONE',  ( 55.35935253854128035, -183.6283474603465606, 69.58857822035041352 ) ) ;
#48385=CARTESIAN_POINT ( 'NONE',  ( -16.77927958806651887, -193.5000000000000000, -120.9136869416130082 ) ) ;
#48386=EDGE_CURVE ( 'NONE', #9307, #44982, #38266, .T. ) ;
#48389=DIRECTION ( 'NONE',  ( -0.000000000000000000, 1.000000000000000000, -0.000000000000000000 ) ) ;
#48390=DIRECTION ( 'NONE',  ( -0.000000000000000000, 1.000000000000000000, -0.000000000000000000 ) ) ;
#48391=ORIENTED_EDGE ( 'NONE', *, *, #14447, .T. ) ;
#48392=EDGE_CURVE ( 'NONE', #38149, #3363, #21586, .T. ) ;
#48395=DIRECTION ( 'NONE',  ( 0.4300652022765115712, 0.000000000000000000, 0.9027978299657477557 ) ) ;
#48396=EDGE_CURVE ( 'NONE', #3624, #25977, #37444, .T. ) ;
#48397=DIRECTION ( 'NONE',  ( 0.9785564922995060311, 0.000000000000000000, -0.2059786187410889424 ) ) ;
#48399=AXIS2_PLACEMENT_3D ( 'NONE', #31492, #15220, #39373 ) ;
#48401=DIRECTION ( 'NONE',  ( -0.6528221181905119463, 0.000000000000000000, -0.7575112421616284619 ) ) ;
#48402=FACE_OUTER_BOUND ( 'NONE', #51818, .T. ) ;
#48403=ADVANCED_FACE ( 'NONE', ( #8971 ), #29705, .T. ) ;
#48404=VERTEX_POINT ( 'NONE', #33131 ) ;
#48405=CARTESIAN_POINT ( 'NONE',  ( -160.2705093830644216, -183.6283474603465606, -55.92572546981520532 ) ) ;
#48407=EDGE_LOOP ( 'NONE', ( #34770, #11851, #5713, #30821 ) ) ;
#48410=AXIS2_PLACEMENT_3D ( 'NONE', #16938, #8268, #25091 ) ;
#48411=AXIS2_PLACEMENT_3D ( 'NONE', #45578, #6412, #50036 ) ;
#48412=DIRECTION ( 'NONE',  ( -0.000000000000000000, 1.000000000000000000, -0.000000000000000000 ) ) ;
#48413=CARTESIAN_POINT ( 'NONE',  ( 75.48825557695654709, -193.5000000000000000, 2.844930291601490246 ) ) ;
#48415=CARTESIAN_POINT ( 'NONE',  ( -71.40672220061269115, -193.5000000000000000, -122.8793122007208751 ) ) ;
#48416=CARTESIAN_POINT ( 'NONE',  ( -49.17567778057185990, -193.5000000000000000, 0.7175072570443320474 ) ) ;
#48418=CARTESIAN_POINT ( 'NONE',  ( -48.47912675150885065, -175.3837268820161057, 6.938893903907228378E-15 ) ) ;
#48419=VECTOR ( 'NONE', #12225, 1000.000000000000114 ) ;
#48421=DIRECTION ( 'NONE',  ( -0.000000000000000000, 1.000000000000000000, -0.000000000000000000 ) ) ;
#48422=FACE_OUTER_BOUND ( 'NONE', #15856, .T. ) ;
#48424=ORIENTED_EDGE ( 'NONE', *, *, #34889, .T. ) ;
#48425=CIRCLE ( 'NONE', #50950, 125.0000000000000000 ) ;
#48426=ORIENTED_EDGE ( 'NONE', *, *, #11812, .T. ) ;
#48428=VECTOR ( 'NONE', #823, 1000.000000000000000 ) ;
#48431=FACE_OUTER_BOUND ( 'NONE', #19171, .T. ) ;
#48432=ORIENTED_EDGE ( 'NONE', *, *, #46741, .F. ) ;
#48433=ORIENTED_EDGE ( 'NONE', *, *, #6416, .T. ) ;
#48436=EDGE_CURVE ( 'NONE', #49012, #47168, #21518, .T. ) ;
#48437=EDGE_CURVE ( 'NONE', #47028, #41848, #7220, .T. ) ;
#48439=DIRECTION ( 'NONE',  ( 0.9266896074318317078, 0.000000000000000000, 0.3758275821142421647 ) ) ;
#48440=DIRECTION ( 'NONE',  ( 0.000000000000000000, 0.000000000000000000, 1.000000000000000000 ) ) ;
#48441=ORIENTED_EDGE ( 'NONE', *, *, #35058, .T. ) ;
#48442=VERTEX_POINT ( 'NONE', #27047 ) ;
#48444=ORIENTED_EDGE ( 'NONE', *, *, #30331, .F. ) ;
#48445=DIRECTION ( 'NONE',  ( -0.000000000000000000, 1.000000000000000000, -0.000000000000000000 ) ) ;
#48446=CARTESIAN_POINT ( 'NONE',  ( 63.39453919430263085, -193.5000000000000000, 53.48161459190911415 ) ) ;
#48447=CIRCLE ( 'NONE', #14884, 125.0000000000000000 ) ;
#48448=LINE ( 'NONE', #44238, #1452 ) ;
#48451=EDGE_CURVE ( 'NONE', #14774, #15949, #26797, .T. ) ;
#48452=CARTESIAN_POINT ( 'NONE',  ( -56.71246971489870958, -193.5000000000000000, -124.7285535218267682 ) ) ;
#48453=DIRECTION ( 'NONE',  ( 0.000000000000000000, 0.000000000000000000, 1.000000000000000000 ) ) ;
#48454=ORIENTED_EDGE ( 'NONE', *, *, #6699, .F. ) ;
#48455=FACE_OUTER_BOUND ( 'NONE', #8541, .T. ) ;
#48456=VECTOR ( 'NONE', #11959, 1000.000000000000000 ) ;
#48458=EDGE_CURVE ( 'NONE', #7752, #6661, #26029, .T. ) ;
#48459=CARTESIAN_POINT ( 'NONE',  ( -47.50057025920934706, -189.7472609257535510, -0.2059786187410884151 ) ) ;
#48461=EDGE_CURVE ( 'NONE', #5412, #19912, #6590, .T. ) ;
#48462=EDGE_LOOP ( 'NONE', ( #3853, #17120, #40689, #45345 ) ) ;
#48465=EDGE_LOOP ( 'NONE', ( #43749, #7624, #18975, #46414 ) ) ;
#48466=CARTESIAN_POINT ( 'NONE',  ( 74.31448861501726810, -193.5000000000000000, -23.38221600314288651 ) ) ;
#48467=EDGE_CURVE ( 'NONE', #246, #26523, #6321, .T. ) ;
#48471=LINE ( 'NONE', #12176, #39137 ) ;
#48473=EDGE_CURVE ( 'NONE', #25260, #32165, #47046, .T. ) ;
#48474=DIRECTION ( 'NONE',  ( -0.9995608365087946812, 0.000000000000000000, 0.02963332782254913048 ) ) ;
#48475=ORIENTED_EDGE ( 'NONE', *, *, #37399, .T. ) ;
#48477=VECTOR ( 'NONE', #20267, 1000.000000000000000 ) ;
#48478=EDGE_CURVE ( 'NONE', #22578, #10499, #6067, .T. ) ;
#48479=PLANE ( 'NONE',  #18870 ) ;
#48480=AXIS2_PLACEMENT_3D ( 'NONE', #24203, #274, #3438 ) ;
#48482=CARTESIAN_POINT ( 'NONE',  ( -48.47912675150885065, -183.6283474603465606, 6.938893903907228378E-15 ) ) ;
#48483=EDGE_LOOP ( 'NONE', ( #33936, #19950, #38981, #45351 ) ) ;
#48484=FACE_BOUND ( 'NONE', #1554, .T. ) ;
#48486=VERTEX_POINT ( 'NONE', #46790 ) ;
#48487=DIRECTION ( 'NONE',  ( -0.000000000000000000, 1.000000000000000000, -0.000000000000000000 ) ) ;
#48488=DIRECTION ( 'NONE',  ( 0.000000000000000000, 1.000000000000000000, 0.000000000000000000 ) ) ;
#48489=DIRECTION ( 'NONE',  ( 0.000000000000000000, 1.000000000000000000, 0.000000000000000000 ) ) ;
#48491=EDGE_CURVE ( 'NONE', #41165, #16448, #2384, .T. ) ;
#48492=ORIENTED_EDGE ( 'NONE', *, *, #33148, .T. ) ;
#48495=ORIENTED_EDGE ( 'NONE', *, *, #44539, .T. ) ;
#48503=PLANE ( 'NONE',  #30324 ) ;
#48504=EDGE_CURVE ( 'NONE', #42645, #48757, #46526, .T. ) ;
#48506=VECTOR ( 'NONE', #28249, 1000.000000000000000 ) ;
#48507=ORIENTED_EDGE ( 'NONE', *, *, #48982, .F. ) ;
#48511=CARTESIAN_POINT ( 'NONE',  ( -78.64590280292341617, -193.5000000000000000, -121.3052580173827408 ) ) ;
#48512=AXIS2_PLACEMENT_3D ( 'NONE', #12955, #627, #4567 ) ;
#48513=EDGE_CURVE ( 'NONE', #43312, #11444, #22862, .T. ) ;
#48517=VERTEX_POINT ( 'NONE', #37853 ) ;
#48518=ORIENTED_EDGE ( 'NONE', *, *, #45894, .F. ) ;
#48519=ADVANCED_FACE ( 'NONE', ( #10778 ), #6836, .T. ) ;
#48520=VERTEX_POINT ( 'NONE', #14471 ) ;
#48521=VECTOR ( 'NONE', #43070, 1000.000000000000114 ) ;
#48522=EDGE_CURVE ( 'NONE', #33847, #16474, #16454, .T. ) ;
#48523=CARTESIAN_POINT ( 'NONE',  ( -48.82732838694325750, -177.1207230881787780, 0.9374196611341252261 ) ) ;
#48524=LINE ( 'NONE', #31947, #41104 ) ;
#48525=DIRECTION ( 'NONE',  ( -0.000000000000000000, -1.000000000000000000, 0.000000000000000000 ) ) ;
#48527=CARTESIAN_POINT ( 'NONE',  ( -77.03256798524179771, -189.7472609257535510, 121.6951149130964751 ) ) ;
#48528=ORIENTED_EDGE ( 'NONE', *, *, #29496, .F. ) ;
#48529=ORIENTED_EDGE ( 'NONE', *, *, #43123, .F. ) ;
#48530=DIRECTION ( 'NONE',  ( 0.4566292373937200777, 0.000000000000000000, -0.8896570909947436601 ) ) ;
#48531=ORIENTED_EDGE ( 'NONE', *, *, #16467, .T. ) ;
#48532=LINE ( 'NONE', #12510, #29664 ) ;
#48534=VERTEX_POINT ( 'NONE', #1849 ) ;
#48535=AXIS2_PLACEMENT_3D ( 'NONE', #15178, #47492, #50660 ) ;
#48536=EDGE_CURVE ( 'NONE', #11081, #29368, #17893, .T. ) ;
#48539=CIRCLE ( 'NONE', #15793, 125.0000000000000000 ) ;
#48542=ORIENTED_EDGE ( 'NONE', *, *, #41028, .T. ) ;
#48543=CARTESIAN_POINT ( 'NONE',  ( -170.9948556092908518, -189.7472609257535510, 19.12855698118476511 ) ) ;
#48544=ORIENTED_EDGE ( 'NONE', *, *, #1381, .T. ) ;
#48545=ADVANCED_FACE ( 'NONE', ( #12047 ), #15779, .T. ) ;
#48546=ORIENTED_EDGE ( 'NONE', *, *, #47554, .T. ) ;
#48547=DIRECTION ( 'NONE',  ( -0.000000000000000000, 1.000000000000000000, -0.000000000000000000 ) ) ;
#48549=DIRECTION ( 'NONE',  ( 0.000000000000000000, 0.000000000000000000, -1.000000000000000000 ) ) ;
#48550=DIRECTION ( 'NONE',  ( 0.000000000000000000, 1.000000000000000000, 0.000000000000000000 ) ) ;
#48552=CARTESIAN_POINT ( 'NONE',  ( -63.43218022845228887, -175.3837268820161057, 124.1024020384604540 ) ) ;
#48553=LINE ( 'NONE', #21192, #17011 ) ;
#48555=CARTESIAN_POINT ( 'NONE',  ( -148.0127667507368585, -177.1207230881787780, -75.61781872352626976 ) ) ;
#48557=CARTESIAN_POINT ( 'NONE',  ( -48.65601702663141737, -189.7472609257535510, -0.9842305779475923888 ) ) ;
#48558=FACE_BOUND ( 'NONE', #3121, .T. ) ;
#48563=DIRECTION ( 'NONE',  ( 0.000000000000000000, -1.000000000000000000, 0.000000000000000000 ) ) ;
#48568=CIRCLE ( 'NONE', #31789, 125.0000000000000000 ) ;
#48569=PLANE ( 'NONE',  #46110 ) ;
#48571=ORIENTED_EDGE ( 'NONE', *, *, #46548, .T. ) ;
#48572=VECTOR ( 'NONE', #26831, 1000.000000000000000 ) ;
#48574=ADVANCED_FACE ( 'NONE', ( #35713 ), #43607, .T. ) ;
#48575=DIRECTION ( 'NONE',  ( -0.000000000000000000, 1.000000000000000000, -0.000000000000000000 ) ) ;
#48576=ORIENTED_EDGE ( 'NONE', *, *, #33618, .T. ) ;
#48577=EDGE_LOOP ( 'NONE', ( #45725, #27974, #32524, #40064 ) ) ;
#48578=PLANE ( 'NONE',  #14183 ) ;
#48579=AXIS2_PLACEMENT_3D ( 'NONE', #733, #24138, #23856 ) ;
#48580=ORIENTED_EDGE ( 'NONE', *, *, #39240, .F. ) ;
#48581=DIRECTION ( 'NONE',  ( 0.000000000000000000, 0.000000000000000000, 1.000000000000000000 ) ) ;
#48582=DIRECTION ( 'NONE',  ( -0.000000000000000000, 1.000000000000000000, -0.000000000000000000 ) ) ;
#48583=DIRECTION ( 'NONE',  ( 0.9960498426152165630, 0.000000000000000000, 0.08879589532293852283 ) ) ;
#48584=AXIS2_PLACEMENT_3D ( 'NONE', #29635, #5488, #41982 ) ;
#48586=LINE ( 'NONE', #16787, #2956 ) ;
#48587=EDGE_LOOP ( 'NONE', ( #45711, #12873, #35885, #48819 ) ) ;
#48588=PLANE ( 'NONE',  #36603 ) ;
#48593=CARTESIAN_POINT ( 'NONE',  ( 33.75048693540708911, -193.5000000000000000, 94.14505102712816154 ) ) ;
#48594=VERTEX_POINT ( 'NONE', #28347 ) ;
#48595=PLANE ( 'NONE',  #8820 ) ;
#48596=ORIENTED_EDGE ( 'NONE', *, *, #36716, .F. ) ;
#48597=CARTESIAN_POINT ( 'NONE',  ( -169.0855799822425638, -183.6283474603465606, -28.81338593823979011 ) ) ;
#48598=CARTESIAN_POINT ( 'NONE',  ( 70.19984492582109681, -189.7472609257535510, 39.24667733211968823 ) ) ;
#48602=ORIENTED_EDGE ( 'NONE', *, *, #33614, .T. ) ;
#48603=ADVANCED_FACE ( 'NONE', ( #7858 ), #15238, .T. ) ;
#48604=ORIENTED_EDGE ( 'NONE', *, *, #1216, .F. ) ;
#48608=CARTESIAN_POINT ( 'NONE',  ( -49.35486169370448550, -189.7472609257535510, -0.4827922027307481878 ) ) ;
#48610=CARTESIAN_POINT ( 'NONE',  ( -172.2289551866394106, -175.3837268820161057, -17.63462396184707970 ) ) ;
#48611=AXIS2_PLACEMENT_3D ( 'NONE', #23858, #52006, #15995 ) ;
#48615=EDGE_CURVE ( 'NONE', #12206, #14876, #16269, .T. ) ;
#48616=DIRECTION ( 'NONE',  ( 0.9960498426152171181, 0.000000000000000000, -0.08879589532293157006 ) ) ;
#48621=ORIENTED_EDGE ( 'NONE', *, *, #20174, .F. ) ;
#48622=CARTESIAN_POINT ( 'NONE',  ( -168.3100285466275636, -175.3837268820161057, -31.88354567335001377 ) ) ;
#48623=DIRECTION ( 'NONE',  ( -0.000000000000000000, -1.000000000000000000, 0.000000000000000000 ) ) ;
#48624=DIRECTION ( 'NONE',  ( -0.000000000000000000, 1.000000000000000000, -0.000000000000000000 ) ) ;
#48626=VERTEX_POINT ( 'NONE', #47824 ) ;
#48628=CIRCLE ( 'NONE', #40227, 125.0000000000000000 ) ;
#48629=ADVANCED_FACE ( 'NONE', ( #39901 ), #19683, .F. ) ;
#48630=FACE_OUTER_BOUND ( 'NONE', #8783, .T. ) ;
#48631=CARTESIAN_POINT ( 'NONE',  ( -48.47912675150885065, -189.7472609257535510, 6.938893903907228378E-15 ) ) ;
#48633=DIRECTION ( 'NONE',  ( 0.000000000000000000, -1.000000000000000000, 0.000000000000000000 ) ) ;
#48637=EDGE_CURVE ( 'NONE', #975, #12201, #13106, .T. ) ;
#48638=CARTESIAN_POINT ( 'NONE',  ( -48.47912675150885065, -183.6283474603465606, 6.938893903907228378E-15 ) ) ;
#48639=VERTEX_POINT ( 'NONE', #23125 ) ;
#48640=PLANE ( 'NONE',  #37381 ) ;
#48641=ORIENTED_EDGE ( 'NONE', *, *, #904, .T. ) ;
#48643=VECTOR ( 'NONE', #3555, 1000.000000000000000 ) ;
#48644=EDGE_LOOP ( 'NONE', ( #26380, #10572, #18069, #5074 ) ) ;
#48645=CARTESIAN_POINT ( 'NONE',  ( 48.06131630543706024, -175.3837268820161057, -79.40367028273054473 ) ) ;
#48646=VECTOR ( 'NONE', #8305, 1000.000000000000000 ) ;
#48647=LINE ( 'NONE', #28383, #25044 ) ;
#48652=EDGE_CURVE ( 'NONE', #13513, #3372, #48068, .T. ) ;
#48655=DIRECTION ( 'NONE',  ( 0.000000000000000000, -1.000000000000000000, 0.000000000000000000 ) ) ;
#48656=LINE ( 'NONE', #811, #20757 ) ;
#48659=DIRECTION ( 'NONE',  ( -0.1768902751225802927, 0.000000000000000000, 0.9842305779475953864 ) ) ;
#48660=DIRECTION ( 'NONE',  ( 0.000000000000000000, -1.000000000000000000, 0.000000000000000000 ) ) ;
#48661=CARTESIAN_POINT ( 'NONE',  ( -47.48307690889363641, -193.5000000000000000, -0.08879589532292464504 ) ) ;
#48662=VECTOR ( 'NONE', #15937, 999.9999999999998863 ) ;
#48663=DIRECTION ( 'NONE',  ( -0.9266896074318343723, 0.000000000000000000, 0.3758275821142357809 ) ) ;
#48666=ORIENTED_EDGE ( 'NONE', *, *, #12465, .F. ) ;
#48668=CARTESIAN_POINT ( 'NONE',  ( -99.02518858244150124, -175.3837268820161057, 114.3245189510261497 ) ) ;
#48669=DIRECTION ( 'NONE',  ( -0.000000000000000000, -1.000000000000000000, 0.000000000000000000 ) ) ;
#48672=EDGE_LOOP ( 'NONE', ( #44630, #23953, #3864, #10679 ) ) ;
#48673=CARTESIAN_POINT ( 'NONE',  ( -99.62791064391784346, -193.5000000000000000, -114.0561348912352173 ) ) ;
#48675=AXIS2_PLACEMENT_3D ( 'NONE', #30204, #29937, #2071 ) ;
#48679=ADVANCED_FACE ( 'NONE', ( #36230 ), #32282, .T. ) ;
#48682=CARTESIAN_POINT ( 'NONE',  ( -89.73513343757494454, -183.6283474603465606, -117.9955164924467397 ) ) ;
#48684=CARTESIAN_POINT ( 'NONE',  ( -154.6193097927903182, -189.7472609257535510, -66.02470404298122730 ) ) ;
#48685=DIRECTION ( 'NONE',  ( -0.000000000000000000, 1.000000000000000000, -0.000000000000000000 ) ) ;
#48690=EDGE_CURVE ( 'NONE', #3147, #25168, #28165, .T. ) ;
#48691=AXIS2_PLACEMENT_3D ( 'NONE', #34783, #46382, #23493 ) ;
#48693=DIRECTION ( 'NONE',  ( 0.000000000000000000, 0.000000000000000000, -1.000000000000000000 ) ) ;
#48694=VERTEX_POINT ( 'NONE', #37276 ) ;
#48695=VERTEX_POINT ( 'NONE', #13622 ) ;
#48703=LINE ( 'NONE', #44754, #8159 ) ;
#48704=DIRECTION ( 'NONE',  ( -0.000000000000000000, 1.000000000000000000, -0.000000000000000000 ) ) ;
#48705=DIRECTION ( 'NONE',  ( 0.000000000000000000, 0.000000000000000000, -1.000000000000000000 ) ) ;
#48707=CIRCLE ( 'NONE', #3374, 125.0000000000000000 ) ;
#48708=DIRECTION ( 'NONE',  ( 0.000000000000000000, 1.000000000000000000, 0.000000000000000000 ) ) ;
#48709=CARTESIAN_POINT ( 'NONE',  ( -25.55153130240594450, -189.7472609257535510, 122.8793122007210741 ) ) ;
#48710=ORIENTED_EDGE ( 'NONE', *, *, #12471, .F. ) ;
#48714=DIRECTION ( 'NONE',  ( 0.5085311186492216251, 0.000000000000000000, -0.8610436117673548884 ) ) ;
#48715=DIRECTION ( 'NONE',  ( -0.5338233779647887367, 0.000000000000000000, -0.8455960035018273979 ) ) ;
#48717=ORIENTED_EDGE ( 'NONE', *, *, #14336, .T. ) ;
#48718=FACE_OUTER_BOUND ( 'NONE', #9082, .T. ) ;
#48719=DIRECTION ( 'NONE',  ( -0.000000000000000000, 1.000000000000000000, -0.000000000000000000 ) ) ;
#48720=ORIENTED_EDGE ( 'NONE', *, *, #41361, .T. ) ;
#48722=PLANE ( 'NONE',  #48046 ) ;
#48726=AXIS2_PLACEMENT_3D ( 'NONE', #30273, #25817, #14777 ) ;
#48728=ORIENTED_EDGE ( 'NONE', *, *, #16324, .F. ) ;
#48730=ORIENTED_EDGE ( 'NONE', *, *, #51118, .T. ) ;
#48732=CARTESIAN_POINT ( 'NONE',  ( 75.32224018181403835, -193.5000000000000000, 7.024906801079474405 ) ) ;
#48735=CARTESIAN_POINT ( 'NONE',  ( 71.87891646118019651, -175.3837268820161057, -33.74820638215423685 ) ) ;
#48738=CARTESIAN_POINT ( 'NONE',  ( -49.21696003055057389, -193.5000000000000000, -0.6749830015182127774 ) ) ;
#48740=DIRECTION ( 'NONE',  ( 0.000000000000000000, -1.000000000000000000, 0.000000000000000000 ) ) ;
#48743=DIRECTION ( 'NONE',  ( 0.000000000000000000, -1.000000000000000000, 0.000000000000000000 ) ) ;
#48744=ORIENTED_EDGE ( 'NONE', *, *, #2892, .T. ) ;
#48745=EDGE_LOOP ( 'NONE', ( #10696, #25804, #37047, #48977 ) ) ;
#48747=EDGE_CURVE ( 'NONE', #12568, #33588, #49118, .T. ) ;
#48748=CARTESIAN_POINT ( 'NONE',  ( -49.42645310536303782, -189.7472609257535510, -0.3202698538628417357 ) ) ;
#48749=FACE_OUTER_BOUND ( 'NONE', #23645, .T. ) ;
#48750=ORIENTED_EDGE ( 'NONE', *, *, #22003, .T. ) ;
#48752=ORIENTED_EDGE ( 'NONE', *, *, #41674, .T. ) ;
#48755=EDGE_CURVE ( 'NONE', #467, #38948, #8385, .T. ) ;
#48757=VERTEX_POINT ( 'NONE', #1540 ) ;
#48758=EDGE_CURVE ( 'NONE', #31354, #26252, #13368, .T. ) ;
#48760=VERTEX_POINT ( 'NONE', #8897 ) ;
#48762=CARTESIAN_POINT ( 'NONE',  ( -48.47912675150885065, -175.3837268820161057, 6.938893903907228378E-15 ) ) ;
#48763=AXIS2_PLACEMENT_3D ( 'NONE', #51083, #23708, #19757 ) ;
#48764=ADVANCED_FACE ( 'NONE', ( #8639 ), #24938, .T. ) ;
#48765=DIRECTION ( 'NONE',  ( -0.000000000000000000, 1.000000000000000000, -0.000000000000000000 ) ) ;
#48766=DIRECTION ( 'NONE',  ( 0.000000000000000000, 0.000000000000000000, 1.000000000000000000 ) ) ;
#48767=VERTEX_POINT ( 'NONE', #40679 ) ;
#48769=CIRCLE ( 'NONE', #33634, 125.0000000000000000 ) ;
#48770=ORIENTED_EDGE ( 'NONE', *, *, #15136, .F. ) ;
#48772=CARTESIAN_POINT ( 'NONE',  ( 76.31829002442924548, -193.5000000000000000, 7.113702696402420145 ) ) ;
#48773=LINE ( 'NONE', #12742, #48646 ) ;
#48775=DIRECTION ( 'NONE',  ( -0.1182731709213730997, 0.000000000000000000, 0.9929810960135161402 ) ) ;
#48776=VERTEX_POINT ( 'NONE', #1011 ) ;
#48777=EDGE_CURVE ( 'NONE', #35850, #10308, #4702, .T. ) ;
#48779=FACE_OUTER_BOUND ( 'NONE', #10201, .T. ) ;
#48780=ORIENTED_EDGE ( 'NONE', *, *, #26463, .T. ) ;
#48782=AXIS2_PLACEMENT_3D ( 'NONE', #37112, #28956, #17687 ) ;
#48783=DIRECTION ( 'NONE',  ( 0.6528221181905174975, 0.000000000000000000, 0.7575112421616236880 ) ) ;
#48784=PLANE ( 'NONE',  #34204 ) ;
#48785=CARTESIAN_POINT ( 'NONE',  ( 66.03142248012325410, -193.5000000000000000, 50.12318939044039467 ) ) ;
#48786=FACE_OUTER_BOUND ( 'NONE', #8230, .T. ) ;
#48788=CARTESIAN_POINT ( 'NONE',  ( 73.62243227112293198, -177.1207230881787780, 21.61797988633237821 ) ) ;
#48789=ORIENTED_EDGE ( 'NONE', *, *, #10213, .F. ) ;
#48790=ADVANCED_FACE ( 'NONE', ( #44910 ), #481, .T. ) ;
#48793=CARTESIAN_POINT ( 'NONE',  ( 32.49319223169170812, -175.3837268820161057, -95.22858582633060109 ) ) ;
#48794=DIRECTION ( 'NONE',  ( 0.000000000000000000, -1.000000000000000000, 0.000000000000000000 ) ) ;
#48795=FACE_OUTER_BOUND ( 'NONE', #1778, .T. ) ;
#48796=AXIS2_PLACEMENT_3D ( 'NONE', #33017, #37740, #29334 ) ;
#48797=EDGE_CURVE ( 'NONE', #44067, #30050, #28950, .T. ) ;
#48799=CARTESIAN_POINT ( 'NONE',  ( -171.1451123608488274, -189.7472609257535510, 18.13990644964088261 ) ) ;
#48800=EDGE_CURVE ( 'NONE', #38881, #49882, #13888, .T. ) ;
#48802=CARTESIAN_POINT ( 'NONE',  ( 75.48400724637754422, -183.6283474603465606, -16.06677968424457248 ) ) ;
#48803=EDGE_CURVE ( 'NONE', #840, #20061, #9951, .T. ) ;
#48805=DIRECTION ( 'NONE',  ( 0.000000000000000000, 0.000000000000000000, -1.000000000000000000 ) ) ;
#48806=DIRECTION ( 'NONE',  ( 0.000000000000000000, 0.000000000000000000, -1.000000000000000000 ) ) ;
#48808=VECTOR ( 'NONE', #31211, 999.9999999999998863 ) ;
#48809=LINE ( 'NONE', #1740, #21964 ) ;
#48810=FACE_BOUND ( 'NONE', #33615, .T. ) ;
#48812=EDGE_CURVE ( 'NONE', #40042, #11813, #46216, .T. ) ;
#48813=CARTESIAN_POINT ( 'NONE',  ( -58.29063029684667185, -193.5000000000000000, 124.6143426664034877 ) ) ;
#48818=ADVANCED_FACE ( 'NONE', ( #6780 ), #10193, .F. ) ;
#48819=ORIENTED_EDGE ( 'NONE', *, *, #24333, .T. ) ;
#48820=CIRCLE ( 'NONE', #23621, 125.0000000000000000 ) ;
#48821=EDGE_CURVE ( 'NONE', #38934, #23682, #25966, .T. ) ;
#48823=AXIS2_PLACEMENT_3D ( 'NONE', #13991, #1377, #41054 ) ;
#48826=LINE ( 'NONE', #49344, #9498 ) ;
#48827=ORIENTED_EDGE ( 'NONE', *, *, #35402, .T. ) ;
#48830=ORIENTED_EDGE ( 'NONE', *, *, #20210, .F. ) ;
#48831=EDGE_CURVE ( 'NONE', #45569, #33712, #33850, .T. ) ;
#48832=VERTEX_POINT ( 'NONE', #45963 ) ;
#48833=DIRECTION ( 'NONE',  ( 0.000000000000000000, 1.000000000000000000, 0.000000000000000000 ) ) ;
#48834=LINE ( 'NONE', #8868, #7534 ) ;
#48835=VERTEX_POINT ( 'NONE', #41742 ) ;
#48836=CARTESIAN_POINT ( 'NONE',  ( 71.35177504360963496, -189.7472609257535510, 31.88354567335082024 ) ) ;
#48838=AXIS2_PLACEMENT_3D ( 'NONE', #3713, #31574, #20521 ) ;
#48839=VECTOR ( 'NONE', #47703, 1000.000000000000000 ) ;
#48840=AXIS2_PLACEMENT_3D ( 'NONE', #9257, #1631, #25278 ) ;
#48841=EDGE_CURVE ( 'NONE', #41328, #19801, #2323, .T. ) ;
#48843=CARTESIAN_POINT ( 'NONE',  ( -48.47912675150885065, -189.7472609257535510, 6.938893903907228378E-15 ) ) ;
#48845=DIRECTION ( 'NONE',  ( 0.000000000000000000, -1.000000000000000000, 0.000000000000000000 ) ) ;
#48847=EDGE_LOOP ( 'NONE', ( #5813, #13501, #17849, #40546 ) ) ;
#48848=ORIENTED_EDGE ( 'NONE', *, *, #44811, .F. ) ;
#48849=CARTESIAN_POINT ( 'NONE',  ( 65.52619748798556998, -193.5000000000000000, 48.77484799213969069 ) ) ;
#48852=ORIENTED_EDGE ( 'NONE', *, *, #20484, .T. ) ;
#48853=CARTESIAN_POINT ( 'NONE',  ( -49.30901192927172616, -175.3837268820161057, -124.9972451320097093 ) ) ;
#48854=LINE ( 'NONE', #29118, #34286 ) ;
#48858=ORIENTED_EDGE ( 'NONE', *, *, #23043, .F. ) ;
#48859=AXIS2_PLACEMENT_3D ( 'NONE', #23717, #39724, #19767 ) ;
#48860=VERTEX_POINT ( 'NONE', #18355 ) ;
#48861=FACE_OUTER_BOUND ( 'NONE', #25962, .T. ) ;
#48863=CARTESIAN_POINT ( 'NONE',  ( -238.7407812814481076, -213.5000000000000000, 10.00000000000000178 ) ) ;
#48865=CARTESIAN_POINT ( 'NONE',  ( -137.2624501260119700, -177.1207230881787780, 87.99159897727969337 ) ) ;
#48868=DIRECTION ( 'NONE',  ( 0.000000000000000000, -1.000000000000000000, 0.000000000000000000 ) ) ;
#48871=PLANE ( 'NONE',  #38773 ) ;
#48872=CARTESIAN_POINT ( 'NONE',  ( -111.8989814360438686, -189.7472609257535510, -107.7168604805787169 ) ) ;
#48873=DIRECTION ( 'NONE',  ( 0.000000000000000000, -1.000000000000000000, 0.000000000000000000 ) ) ;
#48875=ORIENTED_EDGE ( 'NONE', *, *, #43217, .F. ) ;
#48876=ORIENTED_EDGE ( 'NONE', *, *, #15111, .T. ) ;
#48877=DIRECTION ( 'NONE',  ( 0.8455960035018272869, 0.000000000000000000, -0.5338233779647886257 ) ) ;
#48878=AXIS2_PLACEMENT_3D ( 'NONE', #27818, #8123, #19427 ) ;
#48879=DIRECTION ( 'NONE',  ( 0.000000000000000000, 0.000000000000000000, -1.000000000000000000 ) ) ;
#48880=FACE_OUTER_BOUND ( 'NONE', #12723, .T. ) ;
#48881=ORIENTED_EDGE ( 'NONE', *, *, #23597, .F. ) ;
#48885=DIRECTION ( 'NONE',  ( 0.000000000000000000, 0.000000000000000000, 1.000000000000000000 ) ) ;
#48886=FACE_OUTER_BOUND ( 'NONE', #1115, .T. ) ;
#48887=EDGE_CURVE ( 'NONE', #11654, #46759, #50664, .T. ) ;
#48888=DIRECTION ( 'NONE',  ( 0.000000000000000000, -1.000000000000000000, 0.000000000000000000 ) ) ;
#48889=CARTESIAN_POINT ( 'NONE',  ( -48.47912675150885065, -177.1207230881787780, 6.938893903907228378E-15 ) ) ;
#48895=EDGE_CURVE ( 'NONE', #30411, #31046, #38570, .T. ) ;
#48897=ORIENTED_EDGE ( 'NONE', *, *, #51976, .F. ) ;
#48898=CIRCLE ( 'NONE', #30416, 125.0000000000000000 ) ;
#48899=AXIS2_PLACEMENT_3D ( 'NONE', #23031, #3060, #39564 ) ;
#48900=ORIENTED_EDGE ( 'NONE', *, *, #36200, .T. ) ;
#48901=CARTESIAN_POINT ( 'NONE',  ( -48.47912675150885065, -177.1207230881787780, 6.938893903907228378E-15 ) ) ;
#48903=DIRECTION ( 'NONE',  ( 0.000000000000000000, 0.000000000000000000, 1.000000000000000000 ) ) ;
#48905=CARTESIAN_POINT ( 'NONE',  ( -80.85382946868861609, -193.5000000000000000, 119.6996507684852986 ) ) ;
#48906=ORIENTED_EDGE ( 'NONE', *, *, #19549, .F. ) ;
#48907=DIRECTION ( 'NONE',  ( 0.8610436117673585521, 0.000000000000000000, -0.5085311186492154079 ) ) ;
#48909=DIRECTION ( 'NONE',  ( 0.000000000000000000, 0.000000000000000000, -1.000000000000000000 ) ) ;
#48911=CARTESIAN_POINT ( 'NONE',  ( -48.47912675150885065, -177.1207230881787780, 6.938893903907228378E-15 ) ) ;
#48912=EDGE_LOOP ( 'NONE', ( #781, #29145, #51688, #28762 ) ) ;
#48914=DIRECTION ( 'NONE',  ( -0.000000000000000000, 1.000000000000000000, -0.000000000000000000 ) ) ;
#48915=DIRECTION ( 'NONE',  ( -0.6068001458185834363, 0.000000000000000000, -0.7948544414133608127 ) ) ;
#48916=ORIENTED_EDGE ( 'NONE', *, *, #49984, .F. ) ;
#48918=FACE_OUTER_BOUND ( 'NONE', #5864, .T. ) ;
#48919=FACE_OUTER_BOUND ( 'NONE', #31817, .T. ) ;
#48924=EDGE_LOOP ( 'NONE', ( #5772, #24568, #38164, #45622 ) ) ;
#48927=DIRECTION ( 'NONE',  ( 0.000000000000000000, -0.000000000000000000, -1.000000000000000000 ) ) ;
#48929=VERTEX_POINT ( 'NONE', #2570 ) ;
#48931=CIRCLE ( 'NONE', #29595, 125.0000000000000000 ) ;
#48935=CARTESIAN_POINT ( 'NONE',  ( -117.0614752283615161, -175.3837268820161057, 103.3076327631967786 ) ) ;
#48937=VECTOR ( 'NONE', #47268, 1000.000000000000000 ) ;
#48939=CARTESIAN_POINT ( 'NONE',  ( 68.24201764719070695, -183.6283474603465606, -44.73448837594910543 ) ) ;
#48940=EDGE_CURVE ( 'NONE', #7798, #28664, #14659, .T. ) ;
#48941=DIRECTION ( 'NONE',  ( 0.000000000000000000, 0.000000000000000000, 1.000000000000000000 ) ) ;
#48943=ORIENTED_EDGE ( 'NONE', *, *, #12653, .T. ) ;
#48944=VECTOR ( 'NONE', #12252, 999.9999999999998863 ) ;
#48945=ORIENTED_EDGE ( 'NONE', *, *, #15823, .F. ) ;
#48947=AXIS2_PLACEMENT_3D ( 'NONE', #22701, #50826, #38714 ) ;
#48948=LINE ( 'NONE', #46055, #20422 ) ;
#48951=ORIENTED_EDGE ( 'NONE', *, *, #20558, .F. ) ;
#48955=AXIS2_PLACEMENT_3D ( 'NONE', #17405, #33428, #51782 ) ;
#48959=DIRECTION ( 'NONE',  ( 0.000000000000000000, -0.000000000000000000, 1.000000000000000000 ) ) ;
#48960=CYLINDRICAL_SURFACE ( 'NONE', #46772, 125.0000000000000000 ) ;
#48961=VERTEX_POINT ( 'NONE', #45693 ) ;
#48962=VECTOR ( 'NONE', #12129, 1000.000000000000000 ) ;
#48963=DIRECTION ( 'NONE',  ( 0.000000000000000000, 1.000000000000000000, 0.000000000000000000 ) ) ;
#48966=VERTEX_POINT ( 'NONE', #9682 ) ;
#48970=DIRECTION ( 'NONE',  ( 0.000000000000000000, 1.000000000000000000, -0.000000000000000000 ) ) ;
#48971=DIRECTION ( 'NONE',  ( 0.000000000000000000, 0.000000000000000000, 1.000000000000000000 ) ) ;
#48972=ADVANCED_FACE ( 'NONE', ( #19125 ), #36897, .T. ) ;
#48974=ORIENTED_EDGE ( 'NONE', *, *, #45603, .T. ) ;
#48975=DIRECTION ( 'NONE',  ( 0.000000000000000000, 0.000000000000000000, -1.000000000000000000 ) ) ;
#48977=ORIENTED_EDGE ( 'NONE', *, *, #23994, .T. ) ;
#48979=VECTOR ( 'NONE', #20334, 1000.000000000000000 ) ;
#48981=VERTEX_POINT ( 'NONE', #27516 ) ;
#48982=EDGE_CURVE ( 'NONE', #16149, #23737, #51196, .T. ) ;
#48983=DIRECTION ( 'NONE',  ( 0.000000000000000000, -0.000000000000000000, 1.000000000000000000 ) ) ;
#48984=ADVANCED_FACE ( 'NONE', ( #26992 ), #48479, .F. ) ;
#48987=ORIENTED_EDGE ( 'NONE', *, *, #10213, .T. ) ;
#48990=FACE_BOUND ( 'NONE', #18780, .T. ) ;
#48991=ADVANCED_FACE ( 'NONE', ( #39073 ), #7549, .T. ) ;
#48992=DIRECTION ( 'NONE',  ( -0.9960498426152171181, 0.000000000000000000, 0.08879589532293157006 ) ) ;
#48994=LINE ( 'NONE', #33211, #28176 ) ;
#48997=VECTOR ( 'NONE', #20856, 1000.000000000000000 ) ;
#48999=ORIENTED_EDGE ( 'NONE', *, *, #49031, .T. ) ;
#49001=ORIENTED_EDGE ( 'NONE', *, *, #20518, .T. ) ;
#49003=VECTOR ( 'NONE', #23563, 1000.000000000000000 ) ;
#49004=EDGE_CURVE ( 'NONE', #14774, #25561, #7294, .T. ) ;
#49005=DIRECTION ( 'NONE',  ( -0.000000000000000000, -0.000000000000000000, -1.000000000000000000 ) ) ;
#49007=ORIENTED_EDGE ( 'NONE', *, *, #6757, .F. ) ;
#49010=CARTESIAN_POINT ( 'NONE',  ( -173.4787860028527007, -193.5000000000000000, 0.2918682030023981300 ) ) ;
#49011=LINE ( 'NONE', #42082, #13444 ) ;
#49012=VERTEX_POINT ( 'NONE', #7033 ) ;
#49015=DIRECTION ( 'NONE',  ( 0.000000000000000000, -1.000000000000000000, 0.000000000000000000 ) ) ;
#49016=CARTESIAN_POINT ( 'NONE',  ( 54.54686566053560881, -193.5000000000000000, 69.00559874123594284 ) ) ;
#49018=CARTESIAN_POINT ( 'NONE',  ( -160.9694636715425702, -189.7472609257535510, 54.50618404931040573 ) ) ;
#49019=CARTESIAN_POINT ( 'NONE',  ( -47.60339180931321579, -193.5000000000000000, -0.4827922027307358088 ) ) ;
#49021=ORIENTED_EDGE ( 'NONE', *, *, #46036, .F. ) ;
#49022=VECTOR ( 'NONE', #23336, 999.9999999999998863 ) ;
#49024=FACE_OUTER_BOUND ( 'NONE', #2731, .T. ) ;
#49025=DIRECTION ( 'NONE',  ( -0.9890401873221644768, 0.000000000000000000, 0.1476465640024779702 ) ) ;
#49028=DIRECTION ( 'NONE',  ( 0.000000000000000000, -1.000000000000000000, 0.000000000000000000 ) ) ;
#49029=VERTEX_POINT ( 'NONE', #30943 ) ;
#49030=EDGE_CURVE ( 'NONE', #35703, #45018, #44046, .T. ) ;
#49031=EDGE_CURVE ( 'NONE', #50633, #3034, #14934, .T. ) ;
#49032=VECTOR ( 'NONE', #21230, 1000.000000000000000 ) ;
#49033=EDGE_LOOP ( 'NONE', ( #17813, #37396, #16197, #14247 ) ) ;
#49034=CARTESIAN_POINT ( 'NONE',  ( 69.66827051661184100, -175.3837268820161057, -40.81902153125260213 ) ) ;
#49035=VERTEX_POINT ( 'NONE', #20872 ) ;
#49036=DIRECTION ( 'NONE',  ( 0.000000000000000000, -0.000000000000000000, -1.000000000000000000 ) ) ;
#49037=ORIENTED_EDGE ( 'NONE', *, *, #42316, .T. ) ;
#49038=DIRECTION ( 'NONE',  ( 0.000000000000000000, 0.000000000000000000, 1.000000000000000000 ) ) ;
#49039=PLANE ( 'NONE',  #49333 ) ;
#49042=LINE ( 'NONE', #20393, #45262 ) ;
#49045=VERTEX_POINT ( 'NONE', #46987 ) ;
#49047=ORIENTED_EDGE ( 'NONE', *, *, #36515, .F. ) ;
#49049=ADVANCED_FACE ( 'NONE', ( #23060 ), #35391, .T. ) ;
#49050=DIRECTION ( 'NONE',  ( 0.000000000000000000, -1.000000000000000000, 0.000000000000000000 ) ) ;
#49051=AXIS2_PLACEMENT_3D ( 'NONE', #1658, #45803, #40800 ) ;
#49055=CARTESIAN_POINT ( 'NONE',  ( 21.49274850782855495, -175.3837268820161057, -103.5805805771126558 ) ) ;
#49056=FACE_OUTER_BOUND ( 'NONE', #5169, .T. ) ;
#49057=VERTEX_POINT ( 'NONE', #31451 ) ;
#49058=CARTESIAN_POINT ( 'NONE',  ( -68.21229068036657850, -193.5000000000000000, -123.4325817657429809 ) ) ;
#49059=PLANE ( 'NONE',  #26519 ) ;
#49060=CARTESIAN_POINT ( 'NONE',  ( -48.47912675150885065, -175.3837268820161057, 6.938893903907228378E-15 ) ) ;
#49061=FACE_BOUND ( 'NONE', #49575, .T. ) ;
#49067=DIRECTION ( 'NONE',  ( 0.9646355819083576311, 0.000000000000000000, 0.2635871660690715101 ) ) ;
#49068=AXIS2_PLACEMENT_3D ( 'NONE', #39565, #51683, #24084 ) ;
#49070=CARTESIAN_POINT ( 'NONE',  ( -151.1459075827612537, -183.6283474603465606, 69.53890913632950799 ) ) ;
#49073=ORIENTED_EDGE ( 'NONE', *, *, #47195, .T. ) ;
#49075=EDGE_LOOP ( 'NONE', ( #3014, #41113, #40073, #42133 ) ) ;
#49076=ORIENTED_EDGE ( 'NONE', *, *, #15735, .F. ) ;
#49080=CARTESIAN_POINT ( 'NONE',  ( -107.6930423737362190, -193.5000000000000000, 110.0850225811110761 ) ) ;
#49082=EDGE_LOOP ( 'NONE', ( #43982, #40992, #26699, #9605 ) ) ;
#49083=CARTESIAN_POINT ( 'NONE',  ( -48.47912675150883643, -193.5000000000000000, -125.0000000000000000 ) ) ;
#49084=AXIS2_PLACEMENT_3D ( 'NONE', #50464, #46514, #26787 ) ;
#49085=LINE ( 'NONE', #39431, #46311 ) ;
#49086=CARTESIAN_POINT ( 'NONE',  ( 34.93559171950835918, -177.1207230881787780, -93.09664195018496002 ) ) ;
#49087=EDGE_LOOP ( 'NONE', ( #29399, #42869, #31498, #17785 ) ) ;
#49088=VECTOR ( 'NONE', #19766, 1000.000000000000000 ) ;
#49091=EDGE_CURVE ( 'NONE', #39789, #36788, #12700, .T. ) ;
#49093=EDGE_CURVE ( 'NONE', #25190, #50966, #7136, .T. ) ;
#49095=DIRECTION ( 'NONE',  ( 0.000000000000000000, 1.000000000000000000, 0.000000000000000000 ) ) ;
#49099=ORIENTED_EDGE ( 'NONE', *, *, #46587, .T. ) ;
#49103=CARTESIAN_POINT ( 'NONE',  ( -27.18512803868276251, -193.5000000000000000, -123.1729094355498404 ) ) ;
#49108=CARTESIAN_POINT ( 'NONE',  ( -169.6719064342497632, -193.5000000000000000, 30.61552143554992256 ) ) ;
#49109=FACE_OUTER_BOUND ( 'NONE', #22897, .T. ) ;
#49110=ORIENTED_EDGE ( 'NONE', *, *, #43935, .T. ) ;
#49112=DIRECTION ( 'NONE',  ( 0.000000000000000000, -0.000000000000000000, 1.000000000000000000 ) ) ;
#49113=AXIS2_PLACEMENT_3D ( 'NONE', #51123, #31888, #51364 ) ;
#49114=VERTEX_POINT ( 'NONE', #5104 ) ;
#49115=ADVANCED_FACE ( 'NONE', ( #46093 ), #17461, .F. ) ;
#49116=ORIENTED_EDGE ( 'NONE', *, *, #33251, .F. ) ;
#49118=LINE ( 'NONE', #45188, #23083 ) ;
#49120=CARTESIAN_POINT ( 'NONE',  ( -56.65322908700500903, -193.5000000000000000, -123.7303097900624493 ) ) ;
#49122=DIRECTION ( 'NONE',  ( 0.000000000000000000, 0.000000000000000000, 1.000000000000000000 ) ) ;
#49126=DIRECTION ( 'NONE',  ( 0.5586467658036594619, 0.000000000000000000, -0.8294056854501971054 ) ) ;
#49127=DIRECTION ( 'NONE',  ( 0.000000000000000000, 0.000000000000000000, 1.000000000000000000 ) ) ;
#49128=CARTESIAN_POINT ( 'NONE',  ( 65.38692482895589819, -177.1207230881787780, -51.57055649762702387 ) ) ;
#49130=DIRECTION ( 'NONE',  ( -0.000000000000000000, 1.000000000000000000, -0.000000000000000000 ) ) ;
#49133=AXIS2_PLACEMENT_3D ( 'NONE', #51979, #48275, #43554 ) ;
#49138=EDGE_LOOP ( 'NONE', ( #41905, #21045, #7244, #1847 ) ) ;
#49139=EDGE_CURVE ( 'NONE', #40790, #13171, #29769, .T. ) ;
#49140=VECTOR ( 'NONE', #1997, 1000.000000000000000 ) ;
#49141=DIRECTION ( 'NONE',  ( -0.9995608365087940150, 0.000000000000000000, -0.02963332782257007206 ) ) ;
#49143=VECTOR ( 'NONE', #49615, 1000.000000000000114 ) ;
#49144=CARTESIAN_POINT ( 'NONE',  ( -123.4791267515088435, -198.5000000000000000, 80.00000000000000000 ) ) ;
#49145=DIRECTION ( 'NONE',  ( -0.6068001458185834363, 0.000000000000000000, -0.7948544414133608127 ) ) ;
#49149=LINE ( 'NONE', #24441, #47846 ) ;
#49150=DIRECTION ( 'NONE',  ( 0.9266896074318343723, 0.000000000000000000, -0.3758275821142357809 ) ) ;
#49151=VERTEX_POINT ( 'NONE', #17712 ) ;
#49152=AXIS2_PLACEMENT_3D ( 'NONE', #17169, #48970, #32916 ) ;
#49153=DIRECTION ( 'NONE',  ( 0.000000000000000000, 1.000000000000000000, -0.000000000000000000 ) ) ;
#49158=EDGE_CURVE ( 'NONE', #49151, #32802, #5584, .T. ) ;
#49159=EDGE_CURVE ( 'NONE', #28151, #13401, #32933, .T. ) ;
#49160=PLANE ( 'NONE',  #17515 ) ;
#49164=ORIENTED_EDGE ( 'NONE', *, *, #48030, .F. ) ;
#49166=CIRCLE ( 'NONE', #23131, 125.0000000000000000 ) ;
#49167=ORIENTED_EDGE ( 'NONE', *, *, #21395, .T. ) ;
#49168=FACE_OUTER_BOUND ( 'NONE', #35232, .T. ) ;
#49172=CARTESIAN_POINT ( 'NONE',  ( -81.14588623932559130, -177.1207230881787780, 120.6560517527618117 ) ) ;
#49173=CARTESIAN_POINT ( 'NONE',  ( -12.76653800058364574, -189.7472609257535510, -119.7898618611244927 ) ) ;
#49174=DIRECTION ( 'NONE',  ( 0.000000000000000000, -1.000000000000000000, 0.000000000000000000 ) ) ;
#49175=ORIENTED_EDGE ( 'NONE', *, *, #15375, .T. ) ;
#49176=CARTESIAN_POINT ( 'NONE',  ( -5.142695285147754980, -189.7472609257535510, -116.1806952091177578 ) ) ;
#49178=CARTESIAN_POINT ( 'NONE',  ( -106.4764934152196645, -193.5000000000000000, 110.7307791902282759 ) ) ;
#49181=AXIS2_PLACEMENT_3D ( 'NONE', #27367, #27876, #23942 ) ;
#49182=CYLINDRICAL_SURFACE ( 'NONE', #38402, 125.0000000000000000 ) ;
#49183=DIRECTION ( 'NONE',  ( 0.000000000000000000, 0.000000000000000000, -1.000000000000000000 ) ) ;
#49185=VECTOR ( 'NONE', #15642, 1000.000000000000000 ) ;
#49186=DIRECTION ( 'NONE',  ( -0.5586467658036594619, 0.000000000000000000, 0.8294056854501971054 ) ) ;
#49188=AXIS2_PLACEMENT_3D ( 'NONE', #32544, #20193, #44108 ) ;
#49192=CIRCLE ( 'NONE', #24866, 125.0000000000000000 ) ;
#49194=ORIENTED_EDGE ( 'NONE', *, *, #12653, .F. ) ;
#49195=LINE ( 'NONE', #46043, #41568 ) ;
#49196=DIRECTION ( 'NONE',  ( 0.000000000000000000, -1.000000000000000000, 0.000000000000000000 ) ) ;
#49197=DIRECTION ( 'NONE',  ( 0.000000000000000000, 1.000000000000000000, 0.000000000000000000 ) ) ;
#49198=DIRECTION ( 'NONE',  ( 0.000000000000000000, -1.000000000000000000, 0.000000000000000000 ) ) ;
#49199=FACE_OUTER_BOUND ( 'NONE', #45257, .T. ) ;
#49200=AXIS2_PLACEMENT_3D ( 'NONE', #11491, #11746, #24116 ) ;
#49201=VECTOR ( 'NONE', #46728, 1000.000000000000114 ) ;
#49202=CARTESIAN_POINT ( 'NONE',  ( -169.8550585387149852, -193.5000000000000000, 25.37485791684384751 ) ) ;
#49203=DIRECTION ( 'NONE',  ( 0.000000000000000000, 0.000000000000000000, 1.000000000000000000 ) ) ;
#49205=ORIENTED_EDGE ( 'NONE', *, *, #13436, .T. ) ;
#49207=AXIS2_PLACEMENT_3D ( 'NONE', #4513, #32094, #3994 ) ;
#49210=LINE ( 'NONE', #29734, #22948 ) ;
#49216=LINE ( 'NONE', #21350, #4903 ) ;
#49217=VECTOR ( 'NONE', #18297, 1000.000000000000000 ) ;
#49220=CARTESIAN_POINT ( 'NONE',  ( -123.8574911141017765, -175.3837268820161057, 98.45863302693528851 ) ) ;
#49222=CARTESIAN_POINT ( 'NONE',  ( -155.4465502054561057, -177.1207230881787780, 64.67588669375881238 ) ) ;
#49224=AXIS2_PLACEMENT_3D ( 'NONE', #42634, #19480, #14267 ) ;
#49225=DIRECTION ( 'NONE',  ( -0.9995608365087940150, 0.000000000000000000, -0.02963332782257007206 ) ) ;
#49226=CARTESIAN_POINT ( 'NONE',  ( -172.4195137048758397, -193.5000000000000000, -3.844569333772363873 ) ) ;
#49227=VERTEX_POINT ( 'NONE', #17964 ) ;
#49229=ORIENTED_EDGE ( 'NONE', *, *, #49400, .F. ) ;
#49232=CARTESIAN_POINT ( 'NONE',  ( 51.65665342072240662, -183.6283474603465606, 74.81861753132422166 ) ) ;
#49233=PLANE ( 'NONE',  #9527 ) ;
#49234=DIRECTION ( 'NONE',  ( -0.9473263538541876194, 0.000000000000000000, -0.3202698538628486746 ) ) ;
#49235=ORIENTED_EDGE ( 'NONE', *, *, #11825, .F. ) ;
#49237=ORIENTED_EDGE ( 'NONE', *, *, #42262, .F. ) ;
#49239=AXIS2_PLACEMENT_3D ( 'NONE', #49528, #9315, #5642 ) ;
#49240=LINE ( 'NONE', #37395, #27532 ) ;
#49243=DIRECTION ( 'NONE',  ( 0.000000000000000000, -0.000000000000000000, -1.000000000000000000 ) ) ;
#49245=DIRECTION ( 'NONE',  ( 0.000000000000000000, 0.000000000000000000, 1.000000000000000000 ) ) ;
#49246=ORIENTED_EDGE ( 'NONE', *, *, #19405, .F. ) ;
#49251=VERTEX_POINT ( 'NONE', #38442 ) ;
#49252=AXIS2_PLACEMENT_3D ( 'NONE', #675, #24577, #12494 ) ;
#49253=CARTESIAN_POINT ( 'NONE',  ( 75.02564229359539638, -189.7472609257535510, -19.27620354518634826 ) ) ;
#49254=AXIS2_PLACEMENT_3D ( 'NONE', #40180, #47570, #51770 ) ;
#49255=CARTESIAN_POINT ( 'NONE',  ( -48.47912675150885065, -189.7472609257535510, 6.938893903907228378E-15 ) ) ;
#49257=VECTOR ( 'NONE', #32148, 1000.000000000000114 ) ;
#49258=VECTOR ( 'NONE', #30671, 1000.000000000000000 ) ;
#49259=CARTESIAN_POINT ( 'NONE',  ( -133.0671220150036334, -177.1207230881787780, -92.03190238880748097 ) ) ;
#49261=LINE ( 'NONE', #22436, #19037 ) ;
#49264=ORIENTED_EDGE ( 'NONE', *, *, #9939, .F. ) ;
#49265=CARTESIAN_POINT ( 'NONE',  ( -5.142695285147754980, -175.3837268820161057, -116.1806952091177578 ) ) ;
#49269=DIRECTION ( 'NONE',  ( -0.000000000000000000, 1.000000000000000000, -0.000000000000000000 ) ) ;
#49274=EDGE_CURVE ( 'NONE', #32293, #23451, #22935, .T. ) ;
#49277=AXIS2_PLACEMENT_3D ( 'NONE', #8515, #40566, #45068 ) ;
#49280=ORIENTED_EDGE ( 'NONE', *, *, #4258, .F. ) ;
#49281=DIRECTION ( 'NONE',  ( 0.000000000000000000, -1.000000000000000000, 0.000000000000000000 ) ) ;
#49283=AXIS2_PLACEMENT_3D ( 'NONE', #12924, #37363, #20827 ) ;
#49284=EDGE_CURVE ( 'NONE', #49743, #19374, #34244, .T. ) ;
#49285=FACE_OUTER_BOUND ( 'NONE', #32863, .T. ) ;
#49289=VERTEX_POINT ( 'NONE', #6902 ) ;
#49290=CARTESIAN_POINT ( 'NONE',  ( -171.7300019102062549, -183.6283474603465606, -20.83798868929510562 ) ) ;
#49292=VECTOR ( 'NONE', #27990, 1000.000000000000000 ) ;
#49293=ADVANCED_FACE ( 'NONE', ( #15307 ), #15066, .F. ) ;
#49295=VECTOR ( 'NONE', #24214, 1000.000000000000000 ) ;
#49297=DIRECTION ( 'NONE',  ( -0.000000000000000000, 1.000000000000000000, -0.000000000000000000 ) ) ;
#49299=AXIS2_PLACEMENT_3D ( 'NONE', #31617, #39253, #75 ) ;
#49300=AXIS2_PLACEMENT_3D ( 'NONE', #32551, #16015, #39635 ) ;
#49301=EDGE_LOOP ( 'NONE', ( #20103, #2114, #31312, #31825 ) ) ;
#49302=DIRECTION ( 'NONE',  ( 0.000000000000000000, 1.000000000000000000, 0.000000000000000000 ) ) ;
#49307=CARTESIAN_POINT ( 'NONE',  ( -25.72842157752850056, -193.5000000000000000, 121.8950816227734606 ) ) ;
#49308=DIRECTION ( 'NONE',  ( -0.000000000000000000, -1.000000000000000000, 0.000000000000000000 ) ) ;
#49309=CARTESIAN_POINT ( 'NONE',  ( -100.6109117578263152, -177.1207230881787780, 112.5098962032393359 ) ) ;
#49310=CARTESIAN_POINT ( 'NONE',  ( -155.9608607592036833, -193.5000000000000000, 63.81752780153064464 ) ) ;
#49311=ORIENTED_EDGE ( 'NONE', *, *, #35155, .T. ) ;
#49312=DIRECTION ( 'NONE',  ( -0.6528221181905119463, 0.000000000000000000, -0.7575112421616284619 ) ) ;
#49314=ORIENTED_EDGE ( 'NONE', *, *, #4364, .F. ) ;
#49318=DIRECTION ( 'NONE',  ( -0.9890401873221654760, 0.000000000000000000, 0.1476465640024710868 ) ) ;
#49319=VERTEX_POINT ( 'NONE', #38171 ) ;
#49320=AXIS2_PLACEMENT_3D ( 'NONE', #44425, #8413, #29412 ) ;
#49321=CARTESIAN_POINT ( 'NONE',  ( -88.78924379339703421, -183.6283474603465606, -118.3219948448692804 ) ) ;
#49322=DIRECTION ( 'NONE',  ( 0.000000000000000000, 0.000000000000000000, -1.000000000000000000 ) ) ;
#49324=DIRECTION ( 'NONE',  ( -0.1768902751225733261, 0.000000000000000000, 0.9842305779475966077 ) ) ;
#49328=EDGE_LOOP ( 'NONE', ( #37860, #34665, #17728, #4826 ) ) ;
#49329=CIRCLE ( 'NONE', #30033, 125.0000000000000000 ) ;
#49330=CIRCLE ( 'NONE', #29168, 125.0000000000000000 ) ;
#49331=CARTESIAN_POINT ( 'NONE',  ( -98.31070548515593543, -189.7472609257535510, -113.5465278748093567 ) ) ;
#49332=ORIENTED_EDGE ( 'NONE', *, *, #16342, .F. ) ;
#49333=AXIS2_PLACEMENT_3D ( 'NONE', #37199, #13020, #29046 ) ;
#49334=LINE ( 'NONE', #26876, #31978 ) ;
#49335=EDGE_CURVE ( 'NONE', #20197, #42260, #2954, .T. ) ;
#49337=ADVANCED_FACE ( 'NONE', ( #47368 ), #18992, .T. ) ;
#49338=CARTESIAN_POINT ( 'NONE',  ( -18.95304271317703382, -175.3837268820161057, -121.4627941443854837 ) ) ;
#49339=CIRCLE ( 'NONE', #6424, 125.0000000000000000 ) ;
#49340=VERTEX_POINT ( 'NONE', #22677 ) ;
#49341=VECTOR ( 'NONE', #45479, 1000.000000000000000 ) ;
#49342=DIRECTION ( 'NONE',  ( 0.1768902751225666370, 0.000000000000000000, 0.9842305779475979399 ) ) ;
#49343=FACE_BOUND ( 'NONE', #3621, .T. ) ;
#49344=CARTESIAN_POINT ( 'NONE',  ( 69.88207517204678254, -175.3837268820161057, 40.19484891390058579 ) ) ;
#49348=ORIENTED_EDGE ( 'NONE', *, *, #12317, .F. ) ;
#49349=VERTEX_POINT ( 'NONE', #47112 ) ;
#49351=ORIENTED_EDGE ( 'NONE', *, *, #15645, .T. ) ;
#49353=AXIS2_PLACEMENT_3D ( 'NONE', #29043, #33260, #17514 ) ;
#49355=VECTOR ( 'NONE', #1194, 1000.000000000000000 ) ;
#49361=VECTOR ( 'NONE', #2724, 1000.000000000000000 ) ;
#49364=CARTESIAN_POINT ( 'NONE',  ( 26.62880456707186028, -193.5000000000000000, 98.66508442481510599 ) ) ;
#49365=VERTEX_POINT ( 'NONE', #38689 ) ;
#49367=LINE ( 'NONE', #45419, #21447 ) ;
#49370=ORIENTED_EDGE ( 'NONE', *, *, #24652, .F. ) ;
#49371=ORIENTED_EDGE ( 'NONE', *, *, #51070, .F. ) ;
#49372=DIRECTION ( 'NONE',  ( 0.000000000000000000, 1.000000000000000000, -0.000000000000000000 ) ) ;
#49373=EDGE_LOOP ( 'NONE', ( #10764, #17189, #37728, #22322 ) ) ;
#49375=LINE ( 'NONE', #21249, #14971 ) ;
#49381=FACE_OUTER_BOUND ( 'NONE', #24275, .T. ) ;
#49386=CARTESIAN_POINT ( 'NONE',  ( -27.36201831380533989, -193.5000000000000000, -122.1886788576022411 ) ) ;
#49387=DIRECTION ( 'NONE',  ( 0.000000000000000000, -1.000000000000000000, 0.000000000000000000 ) ) ;
#49389=CARTESIAN_POINT ( 'NONE',  ( 64.44365795514079309, -193.5000000000000000, -53.60452120946194299 ) ) ;
#49390=CARTESIAN_POINT ( 'NONE',  ( 58.48829670243886625, -177.1207230881787780, -64.67588669375805921 ) ) ;
#49392=CARTESIAN_POINT ( 'NONE',  ( -213.8817838414232426, -193.5000000000000000, 2.819679052520814125E-14 ) ) ;
#49393=LINE ( 'NONE', #5776, #13159 ) ;
#49394=VERTEX_POINT ( 'NONE', #43154 ) ;
#49395=AXIS2_PLACEMENT_3D ( 'NONE', #32925, #44774, #13750 ) ;
#49399=AXIS2_PLACEMENT_3D ( 'NONE', #30014, #17685, #24768 ) ;
#49400=EDGE_CURVE ( 'NONE', #14548, #43146, #7434, .T. ) ;
#49402=CARTESIAN_POINT ( 'NONE',  ( 75.48825557695654709, -175.3837268820161057, 2.844930291601486694 ) ) ;
#49403=EDGE_CURVE ( 'NONE', #39091, #11866, #46864, .T. ) ;
#49407=EDGE_LOOP ( 'NONE', ( #9648, #3135, #36943, #9608 ) ) ;
#49410=CIRCLE ( 'NONE', #25906, 125.0000000000000000 ) ;
#49411=FACE_OUTER_BOUND ( 'NONE', #9137, .T. ) ;
#49413=PLANE ( 'NONE',  #15297 ) ;
#49414=DIRECTION ( 'NONE',  ( -0.000000000000000000, 1.000000000000000000, -0.000000000000000000 ) ) ;
#49415=CARTESIAN_POINT ( 'NONE',  ( 30.67449672666758431, -177.1207230881787780, 95.45105364470144593 ) ) ;
#49419=EDGE_CURVE ( 'NONE', #12178, #11142, #7174, .T. ) ;
#49423=VECTOR ( 'NONE', #12829, 1000.000000000000000 ) ;
#49424=PLANE ( 'NONE',  #18935 ) ;
#49426=LINE ( 'NONE', #29417, #30070 ) ;
#49427=EDGE_CURVE ( 'NONE', #12206, #19921, #7922, .T. ) ;
#49428=ORIENTED_EDGE ( 'NONE', *, *, #13621, .F. ) ;
#49431=ORIENTED_EDGE ( 'NONE', *, *, #42039, .F. ) ;
#49437=DIRECTION ( 'NONE',  ( 0.1768902751225592818, 0.000000000000000000, 0.9842305779475992722 ) ) ;
#49441=CARTESIAN_POINT ( 'NONE',  ( 68.21542617880035664, -177.1207230881787780, 41.93543928473692262 ) ) ;
#49442=EDGE_LOOP ( 'NONE', ( #27330, #1826, #42914, #50345 ) ) ;
#49443=CARTESIAN_POINT ( 'NONE',  ( -48.47912675150885065, -177.1207230881787780, 6.938893903907228378E-15 ) ) ;
#49444=VECTOR ( 'NONE', #32594, 1000.000000000000000 ) ;
#49445=ORIENTED_EDGE ( 'NONE', *, *, #10349, .F. ) ;
#49446=CARTESIAN_POINT ( 'NONE',  ( 15.23368049493604381, -175.3837268820161057, -107.5438431188757420 ) ) ;
#49447=LINE ( 'NONE', #21579, #22441 ) ;
#49448=CARTESIAN_POINT ( 'NONE',  ( -47.51449116960048968, -193.5000000000000000, 0.2635871660690785045 ) ) ;
#49449=VERTEX_POINT ( 'NONE', #32627 ) ;
#49452=AXIS2_PLACEMENT_3D ( 'NONE', #41697, #42467, #22518 ) ;
#49453=DIRECTION ( 'NONE',  ( 0.000000000000000000, 0.000000000000000000, -1.000000000000000000 ) ) ;
#49455=CARTESIAN_POINT ( 'NONE',  ( -48.47912675150885065, -175.3837268820161057, 6.938893903907228378E-15 ) ) ;
#49456=EDGE_LOOP ( 'NONE', ( #24634, #30110, #45128, #40667 ) ) ;
#49457=CARTESIAN_POINT ( 'NONE',  ( 52.98246549829695340, -193.5000000000000000, 73.01058346660533971 ) ) ;
#49458=DIRECTION ( 'NONE',  ( 0.000000000000000000, 0.000000000000000000, -1.000000000000000000 ) ) ;
#49461=VERTEX_POINT ( 'NONE', #28667 ) ;
#49462=FACE_OUTER_BOUND ( 'NONE', #30964, .T. ) ;
#49463=DIRECTION ( 'NONE',  ( -0.2348860457809707758, 0.000000000000000000, -0.9720229140804138579 ) ) ;
#49464=CIRCLE ( 'NONE', #24229, 125.0000000000000000 ) ;
#49467=ORIENTED_EDGE ( 'NONE', *, *, #19209, .T. ) ;
#49468=CARTESIAN_POINT ( 'NONE',  ( 62.43652093785069468, -193.5000000000000000, 55.44293326708522329 ) ) ;
#49470=ADVANCED_FACE ( 'NONE', ( #43930 ), #44718, .T. ) ;
#49471=DIRECTION ( 'NONE',  ( 0.000000000000000000, -1.000000000000000000, 0.000000000000000000 ) ) ;
#49474=ADVANCED_FACE ( 'NONE', ( #43676 ), #23456, .T. ) ;
#49475=EDGE_CURVE ( 'NONE', #11500, #4839, #8447, .T. ) ;
#49476=FACE_OUTER_BOUND ( 'NONE', #36017, .T. ) ;
#49478=LINE ( 'NONE', #28680, #33711 ) ;
#49481=ORIENTED_EDGE ( 'NONE', *, *, #40919, .T. ) ;
#49482=AXIS2_PLACEMENT_3D ( 'NONE', #8039, #31694, #19866 ) ;
#49484=CARTESIAN_POINT ( 'NONE',  ( 1.150725574412418739, -175.3837268820161057, -114.7252272087845881 ) ) ;
#49485=EDGE_CURVE ( 'NONE', #16796, #48776, #24475, .T. ) ;
#49486=CARTESIAN_POINT ( 'NONE',  ( -84.19171550243319757, -193.5000000000000000, 119.7898618611247628 ) ) ;
#49491=ORIENTED_EDGE ( 'NONE', *, *, #36433, .T. ) ;
#49492=CARTESIAN_POINT ( 'NONE',  ( -47.87232660569025455, -177.1207230881787780, -0.7948544414133454916 ) ) ;
#49493=ADVANCED_FACE ( 'NONE', ( #45507 ), #32873, .T. ) ;
#49494=CARTESIAN_POINT ( 'NONE',  ( -48.47912675150885065, -173.5000000000000284, -14.99999999999999289 ) ) ;
#49495=DIRECTION ( 'NONE',  ( -0.9890401873221633666, 0.000000000000000000, -0.1476465640024850756 ) ) ;
#49496=EDGE_LOOP ( 'NONE', ( #6075, #6307, #41142, #11094 ) ) ;
#49497=EDGE_CURVE ( 'NONE', #17350, #7135, #11359, .T. ) ;
#49499=FACE_OUTER_BOUND ( 'NONE', #3808, .T. ) ;
#49500=PLANE ( 'NONE',  #50164 ) ;
#49503=VERTEX_POINT ( 'NONE', #9499 ) ;
#49504=DIRECTION ( 'NONE',  ( 0.000000000000000000, 1.000000000000000000, 0.000000000000000000 ) ) ;
#49505=EDGE_LOOP ( 'NONE', ( #13056, #34546, #6674, #35651 ) ) ;
#49506=DIRECTION ( 'NONE',  ( 0.7948544414133565938, 0.000000000000000000, -0.6068001458185890984 ) ) ;
#49507=DIRECTION ( 'NONE',  ( -0.6068001458185945385, 0.000000000000000000, 0.7948544414133523750 ) ) ;
#49508=CARTESIAN_POINT ( 'NONE',  ( -169.2746641285359317, -175.3837268820161057, -32.14713283941905786 ) ) ;
#49509=EDGE_CURVE ( 'NONE', #43537, #16076, #44991, .T. ) ;
#49513=DIRECTION ( 'NONE',  ( -0.000000000000000000, 1.000000000000000000, -0.000000000000000000 ) ) ;
#49514=VECTOR ( 'NONE', #15146, 1000.000000000000000 ) ;
#49515=VERTEX_POINT ( 'NONE', #21593 ) ;
#49516=CARTESIAN_POINT ( 'NONE',  ( 8.750818922897904528, -189.7472609257535510, -111.1293539894138434 ) ) ;
#49520=ORIENTED_EDGE ( 'NONE', *, *, #47213, .T. ) ;
#49521=DIRECTION ( 'NONE',  ( 0.1768902751225666370, 0.000000000000000000, 0.9842305779475979399 ) ) ;
#49522=EDGE_LOOP ( 'NONE', ( #48228, #8925, #27790, #36610 ) ) ;
#49523=CARTESIAN_POINT ( 'NONE',  ( -173.3294908491238004, -177.1207230881787780, -6.114457023560960991 ) ) ;
#49525=ORIENTED_EDGE ( 'NONE', *, *, #28306, .F. ) ;
#49526=PLANE ( 'NONE',  #34087 ) ;
#49528=CARTESIAN_POINT ( 'NONE',  ( -47.53180039765465636, -189.7472609257535510, -0.3202698538628280800 ) ) ;
#49530=EDGE_CURVE ( 'NONE', #46184, #42344, #41818, .T. ) ;
#49531=CARTESIAN_POINT ( 'NONE',  ( -48.13092511607445800, -175.3837268820161057, 0.9374196611341301111 ) ) ;
#49533=VERTEX_POINT ( 'NONE', #5046 ) ;
#49535=DIRECTION ( 'NONE',  ( -0.000000000000000000, -1.000000000000000000, 0.000000000000000000 ) ) ;
#49536=ORIENTED_EDGE ( 'NONE', *, *, #51246, .F. ) ;
#49537=ORIENTED_EDGE ( 'NONE', *, *, #44788, .T. ) ;
#49538=LINE ( 'NONE', #41890, #27704 ) ;
#49542=LINE ( 'NONE', #45078, #19818 ) ;
#49545=VECTOR ( 'NONE', #38131, 1000.000000000000114 ) ;
#49546=CARTESIAN_POINT ( 'NONE',  ( -48.47912675150885065, -183.6283474603465606, 6.938893903907228378E-15 ) ) ;
#49550=DIRECTION ( 'NONE',  ( 0.000000000000000000, 0.000000000000000000, -1.000000000000000000 ) ) ;
#49552=LINE ( 'NONE', #45606, #19871 ) ;
#49553=VERTEX_POINT ( 'NONE', #25785 ) ;
#49555=EDGE_CURVE ( 'NONE', #30281, #24385, #5568, .T. ) ;
#49557=CARTESIAN_POINT ( 'NONE',  ( -111.8989814360438828, -193.5000000000000000, -107.7168604805787027 ) ) ;
#49558=FACE_OUTER_BOUND ( 'NONE', #30636, .T. ) ;
#49559=FACE_OUTER_BOUND ( 'NONE', #15905, .T. ) ;
#49561=ORIENTED_EDGE ( 'NONE', *, *, #39098, .T. ) ;
#49564=ORIENTED_EDGE ( 'NONE', *, *, #1739, .T. ) ;
#49567=EDGE_LOOP ( 'NONE', ( #13984, #48830, #30939, #29867 ) ) ;
#49568=CARTESIAN_POINT ( 'NONE',  ( 74.00867759460086859, -193.5000000000000000, 24.93467037017222410 ) ) ;
#49569=CARTESIAN_POINT ( 'NONE',  ( -78.64590280292341617, -193.5000000000000000, -121.3052580173827408 ) ) ;
#49572=ORIENTED_EDGE ( 'NONE', *, *, #50354, .T. ) ;
#49573=CARTESIAN_POINT ( 'NONE',  ( -49.08592689732743963, -175.3837268820161057, -0.7948544414133539293 ) ) ;
#49575=EDGE_LOOP ( 'NONE', ( #40525, #12259, #36544, #30125 ) ) ;
#49577=VECTOR ( 'NONE', #48575, 1000.000000000000000 ) ;
#49578=DIRECTION ( 'NONE',  ( 0.000000000000000000, 0.000000000000000000, 1.000000000000000000 ) ) ;
#49580=DIRECTION ( 'NONE',  ( -0.000000000000000000, 1.000000000000000000, -0.000000000000000000 ) ) ;
#49581=CARTESIAN_POINT ( 'NONE',  ( -48.47912675150885065, -183.6283474603465606, 6.938893903907228378E-15 ) ) ;
#49582=DIRECTION ( 'NONE',  ( -0.7575112421616191360, 0.000000000000000000, -0.6528221181905227155 ) ) ;
#49585=CARTESIAN_POINT ( 'NONE',  ( -141.2664123866436512, -193.5000000000000000, -83.75869879877495805 ) ) ;
#49586=FACE_BOUND ( 'NONE', #45211, .T. ) ;
#49587=ORIENTED_EDGE ( 'NONE', *, *, #13571, .F. ) ;
#49590=CIRCLE ( 'NONE', #4259, 125.0000000000000000 ) ;
#49591=ORIENTED_EDGE ( 'NONE', *, *, #38587, .T. ) ;
#49595=CARTESIAN_POINT ( 'NONE',  ( -88.78924379339714790, -177.1207230881787780, -118.3219948448692520 ) ) ;
#49596=CARTESIAN_POINT ( 'NONE',  ( 50.27798938500056636, -193.5000000000000000, 74.98773087994526065 ) ) ;
#49599=ADVANCED_FACE ( 'NONE', ( #29984 ), #29714, .F. ) ;
#49600=DIRECTION ( 'NONE',  ( 0.000000000000000000, 1.000000000000000000, -0.000000000000000000 ) ) ;
#49601=ORIENTED_EDGE ( 'NONE', *, *, #51709, .T. ) ;
#49602=ORIENTED_EDGE ( 'NONE', *, *, #7626, .T. ) ;
#49604=DIRECTION ( 'NONE',  ( 0.000000000000000000, 0.000000000000000000, 1.000000000000000000 ) ) ;
#49608=CARTESIAN_POINT ( 'NONE',  ( 44.30815888362531041, -175.3837268820161057, 83.75869879877569701 ) ) ;
#49610=LINE ( 'NONE', #33316, #3692 ) ;
#49611=ORIENTED_EDGE ( 'NONE', *, *, #34784, .F. ) ;
#49613=CARTESIAN_POINT ( 'NONE',  ( -48.47912675150885065, -189.7472609257535510, 6.938893903907228378E-15 ) ) ;
#49615=DIRECTION ( 'NONE',  ( -0.8124868780056863082, 0.000000000000000000, 0.5829794791144649047 ) ) ;
#49617=VERTEX_POINT ( 'NONE', #25518 ) ;
#49624=FACE_OUTER_BOUND ( 'NONE', #32771, .T. ) ;
#49625=CARTESIAN_POINT ( 'NONE',  ( -147.6585554144535024, -177.1207230881787780, 76.08180419845385245 ) ) ;
#49626=EDGE_LOOP ( 'NONE', ( #37156, #24395, #19155, #49601 ) ) ;
#49628=ORIENTED_EDGE ( 'NONE', *, *, #19778, .T. ) ;
#49630=EDGE_CURVE ( 'NONE', #46556, #26931, #5511, .T. ) ;
#49631=ORIENTED_EDGE ( 'NONE', *, *, #12811, .F. ) ;
#49633=DIRECTION ( 'NONE',  ( -0.000000000000000000, 1.000000000000000000, -0.000000000000000000 ) ) ;
#49634=AXIS2_PLACEMENT_3D ( 'NONE', #45335, #37691, #1428 ) ;
#49636=ORIENTED_EDGE ( 'NONE', *, *, #37033, .T. ) ;
#49640=CARTESIAN_POINT ( 'NONE',  ( 38.01517884164427130, -193.5000000000000000, -88.85232316304831102 ) ) ;
#49642=EDGE_CURVE ( 'NONE', #38097, #30309, #4778, .T. ) ;
#49643=ORIENTED_EDGE ( 'NONE', *, *, #10893, .T. ) ;
#49645=CARTESIAN_POINT ( 'NONE',  ( -49.29161362951452929, -193.5000000000000000, -0.5829794791144748967 ) ) ;
#49647=CARTESIAN_POINT ( 'NONE',  ( -15.24927435600541692, -193.5000000000000000, 120.5021863277719234 ) ) ;
#49648=ORIENTED_EDGE ( 'NONE', *, *, #11188, .T. ) ;
#49649=EDGE_LOOP ( 'NONE', ( #51837, #2306, #23826, #34831 ) ) ;
#49650=EDGE_CURVE ( 'NONE', #34248, #41454, #45761, .T. ) ;
#49651=VECTOR ( 'NONE', #20838, 1000.000000000000000 ) ;
#49653=LINE ( 'NONE', #44927, #6010 ) ;
#49654=ORIENTED_EDGE ( 'NONE', *, *, #12765, .T. ) ;
#49657=DIRECTION ( 'NONE',  ( 0.000000000000000000, 1.000000000000000000, 0.000000000000000000 ) ) ;
#49658=CARTESIAN_POINT ( 'NONE',  ( -5.113431607746556473, -193.5000000000000000, 117.2365833888819537 ) ) ;
#49659=LINE ( 'NONE', #20486, #1898 ) ;
#49662=AXIS2_PLACEMENT_3D ( 'NONE', #18294, #41672, #37734 ) ;
#49664=VERTEX_POINT ( 'NONE', #16870 ) ;
#49665=AXIS2_PLACEMENT_3D ( 'NONE', #17918, #6349, #2649 ) ;
#49671=ORIENTED_EDGE ( 'NONE', *, *, #2309, .T. ) ;
#49673=DIRECTION ( 'NONE',  ( -0.1182731709213730997, 0.000000000000000000, 0.9929810960135161402 ) ) ;
#49678=EDGE_LOOP ( 'NONE', ( #19159, #22061, #20047, #13596 ) ) ;
#49680=DIRECTION ( 'NONE',  ( 0.1768902751225802927, 0.000000000000000000, -0.9842305779475953864 ) ) ;
#49681=ORIENTED_EDGE ( 'NONE', *, *, #43762, .F. ) ;
#49682=LINE ( 'NONE', #40736, #34773 ) ;
#49683=VERTEX_POINT ( 'NONE', #29454 ) ;
#49684=ADVANCED_FACE ( 'NONE', ( #2394 ), #43098, .T. ) ;
#49685=EDGE_CURVE ( 'NONE', #18737, #9440, #37368, .T. ) ;
#49686=CARTESIAN_POINT ( 'NONE',  ( -54.99637373343399815, -193.5000000000000000, 123.8286356280830915 ) ) ;
#49687=CARTESIAN_POINT ( 'NONE',  ( -43.48323084606168720, -177.1207230881787780, 124.9001241957026167 ) ) ;
#49688=DIRECTION ( 'NONE',  ( 0.000000000000000000, 0.000000000000000000, 1.000000000000000000 ) ) ;
#49689=ORIENTED_EDGE ( 'NONE', *, *, #23057, .F. ) ;
#49690=ORIENTED_EDGE ( 'NONE', *, *, #35606, .F. ) ;
#49691=CARTESIAN_POINT ( 'NONE',  ( -124.9871112439422092, -193.5000000000000000, -98.85104101073275729 ) ) ;
#49692=DIRECTION ( 'NONE',  ( 0.000000000000000000, -0.000000000000000000, -1.000000000000000000 ) ) ;
#49693=LINE ( 'NONE', #41528, #35750 ) ;
#49694=EDGE_LOOP ( 'NONE', ( #16886, #19391, #14739, #28308 ) ) ;
#49697=EDGE_CURVE ( 'NONE', #41328, #28153, #34441, .T. ) ;
#49699=CIRCLE ( 'NONE', #26152, 125.0000000000000000 ) ;
#49701=ORIENTED_EDGE ( 'NONE', *, *, #22029, .F. ) ;
#49702=EDGE_CURVE ( 'NONE', #32000, #9933, #42315, .T. ) ;
#49703=AXIS2_PLACEMENT_3D ( 'NONE', #39224, #11868, #35523 ) ;
#49704=CARTESIAN_POINT ( 'NONE',  ( 43.86477233319988756, -193.5000000000000000, -84.24728067915975771 ) ) ;
#49706=EDGE_CURVE ( 'NONE', #29948, #27304, #14735, .T. ) ;
#49707=VECTOR ( 'NONE', #38333, 1000.000000000000114 ) ;
#49708=CARTESIAN_POINT ( 'NONE',  ( 75.12566530717464275, -175.3837268820161057, 18.62405380494841367 ) ) ;
#49709=ORIENTED_EDGE ( 'NONE', *, *, #25655, .F. ) ;
#49710=ADVANCED_FACE ( 'NONE', ( #47056 ), #30245, .T. ) ;
#49711=CARTESIAN_POINT ( 'NONE',  ( 141.7825277784304205, -213.5000000000000000, -9.999999999999987566 ) ) ;
#49712=DIRECTION ( 'NONE',  ( 0.000000000000000000, -0.000000000000000000, 1.000000000000000000 ) ) ;
#49715=PLANE ( 'NONE',  #4824 ) ;
#49716=AXIS2_PLACEMENT_3D ( 'NONE', #36255, #48633, #35741 ) ;
#49717=DIRECTION ( 'NONE',  ( -0.000000000000000000, 1.000000000000000000, -0.000000000000000000 ) ) ;
#49720=DIRECTION ( 'NONE',  ( 0.000000000000000000, 0.000000000000000000, 1.000000000000000000 ) ) ;
#49721=CARTESIAN_POINT ( 'NONE',  ( -47.48307690889363641, -193.5000000000000000, -0.08879589532292464504 ) ) ;
#49722=DIRECTION ( 'NONE',  ( 0.000000000000000000, 1.000000000000000000, 0.000000000000000000 ) ) ;
#49723=ORIENTED_EDGE ( 'NONE', *, *, #12613, .F. ) ;
#49725=CARTESIAN_POINT ( 'NONE',  ( 1.150725574412418739, -193.5000000000000000, -114.7252272087845881 ) ) ;
#49727=DIRECTION ( 'NONE',  ( 0.000000000000000000, 0.000000000000000000, 1.000000000000000000 ) ) ;
#49730=VERTEX_POINT ( 'NONE', #35208 ) ;
#49731=ORIENTED_EDGE ( 'NONE', *, *, #41824, .F. ) ;
#49733=VECTOR ( 'NONE', #15961, 1000.000000000000000 ) ;
#49734=LINE ( 'NONE', #37896, #45450 ) ;
#49735=DIRECTION ( 'NONE',  ( -0.6068001458185945385, 0.000000000000000000, 0.7948544414133523750 ) ) ;
#49737=AXIS2_PLACEMENT_3D ( 'NONE', #15264, #39927, #39668 ) ;
#49738=EDGE_CURVE ( 'NONE', #17378, #16149, #34944, .T. ) ;
#49739=CARTESIAN_POINT ( 'NONE',  ( -37.08895481556041318, -193.5000000000000000, 124.4799742258550310 ) ) ;
#49740=CARTESIAN_POINT ( 'NONE',  ( -155.4465502054561057, -183.6283474603465606, 64.67588669375881238 ) ) ;
#49742=CARTESIAN_POINT ( 'NONE',  ( -48.64924157374596092, -189.7472609257535510, 124.9998842437354227 ) ) ;
#49743=VERTEX_POINT ( 'NONE', #30493 ) ;
#49749=EDGE_CURVE ( 'NONE', #138, #9404, #22624, .T. ) ;
#49751=CARTESIAN_POINT ( 'NONE',  ( -5.461633243180946451, -175.3837268820161057, 116.2991637277478247 ) ) ;
#49752=CARTESIAN_POINT ( 'NONE',  ( -162.9896759831412965, -183.6283474603465606, -50.12318939043964861 ) ) ;
#49753=AXIS2_PLACEMENT_3D ( 'NONE', #30440, #18381, #43055 ) ;
#49754=VECTOR ( 'NONE', #18531, 1000.000000000000000 ) ;
#49755=EDGE_CURVE ( 'NONE', #38638, #44868, #2184, .T. ) ;
#49759=CARTESIAN_POINT ( 'NONE',  ( -89.73513343757491612, -177.1207230881787780, -117.9955164924467397 ) ) ;
#49762=EDGE_CURVE ( 'NONE', #31150, #45018, #42065, .T. ) ;
#49763=LINE ( 'NONE', #18470, #24155 ) ;
#49764=VERTEX_POINT ( 'NONE', #14227 ) ;
#49765=LINE ( 'NONE', #28983, #36810 ) ;
#49766=ADVANCED_FACE ( 'NONE', ( #46290 ), #10271, .T. ) ;
#49769=VERTEX_POINT ( 'NONE', #35997 ) ;
#49770=DIRECTION ( 'NONE',  ( 0.6528221181905280446, 0.000000000000000000, -0.7575112421616145841 ) ) ;
#49772=DIRECTION ( 'NONE',  ( 0.000000000000000000, -1.000000000000000000, 0.000000000000000000 ) ) ;
#49773=EDGE_CURVE ( 'NONE', #8523, #6100, #41601, .T. ) ;
#49774=CARTESIAN_POINT ( 'NONE',  ( -14.28570516517293676, -193.5000000000000000, 120.2323164553486663 ) ) ;
#49775=CARTESIAN_POINT ( 'NONE',  ( 47.04848625005566731, -183.6283474603465606, 80.61932246194658092 ) ) ;
#49776=EDGE_LOOP ( 'NONE', ( #7067, #8070, #45309, #18138 ) ) ;
#49777=CIRCLE ( 'NONE', #26265, 124.9999999999999858 ) ;
#49778=EDGE_CURVE ( 'NONE', #33733, #602, #10547, .T. ) ;
#49780=CARTESIAN_POINT ( 'NONE',  ( -173.2765435274470178, -183.6283474603465606, -7.113702696401515979 ) ) ;
#49781=LINE ( 'NONE', #33987, #51751 ) ;
#49782=CARTESIAN_POINT ( 'NONE',  ( -166.2107720749849022, -175.3837268820161057, -38.92640747825594616 ) ) ;
#49783=EDGE_CURVE ( 'NONE', #672, #16398, #19964, .T. ) ;
#49784=VECTOR ( 'NONE', #18503, 1000.000000000000000 ) ;
#49785=EDGE_LOOP ( 'NONE', ( #2590, #806, #43151, #45953 ) ) ;
#49787=ORIENTED_EDGE ( 'NONE', *, *, #11052, .T. ) ;
#49789=CARTESIAN_POINT ( 'NONE',  ( -161.4019114581581391, -189.7472609257535510, 53.60452120946272458 ) ) ;
#49790=ORIENTED_EDGE ( 'NONE', *, *, #30675, .F. ) ;
#49791=EDGE_LOOP ( 'NONE', ( #100, #30774, #4290, #9978 ) ) ;
#49792=CIRCLE ( 'NONE', #27103, 125.0000000000000000 ) ;
#49793=VECTOR ( 'NONE', #30376, 1000.000000000000114 ) ;
#49795=EDGE_CURVE ( 'NONE', #24853, #20197, #16030, .T. ) ;
#49797=AXIS2_PLACEMENT_3D ( 'NONE', #40947, #20988, #41460 ) ;
#49803=AXIS2_PLACEMENT_3D ( 'NONE', #8590, #35942, #12790 ) ;
#49804=DIRECTION ( 'NONE',  ( 0.000000000000000000, 1.000000000000000000, 0.000000000000000000 ) ) ;
#49805=FACE_OUTER_BOUND ( 'NONE', #9695, .T. ) ;
#49806=ORIENTED_EDGE ( 'NONE', *, *, #30344, .T. ) ;
#49807=VERTEX_POINT ( 'NONE', #15786 ) ;
#49808=ORIENTED_EDGE ( 'NONE', *, *, #17319, .T. ) ;
#49815=ADVANCED_FACE ( 'NONE', ( #8137 ), #35458, .F. ) ;
#49817=VECTOR ( 'NONE', #37021, 1000.000000000000000 ) ;
#49818=EDGE_CURVE ( 'NONE', #24385, #26442, #39911, .T. ) ;
#49819=EDGE_CURVE ( 'NONE', #23438, #25658, #8038, .T. ) ;
#49820=ORIENTED_EDGE ( 'NONE', *, *, #47159, .T. ) ;
#49822=ORIENTED_EDGE ( 'NONE', *, *, #6453, .F. ) ;
#49823=ORIENTED_EDGE ( 'NONE', *, *, #8663, .T. ) ;
#49826=CARTESIAN_POINT ( 'NONE',  ( -48.47912675150885065, -183.6283474603465606, 6.938893903907228378E-15 ) ) ;
#49827=CARTESIAN_POINT ( 'NONE',  ( -129.9529520667707629, -189.7472609257535510, -94.79987230211960991 ) ) ;
#49829=CARTESIAN_POINT ( 'NONE',  ( 75.37518750349084939, -193.5000000000000000, 6.025661128238930964 ) ) ;
#49831=ORIENTED_EDGE ( 'NONE', *, *, #46210, .T. ) ;
#49833=CARTESIAN_POINT ( 'NONE',  ( -124.1938582159088327, -175.3837268820161057, -99.45993886622791536 ) ) ;
#49834=VECTOR ( 'NONE', #13094, 1000.000000000000000 ) ;
#49839=DIRECTION ( 'NONE',  ( -0.6528221181905227155, 0.000000000000000000, 0.7575112421616191360 ) ) ;
#49842=DIRECTION ( 'NONE',  ( 0.000000000000000000, 0.000000000000000000, 1.000000000000000000 ) ) ;
#49843=FACE_BOUND ( 'NONE', #4020, .T. ) ;
#49844=ORIENTED_EDGE ( 'NONE', *, *, #11521, .F. ) ;
#49845=LINE ( 'NONE', #1217, #49140 ) ;
#49848=EDGE_LOOP ( 'NONE', ( #19167, #37665, #44893, #5197 ) ) ;
#49849=CARTESIAN_POINT ( 'NONE',  ( 9.518239912201957864, -193.5000000000000000, -110.7307791902283043 ) ) ;
#49850=ORIENTED_EDGE ( 'NONE', *, *, #39475, .F. ) ;
#49852=PLANE ( 'NONE',  #30172 ) ;
#49855=ORIENTED_EDGE ( 'NONE', *, *, #17090, .T. ) ;
#49858=CARTESIAN_POINT ( 'NONE',  ( 69.99104047056319189, -189.7472609257535510, -39.87254040532513955 ) ) ;
#49859=ORIENTED_EDGE ( 'NONE', *, *, #22086, .F. ) ;
#49860=VERTEX_POINT ( 'NONE', #19691 ) ;
#49861=ORIENTED_EDGE ( 'NONE', *, *, #933, .T. ) ;
#49862=CARTESIAN_POINT ( 'NONE',  ( 60.90550954139435902, -175.3837268820161057, 60.49794494914085874 ) ) ;
#49864=CARTESIAN_POINT ( 'NONE',  ( -15.48416040178638831, -193.5000000000000000, 119.5301634136915112 ) ) ;
#49865=LINE ( 'NONE', #38549, #11878 ) ;
#49867=EDGE_LOOP ( 'NONE', ( #15934, #20348, #8770, #7482 ) ) ;
#49868=ADVANCED_FACE ( 'NONE', ( #20471 ), #20219, .F. ) ;
#49869=DIRECTION ( 'NONE',  ( 0.2635871660690581320, 0.000000000000000000, 0.9646355819083614058 ) ) ;
#49873=ORIENTED_EDGE ( 'NONE', *, *, #8415, .T. ) ;
#49874=ORIENTED_EDGE ( 'NONE', *, *, #47675, .T. ) ;
#49877=AXIS2_PLACEMENT_3D ( 'NONE', #5346, #33182, #17697 ) ;
#49879=AXIS2_PLACEMENT_3D ( 'NONE', #5239, #44651, #8899 ) ;
#49881=DIRECTION ( 'NONE',  ( -0.000000000000000000, 1.000000000000000000, -0.000000000000000000 ) ) ;
#49882=VERTEX_POINT ( 'NONE', #28356 ) ;
#49886=ORIENTED_EDGE ( 'NONE', *, *, #4016, .T. ) ;
#49887=CARTESIAN_POINT ( 'NONE',  ( -47.51449116960048968, -193.5000000000000000, 0.2635871660690785045 ) ) ;
#49889=EDGE_CURVE ( 'NONE', #37865, #22881, #492, .T. ) ;
#49890=CARTESIAN_POINT ( 'NONE',  ( 75.12566530717464275, -175.3837268820161057, 18.62405380494841367 ) ) ;
#49892=ORIENTED_EDGE ( 'NONE', *, *, #27305, .F. ) ;
#49893=CARTESIAN_POINT ( 'NONE',  ( -118.4380981977755880, -193.5000000000000000, -102.3804074221059892 ) ) ;
#49894=DIRECTION ( 'NONE',  ( 0.5085311186492094127, 0.000000000000000000, 0.8610436117673619938 ) ) ;
#49895=LINE ( 'NONE', #49389, #19601 ) ;
#49896=CARTESIAN_POINT ( 'NONE',  ( -168.8371699641976420, -193.5000000000000000, 33.74820638215509661 ) ) ;
#49897=EDGE_LOOP ( 'NONE', ( #50681, #50544, #36029, #16850 ) ) ;
#49898=CIRCLE ( 'NONE', #21343, 125.0000000000000000 ) ;
#49899=DIRECTION ( 'NONE',  ( 0.000000000000000000, 0.000000000000000000, -1.000000000000000000 ) ) ;
#49903=EDGE_CURVE ( 'NONE', #210, #48594, #23892, .T. ) ;
#49904=CARTESIAN_POINT ( 'NONE',  ( 76.52053249983504202, -177.1207230881787780, -0.2918682030015403162 ) ) ;
#49909=ADVANCED_FACE ( 'NONE', ( #39403 ), #31522, .T. ) ;
#49915=AXIS2_PLACEMENT_3D ( 'NONE', #51054, #50781, #31304 ) ;
#49918=DIRECTION ( 'NONE',  ( 0.000000000000000000, -1.000000000000000000, 0.000000000000000000 ) ) ;
#49919=ORIENTED_EDGE ( 'NONE', *, *, #46483, .F. ) ;
#49920=AXIS2_PLACEMENT_3D ( 'NONE', #21791, #4525, #2340 ) ;
#49922=EDGE_CURVE ( 'NONE', #7465, #48929, #34069, .T. ) ;
#49923=EDGE_LOOP ( 'NONE', ( #8325, #50812, #35920, #4653 ) ) ;
#49925=VERTEX_POINT ( 'NONE', #29654 ) ;
#49926=VECTOR ( 'NONE', #41193, 1000.000000000000000 ) ;
#49927=CARTESIAN_POINT ( 'NONE',  ( -142.9772358822569629, -193.5000000000000000, 81.82363577055969017 ) ) ;
#49928=ORIENTED_EDGE ( 'NONE', *, *, #38827, .F. ) ;
#49931=EDGE_CURVE ( 'NONE', #4823, #5747, #29393, .T. ) ;
#49932=PRODUCT ( 'Angle Mounting Base', 'Angle Mounting Base', '', ( #24673 ) ) ;
#49933=DIRECTION ( 'NONE',  ( 0.000000000000000000, 1.000000000000000000, -0.000000000000000000 ) ) ;
#49936=CYLINDRICAL_SURFACE ( 'NONE', #15759, 124.9999999999999858 ) ;
#49938=EDGE_CURVE ( 'NONE', #25927, #51078, #47512, .T. ) ;
#49939=PLANE ( 'NONE',  #13882 ) ;
#49940=ORIENTED_EDGE ( 'NONE', *, *, #42316, .F. ) ;
#49941=DIRECTION ( 'NONE',  ( 0.000000000000000000, -1.000000000000000000, 0.000000000000000000 ) ) ;
#49947=EDGE_LOOP ( 'NONE', ( #23620, #29377, #22431, #24200 ) ) ;
#49948=DIRECTION ( 'NONE',  ( 0.02963332782256331357, 0.000000000000000000, -0.9995608365087942371 ) ) ;
#49949=ORIENTED_EDGE ( 'NONE', *, *, #13884, .F. ) ;
#49952=CARTESIAN_POINT ( 'NONE',  ( 74.03660210627323579, -193.5000000000000000, -19.12855698118387693 ) ) ;
#49954=EDGE_CURVE ( 'NONE', #46176, #30683, #40687, .T. ) ;
#49955=DIRECTION ( 'NONE',  ( -0.000000000000000000, 1.000000000000000000, 0.000000000000000000 ) ) ;
#49958=VECTOR ( 'NONE', #27296, 1000.000000000000227 ) ;
#49959=CYLINDRICAL_SURFACE ( 'NONE', #16491, 124.9999999999999858 ) ;
#49960=AXIS2_PLACEMENT_3D ( 'NONE', #46100, #30300, #6405 ) ;
#49962=CARTESIAN_POINT ( 'NONE',  ( -213.8817838414232426, -213.5000000000000000, 2.819679052520814125E-14 ) ) ;
#49965=AXIS2_PLACEMENT_3D ( 'NONE', #36843, #1803, #834 ) ;
#49967=ORIENTED_EDGE ( 'NONE', *, *, #25012, .T. ) ;
#49970=AXIS2_PLACEMENT_3D ( 'NONE', #19109, #35126, #30398 ) ;
#49971=VECTOR ( 'NONE', #34769, 1000.000000000000000 ) ;
#49972=DIRECTION ( 'NONE',  ( 0.000000000000000000, 0.000000000000000000, -1.000000000000000000 ) ) ;
#49973=CARTESIAN_POINT ( 'NONE',  ( -135.6699833737243921, -189.7472609257535510, 89.56983042009322560 ) ) ;
#49974=AXIS2_PLACEMENT_3D ( 'NONE', #36533, #33401, #9219 ) ;
#49976=ADVANCED_FACE ( 'NONE', ( #13381 ), #9693, .T. ) ;
#49977=VECTOR ( 'NONE', #20505, 1000.000000000000114 ) ;
#49978=DIRECTION ( 'NONE',  ( 0.000000000000000000, -1.000000000000000000, 0.000000000000000000 ) ) ;
#49979=CARTESIAN_POINT ( 'NONE',  ( -173.4190745413846457, -193.5000000000000000, -3.874202661594927211 ) ) ;
#49984=EDGE_CURVE ( 'NONE', #47736, #30910, #32566, .T. ) ;
#49987=ORIENTED_EDGE ( 'NONE', *, *, #31788, .F. ) ;
#49989=VECTOR ( 'NONE', #51564, 1000.000000000000227 ) ;
#49991=CARTESIAN_POINT ( 'NONE',  ( -77.03256798524175508, -189.7472609257535510, 121.6951149130964893 ) ) ;
#49992=AXIS2_PLACEMENT_3D ( 'NONE', #47938, #40284, #3781 ) ;
#49996=LINE ( 'NONE', #26066, #48127 ) ;
#49997=ORIENTED_EDGE ( 'NONE', *, *, #49938, .T. ) ;
#49998=EDGE_CURVE ( 'NONE', #14667, #32936, #28611, .T. ) ;
#50000=CARTESIAN_POINT ( 'NONE',  ( 39.18328161278951427, -193.5000000000000000, 89.10837311819236106 ) ) ;
#50001=CARTESIAN_POINT ( 'NONE',  ( -49.46816693883101124, -193.5000000000000000, -0.1476465640024848536 ) ) ;
#50002=VERTEX_POINT ( 'NONE', #49128 ) ;
#50004=AXIS2_PLACEMENT_3D ( 'NONE', #12373, #36543, #24218 ) ;
#50005=VECTOR ( 'NONE', #36705, 1000.000000000000114 ) ;
#50006=DIRECTION ( 'NONE',  ( 0.8896570909947436601, 0.000000000000000000, 0.4566292373937200777 ) ) ;
#50008=DIRECTION ( 'NONE',  ( 0.000000000000000000, -0.000000000000000000, 1.000000000000000000 ) ) ;
#50009=ADVANCED_FACE ( 'NONE', ( #37287 ), #44658, .T. ) ;
#50010=VERTEX_POINT ( 'NONE', #12846 ) ;
#50011=DIRECTION ( 'NONE',  ( -0.000000000000000000, 1.000000000000000000, -0.000000000000000000 ) ) ;
#50013=DIRECTION ( 'NONE',  ( 0.000000000000000000, 0.000000000000000000, 1.000000000000000000 ) ) ;
#50014=DIRECTION ( 'NONE',  ( 0.05924062789370006937, 0.000000000000000000, 0.9982437317643222396 ) ) ;
#50016=EDGE_LOOP ( 'NONE', ( #28958, #22849, #19244, #23631 ) ) ;
#50017=ORIENTED_EDGE ( 'NONE', *, *, #15882, .T. ) ;
#50026=CARTESIAN_POINT ( 'NONE',  ( -48.47912675150885065, -193.5000000000000000, 125.0000000000000000 ) ) ;
#50028=AXIS2_PLACEMENT_3D ( 'NONE', #6542, #25979, #18364 ) ;
#50029=DIRECTION ( 'NONE',  ( -0.000000000000000000, 1.000000000000000000, -0.000000000000000000 ) ) ;
#50030=DIRECTION ( 'NONE',  ( -0.000000000000000000, 1.000000000000000000, -0.000000000000000000 ) ) ;
#50034=LINE ( 'NONE', #10337, #1715 ) ;
#50036=DIRECTION ( 'NONE',  ( -0.8124868780056825335, 0.000000000000000000, 0.5829794791144703447 ) ) ;
#50038=VERTEX_POINT ( 'NONE', #13114 ) ;
#50039=DIRECTION ( 'NONE',  ( -0.4031234292879665171, 0.000000000000000000, -0.9151456172430210145 ) ) ;
#50040=ORIENTED_EDGE ( 'NONE', *, *, #43287, .F. ) ;
#50041=AXIS2_PLACEMENT_3D ( 'NONE', #25126, #45871, #37195 ) ;
#50042=EDGE_CURVE ( 'NONE', #51627, #36158, #9438, .T. ) ;
#50043=CARTESIAN_POINT ( 'NONE',  ( 72.31641062551800303, -175.3837268820161057, 32.14713283941989630 ) ) ;
#50044=CARTESIAN_POINT ( 'NONE',  ( -52.47502265695601409, -177.1207230881787780, -123.9361149384469485 ) ) ;
#50045=EDGE_LOOP ( 'NONE', ( #27839, #10411, #31360, #13200 ) ) ;
#50046=VECTOR ( 'NONE', #6151, 1000.000000000000000 ) ;
#50048=ORIENTED_EDGE ( 'NONE', *, *, #33614, .F. ) ;
#50049=EDGE_CURVE ( 'NONE', #42459, #29743, #31545, .T. ) ;
#50050=EDGE_CURVE ( 'NONE', #6177, #50890, #29864, .T. ) ;
#50052=EDGE_CURVE ( 'NONE', #12141, #21231, #20639, .T. ) ;
#50056=CARTESIAN_POINT ( 'NONE',  ( 76.51419089073348800, -193.5000000000000000, -1.292495564988658030 ) ) ;
#50058=ORIENTED_EDGE ( 'NONE', *, *, #30137, .F. ) ;
#50060=PLANE ( 'NONE',  #12383 ) ;
#50061=ADVANCED_FACE ( 'NONE', ( #42254 ), #22034, .T. ) ;
#50062=LINE ( 'NONE', #33511, #16033 ) ;
#50064=ORIENTED_EDGE ( 'NONE', *, *, #42711, .F. ) ;
#50065=VERTEX_POINT ( 'NONE', #26484 ) ;
#50066=ADVANCED_FACE ( 'NONE', ( #50675 ), #6791, .T. ) ;
#50067=ORIENTED_EDGE ( 'NONE', *, *, #12765, .F. ) ;
#50068=CARTESIAN_POINT ( 'NONE',  ( -48.47912675150885065, -183.6283474603465606, 6.938893903907228378E-15 ) ) ;
#50070=VECTOR ( 'NONE', #31977, 1000.000000000000227 ) ;
#50071=VECTOR ( 'NONE', #2827, 1000.000000000000114 ) ;
#50074=PLANE ( 'NONE',  #2054 ) ;
#50076=VECTOR ( 'NONE', #34093, 1000.000000000000000 ) ;
#50078=ADVANCED_FACE ( 'NONE', ( #1799 ), #30681, .T. ) ;
#50079=ORIENTED_EDGE ( 'NONE', *, *, #24481, .F. ) ;
#50080=CARTESIAN_POINT ( 'NONE',  ( 75.12566530717464275, -189.7472609257535510, 18.62405380494842433 ) ) ;
#50081=EDGE_LOOP ( 'NONE', ( #17223, #31904, #45481, #28172 ) ) ;
#50083=DIRECTION ( 'NONE',  ( 0.000000000000000000, 0.000000000000000000, 1.000000000000000000 ) ) ;
#50084=VECTOR ( 'NONE', #47966, 1000.000000000000000 ) ;
#50086=CIRCLE ( 'NONE', #4754, 125.0000000000000000 ) ;
#50087=VECTOR ( 'NONE', #7036, 1000.000000000000000 ) ;
#50088=CARTESIAN_POINT ( 'NONE',  ( 75.95066919219054569, -193.5000000000000000, -11.92584929509534852 ) ) ;
#50089=PLANE ( 'NONE',  #31011 ) ;
#50090=ORIENTED_EDGE ( 'NONE', *, *, #33005, .F. ) ;
#50092=AXIS2_PLACEMENT_3D ( 'NONE', #39809, #40326, #43767 ) ;
#50093=EDGE_LOOP ( 'NONE', ( #48231, #31168, #24431, #36612 ) ) ;
#50095=VECTOR ( 'NONE', #12167, 1000.000000000000000 ) ;
#50096=ORIENTED_EDGE ( 'NONE', *, *, #14101, .F. ) ;
#50097=CARTESIAN_POINT ( 'NONE',  ( -55.71438232577009586, -193.5000000000000000, -124.7904286264580804 ) ) ;
#50100=DIRECTION ( 'NONE',  ( 0.000000000000000000, -0.000000000000000000, -1.000000000000000000 ) ) ;
#50105=ADVANCED_FACE ( 'NONE', ( #2581 ), #14419, .T. ) ;
#50107=CIRCLE ( 'NONE', #27420, 125.0000000000000000 ) ;
#50109=CARTESIAN_POINT ( 'NONE',  ( -168.1141659785444915, -177.1207230881787780, -36.22785377503943494 ) ) ;
#50110=VERTEX_POINT ( 'NONE', #18613 ) ;
#50111=AXIS2_PLACEMENT_3D ( 'NONE', #4114, #20129, #15945 ) ;
#50113=EDGE_LOOP ( 'NONE', ( #29446, #24043, #43570, #13807 ) ) ;
#50115=LINE ( 'NONE', #17542, #43928 ) ;
#50116=ORIENTED_EDGE ( 'NONE', *, *, #45011, .T. ) ;
#50117=EDGE_CURVE ( 'NONE', #49394, #48961, #38317, .T. ) ;
#50118=DIRECTION ( 'NONE',  ( 0.9266896074318343723, 0.000000000000000000, -0.3758275821142357809 ) ) ;
#50119=AXIS2_PLACEMENT_3D ( 'NONE', #36400, #396, #16450 ) ;
#50121=AXIS2_PLACEMENT_3D ( 'NONE', #52039, #16025, #3507 ) ;
#50124=DIRECTION ( 'NONE',  ( 0.000000000000000000, 0.000000000000000000, 1.000000000000000000 ) ) ;
#50125=VECTOR ( 'NONE', #4294, 1000.000000000000000 ) ;
#50126=CIRCLE ( 'NONE', #27442, 125.0000000000000000 ) ;
#50127=CIRCLE ( 'NONE', #37553, 125.0000000000000000 ) ;
#50130=ORIENTED_EDGE ( 'NONE', *, *, #1230, .T. ) ;
#50131=ORIENTED_EDGE ( 'NONE', *, *, #41907, .T. ) ;
#50132=ORIENTED_EDGE ( 'NONE', *, *, #4710, .F. ) ;
#50133=CIRCLE ( 'NONE', #9835, 125.0000000000000000 ) ;
#50135=DIRECTION ( 'NONE',  ( -0.9266896074318370369, 0.000000000000000000, 0.3758275821142292306 ) ) ;
#50137=DIRECTION ( 'NONE',  ( 0.000000000000000000, 0.000000000000000000, 1.000000000000000000 ) ) ;
#50138=FACE_OUTER_BOUND ( 'NONE', #49456, .T. ) ;
#50139=CARTESIAN_POINT ( 'NONE',  ( 49.10711742958949344, -189.7472609257535510, 78.11481899503480975 ) ) ;
#50140=EDGE_LOOP ( 'NONE', ( #42043, #1123, #49874, #41148 ) ) ;
#50141=ADVANCED_FACE ( 'NONE', ( #14946 ), #30952, .F. ) ;
#50142=EDGE_CURVE ( 'NONE', #30515, #46184, #9768, .T. ) ;
#50147=VECTOR ( 'NONE', #50398, 1000.000000000000000 ) ;
#50155=CARTESIAN_POINT ( 'NONE',  ( 26.70958190211001337, -175.3837268820161057, -99.85818990449013199 ) ) ;
#50157=VERTEX_POINT ( 'NONE', #35400 ) ;
#50159=ORIENTED_EDGE ( 'NONE', *, *, #21164, .T. ) ;
#50160=ORIENTED_EDGE ( 'NONE', *, *, #44431, .T. ) ;
#50164=AXIS2_PLACEMENT_3D ( 'NONE', #37902, #26070, #9531 ) ;
#50166=CARTESIAN_POINT ( 'NONE',  ( -170.8336150310145172, -189.7472609257535510, 25.58083653558488280 ) ) ;
#50168=CIRCLE ( 'NONE', #28302, 125.0000000000000000 ) ;
#50169=FACE_OUTER_BOUND ( 'NONE', #13177, .T. ) ;
#50170=DIRECTION ( 'NONE',  ( 1.000000000000000000, 0.000000000000000000, 0.000000000000000000 ) ) ;
#50171=LINE ( 'NONE', #49640, #7853 ) ;
#50172=LINE ( 'NONE', #9959, #5236 ) ;
#50173=VERTEX_POINT ( 'NONE', #43296 ) ;
#50175=DIRECTION ( 'NONE',  ( 0.000000000000000000, 0.000000000000000000, 1.000000000000000000 ) ) ;
#50176=VECTOR ( 'NONE', #31041, 1000.000000000000000 ) ;
#50177=DIRECTION ( 'NONE',  ( -0.000000000000000000, 1.000000000000000000, 0.000000000000000000 ) ) ;
#50178=VERTEX_POINT ( 'NONE', #43806 ) ;
#50179=CARTESIAN_POINT ( 'NONE',  ( -171.1451123608488274, -193.5000000000000000, 18.13990644964089682 ) ) ;
#50180=CARTESIAN_POINT ( 'NONE',  ( -48.47912675150885065, -189.7472609257535510, 6.938893903907228378E-15 ) ) ;
#50183=EDGE_CURVE ( 'NONE', #16275, #16384, #35663, .T. ) ;
#50188=FACE_OUTER_BOUND ( 'NONE', #40835, .T. ) ;
#50190=PLANE ( 'NONE',  #33749 ) ;
#50191=CARTESIAN_POINT ( 'NONE',  ( -32.98951909085346301, -189.7472609257535510, 123.0287672223653033 ) ) ;
#50193=CARTESIAN_POINT ( 'NONE',  ( -171.9838957966129556, -189.7472609257535510, 19.27620354518722579 ) ) ;
#50194=CARTESIAN_POINT ( 'NONE',  ( -112.1919339979530150, -175.3837268820161057, 107.5438431188761825 ) ) ;
#50197=VERTEX_POINT ( 'NONE', #8337 ) ;
#50198=CARTESIAN_POINT ( 'NONE',  ( -116.2964108826154330, -183.6283474603465606, -105.0038855142073260 ) ) ;
#50199=CIRCLE ( 'NONE', #42597, 125.0000000000000000 ) ;
#50200=ORIENTED_EDGE ( 'NONE', *, *, #39133, .T. ) ;
#50201=ADVANCED_FACE ( 'NONE', ( #19638 ), #51985, .T. ) ;
#50202=LINE ( 'NONE', #42279, #28429 ) ;
#50203=EDGE_CURVE ( 'NONE', #14153, #27547, #41639, .T. ) ;
#50205=CARTESIAN_POINT ( 'NONE',  ( -40.90423906728908321, -175.3837268820161057, -124.7702732086912221 ) ) ;
#50206=EDGE_LOOP ( 'NONE', ( #36411, #50238, #19083, #18808 ) ) ;
#50208=LINE ( 'NONE', #13670, #33970 ) ;
#50209=VERTEX_POINT ( 'NONE', #12261 ) ;
#50211=VERTEX_POINT ( 'NONE', #23340 ) ;
#50213=ORIENTED_EDGE ( 'NONE', *, *, #42687, .T. ) ;
#50214=CARTESIAN_POINT ( 'NONE',  ( -48.47912675150885065, -175.3837268820161057, 6.938893903907228378E-15 ) ) ;
#50215=DIRECTION ( 'NONE',  ( 0.9473263538541923934, 0.000000000000000000, -0.3202698538628350744 ) ) ;
#50219=CARTESIAN_POINT ( 'NONE',  ( 75.01583293582056911, -189.7472609257535510, 11.18012358327988665 ) ) ;
#50221=EDGE_LOOP ( 'NONE', ( #28445, #17477, #39162, #26736 ) ) ;
#50223=CIRCLE ( 'NONE', #14130, 125.0000000000000000 ) ;
#50225=ORIENTED_EDGE ( 'NONE', *, *, #3488, .F. ) ;
#50227=LINE ( 'NONE', #47049, #26384 ) ;
#50229=CARTESIAN_POINT ( 'NONE',  ( -104.8182102393454045, -189.7472609257535510, 111.5836353223472912 ) ) ;
#50230=CARTESIAN_POINT ( 'NONE',  ( -47.87232660569025455, -193.5000000000000000, -0.7948544414133454916 ) ) ;
#50232=DIRECTION ( 'NONE',  ( 0.000000000000000000, -1.000000000000000000, -0.000000000000000000 ) ) ;
#50233=ORIENTED_EDGE ( 'NONE', *, *, #13093, .F. ) ;
#50235=DIRECTION ( 'NONE',  ( 0.000000000000000000, 0.000000000000000000, -1.000000000000000000 ) ) ;
#50236=EDGE_CURVE ( 'NONE', #44743, #29510, #27257, .T. ) ;
#50237=DIRECTION ( 'NONE',  ( 0.000000000000000000, 1.000000000000000000, 0.000000000000000000 ) ) ;
#50238=ORIENTED_EDGE ( 'NONE', *, *, #35248, .F. ) ;
#50242=LINE ( 'NONE', #33673, #38387 ) ;
#50245=VECTOR ( 'NONE', #48061, 1000.000000000000114 ) ;
#50246=EDGE_CURVE ( 'NONE', #37933, #25927, #15193, .T. ) ;
#50247=DIRECTION ( 'NONE',  ( 0.000000000000000000, 0.000000000000000000, -1.000000000000000000 ) ) ;
#50248=CARTESIAN_POINT ( 'NONE',  ( 26.52087324849106054, -173.5000000000000284, -80.00000000000002842 ) ) ;
#50249=FACE_OUTER_BOUND ( 'NONE', #34713, .T. ) ;
#50250=VERTEX_POINT ( 'NONE', #174 ) ;
#50251=CARTESIAN_POINT ( 'NONE',  ( 7.403327498934737960, -193.5000000000000000, -110.6939782313521192 ) ) ;
#50252=CARTESIAN_POINT ( 'NONE',  ( -47.74129347246712740, -183.6283474603465606, -0.6749830015182022303 ) ) ;
#50253=DIRECTION ( 'NONE',  ( 0.9929810960135161402, 0.000000000000000000, 0.1182731709213730997 ) ) ;
#50256=ORIENTED_EDGE ( 'NONE', *, *, #43283, .F. ) ;
#50257=VECTOR ( 'NONE', #51230, 1000.000000000000000 ) ;
#50258=EDGE_LOOP ( 'NONE', ( #25391, #49987, #28146, #50318 ) ) ;
#50260=DIRECTION ( 'NONE',  ( -0.2348860457809775482, 0.000000000000000000, -0.9720229140804121926 ) ) ;
#50262=FACE_OUTER_BOUND ( 'NONE', #26278, .T. ) ;
#50263=CARTESIAN_POINT ( 'NONE',  ( -48.07600332222087758, -175.3837268820161057, -0.9151456172430111335 ) ) ;
#50265=LINE ( 'NONE', #15036, #14131 ) ;
#50267=CIRCLE ( 'NONE', #34309, 125.0000000000000000 ) ;
#50269=CARTESIAN_POINT ( 'NONE',  ( -47.48307690889363641, -177.1207230881787780, 0.08879589532294547560 ) ) ;
#50271=FACE_OUTER_BOUND ( 'NONE', #997, .T. ) ;
#50274=ORIENTED_EDGE ( 'NONE', *, *, #13453, .F. ) ;
#50276=CYLINDRICAL_SURFACE ( 'NONE', #33036, 125.0000000000000000 ) ;
#50278=AXIS2_PLACEMENT_3D ( 'NONE', #28528, #36952, #12758 ) ;
#50279=CARTESIAN_POINT ( 'NONE',  ( -135.4258661347518853, -175.3837268820161057, -89.80681772907010441 ) ) ;
#50281=CARTESIAN_POINT ( 'NONE',  ( 51.05451324771860300, -177.1207230881787780, 75.61781872352698031 ) ) ;
#50282=DIRECTION ( 'NONE',  ( -0.9995608365087946812, 0.000000000000000000, 0.02963332782254913048 ) ) ;
#50283=ORIENTED_EDGE ( 'NONE', *, *, #51209, .T. ) ;
#50286=EDGE_CURVE ( 'NONE', #15404, #23646, #28296, .T. ) ;
#50287=EDGE_LOOP ( 'NONE', ( #22751, #41464, #20841, #20625 ) ) ;
#50288=DIRECTION ( 'NONE',  ( -0.9960498426152177842, 0.000000000000000000, 0.08879589532292482545 ) ) ;
#50290=ORIENTED_EDGE ( 'NONE', *, *, #26239, .F. ) ;
#50293=CIRCLE ( 'NONE', #38534, 125.0000000000000000 ) ;
#50295=DIRECTION ( 'NONE',  ( 0.5586467658036476935, 0.000000000000000000, 0.8294056854502049880 ) ) ;
#50299=CARTESIAN_POINT ( 'NONE',  ( -124.3803110981236273, -189.7472609257535510, -98.05618656931940791 ) ) ;
#50300=LINE ( 'NONE', #45327, #8109 ) ;
#50301=ADVANCED_FACE ( 'NONE', ( #11229 ), #3093, .T. ) ;
#50302=EDGE_CURVE ( 'NONE', #49743, #24932, #20679, .T. ) ;
#50308=EDGE_CURVE ( 'NONE', #11814, #49251, #51456, .T. ) ;
#50311=CARTESIAN_POINT ( 'NONE',  ( -108.5723883981723930, -177.1207230881787780, 109.6074810615846360 ) ) ;
#50312=ORIENTED_EDGE ( 'NONE', *, *, #17620, .T. ) ;
#50316=VECTOR ( 'NONE', #30879, 1000.000000000000000 ) ;
#50317=DIRECTION ( 'NONE',  ( 0.9890401873221623674, 0.000000000000000000, 0.1476465640024917925 ) ) ;
#50318=ORIENTED_EDGE ( 'NONE', *, *, #12108, .T. ) ;
#50320=EDGE_LOOP ( 'NONE', ( #36794, #16838, #26830, #27558 ) ) ;
#50321=CARTESIAN_POINT ( 'NONE',  ( -173.3968853974275817, -175.3837268820161057, 4.533605064404221174 ) ) ;
#50322=DIRECTION ( 'NONE',  ( 0.000000000000000000, 0.000000000000000000, -1.000000000000000000 ) ) ;
#50323=DIRECTION ( 'NONE',  ( 0.000000000000000000, 0.000000000000000000, 1.000000000000000000 ) ) ;
#50324=DIRECTION ( 'NONE',  ( -0.6528221181905227155, 0.000000000000000000, 0.7575112421616191360 ) ) ;
#50325=ORIENTED_EDGE ( 'NONE', *, *, #12406, .F. ) ;
#50326=ORIENTED_EDGE ( 'NONE', *, *, #28899, .T. ) ;
#50328=CARTESIAN_POINT ( 'NONE',  ( 4.558749771216711544, -177.1207230881787780, -112.0852863853379233 ) ) ;
#50329=DIRECTION ( 'NONE',  ( 0.000000000000000000, 1.000000000000000000, -0.000000000000000000 ) ) ;
#50331=LINE ( 'NONE', #41911, #7730 ) ;
#50332=CARTESIAN_POINT ( 'NONE',  ( -48.47912675150885065, -189.7472609257535510, 6.938893903907228378E-15 ) ) ;
#50338=DIRECTION ( 'NONE',  ( 0.000000000000000000, 0.000000000000000000, 1.000000000000000000 ) ) ;
#50344=LINE ( 'NONE', #22491, #1621 ) ;
#50345=ORIENTED_EDGE ( 'NONE', *, *, #48112, .F. ) ;
#50346=DIRECTION ( 'NONE',  ( -0.000000000000000000, 1.000000000000000000, -0.000000000000000000 ) ) ;
#50349=CIRCLE ( 'NONE', #29353, 125.0000000000000000 ) ;
#50350=VERTEX_POINT ( 'NONE', #44590 ) ;
#50351=DIRECTION ( 'NONE',  ( -0.000000000000000000, 1.000000000000000000, -0.000000000000000000 ) ) ;
#50352=DIRECTION ( 'NONE',  ( 0.000000000000000000, -0.000000000000000000, -1.000000000000000000 ) ) ;
#50354=EDGE_CURVE ( 'NONE', #38913, #39413, #1357, .T. ) ;
#50356=LINE ( 'NONE', #22503, #30581 ) ;
#50357=DIRECTION ( 'NONE',  ( -0.9720229140804107493, 0.000000000000000000, -0.2348860457809842095 ) ) ;
#50359=LINE ( 'NONE', #18300, #12299 ) ;
#50361=CARTESIAN_POINT ( 'NONE',  ( -95.18697522258266019, -177.1207230881787780, 115.9455772817713353 ) ) ;
#50364=VECTOR ( 'NONE', #17359, 1000.000000000000000 ) ;
#50366=ORIENTED_EDGE ( 'NONE', *, *, #8035, .T. ) ;
#50367=EDGE_CURVE ( 'NONE', #20252, #5652, #25707, .T. ) ;
#50368=ORIENTED_EDGE ( 'NONE', *, *, #42309, .F. ) ;
#50372=CARTESIAN_POINT ( 'NONE',  ( -161.6832731452239784, -189.7472609257535510, -53.00774697410100345 ) ) ;
#50373=ORIENTED_EDGE ( 'NONE', *, *, #24198, .T. ) ;
#50374=FACE_OUTER_BOUND ( 'NONE', #287, .T. ) ;
#50375=CARTESIAN_POINT ( 'NONE',  ( -163.3872488209693472, -183.6283474603465606, -49.20491319441547517 ) ) ;
#50377=DIRECTION ( 'NONE',  ( 0.6068001458186002006, 0.000000000000000000, -0.7948544414133481562 ) ) ;
#50378=CARTESIAN_POINT ( 'NONE',  ( -157.8637630444124511, -189.7472609257535510, -60.49794494914015530 ) ) ;
#50379=DIRECTION ( 'NONE',  ( -0.9473263538541946138, 0.000000000000000000, 0.3202698538628279690 ) ) ;
#50380=EDGE_CURVE ( 'NONE', #37183, #29247, #1485, .T. ) ;
#50383=AXIS2_PLACEMENT_3D ( 'NONE', #24776, #40794, #37116 ) ;
#50384=VECTOR ( 'NONE', #40840, 1000.000000000000114 ) ;
#50385=ORIENTED_EDGE ( 'NONE', *, *, #39739, .F. ) ;
#50388=CARTESIAN_POINT ( 'NONE',  ( -45.12595152424214007, -183.6283474603465606, -123.9551692589637497 ) ) ;
#50389=DIRECTION ( 'NONE',  ( -0.000000000000000000, 1.000000000000000000, -0.000000000000000000 ) ) ;
#50390=ORIENTED_EDGE ( 'NONE', *, *, #18532, .T. ) ;
#50392=EDGE_CURVE ( 'NONE', #10684, #17102, #15662, .T. ) ;
#50394=CARTESIAN_POINT ( 'NONE',  ( 69.72248760683812918, -183.6283474603465606, -37.47770156625421833 ) ) ;
#50395=ORIENTED_EDGE ( 'NONE', *, *, #12712, .F. ) ;
#50396=ORIENTED_EDGE ( 'NONE', *, *, #34609, .T. ) ;
#50397=VECTOR ( 'NONE', #35418, 1000.000000000000000 ) ;
#50398=DIRECTION ( 'NONE',  ( 0.7378332790417285736, 0.000000000000000000, -0.6749830015182091136 ) ) ;
#50399=EDGE_LOOP ( 'NONE', ( #1885, #24381, #39074, #40197 ) ) ;
#50401=ORIENTED_EDGE ( 'NONE', *, *, #50236, .F. ) ;
#50403=EDGE_CURVE ( 'NONE', #31054, #5412, #14805, .T. ) ;
#50404=CARTESIAN_POINT ( 'NONE',  ( -126.3604277550461035, -177.1207230881787780, 96.49160960477098570 ) ) ;
#50406=ADVANCED_FACE ( 'NONE', ( #17005 ), #13314, .F. ) ;
#50407=CARTESIAN_POINT ( 'NONE',  ( -109.9568094315246327, -177.1207230881787780, -108.8370090194290611 ) ) ;
#50410=ORIENTED_EDGE ( 'NONE', *, *, #3326, .F. ) ;
#50411=ADVANCED_FACE ( 'NONE', ( #5181 ), #49059, .T. ) ;
#50412=VERTEX_POINT ( 'NONE', #9119 ) ;
#50415=EDGE_CURVE ( 'NONE', #10170, #13304, #4384, .T. ) ;
#50418=DIRECTION ( 'NONE',  ( 0.000000000000000000, 1.000000000000000000, 0.000000000000000000 ) ) ;
#50419=ORIENTED_EDGE ( 'NONE', *, *, #8806, .T. ) ;
#50420=DIRECTION ( 'NONE',  ( -0.000000000000000000, 1.000000000000000000, -0.000000000000000000 ) ) ;
#50421=CARTESIAN_POINT ( 'NONE',  ( -171.5708553757489767, -193.5000000000000000, 14.98512977653260414 ) ) ;
#50422=CARTESIAN_POINT ( 'NONE',  ( -48.47912675150885065, -183.6283474603465606, 6.938893903907228378E-15 ) ) ;
#50423=LINE ( 'NONE', #26746, #14496 ) ;
#50424=EDGE_CURVE ( 'NONE', #35744, #48832, #20410, .T. ) ;
#50425=ORIENTED_EDGE ( 'NONE', *, *, #44431, .F. ) ;
#50426=FACE_OUTER_BOUND ( 'NONE', #12432, .T. ) ;
#50427=DIRECTION ( 'NONE',  ( 0.000000000000000000, 0.000000000000000000, 1.000000000000000000 ) ) ;
#50428=AXIS2_PLACEMENT_3D ( 'NONE', #28904, #24716, #28384 ) ;
#50430=AXIS2_PLACEMENT_3D ( 'NONE', #31591, #3475, #19505 ) ;
#50432=VERTEX_POINT ( 'NONE', #29848 ) ;
#50433=EDGE_CURVE ( 'NONE', #16426, #42195, #10393, .T. ) ;
#50434=CARTESIAN_POINT ( 'NONE',  ( -81.47409310123215676, -193.5000000000000000, -119.5301634136912412 ) ) ;
#50435=CARTESIAN_POINT ( 'NONE',  ( -48.36085358058748795, -177.1207230881787780, 0.9929810960135245779 ) ) ;
#50437=VERTEX_POINT ( 'NONE', #42186 ) ;
#50438=CARTESIAN_POINT ( 'NONE',  ( -169.1033029113419559, -189.7472609257535510, 32.78426643622744052 ) ) ;
#50439=EDGE_LOOP ( 'NONE', ( #41630, #20981, #2555, #732 ) ) ;
#50441=LINE ( 'NONE', #21799, #12498 ) ;
#50442=AXIS2_PLACEMENT_3D ( 'NONE', #22463, #38480, #43185 ) ;
#50444=LINE ( 'NONE', #14960, #32959 ) ;
#50446=DIRECTION ( 'NONE',  ( 0.000000000000000000, 0.000000000000000000, 1.000000000000000000 ) ) ;
#50447=ORIENTED_EDGE ( 'NONE', *, *, #17297, .F. ) ;
#50448=CARTESIAN_POINT ( 'NONE',  ( -49.25565061422690150, -193.5000000000000000, 0.6300878435817109935 ) ) ;
#50449=EDGE_CURVE ( 'NONE', #28974, #36109, #1738, .T. ) ;
#50451=LINE ( 'NONE', #51476, #27549 ) ;
#50452=ORIENTED_EDGE ( 'NONE', *, *, #8869, .T. ) ;
#50453=CARTESIAN_POINT ( 'NONE',  ( 67.64905612629584652, -177.1207230881787780, -43.47841891815122750 ) ) ;
#50457=DIRECTION ( 'NONE',  ( 0.000000000000000000, -1.000000000000000000, 0.000000000000000000 ) ) ;
#50458=EDGE_LOOP ( 'NONE', ( #17272, #3214, #33307, #21784 ) ) ;
#50459=CARTESIAN_POINT ( 'NONE',  ( -48.47912675150885065, -189.7472609257535510, 6.938893903907228378E-15 ) ) ;
#50460=DIRECTION ( 'NONE',  ( 0.000000000000000000, 1.000000000000000000, 0.000000000000000000 ) ) ;
#50462=LINE ( 'NONE', #17877, #19750 ) ;
#50464=CARTESIAN_POINT ( 'NONE',  ( -49.47517659412407198, -189.7472609257535510, 0.08879589532293177823 ) ) ;
#50468=CARTESIAN_POINT ( 'NONE',  ( -152.8713435144644848, -177.1207230881787780, -68.75510947788595217 ) ) ;
#50470=FACE_OUTER_BOUND ( 'NONE', #34721, .T. ) ;
#50471=ORIENTED_EDGE ( 'NONE', *, *, #10777, .T. ) ;
#50472=EDGE_LOOP ( 'NONE', ( #20397, #10408, #43991, #20046 ) ) ;
#50473=DIRECTION ( 'NONE',  ( -0.000000000000000000, 1.000000000000000000, -0.000000000000000000 ) ) ;
#50476=DIRECTION ( 'NONE',  ( 0.000000000000000000, -0.000000000000000000, -1.000000000000000000 ) ) ;
#50477=AXIS2_PLACEMENT_3D ( 'NONE', #42867, #10552, #6363 ) ;
#50479=CARTESIAN_POINT ( 'NONE',  ( 71.73509643893275722, -193.5000000000000000, -30.40954281680804172 ) ) ;
#50480=DIRECTION ( 'NONE',  ( -0.000000000000000000, 1.000000000000000000, -0.000000000000000000 ) ) ;
#50483=PLANE ( 'NONE',  #36624 ) ;
#50484=ORIENTED_EDGE ( 'NONE', *, *, #36154, .T. ) ;
#50486=LINE ( 'NONE', #46289, #34669 ) ;
#50487=DIRECTION ( 'NONE',  ( -0.000000000000000000, -1.000000000000000000, 0.000000000000000000 ) ) ;
#50489=EDGE_LOOP ( 'NONE', ( #24442, #29091, #20163, #47217 ) ) ;
#50490=CARTESIAN_POINT ( 'NONE',  ( 75.51463005422468200, -177.1207230881787780, -1.322128892811231360 ) ) ;
#50492=ADVANCED_FACE ( 'NONE', ( #37990 ), #5952, .T. ) ;
#50494=FACE_OUTER_BOUND ( 'NONE', #30414, .T. ) ;
#50495=DIRECTION ( 'NONE',  ( 0.000000000000000000, 0.000000000000000000, 1.000000000000000000 ) ) ;
#50497=VECTOR ( 'NONE', #19630, 1000.000000000000114 ) ;
#50499=AXIS2_PLACEMENT_3D ( 'NONE', #12130, #39234, #43693 ) ;
#50500=DIRECTION ( 'NONE',  ( 0.000000000000000000, -1.000000000000000000, 0.000000000000000000 ) ) ;
#50501=CARTESIAN_POINT ( 'NONE',  ( 49.10711742958948633, -175.3837268820161057, 78.11481899503480975 ) ) ;
#50502=LINE ( 'NONE', #10285, #22873 ) ;
#50504=EDGE_LOOP ( 'NONE', ( #49491, #30992, #24681, #49808 ) ) ;
#50505=DIRECTION ( 'NONE',  ( 0.000000000000000000, 0.000000000000000000, 1.000000000000000000 ) ) ;
#50506=AXIS2_PLACEMENT_3D ( 'NONE', #44800, #24821, #8277 ) ;
#50507=DIRECTION ( 'NONE',  ( -0.3482016354344059095, 0.000000000000000000, 0.9374196611341183427 ) ) ;
#50509=ORIENTED_EDGE ( 'NONE', *, *, #31759, .F. ) ;
#50511=ORIENTED_EDGE ( 'NONE', *, *, #644, .T. ) ;
#50513=DIRECTION ( 'NONE',  ( -0.000000000000000000, 1.000000000000000000, 0.000000000000000000 ) ) ;
#50514=DIRECTION ( 'NONE',  ( 0.000000000000000000, 0.000000000000000000, -1.000000000000000000 ) ) ;
#50515=EDGE_LOOP ( 'NONE', ( #3520, #12, #1820, #30995 ) ) ;
#50517=CARTESIAN_POINT ( 'NONE',  ( 72.95485052494851175, -177.1207230881787780, -29.64437826672757481 ) ) ;
#50519=DIRECTION ( 'NONE',  ( 0.000000000000000000, -1.000000000000000000, 0.000000000000000000 ) ) ;
#50520=ORIENTED_EDGE ( 'NONE', *, *, #26750, .T. ) ;
#50521=DIRECTION ( 'NONE',  ( -0.000000000000000000, 1.000000000000000000, -0.000000000000000000 ) ) ;
#50522=ORIENTED_EDGE ( 'NONE', *, *, #9829, .T. ) ;
#50525=ORIENTED_EDGE ( 'NONE', *, *, #28177, .T. ) ;
#50528=CARTESIAN_POINT ( 'NONE',  ( 40.26790151320560085, -193.5000000000000000, -86.60307583628353711 ) ) ;
#50529=VECTOR ( 'NONE', #12966, 1000.000000000000114 ) ;
#50530=DIRECTION ( 'NONE',  ( 0.000000000000000000, 0.000000000000000000, -1.000000000000000000 ) ) ;
#50531=AXIS2_PLACEMENT_3D ( 'NONE', #26820, #6860, #30256 ) ;
#50533=CYLINDRICAL_SURFACE ( 'NONE', #47470, 125.0000000000000000 ) ;
#50535=ORIENTED_EDGE ( 'NONE', *, *, #31824, .F. ) ;
#50536=DIRECTION ( 'NONE',  ( -0.000000000000000000, 1.000000000000000000, -0.000000000000000000 ) ) ;
#50537=CARTESIAN_POINT ( 'NONE',  ( -47.50057025920934706, -193.5000000000000000, -0.2059786187410884151 ) ) ;
#50538=ORIENTED_EDGE ( 'NONE', *, *, #31519, .T. ) ;
#50540=AXIS2_PLACEMENT_3D ( 'NONE', #46886, #3737, #3247 ) ;
#50542=ORIENTED_EDGE ( 'NONE', *, *, #16216, .T. ) ;
#50543=CARTESIAN_POINT ( 'NONE',  ( 18.82962626094778003, -183.6283474603465606, 104.1428419024404377 ) ) ;
#50544=ORIENTED_EDGE ( 'NONE', *, *, #8351, .F. ) ;
#50545=AXIS2_PLACEMENT_3D ( 'NONE', #1018, #28609, #49126 ) ;
#50550=ORIENTED_EDGE ( 'NONE', *, *, #7554, .T. ) ;
#50552=DIRECTION ( 'NONE',  ( 0.000000000000000000, 0.000000000000000000, -1.000000000000000000 ) ) ;
#50553=DIRECTION ( 'NONE',  ( 0.000000000000000000, 0.000000000000000000, 1.000000000000000000 ) ) ;
#50555=CARTESIAN_POINT ( 'NONE',  ( 56.81546028627039391, -189.7472609257535510, 65.49088066501711580 ) ) ;
#50556=EDGE_LOOP ( 'NONE', ( #11279, #30624, #6007, #7212 ) ) ;
#50560=ORIENTED_EDGE ( 'NONE', *, *, #48145, .F. ) ;
#50563=AXIS2_PLACEMENT_3D ( 'NONE', #21072, #37096, #40772 ) ;
#50564=DIRECTION ( 'NONE',  ( 0.000000000000000000, 0.000000000000000000, -1.000000000000000000 ) ) ;
#50565=VERTEX_POINT ( 'NONE', #34058 ) ;
#50566=CARTESIAN_POINT ( 'NONE',  ( -173.4724443937511467, -183.6283474603465606, 1.292495564989519785 ) ) ;
#50568=LINE ( 'NONE', #6933, #8200 ) ;
#50569=DIRECTION ( 'NONE',  ( 0.000000000000000000, 0.000000000000000000, -1.000000000000000000 ) ) ;
#50570=EDGE_CURVE ( 'NONE', #35696, #43188, #3878, .T. ) ;
#50571=DIRECTION ( 'NONE',  ( 0.000000000000000000, 0.000000000000000000, -1.000000000000000000 ) ) ;
#50573=ORIENTED_EDGE ( 'NONE', *, *, #35633, .T. ) ;
#50575=VECTOR ( 'NONE', #12956, 1000.000000000000000 ) ;
#50578=DIRECTION ( 'NONE',  ( 0.000000000000000000, 0.000000000000000000, -1.000000000000000000 ) ) ;
#50579=DIRECTION ( 'NONE',  ( -0.000000000000000000, 1.000000000000000000, -0.000000000000000000 ) ) ;
#50580=VECTOR ( 'NONE', #44586, 1000.000000000000000 ) ;
#50581=CIRCLE ( 'NONE', #20361, 125.0000000000000000 ) ;
#50583=CARTESIAN_POINT ( 'NONE',  ( -48.47912675150885065, -189.7472609257535510, 6.938893903907228378E-15 ) ) ;
#50584=EDGE_LOOP ( 'NONE', ( #41983, #35006, #4893, #14103 ) ) ;
#50586=AXIS2_PLACEMENT_3D ( 'NONE', #1561, #25987, #42261 ) ;
#50589=EDGE_CURVE ( 'NONE', #43312, #28285, #50359, .T. ) ;
#50593=EDGE_CURVE ( 'NONE', #46272, #34416, #3296, .T. ) ;
#50595=DIRECTION ( 'NONE',  ( 0.000000000000000000, -0.000000000000000000, 1.000000000000000000 ) ) ;
#50598=DIRECTION ( 'NONE',  ( -0.000000000000000000, 1.000000000000000000, 0.000000000000000000 ) ) ;
#50599=ORIENTED_EDGE ( 'NONE', *, *, #30162, .T. ) ;
#50600=PLANE ( 'NONE',  #47739 ) ;
#50601=VECTOR ( 'NONE', #41232, 1000.000000000000000 ) ;
#50602=EDGE_LOOP ( 'NONE', ( #48750, #8604, #28499, #7796 ) ) ;
#50603=FACE_OUTER_BOUND ( 'NONE', #36524, .T. ) ;
#50606=ORIENTED_EDGE ( 'NONE', *, *, #42247, .T. ) ;
#50607=CARTESIAN_POINT ( 'NONE',  ( -143.3583119192899460, -183.6283474603465606, -81.38144888055207105 ) ) ;
#50609=DIRECTION ( 'NONE',  ( -0.000000000000000000, 1.000000000000000000, 0.000000000000000000 ) ) ;
#50610=CIRCLE ( 'NONE', #27929, 125.0000000000000000 ) ;
#50611=DIRECTION ( 'NONE',  ( 0.000000000000000000, 1.000000000000000000, 0.000000000000000000 ) ) ;
#50612=AXIS2_PLACEMENT_3D ( 'NONE', #31991, #8595, #47784 ) ;
#50613=DIRECTION ( 'NONE',  ( -0.000000000000000000, 1.000000000000000000, -0.000000000000000000 ) ) ;
#50614=EDGE_LOOP ( 'NONE', ( #30067, #23773, #31896, #35377 ) ) ;
#50615=AXIS2_PLACEMENT_3D ( 'NONE', #4265, #36314, #41038 ) ;
#50616=FACE_OUTER_BOUND ( 'NONE', #44007, .T. ) ;
#50618=ORIENTED_EDGE ( 'NONE', *, *, #36276, .F. ) ;
#50619=DIRECTION ( 'NONE',  ( -0.000000000000000000, -1.000000000000000000, 0.000000000000000000 ) ) ;
#50620=AXIS2_PLACEMENT_3D ( 'NONE', #34568, #50619, #7245 ) ;
#50622=CARTESIAN_POINT ( 'NONE',  ( -48.47912675150885065, -177.1207230881787780, 6.938893903907228378E-15 ) ) ;
#50623=ORIENTED_EDGE ( 'NONE', *, *, #27243, .F. ) ;
#50624=DIRECTION ( 'NONE',  ( -0.3202698538628350744, 0.000000000000000000, -0.9473263538541923934 ) ) ;
#50625=CARTESIAN_POINT ( 'NONE',  ( -170.9669310976187830, -189.7472609257535510, -24.93467037017130394 ) ) ;
#50626=EDGE_LOOP ( 'NONE', ( #22984, #39461, #8850, #13711 ) ) ;
#50630=EDGE_CURVE ( 'NONE', #8865, #48981, #19329, .T. ) ;
#50632=LINE ( 'NONE', #30382, #22356 ) ;
#50633=VERTEX_POINT ( 'NONE', #47187 ) ;
#50634=VERTEX_POINT ( 'NONE', #20094 ) ;
#50635=VECTOR ( 'NONE', #40516, 1000.000000000000000 ) ;
#50636=ORIENTED_EDGE ( 'NONE', *, *, #36507, .F. ) ;
#50637=CARTESIAN_POINT ( 'NONE',  ( 2.669657140899374337, -189.7472609257535510, 114.0561348912355868 ) ) ;
#50638=CARTESIAN_POINT ( 'NONE',  ( -49.46816693883101834, -177.1207230881787780, 0.1476465640024780257 ) ) ;
#50639=CARTESIAN_POINT ( 'NONE',  ( -144.0067397530739584, -183.6283474603465606, -80.61932246194587037 ) ) ;
#50641=CARTESIAN_POINT ( 'NONE',  ( -48.47912675150885065, -177.1207230881787780, 6.938893903907228378E-15 ) ) ;
#50642=ORIENTED_EDGE ( 'NONE', *, *, #3174, .F. ) ;
#50645=EDGE_CURVE ( 'NONE', #45117, #50764, #35863, .T. ) ;
#50647=EDGE_LOOP ( 'NONE', ( #9778, #21137, #18384, #22335 ) ) ;
#50648=CARTESIAN_POINT ( 'NONE',  ( -137.6740394605055542, -183.6283474603465606, -86.14171647324867820 ) ) ;
#50650=VECTOR ( 'NONE', #26202, 1000.000000000000000 ) ;
#50651=ORIENTED_EDGE ( 'NONE', *, *, #23988, .F. ) ;
#50652=ADVANCED_FACE ( 'NONE', ( #27712 ), #11164, .F. ) ;
#50653=CARTESIAN_POINT ( 'NONE',  ( -12.13476221271687905, -189.7472609257535510, 119.5996955107804780 ) ) ;
#50655=CARTESIAN_POINT ( 'NONE',  ( -108.6269575285486724, -183.6283474603465606, -108.4360005853207696 ) ) ;
#50657=CARTESIAN_POINT ( 'NONE',  ( -139.0630283577175987, -183.6283474603465606, -86.13684908212448477 ) ) ;
#50659=ORIENTED_EDGE ( 'NONE', *, *, #5440, .T. ) ;
#50660=DIRECTION ( 'NONE',  ( 0.000000000000000000, 0.000000000000000000, -1.000000000000000000 ) ) ;
#50662=ORIENTED_EDGE ( 'NONE', *, *, #33318, .T. ) ;
#50663=LINE ( 'NONE', #14658, #43005 ) ;
#50664=LINE ( 'NONE', #26212, #21396 ) ;
#50665=DIRECTION ( 'NONE',  ( 0.000000000000000000, 0.000000000000000000, -1.000000000000000000 ) ) ;
#50666=VERTEX_POINT ( 'NONE', #47710 ) ;
#50667=DIRECTION ( 'NONE',  ( 0.000000000000000000, -0.000000000000000000, -1.000000000000000000 ) ) ;
#50669=DIRECTION ( 'NONE',  ( -0.000000000000000000, 1.000000000000000000, -0.000000000000000000 ) ) ;
#50671=DIRECTION ( 'NONE',  ( -0.000000000000000000, 1.000000000000000000, -0.000000000000000000 ) ) ;
#50672=LINE ( 'NONE', #46471, #11095 ) ;
#50673=VERTEX_POINT ( 'NONE', #23005 ) ;
#50674=DIRECTION ( 'NONE',  ( -0.4300652022765183435, 0.000000000000000000, -0.9027978299657446470 ) ) ;
#50675=FACE_OUTER_BOUND ( 'NONE', #35409, .T. ) ;
#50677=FACE_BOUND ( 'NONE', #7031, .T. ) ;
#50678=VERTEX_POINT ( 'NONE', #19830 ) ;
#50679=DIRECTION ( 'NONE',  ( 0.000000000000000000, -1.000000000000000000, 0.000000000000000000 ) ) ;
#50680=CARTESIAN_POINT ( 'NONE',  ( -123.4791267515088435, -198.5000000000000000, 70.00000000000000000 ) ) ;
#50681=ORIENTED_EDGE ( 'NONE', *, *, #28488, .T. ) ;
#50682=LINE ( 'NONE', #43049, #38826 ) ;
#50683=AXIS2_PLACEMENT_3D ( 'NONE', #30270, #46317, #10301 ) ;
#50684=ORIENTED_EDGE ( 'NONE', *, *, #29374, .T. ) ;
#50685=EDGE_CURVE ( 'NONE', #30315, #13271, #15647, .T. ) ;
#50688=DIRECTION ( 'NONE',  ( -0.000000000000000000, 1.000000000000000000, -0.000000000000000000 ) ) ;
#50689=ADVANCED_FACE ( 'NONE', ( #51920 ), #35091, .T. ) ;
#50690=EDGE_CURVE ( 'NONE', #43082, #45236, #35590, .T. ) ;
#50692=EDGE_CURVE ( 'NONE', #29039, #5201, #23275, .T. ) ;
#50693=CARTESIAN_POINT ( 'NONE',  ( -47.53180039765466347, -177.1207230881787780, 0.3202698538628485636 ) ) ;
#50695=ADVANCED_FACE ( 'NONE', ( #39534 ), #47955, .T. ) ;
#50696=CARTESIAN_POINT ( 'NONE',  ( 17.44316424268010834, -177.1207230881787780, -105.0256126866231483 ) ) ;
#50698=PLANE ( 'NONE',  #51880 ) ;
#50699=ORIENTED_EDGE ( 'NONE', *, *, #24967, .T. ) ;
#50701=DIRECTION ( 'NONE',  ( 0.5586467658036535777, 0.000000000000000000, -0.8294056854502011022 ) ) ;
#50702=CIRCLE ( 'NONE', #43970, 125.0000000000000000 ) ;
#50703=VECTOR ( 'NONE', #26032, 1000.000000000000000 ) ;
#50704=ADVANCED_FACE ( 'NONE', ( #11688 ), #27973, .T. ) ;
#50705=VECTOR ( 'NONE', #51981, 999.9999999999998863 ) ;
#50706=EDGE_CURVE ( 'NONE', #49151, #25657, #26935, .T. ) ;
#50708=DIRECTION ( 'NONE',  ( -0.2348860457809911206, 0.000000000000000000, 0.9720229140804089729 ) ) ;
#50709=ORIENTED_EDGE ( 'NONE', *, *, #10244, .T. ) ;
#50711=DIRECTION ( 'NONE',  ( -0.1768902751225592818, 0.000000000000000000, -0.9842305779475992722 ) ) ;
#50712=ORIENTED_EDGE ( 'NONE', *, *, #30976, .F. ) ;
#50715=ORIENTED_EDGE ( 'NONE', *, *, #6550, .F. ) ;
#50718=ADVANCED_FACE ( 'NONE', ( #24298 ), #32178, .F. ) ;
#50719=CARTESIAN_POINT ( 'NONE',  ( -62.97606545226381058, -193.5000000000000000, -123.1496609813404177 ) ) ;
#50720=CARTESIAN_POINT ( 'NONE',  ( -134.2540868116286958, -175.3837268820161057, 89.54698061029652933 ) ) ;
#50721=CARTESIAN_POINT ( 'NONE',  ( 65.79610465833508215, -183.6283474603465606, -50.65739320401927870 ) ) ;
#50722=ORIENTED_EDGE ( 'NONE', *, *, #46858, .F. ) ;
#50723=AXIS2_PLACEMENT_3D ( 'NONE', #43004, #7010, #39048 ) ;
#50724=ORIENTED_EDGE ( 'NONE', *, *, #13149, .F. ) ;
#50725=EDGE_CURVE ( 'NONE', #32264, #49349, #50107, .T. ) ;
#50727=FACE_OUTER_BOUND ( 'NONE', #9010, .T. ) ;
#50729=DIRECTION ( 'NONE',  ( 0.000000000000000000, 0.000000000000000000, 1.000000000000000000 ) ) ;
#50731=ORIENTED_EDGE ( 'NONE', *, *, #12852, .T. ) ;
#50732=CARTESIAN_POINT ( 'NONE',  ( -155.9155026329808607, -183.6283474603465606, -61.91627321685029983 ) ) ;
#50733=DIRECTION ( 'NONE',  ( 0.000000000000000000, 0.000000000000000000, -1.000000000000000000 ) ) ;
#50734=CARTESIAN_POINT ( 'NONE',  ( 29.27398957514434130, -183.6283474603465606, -97.87467957287998388 ) ) ;
#50735=DIRECTION ( 'NONE',  ( 0.000000000000000000, 1.000000000000000000, 0.000000000000000000 ) ) ;
#50736=CARTESIAN_POINT ( 'NONE',  ( 76.48781641346532467, -193.5000000000000000, 2.874563619424060246 ) ) ;
#50737=ORIENTED_EDGE ( 'NONE', *, *, #47229, .T. ) ;
#50739=CYLINDRICAL_SURFACE ( 'NONE', #25458, 125.0000000000000000 ) ;
#50740=ADVANCED_FACE ( 'NONE', ( #41102 ), #44792, .T. ) ;
#50741=CARTESIAN_POINT ( 'NONE',  ( 33.75048693540708911, -193.5000000000000000, 94.14505102712816154 ) ) ;
#50743=ORIENTED_EDGE ( 'NONE', *, *, #35248, .T. ) ;
#50744=CARTESIAN_POINT ( 'NONE',  ( -156.6671849566220089, -189.7472609257535510, 60.59166255800404599 ) ) ;
#50747=AXIS2_PLACEMENT_3D ( 'NONE', #21520, #16812, #41214 ) ;
#50748=LINE ( 'NONE', #10033, #28562 ) ;
#50750=VERTEX_POINT ( 'NONE', #28481 ) ;
#50754=CARTESIAN_POINT ( 'NONE',  ( -164.2529447963538871, -177.1207230881787780, 44.41421852208711840 ) ) ;
#50756=VERTEX_POINT ( 'NONE', #29277 ) ;
#50757=ADVANCED_FACE ( 'NONE', ( #44275 ), #5375, .T. ) ;
#50759=VECTOR ( 'NONE', #13222, 1000.000000000000000 ) ;
#50760=CARTESIAN_POINT ( 'NONE',  ( 14.72514937628682574, -175.3837268820161057, -106.6827995071083848 ) ) ;
#50761=EDGE_CURVE ( 'NONE', #46206, #28789, #32945, .T. ) ;
#50763=CARTESIAN_POINT ( 'NONE',  ( -40.24578378811990831, -175.3837268820161057, 124.7285535218268251 ) ) ;
#50764=VERTEX_POINT ( 'NONE', #28999 ) ;
#50768=LINE ( 'NONE', #38917, #21082 ) ;
#50770=EDGE_LOOP ( 'NONE', ( #42404, #34072, #45688, #23674 ) ) ;
#50772=CARTESIAN_POINT ( 'NONE',  ( -166.6265240196292439, -193.5000000000000000, 40.81902153125349741 ) ) ;
#50773=LINE ( 'NONE', #38666, #42606 ) ;
#50776=AXIS2_PLACEMENT_3D ( 'NONE', #44516, #11219, #36630 ) ;
#50777=EDGE_CURVE ( 'NONE', #30132, #13839, #45906, .T. ) ;
#50779=VECTOR ( 'NONE', #3644, 1000.000000000000000 ) ;
#50780=ORIENTED_EDGE ( 'NONE', *, *, #49762, .F. ) ;
#50781=DIRECTION ( 'NONE',  ( 0.000000000000000000, 1.000000000000000000, -0.000000000000000000 ) ) ;
#50782=ORIENTED_EDGE ( 'NONE', *, *, #43262, .F. ) ;
#50785=CARTESIAN_POINT ( 'NONE',  ( 67.29303306501927295, -193.5000000000000000, 47.13604789772129777 ) ) ;
#50786=EDGE_LOOP ( 'NONE', ( #33268, #2684, #2025, #5995 ) ) ;
#50788=ORIENTED_EDGE ( 'NONE', *, *, #28834, .F. ) ;
#50790=DIRECTION ( 'NONE',  ( -0.4031234292879730674, 0.000000000000000000, 0.9151456172430181280 ) ) ;
#50791=ORIENTED_EDGE ( 'NONE', *, *, #39174, .T. ) ;
#50792=CIRCLE ( 'NONE', #41544, 125.0000000000000000 ) ;
#50793=CARTESIAN_POINT ( 'NONE',  ( -48.30901192927175458, -175.3837268820161057, -124.9998842437354227 ) ) ;
#50796=ORIENTED_EDGE ( 'NONE', *, *, #8348, .F. ) ;
#50797=DIRECTION ( 'NONE',  ( 0.000000000000000000, 1.000000000000000000, 0.000000000000000000 ) ) ;
#50798=AXIS2_PLACEMENT_3D ( 'NONE', #32325, #36812, #808 ) ;
#50804=EDGE_LOOP ( 'NONE', ( #42892, #5933, #20493, #4532 ) ) ;
#50806=DIRECTION ( 'NONE',  ( -0.000000000000000000, 1.000000000000000000, 0.000000000000000000 ) ) ;
#50808=PLANE ( 'NONE',  #13463 ) ;
#50809=DIRECTION ( 'NONE',  ( -0.9960498426152177842, 0.000000000000000000, 0.08879589532292482545 ) ) ;
#50810=CARTESIAN_POINT ( 'NONE',  ( -126.2322430781613605, -193.5000000000000000, 97.87467957288053810 ) ) ;
#50812=ORIENTED_EDGE ( 'NONE', *, *, #6757, .T. ) ;
#50815=DIRECTION ( 'NONE',  ( 0.000000000000000000, 1.000000000000000000, 0.000000000000000000 ) ) ;
#50816=DIRECTION ( 'NONE',  ( -0.000000000000000000, 1.000000000000000000, 0.000000000000000000 ) ) ;
#50817=CYLINDRICAL_SURFACE ( 'NONE', #48859, 125.0000000000000000 ) ;
#50819=AXIS2_PLACEMENT_3D ( 'NONE', #30538, #15057, #26854 ) ;
#50820=VECTOR ( 'NONE', #26045, 1000.000000000000114 ) ;
#50822=EDGE_CURVE ( 'NONE', #29368, #32936, #33326, .T. ) ;
#50824=PLANE ( 'NONE',  #40854 ) ;
#50825=AXIS2_PLACEMENT_3D ( 'NONE', #38764, #3030, #42457 ) ;
#50826=DIRECTION ( 'NONE',  ( 0.000000000000000000, -1.000000000000000000, 0.000000000000000000 ) ) ;
#50827=ORIENTED_EDGE ( 'NONE', *, *, #15792, .F. ) ;
#50829=CIRCLE ( 'NONE', #34005, 125.0000000000000000 ) ;
#50830=ORIENTED_EDGE ( 'NONE', *, *, #32711, .T. ) ;
#50834=DIRECTION ( 'NONE',  ( -0.9890401873221654760, 0.000000000000000000, 0.1476465640024710868 ) ) ;
#50835=VECTOR ( 'NONE', #44966, 1000.000000000000000 ) ;
#50837=ORIENTED_EDGE ( 'NONE', *, *, #51268, .F. ) ;
#50839=ORIENTED_EDGE ( 'NONE', *, *, #13135, .T. ) ;
#50840=CIRCLE ( 'NONE', #31534, 125.0000000000000000 ) ;
#50841=DIRECTION ( 'NONE',  ( -0.000000000000000000, 1.000000000000000000, -0.000000000000000000 ) ) ;
#50843=CARTESIAN_POINT ( 'NONE',  ( 141.7825277784304205, -193.5000000000000000, -41.45482488023466061 ) ) ;
#50844=EDGE_CURVE ( 'NONE', #39155, #3968, #37414, .T. ) ;
#50845=DIRECTION ( 'NONE',  ( 0.000000000000000000, -0.000000000000000000, 1.000000000000000000 ) ) ;
#50846=CARTESIAN_POINT ( 'NONE',  ( -74.51199343215195370, -183.6283474603465606, -122.2591094863195025 ) ) ;
#50847=ORIENTED_EDGE ( 'NONE', *, *, #27253, .T. ) ;
#50848=DIRECTION ( 'NONE',  ( -0.000000000000000000, 1.000000000000000000, -0.000000000000000000 ) ) ;
#50849=CARTESIAN_POINT ( 'NONE',  ( 20.66186849114819069, -189.7472609257535510, -104.1370384486465070 ) ) ;
#50850=EDGE_CURVE ( 'NONE', #18822, #15614, #13510, .T. ) ;
#50851=ORIENTED_EDGE ( 'NONE', *, *, #45847, .T. ) ;
#50855=CARTESIAN_POINT ( 'NONE',  ( 73.87536152799695799, -189.7472609257535510, -25.58083653558412252 ) ) ;
#50856=CARTESIAN_POINT ( 'NONE',  ( -28.74596282265200387, -177.1207230881787780, 123.4325817657431230 ) ) ;
#50860=CARTESIAN_POINT ( 'NONE',  ( -155.9608607592037401, -183.6283474603465606, 63.81752780153057358 ) ) ;
#50861=LINE ( 'NONE', #14868, #50316 ) ;
#50862=EDGE_LOOP ( 'NONE', ( #13000, #1215, #49371, #8803 ) ) ;
#50864=ADVANCED_FACE ( 'NONE', ( #5644 ), #10795, .T. ) ;
#50865=ORIENTED_EDGE ( 'NONE', *, *, #35449, .F. ) ;
#50866=CARTESIAN_POINT ( 'NONE',  ( -23.01747912075234836, -193.5000000000000000, -122.3793467049370634 ) ) ;
#50867=CARTESIAN_POINT ( 'NONE',  ( -49.03777351731249468, -189.7472609257535510, -0.8294056854502022125 ) ) ;
#50868=EDGE_LOOP ( 'NONE', ( #21042, #40487, #22615, #40744 ) ) ;
#50870=DIRECTION ( 'NONE',  ( 0.000000000000000000, -0.000000000000000000, 1.000000000000000000 ) ) ;
#50871=DIRECTION ( 'NONE',  ( 0.1768902751225733261, 0.000000000000000000, -0.9842305779475966077 ) ) ;
#50873=VECTOR ( 'NONE', #32864, 1000.000000000000114 ) ;
#50874=CARTESIAN_POINT ( 'NONE',  ( -48.47912675150885065, -183.6283474603465606, 6.938893903907228378E-15 ) ) ;
#50878=VERTEX_POINT ( 'NONE', #41612 ) ;
#50879=CARTESIAN_POINT ( 'NONE',  ( -129.5578577291867646, -193.5000000000000000, 93.82025162278056030 ) ) ;
#50881=ORIENTED_EDGE ( 'NONE', *, *, #10270, .F. ) ;
#50883=PLANE ( 'NONE',  #46457 ) ;
#50885=VERTEX_POINT ( 'NONE', #9831 ) ;
#50886=DIRECTION ( 'NONE',  ( 0.6749830015182038956, 0.000000000000000000, 0.7378332790417333475 ) ) ;
#50888=AXIS2_PLACEMENT_3D ( 'NONE', #17532, #33281, #24878 ) ;
#50889=VECTOR ( 'NONE', #7038, 1000.000000000000114 ) ;
#50890=VERTEX_POINT ( 'NONE', #37686 ) ;
#50893=EDGE_LOOP ( 'NONE', ( #47372, #32079, #30883, #34650 ) ) ;
#50895=AXIS2_PLACEMENT_3D ( 'NONE', #12899, #5038, #11019 ) ;
#50898=LINE ( 'NONE', #11440, #21053 ) ;
#50899=CARTESIAN_POINT ( 'NONE',  ( -172.9089226952081901, -175.3837268820161057, 11.92584929509617986 ) ) ;
#50900=ORIENTED_EDGE ( 'NONE', *, *, #43803, .F. ) ;
#50902=ORIENTED_EDGE ( 'NONE', *, *, #21951, .T. ) ;
#50905=AXIS2_PLACEMENT_3D ( 'NONE', #19557, #39275, #3281 ) ;
#50906=AXIS2_PLACEMENT_3D ( 'NONE', #12638, #3992, #44191 ) ;
#50908=( NAMED_UNIT ( * ) PLANE_ANGLE_UNIT ( ) SI_UNIT ( $, .RADIAN. ) );
#50909=AXIS2_PLACEMENT_3D ( 'NONE', #2338, #14172, #5509 ) ;
#50910=DIRECTION ( 'NONE',  ( -0.000000000000000000, 1.000000000000000000, -0.000000000000000000 ) ) ;
#50915=FACE_OUTER_BOUND ( 'NONE', #9445, .T. ) ;
#50917=PLANE ( 'NONE',  #37380 ) ;
#50918=VERTEX_POINT ( 'NONE', #49782 ) ;
#50919=EDGE_LOOP ( 'NONE', ( #11310, #18741, #16229, #2479 ) ) ;
#50920=DIRECTION ( 'NONE',  ( 0.000000000000000000, -1.000000000000000000, -0.000000000000000000 ) ) ;
#50921=CARTESIAN_POINT ( 'NONE',  ( -172.9089226952081617, -189.7472609257535510, 11.92584929509620117 ) ) ;
#50922=PLANE ( 'NONE',  #4508 ) ;
#50923=CARTESIAN_POINT ( 'NONE',  ( -65.65563056894596627, -177.1207230881787780, 123.8142468240612999 ) ) ;
#50924=ORIENTED_EDGE ( 'NONE', *, *, #22051, .T. ) ;
#50926=ORIENTED_EDGE ( 'NONE', *, *, #22122, .F. ) ;
#50927=VERTEX_POINT ( 'NONE', #27063 ) ;
#50929=VECTOR ( 'NONE', #14038, 1000.000000000000000 ) ;
#50932=DIRECTION ( 'NONE',  ( -0.000000000000000000, 1.000000000000000000, -0.000000000000000000 ) ) ;
#50933=DIRECTION ( 'NONE',  ( -0.000000000000000000, -1.000000000000000000, 0.000000000000000000 ) ) ;
#50936=CYLINDRICAL_SURFACE ( 'NONE', #41534, 125.0000000000000000 ) ;
#50937=VECTOR ( 'NONE', #19189, 1000.000000000000000 ) ;
#50939=EDGE_CURVE ( 'NONE', #18052, #7546, #33988, .T. ) ;
#50940=CARTESIAN_POINT ( 'NONE',  ( -154.5708152632604708, -193.5000000000000000, 64.19309449102807719 ) ) ;
#50941=LINE ( 'NONE', #14942, #25406 ) ;
#50943=DIRECTION ( 'NONE',  ( 0.9266896074318317078, 0.000000000000000000, 0.3758275821142421647 ) ) ;
#50945=DIRECTION ( 'NONE',  ( 0.000000000000000000, 0.000000000000000000, -1.000000000000000000 ) ) ;
#50946=ORIENTED_EDGE ( 'NONE', *, *, #31699, .T. ) ;
#50947=CIRCLE ( 'NONE', #30778, 125.0000000000000000 ) ;
#50948=AXIS2_PLACEMENT_3D ( 'NONE', #17651, #9238, #26034 ) ;
#50950=AXIS2_PLACEMENT_3D ( 'NONE', #9540, #37657, #18209 ) ;
#50952=CARTESIAN_POINT ( 'NONE',  ( -153.7332855749581881, -193.5000000000000000, 67.42819922234390617 ) ) ;
#50954=PLANE ( 'NONE',  #9467 ) ;
#50955=EDGE_CURVE ( 'NONE', #31330, #6494, #43104, .T. ) ;
#50956=VECTOR ( 'NONE', #43520, 1000.000000000000000 ) ;
#50957=ORIENTED_EDGE ( 'NONE', *, *, #47509, .T. ) ;
#50958=EDGE_CURVE ( 'NONE', #44532, #38288, #37939, .T. ) ;
#50959=VECTOR ( 'NONE', #13169, 1000.000000000000114 ) ;
#50962=FACE_BOUND ( 'NONE', #26902, .T. ) ;
#50963=PLANE ( 'NONE',  #18722 ) ;
#50964=DIRECTION ( 'NONE',  ( 0.9266896074318343723, 0.000000000000000000, -0.3758275821142357809 ) ) ;
#50966=VERTEX_POINT ( 'NONE', #30760 ) ;
#50970=VERTEX_POINT ( 'NONE', #33737 ) ;
#50971=DIRECTION ( 'NONE',  ( -0.1182731709213592358, 0.000000000000000000, -0.9929810960135178055 ) ) ;
#50972=VECTOR ( 'NONE', #28168, 1000.000000000000000 ) ;
#50973=DIRECTION ( 'NONE',  ( -0.000000000000000000, 1.000000000000000000, 0.000000000000000000 ) ) ;
#50974=CARTESIAN_POINT ( 'NONE',  ( -19.92568551777507224, -189.7472609257535510, -121.6951149130962904 ) ) ;
#50975=VERTEX_POINT ( 'NONE', #25856 ) ;
#50977=CARTESIAN_POINT ( 'NONE',  ( -49.17567778057184569, -189.7472609257535510, -0.7175072570443327136 ) ) ;
#50981=CIRCLE ( 'NONE', #24122, 125.0000000000000000 ) ;
#50982=CARTESIAN_POINT ( 'NONE',  ( -161.6832731452239784, -193.5000000000000000, -53.00774697410100345 ) ) ;
#50983=ORIENTED_EDGE ( 'NONE', *, *, #8758, .T. ) ;
#50984=DIRECTION ( 'NONE',  ( 0.000000000000000000, -1.000000000000000000, 0.000000000000000000 ) ) ;
#50985=ORIENTED_EDGE ( 'NONE', *, *, #33184, .F. ) ;
#50986=AXIS2_PLACEMENT_3D ( 'NONE', #5073, #40789, #17434 ) ;
#50987=DIRECTION ( 'NONE',  ( -0.000000000000000000, 1.000000000000000000, -0.000000000000000000 ) ) ;
#50988=EDGE_LOOP ( 'NONE', ( #22764, #31434, #26472, #18735 ) ) ;
#50989=FACE_OUTER_BOUND ( 'NONE', #12745, .T. ) ;
#50992=VERTEX_POINT ( 'NONE', #33492 ) ;
#50993=CIRCLE ( 'NONE', #30835, 125.0000000000000000 ) ;
#50994=DIRECTION ( 'NONE',  ( 0.000000000000000000, 0.000000000000000000, -1.000000000000000000 ) ) ;
#50995=ORIENTED_EDGE ( 'NONE', *, *, #46373, .T. ) ;
#50997=CARTESIAN_POINT ( 'NONE',  ( -49.29161362951453640, -189.7472609257535510, 0.5829794791144718991 ) ) ;
#50998=ORIENTED_EDGE ( 'NONE', *, *, #11520, .T. ) ;
#50999=FACE_OUTER_BOUND ( 'NONE', #34154, .T. ) ;
#51000=FACE_OUTER_BOUND ( 'NONE', #2882, .T. ) ;
#51001=PLANE ( 'NONE',  #10641 ) ;
#51003=EDGE_CURVE ( 'NONE', #30945, #9782, #46722, .T. ) ;
#51005=VERTEX_POINT ( 'NONE', #14145 ) ;
#51006=EDGE_CURVE ( 'NONE', #36852, #20677, #5616, .T. ) ;
#51008=CARTESIAN_POINT ( 'NONE',  ( -47.47956591500005885, -193.5000000000000000, 0.02963332782257025594 ) ) ;
#51011=CARTESIAN_POINT ( 'NONE',  ( -135.6699833737243353, -175.3837268820161057, 89.56983042009328244 ) ) ;
#51012=ORIENTED_EDGE ( 'NONE', *, *, #40249, .T. ) ;
#51015=CARTESIAN_POINT ( 'NONE',  ( -92.16375985330358844, -189.7472609257535510, 117.1181148702521710 ) ) ;
#51016=ADVANCED_FACE ( 'NONE', ( #20784 ), #37063, .T. ) ;
#51017=CARTESIAN_POINT ( 'NONE',  ( -48.47912675150885065, -175.3837268820161057, 6.938893903907228378E-15 ) ) ;
#51019=DIRECTION ( 'NONE',  ( -0.000000000000000000, 1.000000000000000000, -0.000000000000000000 ) ) ;
#51020=CIRCLE ( 'NONE', #33372, 125.0000000000000000 ) ;
#51022=DIRECTION ( 'NONE',  ( 0.000000000000000000, 0.000000000000000000, 1.000000000000000000 ) ) ;
#51026=ADVANCED_FACE ( 'NONE', ( #34360 ), #34098, .T. ) ;
#51028=DIRECTION ( 'NONE',  ( 0.000000000000000000, 0.000000000000000000, -1.000000000000000000 ) ) ;
#51029=EDGE_CURVE ( 'NONE', #14630, #23392, #44443, .T. ) ;
#51031=DIRECTION ( 'NONE',  ( -0.9266896074318317078, 0.000000000000000000, -0.3758275821142421647 ) ) ;
#51034=EDGE_CURVE ( 'NONE', #1472, #44801, #48656, .T. ) ;
#51037=CIRCLE ( 'NONE', #17463, 125.0000000000000000 ) ;
#51038=DIRECTION ( 'NONE',  ( 0.000000000000000000, 0.000000000000000000, -1.000000000000000000 ) ) ;
#51041=ORIENTED_EDGE ( 'NONE', *, *, #35748, .F. ) ;
#51043=CARTESIAN_POINT ( 'NONE',  ( -37.67038537088847505, -183.6283474603465606, -124.5318076226586470 ) ) ;
#51044=VERTEX_POINT ( 'NONE', #38029 ) ;
#51045=EDGE_CURVE ( 'NONE', #27304, #4539, #44970, .T. ) ;
#51047=DIRECTION ( 'NONE',  ( 0.000000000000000000, -1.000000000000000000, 0.000000000000000000 ) ) ;
#51048=DIRECTION ( 'NONE',  ( 0.000000000000000000, 1.000000000000000000, 0.000000000000000000 ) ) ;
#51050=ORIENTED_EDGE ( 'NONE', *, *, #16, .F. ) ;
#51051=AXIS2_PLACEMENT_3D ( 'NONE', #49573, #34045, #38236 ) ;
#51053=EDGE_LOOP ( 'NONE', ( #6802, #19091, #21648, #35736 ) ) ;
#51054=CARTESIAN_POINT ( 'NONE',  ( -136.1415351158078693, -189.7472609257535510, -89.10837311819173578 ) ) ;
#51056=EDGE_LOOP ( 'NONE', ( #51748, #45050, #15542, #2720 ) ) ;
#51058=CYLINDRICAL_SURFACE ( 'NONE', #18756, 125.0000000000000000 ) ;
#51059=CARTESIAN_POINT ( 'NONE',  ( -70.75782287548091176, -175.3837268820161057, 122.9986166548864901 ) ) ;
#51060=CARTESIAN_POINT ( 'NONE',  ( -49.35486169370449971, -193.5000000000000000, 0.4827922027307437469 ) ) ;
#51061=ORIENTED_EDGE ( 'NONE', *, *, #31542, .T. ) ;
#51063=AXIS2_PLACEMENT_3D ( 'NONE', #51344, #5010, #27675 ) ;
#51065=DIRECTION ( 'NONE',  ( 0.000000000000000000, 0.000000000000000000, 1.000000000000000000 ) ) ;
#51066=DIRECTION ( 'NONE',  ( -0.000000000000000000, 1.000000000000000000, -0.000000000000000000 ) ) ;
#51068=CARTESIAN_POINT ( 'NONE',  ( -97.70585564814136603, -193.5000000000000000, 113.8100815915419304 ) ) ;
#51069=CARTESIAN_POINT ( 'NONE',  ( 66.11593792271145276, -189.7472609257535510, -47.37063079638321739 ) ) ;
#51070=EDGE_CURVE ( 'NONE', #20987, #47304, #41005, .T. ) ;
#51071=EDGE_CURVE ( 'NONE', #18280, #40458, #7331, .T. ) ;
#51072=ORIENTED_EDGE ( 'NONE', *, *, #50308, .F. ) ;
#51074=CARTESIAN_POINT ( 'NONE',  ( 58.45385938022560168, -183.6283474603465606, 62.78108192022013867 ) ) ;
#51076=EDGE_CURVE ( 'NONE', #36064, #28789, #42229, .T. ) ;
#51077=VECTOR ( 'NONE', #9738, 1000.000000000000000 ) ;
#51078=VERTEX_POINT ( 'NONE', #20512 ) ;
#51082=EDGE_CURVE ( 'NONE', #32088, #38087, #8148, .T. ) ;
#51083=CARTESIAN_POINT ( 'NONE',  ( -49.29161362951452929, -177.1207230881787780, -0.5829794791144748967 ) ) ;
#51084=EDGE_LOOP ( 'NONE', ( #6783, #35959, #9399, #40517 ) ) ;
#51086=LINE ( 'NONE', #30556, #41499 ) ;
#51087=DIRECTION ( 'NONE',  ( -0.000000000000000000, 1.000000000000000000, -0.000000000000000000 ) ) ;
#51088=ADVANCED_FACE ( 'NONE', ( #7540 ), #42495, .F. ) ;
#51090=DIRECTION ( 'NONE',  ( 0.000000000000000000, -0.000000000000000000, -1.000000000000000000 ) ) ;
#51092=AXIS2_PLACEMENT_3D ( 'NONE', #16989, #2755, #47176 ) ;
#51093=EDGE_CURVE ( 'NONE', #22006, #34216, #35869, .T. ) ;
#51095=DIRECTION ( 'NONE',  ( 0.000000000000000000, 0.000000000000000000, 1.000000000000000000 ) ) ;
#51096=CARTESIAN_POINT ( 'NONE',  ( -49.46816693883101124, -175.3837268820161057, -0.1476465640024848536 ) ) ;
#51099=CIRCLE ( 'NONE', #19188, 125.0000000000000000 ) ;
#51102=CARTESIAN_POINT ( 'NONE',  ( 58.95724912996274725, -193.5000000000000000, 61.91627321685103880 ) ) ;
#51103=EDGE_CURVE ( 'NONE', #39243, #9591, #47482, .T. ) ;
#51104=DIRECTION ( 'NONE',  ( 0.000000000000000000, 1.000000000000000000, 0.000000000000000000 ) ) ;
#51105=ORIENTED_EDGE ( 'NONE', *, *, #15462, .T. ) ;
#51109=EDGE_LOOP ( 'NONE', ( #5564, #14230, #1232, #25845 ) ) ;
#51111=CARTESIAN_POINT ( 'NONE',  ( 62.13187335169531167, -193.5000000000000000, -58.22548115875872554 ) ) ;
#51113=LINE ( 'NONE', #48177, #23266 ) ;
#51115=EDGE_LOOP ( 'NONE', ( #13836, #14844, #3950, #3654 ) ) ;
#51117=VECTOR ( 'NONE', #23050, 1000.000000000000000 ) ;
#51118=EDGE_CURVE ( 'NONE', #35424, #25619, #43269, .T. ) ;
#51120=CARTESIAN_POINT ( 'NONE',  ( -121.5885020763900854, -183.6283474603465606, -101.3904297239421055 ) ) ;
#51122=CARTESIAN_POINT ( 'NONE',  ( -99.62791064391784346, -175.3837268820161057, -114.0561348912352173 ) ) ;
#51123=CARTESIAN_POINT ( 'NONE',  ( -48.88225018079683082, -189.7472609257535510, 0.9151456172430223468 ) ) ;
#51124=ORIENTED_EDGE ( 'NONE', *, *, #19417, .T. ) ;
#51125=CARTESIAN_POINT ( 'NONE',  ( -48.47912675150885065, -183.6283474603465606, 6.938893903907228378E-15 ) ) ;
#51126=CARTESIAN_POINT ( 'NONE',  ( 52.75081385575904136, -175.3837268820161057, 71.61357856150601719 ) ) ;
#51127=ORIENTED_EDGE ( 'NONE', *, *, #39475, .T. ) ;
#51129=AXIS2_PLACEMENT_3D ( 'NONE', #28410, #43927, #8446 ) ;
#51130=LINE ( 'NONE', #18017, #34057 ) ;
#51131=CARTESIAN_POINT ( 'NONE',  ( -59.86929868745821182, -193.5000000000000000, -124.4799742258549600 ) ) ;
#51132=DIRECTION ( 'NONE',  ( 0.000000000000000000, 0.000000000000000000, 1.000000000000000000 ) ) ;
#51133=AXIS2_PLACEMENT_3D ( 'NONE', #51725, #34892, #42533 ) ;
#51135=VECTOR ( 'NONE', #33044, 1000.000000000000000 ) ;
#51138=EDGE_CURVE ( 'NONE', #46759, #41926, #15436, .T. ) ;
#51139=EDGE_LOOP ( 'NONE', ( #43513, #25306, #50642, #48974 ) ) ;
#51140=CARTESIAN_POINT ( 'NONE',  ( -147.0463339291295881, -193.5000000000000000, 76.87330921200150158 ) ) ;
#51142=CARTESIAN_POINT ( 'NONE',  ( -166.8403286750647965, -175.3837268820161057, -40.19484891389966918 ) ) ;
#51143=VECTOR ( 'NONE', #39800, 1000.000000000000000 ) ;
#51145=ORIENTED_EDGE ( 'NONE', *, *, #49485, .T. ) ;
#51146=DIRECTION ( 'NONE',  ( -0.000000000000000000, 1.000000000000000000, -0.000000000000000000 ) ) ;
#51147=FACE_OUTER_BOUND ( 'NONE', #37581, .T. ) ;
#51148=DIRECTION ( 'NONE',  ( 0.000000000000000000, 1.000000000000000000, 0.000000000000000000 ) ) ;
#51149=DIRECTION ( 'NONE',  ( -0.5586467658036415873, 0.000000000000000000, -0.8294056854502090959 ) ) ;
#51150=VECTOR ( 'NONE', #41403, 999.9999999999998863 ) ;
#51153=EDGE_CURVE ( 'NONE', #42763, #138, #51828, .T. ) ;
#51155=LINE ( 'NONE', #15141, #21115 ) ;
#51156=ORIENTED_EDGE ( 'NONE', *, *, #17958, .F. ) ;
#51157=EDGE_LOOP ( 'NONE', ( #45422, #48528, #23546, #44856 ) ) ;
#51160=EDGE_CURVE ( 'NONE', #9630, #23170, #31667, .T. ) ;
#51161=CARTESIAN_POINT ( 'NONE',  ( 73.32544842769512172, -177.1207230881787780, -23.23456943914042228 ) ) ;
#51162=EDGE_LOOP ( 'NONE', ( #12715, #30937, #24647, #21426 ) ) ;
#51163=AXIS2_PLACEMENT_3D ( 'NONE', #25663, #41695, #13579 ) ;
#51164=CARTESIAN_POINT ( 'NONE',  ( 76.21810084846656252, -177.1207230881787780, -8.694908215727989997 ) ) ;
#51165=LINE ( 'NONE', #6995, #49793 ) ;
#51166=EDGE_LOOP ( 'NONE', ( #40009, #24418, #12484, #9961 ) ) ;
#51167=CARTESIAN_POINT ( 'NONE',  ( -114.4014177456970884, -183.6283474603465606, 105.0256126866236031 ) ) ;
#51168=AXIS2_PLACEMENT_3D ( 'NONE', #44035, #23030, #39817 ) ;
#51169=FACE_OUTER_BOUND ( 'NONE', #39123, .T. ) ;
#51170=LINE ( 'NONE', #47733, #15686 ) ;
#51173=EDGE_LOOP ( 'NONE', ( #16199, #2139, #9027, #2874 ) ) ;
#51174=CARTESIAN_POINT ( 'NONE',  ( -82.67254833784559764, -177.1207230881787780, -120.2323164553483963 ) ) ;
#51175=CARTESIAN_POINT ( 'NONE',  ( -47.66663987350317200, -183.6283474603465606, -0.5829794791144634614 ) ) ;
#51176=CARTESIAN_POINT ( 'NONE',  ( -160.2705093830644216, -193.5000000000000000, -55.92572546981520532 ) ) ;
#51178=FACE_OUTER_BOUND ( 'NONE', #42559, .T. ) ;
#51180=VECTOR ( 'NONE', #14129, 1000.000000000000114 ) ;
#51181=DIRECTION ( 'NONE',  ( 0.02963332782254913048, 0.000000000000000000, 0.9995608365087946812 ) ) ;
#51182=VERTEX_POINT ( 'NONE', #23044 ) ;
#51183=CARTESIAN_POINT ( 'NONE',  ( -47.49008656418669005, -189.7472609257535510, -0.1476465640024710591 ) ) ;
#51185=ORIENTED_EDGE ( 'NONE', *, *, #34552, .T. ) ;
#51186=DIRECTION ( 'NONE',  ( -0.9785564922995046988, 0.000000000000000000, 0.2059786187410953262 ) ) ;
#51188=FACE_OUTER_BOUND ( 'NONE', #51115, .T. ) ;
#51189=EDGE_CURVE ( 'NONE', #39634, #42649, #27504, .T. ) ;
#51191=EDGE_LOOP ( 'NONE', ( #9158, #9816, #24492, #30819 ) ) ;
#51193=ORIENTED_EDGE ( 'NONE', *, *, #26947, .F. ) ;
#51196=LINE ( 'NONE', #357, #27270 ) ;
#51197=AXIS2_PLACEMENT_3D ( 'NONE', #4218, #33102, #45221 ) ;
#51201=CARTESIAN_POINT ( 'NONE',  ( -138.3705904895685137, -183.6283474603465606, -86.85922373029302435 ) ) ;
#51203=CARTESIAN_POINT ( 'NONE',  ( -48.65601702663141737, -193.5000000000000000, -0.9842305779475923888 ) ) ;
#51204=VERTEX_POINT ( 'NONE', #3585 ) ;
#51205=DIRECTION ( 'NONE',  ( -0.000000000000000000, 1.000000000000000000, -0.000000000000000000 ) ) ;
#51206=DIRECTION ( 'NONE',  ( 0.000000000000000000, -0.000000000000000000, 1.000000000000000000 ) ) ;
#51207=FACE_BOUND ( 'NONE', #46462, .T. ) ;
#51209=EDGE_CURVE ( 'NONE', #18089, #27933, #23321, .T. ) ;
#51210=DIRECTION ( 'NONE',  ( -0.02963332782255633305, 0.000000000000000000, -0.9995608365087944591 ) ) ;
#51211=DIRECTION ( 'NONE',  ( -0.000000000000000000, 1.000000000000000000, 0.000000000000000000 ) ) ;
#51212=ORIENTED_EDGE ( 'NONE', *, *, #42998, .F. ) ;
#51213=CARTESIAN_POINT ( 'NONE',  ( 33.75048693540709621, -189.7472609257535510, 94.14505102712816154 ) ) ;
#51214=ORIENTED_EDGE ( 'NONE', *, *, #14510, .F. ) ;
#51215=VECTOR ( 'NONE', #14067, 1000.000000000000000 ) ;
#51216=VECTOR ( 'NONE', #6420, 1000.000000000000000 ) ;
#51217=CARTESIAN_POINT ( 'NONE',  ( -9.671950287350391307, -193.5000000000000000, -118.8234112238815499 ) ) ;
#51218=FACE_BOUND ( 'NONE', #24093, .T. ) ;
#51219=CARTESIAN_POINT ( 'NONE',  ( 55.92943606843918047, -193.5000000000000000, -66.89437584437831674 ) ) ;
#51220=ORIENTED_EDGE ( 'NONE', *, *, #38767, .F. ) ;
#51221=CARTESIAN_POINT ( 'NONE',  ( -49.08592689732745384, -189.7472609257535510, 0.7948544414133550395 ) ) ;
#51222=VERTEX_POINT ( 'NONE', #3334 ) ;
#51223=VERTEX_POINT ( 'NONE', #14389 ) ;
#51224=CARTESIAN_POINT ( 'NONE',  ( -5.461633243180957109, -189.7472609257535510, 116.2991637277478247 ) ) ;
#51227=DIRECTION ( 'NONE',  ( -0.000000000000000000, 1.000000000000000000, -0.000000000000000000 ) ) ;
#51229=EDGE_CURVE ( 'NONE', #49925, #33429, #10431, .T. ) ;
#51230=DIRECTION ( 'NONE',  ( -0.000000000000000000, 1.000000000000000000, -0.000000000000000000 ) ) ;
#51232=EDGE_LOOP ( 'NONE', ( #37107, #11827, #22055, #24059 ) ) ;
#51234=CARTESIAN_POINT ( 'NONE',  ( -112.2501518587238962, -175.3837268820161057, -106.3450133598699807 ) ) ;
#51235=VERTEX_POINT ( 'NONE', #22545 ) ;
#51236=DIRECTION ( 'NONE',  ( 0.9646355819083594074, 0.000000000000000000, -0.2635871660690647933 ) ) ;
#51237=ORIENTED_EDGE ( 'NONE', *, *, #7569, .F. ) ;
#51238=FACE_OUTER_BOUND ( 'NONE', #609, .T. ) ;
#51240=ADVANCED_FACE ( 'NONE', ( #46712 ), #10957, .F. ) ;
#51243=FACE_OUTER_BOUND ( 'NONE', #16472, .T. ) ;
#51244=CARTESIAN_POINT ( 'NONE',  ( 8.294189685504184339, -193.5000000000000000, -110.2396968984190977 ) ) ;
#51245=EDGE_LOOP ( 'NONE', ( #40883, #23114, #18699, #48852 ) ) ;
#51246=EDGE_CURVE ( 'NONE', #41798, #44424, #40014, .T. ) ;
#51247=VECTOR ( 'NONE', #23665, 1000.000000000000114 ) ;
#51248=AXIS2_PLACEMENT_3D ( 'NONE', #46812, #18430, #14490 ) ;
#51251=LINE ( 'NONE', #27046, #8597 ) ;
#51254=VERTEX_POINT ( 'NONE', #7019 ) ;
#51255=DIRECTION ( 'NONE',  ( -0.000000000000000000, 1.000000000000000000, -0.000000000000000000 ) ) ;
#51257=PLANE ( 'NONE',  #46742 ) ;
#51258=PLANE ( 'NONE',  #18177 ) ;
#51259=ORIENTED_EDGE ( 'NONE', *, *, #48478, .F. ) ;
#51261=DIRECTION ( 'NONE',  ( -0.6528221181905119463, 0.000000000000000000, -0.7575112421616284619 ) ) ;
#51262=CARTESIAN_POINT ( 'NONE',  ( -47.97059563285963435, -177.1207230881787780, 0.8610436117673654355 ) ) ;
#51263=CARTESIAN_POINT ( 'NONE',  ( -72.72541169915515979, -183.6283474603465606, 121.6072260099955429 ) ) ;
#51264=VERTEX_POINT ( 'NONE', #40344 ) ;
#51265=CIRCLE ( 'NONE', #2559, 125.0000000000000000 ) ;
#51266=CARTESIAN_POINT ( 'NONE',  ( 9.336583202542589888, -193.5000000000000000, 110.8257356506556306 ) ) ;
#51267=PLANE ( 'NONE',  #21066 ) ;
#51268=EDGE_CURVE ( 'NONE', #12134, #3363, #51692, .T. ) ;
#51269=CARTESIAN_POINT ( 'NONE',  ( -113.5519059482138857, -177.1207230881787780, 105.5544085257715210 ) ) ;
#51270=CARTESIAN_POINT ( 'NONE',  ( 2.266533711611407043, -175.3837268820161057, 113.1409892739925453 ) ) ;
#51271=VERTEX_POINT ( 'NONE', #44832 ) ;
#51273=DIRECTION ( 'NONE',  ( 0.000000000000000000, -1.000000000000000000, 0.000000000000000000 ) ) ;
#51274=LINE ( 'NONE', #48098, #11937 ) ;
#51276=DIRECTION ( 'NONE',  ( 0.1182731709213592358, 0.000000000000000000, 0.9929810960135178055 ) ) ;
#51277=AXIS2_PLACEMENT_3D ( 'NONE', #5843, #29991, #49712 ) ;
#51278=ORIENTED_EDGE ( 'NONE', *, *, #9893, .F. ) ;
#51281=VERTEX_POINT ( 'NONE', #51963 ) ;
#51282=ORIENTED_EDGE ( 'NONE', *, *, #46811, .T. ) ;
#51285=ADVANCED_FACE ( 'NONE', ( #35640 ), #4365, .F. ) ;
#51286=DIRECTION ( 'NONE',  ( 0.000000000000000000, 0.000000000000000000, 1.000000000000000000 ) ) ;
#51287=ORIENTED_EDGE ( 'NONE', *, *, #46279, .F. ) ;
#51288=DIRECTION ( 'NONE',  ( -0.000000000000000000, 1.000000000000000000, -0.000000000000000000 ) ) ;
#51290=CARTESIAN_POINT ( 'NONE',  ( -5.461633243180942898, -193.5000000000000000, 116.2991637277478247 ) ) ;
#51292=VERTEX_POINT ( 'NONE', #44047 ) ;
#51294=DIRECTION ( 'NONE',  ( 0.000000000000000000, 0.000000000000000000, -1.000000000000000000 ) ) ;
#51295=ORIENTED_EDGE ( 'NONE', *, *, #3543, .T. ) ;
#51296=CARTESIAN_POINT ( 'NONE',  ( -47.55243714407701816, -177.1207230881787780, -0.3758275821142288420 ) ) ;
#51298=CARTESIAN_POINT ( 'NONE',  ( -49.03777351731250889, -189.7472609257535510, 0.8294056854502042109 ) ) ;
#51299=ADVANCED_FACE ( 'NONE', ( #36412 ), #24592, .T. ) ;
#51301=CARTESIAN_POINT ( 'NONE',  ( -84.19171550243319757, -189.7472609257535510, 119.7898618611247628 ) ) ;
#51303=ORIENTED_EDGE ( 'NONE', *, *, #21703, .T. ) ;
#51304=EDGE_CURVE ( 'NONE', #3228, #4055, #48447, .T. ) ;
#51305=CARTESIAN_POINT ( 'NONE',  ( -47.92047998570520662, -175.3837268820161057, 0.8294056854502119824 ) ) ;
#51306=ORIENTED_EDGE ( 'NONE', *, *, #39433, .F. ) ;
#51307=CARTESIAN_POINT ( 'NONE',  ( -49.32472275501067571, -193.5000000000000000, -0.5338233779647935107 ) ) ;
#51309=CARTESIAN_POINT ( 'NONE',  ( -106.4764934152197497, -213.5000000000000000, -110.7307791902282759 ) ) ;
#51312=VECTOR ( 'NONE', #47119, 1000.000000000000114 ) ;
#51313=LINE ( 'NONE', #23196, #34885 ) ;
#51315=EDGE_LOOP ( 'NONE', ( #27432, #12999, #17512, #5097 ) ) ;
#51318=AXIS2_PLACEMENT_3D ( 'NONE', #30837, #50815, #42910 ) ;
#51319=VERTEX_POINT ( 'NONE', #12512 ) ;
#51320=CARTESIAN_POINT ( 'NONE',  ( 66.03142248012325410, -177.1207230881787780, 50.12318939044039467 ) ) ;
#51321=ORIENTED_EDGE ( 'NONE', *, *, #14766, .F. ) ;
#51322=DIRECTION ( 'NONE',  ( -0.000000000000000000, 1.000000000000000000, -0.000000000000000000 ) ) ;
#51323=DIRECTION ( 'NONE',  ( 0.000000000000000000, 0.000000000000000000, 1.000000000000000000 ) ) ;
#51325=DIRECTION ( 'NONE',  ( -0.000000000000000000, 1.000000000000000000, -0.000000000000000000 ) ) ;
#51326=CARTESIAN_POINT ( 'NONE',  ( -48.47912675150885065, -183.6283474603465606, 6.938893903907228378E-15 ) ) ;
#51327=LINE ( 'NONE', #39474, #46724 ) ;
#51328=VECTOR ( 'NONE', #28746, 1000.000000000000000 ) ;
#51329=CARTESIAN_POINT ( 'NONE',  ( -49.40581635894068313, -177.1207230881787780, -0.3758275821142418316 ) ) ;
#51330=EDGE_CURVE ( 'NONE', #20850, #6563, #31709, .T. ) ;
#51331=VECTOR ( 'NONE', #42347, 1000.000000000000000 ) ;
#51332=LINE ( 'NONE', #3482, #14439 ) ;
#51333=CARTESIAN_POINT ( 'NONE',  ( -48.47912675150885065, -175.3837268820161057, 6.938893903907228378E-15 ) ) ;
#51334=LINE ( 'NONE', #6673, #27002 ) ;
#51336=ORIENTED_EDGE ( 'NONE', *, *, #4140, .F. ) ;
#51337=DIRECTION ( 'NONE',  ( 0.000000000000000000, 0.000000000000000000, -1.000000000000000000 ) ) ;
#51338=EDGE_CURVE ( 'NONE', #41926, #43754, #40887, .T. ) ;
#51339=CARTESIAN_POINT ( 'NONE',  ( -153.2421220336517820, -193.5000000000000000, -66.33788548805446794 ) ) ;
#51342=FACE_OUTER_BOUND ( 'NONE', #45425, .T. ) ;
#51343=EDGE_LOOP ( 'NONE', ( #26994, #1729, #6140, #7944 ) ) ;
#51344=CARTESIAN_POINT ( 'NONE',  ( -48.47912675150885065, -175.3837268820161057, 6.938893903907228378E-15 ) ) ;
#51345=CARTESIAN_POINT ( 'NONE',  ( -48.47912675150885065, -189.7472609257535510, 6.938893903907228378E-15 ) ) ;
#51346=VECTOR ( 'NONE', #47189, 1000.000000000000114 ) ;
#51347=EDGE_CURVE ( 'NONE', #39427, #43863, #15952, .T. ) ;
#51348=ADVANCED_FACE ( 'NONE', ( #35910 ), #31959, .T. ) ;
#51350=EDGE_CURVE ( 'NONE', #44477, #45342, #18252, .T. ) ;
#51351=CARTESIAN_POINT ( 'NONE',  ( 74.31448861501726810, -183.6283474603465606, -23.38221600314288651 ) ) ;
#51352=DIRECTION ( 'NONE',  ( 0.000000000000000000, -1.000000000000000000, -0.000000000000000000 ) ) ;
#51353=CIRCLE ( 'NONE', #27797, 124.9999999999999858 ) ;
#51354=VERTEX_POINT ( 'NONE', #28778 ) ;
#51355=ORIENTED_EDGE ( 'NONE', *, *, #5805, .F. ) ;
#51356=ADVANCED_FACE ( 'NONE', ( #8051 ), #28010, .T. ) ;
#51357=AXIS2_PLACEMENT_3D ( 'NONE', #14237, #49978, #50247 ) ;
#51358=EDGE_LOOP ( 'NONE', ( #33232, #51737, #2392, #15762 ) ) ;
#51359=CARTESIAN_POINT ( 'NONE',  ( -48.24424070572786860, -177.1207230881787780, -0.9720229140804037549 ) ) ;
#51360=CARTESIAN_POINT ( 'NONE',  ( -99.22478721462985618, -175.3837268820161057, -113.1409892739921901 ) ) ;
#51361=CARTESIAN_POINT ( 'NONE',  ( -47.82630463331832971, -193.5000000000000000, -0.7575112421616121416 ) ) ;
#51362=EDGE_CURVE ( 'NONE', #23489, #48517, #44328, .T. ) ;
#51363=CARTESIAN_POINT ( 'NONE',  ( -49.45768324380835423, -175.3837268820161057, -0.2059786187411025149 ) ) ;
#51364=DIRECTION ( 'NONE',  ( 0.000000000000000000, 0.000000000000000000, 1.000000000000000000 ) ) ;
#51367=CARTESIAN_POINT ( 'NONE',  ( -123.4791267515088435, -198.5000000000000000, 70.00000000000000000 ) ) ;
#51368=CARTESIAN_POINT ( 'NONE',  ( 15.29189835570547551, -189.7472609257535510, 106.3450133598704213 ) ) ;
#51370=VERTEX_POINT ( 'NONE', #42168 ) ;
#51371=ORIENTED_EDGE ( 'NONE', *, *, #32776, .T. ) ;
#51373=AXIS2_PLACEMENT_3D ( 'NONE', #34587, #25939, #41713 ) ;
#51374=CARTESIAN_POINT ( 'NONE',  ( -172.6359455740846442, -193.5000000000000000, -14.49428645563791562 ) ) ;
#51375=EDGE_CURVE ( 'NONE', #44410, #45844, #5417, .T. ) ;
#51376=DIRECTION ( 'NONE',  ( -0.000000000000000000, 1.000000000000000000, -0.000000000000000000 ) ) ;
#51377=ORIENTED_EDGE ( 'NONE', *, *, #41395, .T. ) ;
#51379=ADVANCED_FACE ( 'NONE', ( #5159 ), #13293, .T. ) ;
#51380=CARTESIAN_POINT ( 'NONE',  ( -82.67254833784559764, -183.6283474603465606, -120.2323164553484105 ) ) ;
#51381=LINE ( 'NONE', #11149, #25946 ) ;
#51382=EDGE_LOOP ( 'NONE', ( #9236, #934, #39309, #4120 ) ) ;
#51383=CARTESIAN_POINT ( 'NONE',  ( -120.2975302769383177, -183.6283474603465606, 102.3089288139534005 ) ) ;
#51387=CARTESIAN_POINT ( 'NONE',  ( -167.1580984288390823, -193.5000000000000000, -39.24667733211878584 ) ) ;
#51389=AXIS2_PLACEMENT_3D ( 'NONE', #28741, #37157, #41106 ) ;
#51391=CARTESIAN_POINT ( 'NONE',  ( -48.41988612361515010, -189.7472609257535510, 0.9982437317643287900 ) ) ;
#51393=CARTESIAN_POINT ( 'NONE',  ( -117.6201219941651601, -189.7472609257535510, 104.1370384486469902 ) ) ;
#51394=ADVANCED_FACE ( 'NONE', ( #13812 ), #30092, .T. ) ;
#51395=AXIS2_PLACEMENT_3D ( 'NONE', #7631, #39926, #23651 ) ;
#51396=EDGE_CURVE ( 'NONE', #50209, #512, #21950, .T. ) ;
#51397=CARTESIAN_POINT ( 'NONE',  ( -0.6536498292959314060, -183.6283474603465606, 114.4068333132749160 ) ) ;
#51398=VERTEX_POINT ( 'NONE', #36948 ) ;
#51400=CARTESIAN_POINT ( 'NONE',  ( -152.3176060415594861, -183.6283474603465606, -69.58857822034966034 ) ) ;
#51401=DIRECTION ( 'NONE',  ( -0.000000000000000000, 1.000000000000000000, -0.000000000000000000 ) ) ;
#51402=EDGE_LOOP ( 'NONE', ( #47282, #22923, #7102, #29405 ) ) ;
#51403=ORIENTED_EDGE ( 'NONE', *, *, #41074, .T. ) ;
#51404=LINE ( 'NONE', #35098, #11176 ) ;
#51408=AXIS2_PLACEMENT_3D ( 'NONE', #3090, #7042, #19132 ) ;
#51409=VECTOR ( 'NONE', #29818, 999.9999999999998863 ) ;
#51411=CARTESIAN_POINT ( 'NONE',  ( -166.0019676197264005, -193.5000000000000000, 39.55227055146320225 ) ) ;
#51412=CARTESIAN_POINT ( 'NONE',  ( -84.82349129030166068, -175.3837268820161057, -119.5996955107802222 ) ) ;
#51413=VERTEX_POINT ( 'NONE', #25625 ) ;
#51414=DIRECTION ( 'NONE',  ( 0.000000000000000000, 1.000000000000000000, 0.000000000000000000 ) ) ;
#51415=EDGE_CURVE ( 'NONE', #42978, #25561, #11564, .T. ) ;
#51416=ADVANCED_FACE ( 'NONE', ( #5684 ), #939, .T. ) ;
#51417=CARTESIAN_POINT ( 'NONE',  ( -68.21229068036657850, -183.6283474603465606, -123.4325817657429809 ) ) ;
#51418=FACE_OUTER_BOUND ( 'NONE', #47586, .T. ) ;
#51419=EDGE_LOOP ( 'NONE', ( #31425, #17500, #34172, #26533 ) ) ;
#51420=EDGE_LOOP ( 'NONE', ( #20430, #2181, #43241, #16988 ) ) ;
#51421=EDGE_CURVE ( 'NONE', #22277, #6242, #37198, .T. ) ;
#51422=EDGE_LOOP ( 'NONE', ( #44307, #21340, #36408, #23971 ) ) ;
#51426=FACE_OUTER_BOUND ( 'NONE', #25941, .T. ) ;
#51429=VECTOR ( 'NONE', #14932, 1000.000000000000000 ) ;
#51431=CIRCLE ( 'NONE', #28739, 125.0000000000000000 ) ;
#51434=DIRECTION ( 'NONE',  ( -0.2920567706369694982, 0.000000000000000000, -0.9564009842765243130 ) ) ;
#51435=ORIENTED_EDGE ( 'NONE', *, *, #1130, .T. ) ;
#51437=DIRECTION ( 'NONE',  ( -0.2920567706369628924, 0.000000000000000000, -0.9564009842765264224 ) ) ;
#51438=DIRECTION ( 'NONE',  ( -0.000000000000000000, 1.000000000000000000, -0.000000000000000000 ) ) ;
#51439=DIRECTION ( 'NONE',  ( 0.9842305779475980509, 0.000000000000000000, -0.1768902751225666647 ) ) ;
#51441=ORIENTED_EDGE ( 'NONE', *, *, #47971, .F. ) ;
#51443=ORIENTED_EDGE ( 'NONE', *, *, #16609, .F. ) ;
#51444=VECTOR ( 'NONE', #33622, 1000.000000000000000 ) ;
#51446=ORIENTED_EDGE ( 'NONE', *, *, #49091, .T. ) ;
#51447=AXIS2_PLACEMENT_3D ( 'NONE', #20617, #1156, #17204 ) ;
#51448=CARTESIAN_POINT ( 'NONE',  ( -48.47912675150885065, -193.5000000000000000, -0.9999999999999931166 ) ) ;
#51449=AXIS2_PLACEMENT_3D ( 'NONE', #18691, #35471, #51791 ) ;
#51452=DIRECTION ( 'NONE',  ( -0.3482016354343995812, 0.000000000000000000, 0.9374196611341205632 ) ) ;
#51454=EDGE_LOOP ( 'NONE', ( #24394, #18339, #34877, #8046 ) ) ;
#51455=CARTESIAN_POINT ( 'NONE',  ( 32.49319223169170812, -193.5000000000000000, -95.22858582633060109 ) ) ;
#51456=LINE ( 'NONE', #35932, #39935 ) ;
#51457=LINE ( 'NONE', #14422, #47571 ) ;
#51459=DIRECTION ( 'NONE',  ( 0.000000000000000000, -1.000000000000000000, 0.000000000000000000 ) ) ;
#51460=CIRCLE ( 'NONE', #34634, 125.0000000000000000 ) ;
#51467=FACE_BOUND ( 'NONE', #5637, .T. ) ;
#51468=DIRECTION ( 'NONE',  ( -0.8455960035018311727, 0.000000000000000000, 0.5338233779647826305 ) ) ;
#51469=EDGE_LOOP ( 'NONE', ( #7186, #1949, #32537, #45401 ) ) ;
#51470=ADVANCED_FACE ( 'NONE', ( #16983 ), #37973, .T. ) ;
#51471=DIRECTION ( 'NONE',  ( 0.000000000000000000, 1.000000000000000000, 0.000000000000000000 ) ) ;
#51472=VECTOR ( 'NONE', #21594, 1000.000000000000114 ) ;
#51475=ORIENTED_EDGE ( 'NONE', *, *, #8860, .T. ) ;
#51476=CARTESIAN_POINT ( 'NONE',  ( -145.0195698084541505, -175.3837268820161057, 79.40367028273128369 ) ) ;
#51477=VECTOR ( 'NONE', #39721, 1000.000000000000114 ) ;
#51478=ORIENTED_EDGE ( 'NONE', *, *, #46397, .T. ) ;
#51481=CARTESIAN_POINT ( 'NONE',  ( -48.47912675150885065, -189.7472609257535510, 6.938893903907228378E-15 ) ) ;
#51483=LINE ( 'NONE', #52016, #46006 ) ;
#51485=VERTEX_POINT ( 'NONE', #9870 ) ;
#51486=ADVANCED_FACE ( 'NONE', ( #13018 ), #41922, .T. ) ;
#51487=CARTESIAN_POINT ( 'NONE',  ( -150.5215542367829755, -175.3837268820161057, -72.19655804061973470 ) ) ;
#51491=ORIENTED_EDGE ( 'NONE', *, *, #51268, .T. ) ;
#51493=EDGE_LOOP ( 'NONE', ( #21529, #27319, #292, #937 ) ) ;
#51494=CARTESIAN_POINT ( 'NONE',  ( -48.47912675150885065, -188.5000000000000284, 6.938893903907228378E-15 ) ) ;
#51495=CARTESIAN_POINT ( 'NONE',  ( 74.28166149629942083, -189.7472609257535510, 17.48697739784543259 ) ) ;
#51497=AXIS2_PLACEMENT_3D ( 'NONE', #14503, #6619, #51038 ) ;
#51501=DIRECTION ( 'NONE',  ( -0.000000000000000000, 1.000000000000000000, -0.000000000000000000 ) ) ;
#51502=CARTESIAN_POINT ( 'NONE',  ( -167.4530144994566285, -193.5000000000000000, -34.94873081740325205 ) ) ;
#51503=CARTESIAN_POINT ( 'NONE',  ( -48.47912675150885065, -213.5000000000000000, 6.938893903907228378E-15 ) ) ;
#51505=CYLINDRICAL_SURFACE ( 'NONE', #28053, 125.0000000000000000 ) ;
#51507=ADVANCED_FACE ( 'NONE', ( #13547 ), #38502, .T. ) ;
#51508=VECTOR ( 'NONE', #23442, 1000.000000000000000 ) ;
#51510=DIRECTION ( 'NONE',  ( 0.000000000000000000, -1.000000000000000000, 0.000000000000000000 ) ) ;
#51511=DIRECTION ( 'NONE',  ( 0.000000000000000000, 0.000000000000000000, 1.000000000000000000 ) ) ;
#51513=VECTOR ( 'NONE', #45684, 1000.000000000000000 ) ;
#51514=CARTESIAN_POINT ( 'NONE',  ( -78.00521078983979351, -193.5000000000000000, 121.4627941443857111 ) ) ;
#51517=LINE ( 'NONE', #26561, #34190 ) ;
#51520=ORIENTED_EDGE ( 'NONE', *, *, #23464, .F. ) ;
#51521=ADVANCED_FACE ( 'NONE', ( #34296 ), #2748, .F. ) ;
#51522=CARTESIAN_POINT ( 'NONE',  ( -48.47912675150885065, -177.1207230881787780, 6.938893903907228378E-15 ) ) ;
#51524=FACE_OUTER_BOUND ( 'NONE', #8826, .T. ) ;
#51525=CARTESIAN_POINT ( 'NONE',  ( 59.00260725618640123, -177.1207230881787780, -63.81752780152988436 ) ) ;
#51526=AXIS2_PLACEMENT_3D ( 'NONE', #29653, #1019, #49899 ) ;
#51535=ORIENTED_EDGE ( 'NONE', *, *, #26501, .F. ) ;
#51536=PLANE ( 'NONE',  #20002 ) ;
#51537=DIRECTION ( 'NONE',  ( 0.000000000000000000, -0.000000000000000000, -1.000000000000000000 ) ) ;
#51538=CIRCLE ( 'NONE', #34720, 125.0000000000000000 ) ;
#51544=ORIENTED_EDGE ( 'NONE', *, *, #38051, .T. ) ;
#51545=EDGE_CURVE ( 'NONE', #3888, #27923, #27170, .T. ) ;
#51549=ORIENTED_EDGE ( 'NONE', *, *, #1585, .T. ) ;
#51550=FACE_OUTER_BOUND ( 'NONE', #50093, .T. ) ;
#51552=LINE ( 'NONE', #33, #38331 ) ;
#51554=EDGE_CURVE ( 'NONE', #18044, #33019, #26676, .T. ) ;
#51555=ORIENTED_EDGE ( 'NONE', *, *, #13741, .F. ) ;
#51556=CARTESIAN_POINT ( 'NONE',  ( 12.12533326292403935, -193.5000000000000000, 109.3256576763158847 ) ) ;
#51557=LINE ( 'NONE', #44187, #32039 ) ;
#51559=DIRECTION ( 'NONE',  ( -0.000000000000000000, 1.000000000000000000, -0.000000000000000000 ) ) ;
#51560=VECTOR ( 'NONE', #10312, 1000.000000000000000 ) ;
#51562=ORIENTED_EDGE ( 'NONE', *, *, #8679, .F. ) ;
#51563=PLANE ( 'NONE',  #5814 ) ;
#51564=DIRECTION ( 'NONE',  ( -0.9473263538541876194, 0.000000000000000000, -0.3202698538628486746 ) ) ;
#51567=VERTEX_POINT ( 'NONE', #34542 ) ;
#51568=DIRECTION ( 'NONE',  ( -0.000000000000000000, -1.000000000000000000, 0.000000000000000000 ) ) ;
#51569=ORIENTED_EDGE ( 'NONE', *, *, #946, .F. ) ;
#51571=FACE_OUTER_BOUND ( 'NONE', #38024, .T. ) ;
#51572=FACE_OUTER_BOUND ( 'NONE', #38475, .T. ) ;
#51574=DIRECTION ( 'NONE',  ( -0.000000000000000000, 1.000000000000000000, -0.000000000000000000 ) ) ;
#51575=DIRECTION ( 'NONE',  ( 0.000000000000000000, 0.000000000000000000, 1.000000000000000000 ) ) ;
#51576=EDGE_CURVE ( 'NONE', #31784, #32782, #27438, .T. ) ;
#51577=AXIS2_PLACEMENT_3D ( 'NONE', #43256, #48251, #27492 ) ;
#51579=CARTESIAN_POINT ( 'NONE',  ( -70.42295845586433245, -193.5000000000000000, -123.0587999703024877 ) ) ;
#51580=DIRECTION ( 'NONE',  ( -0.000000000000000000, 1.000000000000000000, -0.000000000000000000 ) ) ;
#51582=ORIENTED_EDGE ( 'NONE', *, *, #9516, .T. ) ;
#51583=ORIENTED_EDGE ( 'NONE', *, *, #44529, .T. ) ;
#51584=CARTESIAN_POINT ( 'NONE',  ( -133.1483155860611021, -177.1207230881787780, -90.59430563621275212 ) ) ;
#51585=ADVANCED_FACE ( 'NONE', ( #42707 ), #19050, .T. ) ;
#51586=EDGE_CURVE ( 'NONE', #51869, #36336, #15789, .T. ) ;
#51588=ORIENTED_EDGE ( 'NONE', *, *, #14298, .T. ) ;
#51589=VERTEX_POINT ( 'NONE', #22207 ) ;
#51590=EDGE_CURVE ( 'NONE', #21919, #9092, #31706, .T. ) ;
#51591=DIRECTION ( 'NONE',  ( -0.3482016354343995812, 0.000000000000000000, 0.9374196611341205632 ) ) ;
#51593=CARTESIAN_POINT ( 'NONE',  ( -137.2624501260119700, -183.6283474603465606, 87.99159897727969337 ) ) ;
#51594=LINE ( 'NONE', #27926, #25825 ) ;
#51595=AXIS2_PLACEMENT_3D ( 'NONE', #8960, #41797, #24994 ) ;
#51598=DIRECTION ( 'NONE',  ( 0.000000000000000000, 1.000000000000000000, 0.000000000000000000 ) ) ;
#51599=CARTESIAN_POINT ( 'NONE',  ( -168.6933499419502880, -177.1207230881787780, 30.40954281680879845 ) ) ;
#51600=VERTEX_POINT ( 'NONE', #30875 ) ;
#51601=ORIENTED_EDGE ( 'NONE', *, *, #51732, .T. ) ;
#51602=CIRCLE ( 'NONE', #27242, 125.0000000000000000 ) ;
#51603=VERTEX_POINT ( 'NONE', #14862 ) ;
#51604=CARTESIAN_POINT ( 'NONE',  ( -48.64924157374594671, -193.5000000000000000, 124.9998842437354227 ) ) ;
#51605=DIRECTION ( 'NONE',  ( 0.000000000000000000, 0.000000000000000000, 1.000000000000000000 ) ) ;
#51606=DIRECTION ( 'NONE',  ( -0.4031234292879730674, 0.000000000000000000, 0.9151456172430181280 ) ) ;
#51607=AXIS2_PLACEMENT_3D ( 'NONE', #9217, #41254, #5281 ) ;
#51609=CARTESIAN_POINT ( 'NONE',  ( -49.17567778057184569, -177.1207230881787780, -0.7175072570443327136 ) ) ;
#51610=ORIENTED_EDGE ( 'NONE', *, *, #16616, .F. ) ;
#51611=DIRECTION ( 'NONE',  ( 0.000000000000000000, -1.000000000000000000, 0.000000000000000000 ) ) ;
#51613=VECTOR ( 'NONE', #5607, 1000.000000000000114 ) ;
#51614=CARTESIAN_POINT ( 'NONE',  ( 43.86477233319989466, -189.7472609257535510, -84.24728067915975771 ) ) ;
#51615=CARTESIAN_POINT ( 'NONE',  ( -153.2421220336517536, -175.3837268820161057, -66.33788548805449636 ) ) ;
#51617=ORIENTED_EDGE ( 'NONE', *, *, #33302, .F. ) ;
#51622=DIRECTION ( 'NONE',  ( -0.000000000000000000, 1.000000000000000000, -0.000000000000000000 ) ) ;
#51624=DIRECTION ( 'NONE',  ( 0.000000000000000000, 1.000000000000000000, -0.000000000000000000 ) ) ;
#51625=ORIENTED_EDGE ( 'NONE', *, *, #23052, .T. ) ;
#51627=VERTEX_POINT ( 'NONE', #31125 ) ;
#51629=FACE_BOUND ( 'NONE', #32671, .T. ) ;
#51632=DIRECTION ( 'NONE',  ( 0.000000000000000000, 0.000000000000000000, -1.000000000000000000 ) ) ;
#51634=AXIS2_PLACEMENT_3D ( 'NONE', #44387, #4179, #15489 ) ;
#51635=VECTOR ( 'NONE', #37931, 1000.000000000000000 ) ;
#51636=EDGE_CURVE ( 'NONE', #6855, #10180, #43453, .T. ) ;
#51638=EDGE_CURVE ( 'NONE', #26450, #44661, #47417, .T. ) ;
#51639=FACE_OUTER_BOUND ( 'NONE', #30570, .T. ) ;
#51640=DIRECTION ( 'NONE',  ( 0.000000000000000000, -1.000000000000000000, -0.000000000000000000 ) ) ;
#51641=EDGE_CURVE ( 'NONE', #43457, #22526, #14331, .T. ) ;
#51643=AXIS2_PLACEMENT_3D ( 'NONE', #2772, #23008, #42975 ) ;
#51644=EDGE_CURVE ( 'NONE', #15404, #17350, #16674, .T. ) ;
#51645=VERTEX_POINT ( 'NONE', #27696 ) ;
#51646=DIRECTION ( 'NONE',  ( -0.9646355819083614058, 0.000000000000000000, 0.2635871660690581320 ) ) ;
#51647=ORIENTED_EDGE ( 'NONE', *, *, #50690, .F. ) ;
#51649=EDGE_CURVE ( 'NONE', #35024, #16698, #11670, .T. ) ;
#51651=DIRECTION ( 'NONE',  ( 0.000000000000000000, 1.000000000000000000, -0.000000000000000000 ) ) ;
#51656=ORIENTED_EDGE ( 'NONE', *, *, #22554, .F. ) ;
#51657=DIRECTION ( 'NONE',  ( 0.000000000000000000, 1.000000000000000000, 0.000000000000000000 ) ) ;
#51660=EDGE_CURVE ( 'NONE', #25409, #28008, #654, .T. ) ;
#51662=CARTESIAN_POINT ( 'NONE',  ( 13.86276369408136411, -193.5000000000000000, -107.1890582354654669 ) ) ;
#51663=ORIENTED_EDGE ( 'NONE', *, *, #47130, .F. ) ;
#51664=ADVANCED_FACE ( 'NONE', ( #47692 ), #24531, .T. ) ;
#51665=CARTESIAN_POINT ( 'NONE',  ( -103.4012653778457320, -183.6283474603465606, -112.2878385610366649 ) ) ;
#51666=DIRECTION ( 'NONE',  ( 0.000000000000000000, -1.000000000000000000, 0.000000000000000000 ) ) ;
#51668=FACE_OUTER_BOUND ( 'NONE', #34948, .T. ) ;
#51671=LINE ( 'NONE', #39037, #22739 ) ;
#51672=CARTESIAN_POINT ( 'NONE',  ( -49.13194886969936448, -193.5000000000000000, -0.7575112421616214675 ) ) ;
#51673=ORIENTED_EDGE ( 'NONE', *, *, #26528, .T. ) ;
#51675=ADVANCED_FACE ( 'NONE', ( #47939 ), #16400, .T. ) ;
#51676=ORIENTED_EDGE ( 'NONE', *, *, #40714, .T. ) ;
#51678=PLANE ( 'NONE',  #42792 ) ;
#51679=VECTOR ( 'NONE', #34746, 1000.000000000000000 ) ;
#51680=DIRECTION ( 'NONE',  ( 0.9646355819083556327, 0.000000000000000000, 0.2635871660690782825 ) ) ;
#51681=CIRCLE ( 'NONE', #34039, 125.0000000000000000 ) ;
#51682=DIRECTION ( 'NONE',  ( -0.8455960035018234011, 0.000000000000000000, -0.5338233779647948429 ) ) ;
#51683=DIRECTION ( 'NONE',  ( 0.8294056854501971054, 0.000000000000000000, 0.5586467658036594619 ) ) ;
#51687=LINE ( 'NONE', #15688, #20721 ) ;
#51688=ORIENTED_EDGE ( 'NONE', *, *, #27130, .F. ) ;
#51689=PLANE ( 'NONE',  #16429 ) ;
#51690=ORIENTED_EDGE ( 'NONE', *, *, #48156, .T. ) ;
#51692=LINE ( 'NONE', #40104, #11514 ) ;
#51693=CARTESIAN_POINT ( 'NONE',  ( -160.7804753152582293, -189.7472609257535510, -52.57768177182448710 ) ) ;
#51694=DIRECTION ( 'NONE',  ( -0.000000000000000000, 1.000000000000000000, -0.000000000000000000 ) ) ;
#51695=PLANE ( 'NONE',  #12478 ) ;
#51697=DIRECTION ( 'NONE',  ( 0.000000000000000000, 1.000000000000000000, 0.000000000000000000 ) ) ;
#51698=ORIENTED_EDGE ( 'NONE', *, *, #26665, .F. ) ;
#51700=EDGE_CURVE ( 'NONE', #17596, #4, #3162, .T. ) ;
#51706=EDGE_CURVE ( 'NONE', #1891, #30689, #40030, .T. ) ;
#51707=DIRECTION ( 'NONE',  ( 0.000000000000000000, 1.000000000000000000, 0.000000000000000000 ) ) ;
#51708=LINE ( 'NONE', #7556, #3556 ) ;
#51709=EDGE_CURVE ( 'NONE', #31952, #2646, #4054, .T. ) ;
#51712=CARTESIAN_POINT ( 'NONE',  ( -49.40581635894069024, -177.1207230881787780, 0.3758275821142362250 ) ) ;
#51713=EDGE_CURVE ( 'NONE', #9367, #5804, #12174, .T. ) ;
#51714=FACE_BOUND ( 'NONE', #51402, .T. ) ;
#51715=ORIENTED_EDGE ( 'NONE', *, *, #31701, .F. ) ;
#51718=CARTESIAN_POINT ( 'NONE',  ( 57.66105628977221187, -189.7472609257535510, 66.02470404298190942 ) ) ;
#51719=AXIS2_PLACEMENT_3D ( 'NONE', #38883, #46277, #50476 ) ;
#51720=VECTOR ( 'NONE', #30811, 1000.000000000000000 ) ;
#51721=CARTESIAN_POINT ( 'NONE',  ( 26.52087324849106054, -198.5000000000000000, -70.00000000000002842 ) ) ;
#51722=ORIENTED_EDGE ( 'NONE', *, *, #842, .F. ) ;
#51725=CARTESIAN_POINT ( 'NONE',  ( -157.5429198988176438, -193.5000000000000000, 61.07445476073480961 ) ) ;
#51727=FACE_BOUND ( 'NONE', #36940, .T. ) ;
#51729=CARTESIAN_POINT ( 'NONE',  ( -52.47502265695594303, -183.6283474603465606, -123.9361149384469627 ) ) ;
#51731=VECTOR ( 'NONE', #12583, 1000.000000000000000 ) ;
#51732=EDGE_CURVE ( 'NONE', #12493, #50437, #33413, .T. ) ;
#51735=ORIENTED_EDGE ( 'NONE', *, *, #44228, .F. ) ;
#51737=ORIENTED_EDGE ( 'NONE', *, *, #50589, .F. ) ;
#51738=VECTOR ( 'NONE', #16521, 1000.000000000000000 ) ;
#51741=DIRECTION ( 'NONE',  ( 0.000000000000000000, -1.000000000000000000, 0.000000000000000000 ) ) ;
#51744=PLANE ( 'NONE',  #23917 ) ;
#51746=CARTESIAN_POINT ( 'NONE',  ( 70.19984492582109681, -193.5000000000000000, 39.24667733211968823 ) ) ;
#51747=DIRECTION ( 'NONE',  ( 0.9890401873221633666, 0.000000000000000000, 0.1476465640024850756 ) ) ;
#51748=ORIENTED_EDGE ( 'NONE', *, *, #42488, .T. ) ;
#51749=VECTOR ( 'NONE', #41938, 1000.000000000000000 ) ;
#51750=ORIENTED_EDGE ( 'NONE', *, *, #8646, .F. ) ;
#51751=VECTOR ( 'NONE', #21387, 999.9999999999998863 ) ;
#51752=DIRECTION ( 'NONE',  ( 0.000000000000000000, 0.000000000000000000, -1.000000000000000000 ) ) ;
#51753=EDGE_LOOP ( 'NONE', ( #11728, #8492, #6171, #32986 ) ) ;
#51755=VERTEX_POINT ( 'NONE', #17176 ) ;
#51756=CIRCLE ( 'NONE', #8947, 125.0000000000000000 ) ;
#51757=LINE ( 'NONE', #15768, #50245 ) ;
#51761=VERTEX_POINT ( 'NONE', #37133 ) ;
#51763=VERTEX_POINT ( 'NONE', #33194 ) ;
#51766=CARTESIAN_POINT ( 'NONE',  ( -148.0127667507368585, -193.5000000000000000, -75.61781872352626976 ) ) ;
#51767=AXIS2_PLACEMENT_3D ( 'NONE', #44402, #8388, #19686 ) ;
#51768=CARTESIAN_POINT ( 'NONE',  ( 24.07160180756802248, -183.6283474603465606, 100.5610240384924481 ) ) ;
#51769=CARTESIAN_POINT ( 'NONE',  ( -173.2765435274470178, -177.1207230881787780, -7.113702696401505321 ) ) ;
#51770=DIRECTION ( 'NONE',  ( 0.000000000000000000, 0.000000000000000000, 1.000000000000000000 ) ) ;
#51771=AXIS2_PLACEMENT_3D ( 'NONE', #10205, #21787, #25212 ) ;
#51773=DIRECTION ( 'NONE',  ( 0.000000000000000000, -0.000000000000000000, 1.000000000000000000 ) ) ;
#51776=EDGE_CURVE ( 'NONE', #40054, #43244, #41334, .T. ) ;
#51778=CIRCLE ( 'NONE', #9788, 125.0000000000000000 ) ;
#51780=CARTESIAN_POINT ( 'NONE',  ( -26.53529504715431031, -175.3837268820161057, 123.0587999703026725 ) ) ;
#51782=DIRECTION ( 'NONE',  ( 0.9646355819083614058, 0.000000000000000000, -0.2635871660690581320 ) ) ;
#51783=ORIENTED_EDGE ( 'NONE', *, *, #46495, .T. ) ;
#51785=CARTESIAN_POINT ( 'NONE',  ( -48.24424070572787571, -193.5000000000000000, 0.9720229140804191870 ) ) ;
#51788=ORIENTED_EDGE ( 'NONE', *, *, #2368, .T. ) ;
#51789=ORIENTED_EDGE ( 'NONE', *, *, #34796, .T. ) ;
#51791=DIRECTION ( 'NONE',  ( 0.000000000000000000, 0.000000000000000000, -1.000000000000000000 ) ) ;
#51795=CARTESIAN_POINT ( 'NONE',  ( -170.2837019307126809, -183.6283474603465606, 23.23456943914128203 ) ) ;
#51796=CARTESIAN_POINT ( 'NONE',  ( -102.5006284722403933, -183.6283474603465606, -112.7238987608084670 ) ) ;
#51798=VERTEX_POINT ( 'NONE', #4837 ) ;
#51801=ORIENTED_EDGE ( 'NONE', *, *, #21090, .T. ) ;
#51802=CIRCLE ( 'NONE', #38395, 125.0000000000000000 ) ;
#51805=VERTEX_POINT ( 'NONE', #37664 ) ;
#51806=LINE ( 'NONE', #19462, #25896 ) ;
#51807=CIRCLE ( 'NONE', #4801, 125.0000000000000000 ) ;
#51814=CYLINDRICAL_SURFACE ( 'NONE', #27487, 125.0000000000000000 ) ;
#51815=PLANE ( 'NONE',  #41743 ) ;
#51817=CARTESIAN_POINT ( 'NONE',  ( -115.7878797639662025, -183.6283474603465606, -104.1428419024399687 ) ) ;
#51818=EDGE_LOOP ( 'NONE', ( #22605, #21629, #13653, #46466 ) ) ;
#51819=DIRECTION ( 'NONE',  ( -0.8124868780056742068, 0.000000000000000000, -0.5829794791144820021 ) ) ;
#51820=EDGE_LOOP ( 'NONE', ( #46879, #31165, #30314, #28742 ) ) ;
#51821=CARTESIAN_POINT ( 'NONE',  ( -25.55153130240594450, -175.3837268820161057, 122.8793122007210741 ) ) ;
#51822=DIRECTION ( 'NONE',  ( 0.8455960035018311727, 0.000000000000000000, -0.5338233779647826305 ) ) ;
#51823=CARTESIAN_POINT ( 'NONE',  ( -48.47912675150885065, -175.3837268820161057, 6.938893903907228378E-15 ) ) ;
#51824=FACE_OUTER_BOUND ( 'NONE', #21685, .T. ) ;
#51825=ORIENTED_EDGE ( 'NONE', *, *, #31719, .T. ) ;
#51826=EDGE_CURVE ( 'NONE', #10561, #39220, #29255, .T. ) ;
#51828=CIRCLE ( 'NONE', #10663, 125.0000000000000000 ) ;
#51829=DIRECTION ( 'NONE',  ( 0.9027978299657477557, 0.000000000000000000, -0.4300652022765115712 ) ) ;
#51830=CIRCLE ( 'NONE', #30023, 125.0000000000000000 ) ;
#51832=ORIENTED_EDGE ( 'NONE', *, *, #25336, .T. ) ;
#51833=CARTESIAN_POINT ( 'NONE',  ( -106.4764934152196645, -193.5000000000000000, 110.7307791902283043 ) ) ;
#51835=VECTOR ( 'NONE', #4881, 1000.000000000000114 ) ;
#51836=DIRECTION ( 'NONE',  ( -0.05924062789372142729, 0.000000000000000000, 0.9982437317643209074 ) ) ;
#51837=ORIENTED_EDGE ( 'NONE', *, *, #15114, .F. ) ;
#51838=EDGE_CURVE ( 'NONE', #44335, #27341, #9883, .T. ) ;
#51839=DIRECTION ( 'NONE',  ( 0.000000000000000000, 0.000000000000000000, 1.000000000000000000 ) ) ;
#51841=ORIENTED_EDGE ( 'NONE', *, *, #13221, .F. ) ;
#51844=VECTOR ( 'NONE', #42413, 1000.000000000000000 ) ;
#51845=ADVANCED_FACE ( 'NONE', ( #9035 ), #29506, .T. ) ;
#51846=CARTESIAN_POINT ( 'NONE',  ( -157.5429198988176438, -189.7472609257535510, 61.07445476073480961 ) ) ;
#51848=CARTESIAN_POINT ( 'NONE',  ( -55.65514169787639531, -193.5000000000000000, -123.7921848946937473 ) ) ;
#51849=AXIS2_PLACEMENT_3D ( 'NONE', #49569, #34038, #6712 ) ;
#51852=DIRECTION ( 'NONE',  ( -0.000000000000000000, 1.000000000000000000, -0.000000000000000000 ) ) ;
#51858=EDGE_CURVE ( 'NONE', #43700, #39182, #47662, .T. ) ;
#51859=LINE ( 'NONE', #31339, #34774 ) ;
#51860=CARTESIAN_POINT ( 'NONE',  ( 75.02564229359539638, -175.3837268820161057, -19.27620354518635182 ) ) ;
#51861=ORIENTED_EDGE ( 'NONE', *, *, #28856, .T. ) ;
#51862=ORIENTED_EDGE ( 'NONE', *, *, #26783, .T. ) ;
#51864=DIRECTION ( 'NONE',  ( 0.4566292373937140270, 0.000000000000000000, -0.8896570909947467687 ) ) ;
#51866=VECTOR ( 'NONE', #40545, 1000.000000000000000 ) ;
#51867=CIRCLE ( 'NONE', #6554, 125.0000000000000000 ) ;
#51868=ORIENTED_EDGE ( 'NONE', *, *, #447, .T. ) ;
#51869=VERTEX_POINT ( 'NONE', #9808 ) ;
#51870=DIRECTION ( 'NONE',  ( -0.000000000000000000, 1.000000000000000000, -0.000000000000000000 ) ) ;
#51871=DIRECTION ( 'NONE',  ( 0.000000000000000000, 1.000000000000000000, -0.000000000000000000 ) ) ;
#51872=AXIS2_PLACEMENT_3D ( 'NONE', #7948, #31615, #40520 ) ;
#51873=CARTESIAN_POINT ( 'NONE',  ( -165.7578939544008847, -177.1207230881787780, -43.25148278810626579 ) ) ;
#51876=ORIENTED_EDGE ( 'NONE', *, *, #17462, .F. ) ;
#51877=EDGE_LOOP ( 'NONE', ( #28491, #13105, #11087, #5589 ) ) ;
#51878=CARTESIAN_POINT ( 'NONE',  ( 47.91692961953209107, -189.7472609257535510, -77.99872144864700374 ) ) ;
#51879=CARTESIAN_POINT ( 'NONE',  ( 72.14504940832448199, -189.7472609257535510, -32.78426643622660919 ) ) ;
#51880=AXIS2_PLACEMENT_3D ( 'NONE', #18884, #3117, #39107 ) ;
#51881=CARTESIAN_POINT ( 'NONE',  ( 36.84288420123323249, -193.5000000000000000, 91.35181687837503262 ) ) ;
#51882=PLANE ( 'NONE',  #9427 ) ;
#51885=CARTESIAN_POINT ( 'NONE',  ( -70.58093260035836636, -175.3837268820161057, 122.0143860769388766 ) ) ;
#51886=EDGE_CURVE ( 'NONE', #38808, #779, #12953, .T. ) ;
#51887=EDGE_CURVE ( 'NONE', #5285, #24408, #29763, .T. ) ;
#51888=CARTESIAN_POINT ( 'NONE',  ( 62.59443091842027940, -193.5000000000000000, -57.33816169485140790 ) ) ;
#51889=DIRECTION ( 'NONE',  ( -0.000000000000000000, 1.000000000000000000, -0.000000000000000000 ) ) ;
#51890=AXIS2_PLACEMENT_3D ( 'NONE', #25249, #9227, #9481 ) ;
#51891=EDGE_CURVE ( 'NONE', #39380, #4089, #49240, .T. ) ;
#51892=VERTEX_POINT ( 'NONE', #25564 ) ;
#51894=EDGE_LOOP ( 'NONE', ( #11191, #21500, #34461, #48789 ) ) ;
#51895=FACE_OUTER_BOUND ( 'NONE', #43494, .T. ) ;
#51896=CARTESIAN_POINT ( 'NONE',  ( -4.176930889631405464, -189.7472609257535510, 116.8859077982279615 ) ) ;
#51897=VERTEX_POINT ( 'NONE', #5096 ) ;
#51899=CARTESIAN_POINT ( 'NONE',  ( 37.99238433767461487, -193.5000000000000000, -90.26448786734027863 ) ) ;
#51903=CARTESIAN_POINT ( 'NONE',  ( -48.47912675150885065, -175.3837268820161057, 6.938893903907228378E-15 ) ) ;
#51904=EDGE_CURVE ( 'NONE', #34663, #40286, #1125, .T. ) ;
#51906=EDGE_LOOP ( 'NONE', ( #22570, #21049, #39595, #28588 ) ) ;
#51908=FACE_OUTER_BOUND ( 'NONE', #51877, .T. ) ;
#51909=AXIS2_PLACEMENT_3D ( 'NONE', #47105, #18986, #10323 ) ;
#51911=EDGE_CURVE ( 'NONE', #43506, #16176, #23350, .T. ) ;
#51913=EDGE_CURVE ( 'NONE', #39607, #18605, #24796, .T. ) ;
#51915=EDGE_LOOP ( 'NONE', ( #30364, #39659, #51933, #1581 ) ) ;
#51918=FACE_OUTER_BOUND ( 'NONE', #51191, .T. ) ;
#51920=FACE_OUTER_BOUND ( 'NONE', #51454, .T. ) ;
#51921=ORIENTED_EDGE ( 'NONE', *, *, #6979, .F. ) ;
#51922=DIRECTION ( 'NONE',  ( 0.000000000000000000, -0.000000000000000000, 1.000000000000000000 ) ) ;
#51925=VECTOR ( 'NONE', #9991, 1000.000000000000000 ) ;
#51927=DIRECTION ( 'NONE',  ( -0.000000000000000000, 1.000000000000000000, 0.000000000000000000 ) ) ;
#51928=EDGE_LOOP ( 'NONE', ( #19350, #13720, #44009, #41920 ) ) ;
#51929=VERTEX_POINT ( 'NONE', #38436 ) ;
#51932=LINE ( 'NONE', #15920, #36921 ) ;
#51933=ORIENTED_EDGE ( 'NONE', *, *, #44164, .T. ) ;
#51934=DIRECTION ( 'NONE',  ( -0.000000000000000000, 1.000000000000000000, -0.000000000000000000 ) ) ;
#51937=DIRECTION ( 'NONE',  ( 0.000000000000000000, 0.000000000000000000, -1.000000000000000000 ) ) ;
#51940=DIRECTION ( 'NONE',  ( 0.6300878435817038881, 0.000000000000000000, 0.7765238627180482966 ) ) ;
#51941=EDGE_LOOP ( 'NONE', ( #791, #35078, #1592, #11927 ) ) ;
#51943=ORIENTED_EDGE ( 'NONE', *, *, #51838, .F. ) ;
#51947=AXIS2_PLACEMENT_3D ( 'NONE', #41087, #25568, #1672 ) ;
#51949=FACE_OUTER_BOUND ( 'NONE', #49407, .T. ) ;
#51951=CARTESIAN_POINT ( 'NONE',  ( 48.06131630543706024, -189.7472609257535510, -79.40367028273054473 ) ) ;
#51952=ORIENTED_EDGE ( 'NONE', *, *, #20788, .T. ) ;
#51954=EDGE_CURVE ( 'NONE', #1774, #11977, #42640, .T. ) ;
#51955=ADVANCED_FACE ( 'NONE', ( #46590 ), #34485, .T. ) ;
#51956=EDGE_CURVE ( 'NONE', #4337, #43203, #2174, .T. ) ;
#51958=ORIENTED_EDGE ( 'NONE', *, *, #2875, .T. ) ;
#51959=LINE ( 'NONE', #48254, #15559 ) ;
#51961=VECTOR ( 'NONE', #44876, 999.9999999999998863 ) ;
#51962=EDGE_LOOP ( 'NONE', ( #7029, #39836, #12728, #8356 ) ) ;
#51963=CARTESIAN_POINT ( 'NONE',  ( -48.64924157374596092, -189.7472609257535510, 123.9998842437354227 ) ) ;
#51965=CARTESIAN_POINT ( 'NONE',  ( -48.47912675150885065, -189.7472609257535510, 6.938893903907228378E-15 ) ) ;
#51966=DIRECTION ( 'NONE',  ( -0.000000000000000000, -1.000000000000000000, 0.000000000000000000 ) ) ;
#51967=FACE_OUTER_BOUND ( 'NONE', #33471, .T. ) ;
#51972=EDGE_CURVE ( 'NONE', #28974, #39629, #43491, .T. ) ;
#51975=LINE ( 'NONE', #19375, #49733 ) ;
#51976=EDGE_CURVE ( 'NONE', #16698, #25045, #38163, .T. ) ;
#51977=FACE_OUTER_BOUND ( 'NONE', #21687, .T. ) ;
#51978=CARTESIAN_POINT ( 'NONE',  ( -48.47912675150885065, -183.6283474603465606, 6.938893903907228378E-15 ) ) ;
#51979=CARTESIAN_POINT ( 'NONE',  ( 141.7825277784304205, -213.5000000000000000, -9.999999999999987566 ) ) ;
#51980=ADVANCED_FACE ( 'NONE', ( #43145 ), #35259, .T. ) ;
#51981=DIRECTION ( 'NONE',  ( -0.8124868780056742068, 0.000000000000000000, -0.5829794791144820021 ) ) ;
#51983=ORIENTED_EDGE ( 'NONE', *, *, #6272, .T. ) ;
#51984=CARTESIAN_POINT ( 'NONE',  ( 64.44365795514079309, -189.7472609257535510, -53.60452120946192878 ) ) ;
#51985=PLANE ( 'NONE',  #38302 ) ;
#51986=FACE_BOUND ( 'NONE', #16748, .T. ) ;
#51989=DIRECTION ( 'NONE',  ( -0.9929810960135169173, 0.000000000000000000, -0.1182731709213660498 ) ) ;
#51992=VERTEX_POINT ( 'NONE', #6652 ) ;
#51993=CARTESIAN_POINT ( 'NONE',  ( 60.90550954139437323, -189.7472609257535510, 60.49794494914088006 ) ) ;
#51995=ADVANCED_FACE ( 'NONE', ( #46335 ), #26605, .F. ) ;
#51996=DIRECTION ( 'NONE',  ( 0.000000000000000000, 0.000000000000000000, 1.000000000000000000 ) ) ;
#51997=FACE_BOUND ( 'NONE', #8635, .T. ) ;
#51998=DIRECTION ( 'NONE',  ( -0.000000000000000000, 1.000000000000000000, -0.000000000000000000 ) ) ;
#51999=LINE ( 'NONE', #44611, #24384 ) ;
#52000=ORIENTED_EDGE ( 'NONE', *, *, #43212, .F. ) ;
#52005=ORIENTED_EDGE ( 'NONE', *, *, #49702, .T. ) ;
#52006=DIRECTION ( 'NONE',  ( -0.7175072570443299380, 0.000000000000000000, -0.6965510290629983725 ) ) ;
#52008=EDGE_CURVE ( 'NONE', #21927, #40700, #26715, .T. ) ;
#52009=EDGE_CURVE ( 'NONE', #5680, #42978, #42369, .T. ) ;
#52010=EDGE_CURVE ( 'NONE', #13886, #39193, #2443, .T. ) ;
#52013=CARTESIAN_POINT ( 'NONE',  ( -56.71246971489870958, -175.3837268820161057, -124.7285535218267540 ) ) ;
#52016=CARTESIAN_POINT ( 'NONE',  ( -0.3054481938615516423, -193.5000000000000000, 115.3442529744090450 ) ) ;
#52017=CARTESIAN_POINT ( 'NONE',  ( -156.9880281022168447, -175.3837268820161057, -60.01515274640934905 ) ) ;
#52018=ORIENTED_EDGE ( 'NONE', *, *, #14962, .F. ) ;
#52019=ORIENTED_EDGE ( 'NONE', *, *, #2875, .F. ) ;
#52020=AXIS2_PLACEMENT_3D ( 'NONE', #44606, #4660, #20688 ) ;
#52021=ADVANCED_FACE ( 'NONE', ( #3220 ), #19250, .F. ) ;
#52022=DIRECTION ( 'NONE',  ( -0.000000000000000000, 1.000000000000000000, 0.000000000000000000 ) ) ;
#52023=ORIENTED_EDGE ( 'NONE', *, *, #2418, .F. ) ;
#52024=CARTESIAN_POINT ( 'NONE',  ( -49.29161362951452929, -175.3837268820161057, -0.5829794791144748967 ) ) ;
#52025=EDGE_LOOP ( 'NONE', ( #39500, #24118, #29609, #14397 ) ) ;
#52026=FACE_OUTER_BOUND ( 'NONE', #1548, .T. ) ;
#52027=VERTEX_POINT ( 'NONE', #51309 ) ;
#52029=FACE_OUTER_BOUND ( 'NONE', #45931, .T. ) ;
#52031=ORIENTED_EDGE ( 'NONE', *, *, #26130, .F. ) ;
#52032=ADVANCED_FACE ( 'NONE', ( #36041 ), #43668, .F. ) ;
#52036=EDGE_CURVE ( 'NONE', #50002, #45115, #39283, .T. ) ;
#52037=CARTESIAN_POINT ( 'NONE',  ( 76.01188277843579044, -193.5000000000000000, 11.26891947860284482 ) ) ;
#52038=LINE ( 'NONE', #8387, #8916 ) ;
#52039=CARTESIAN_POINT ( 'NONE',  ( -238.7407812814481076, -213.5000000000000000, 10.00000000000000178 ) ) ;
ENDSEC;
END-ISO-10303-21;
